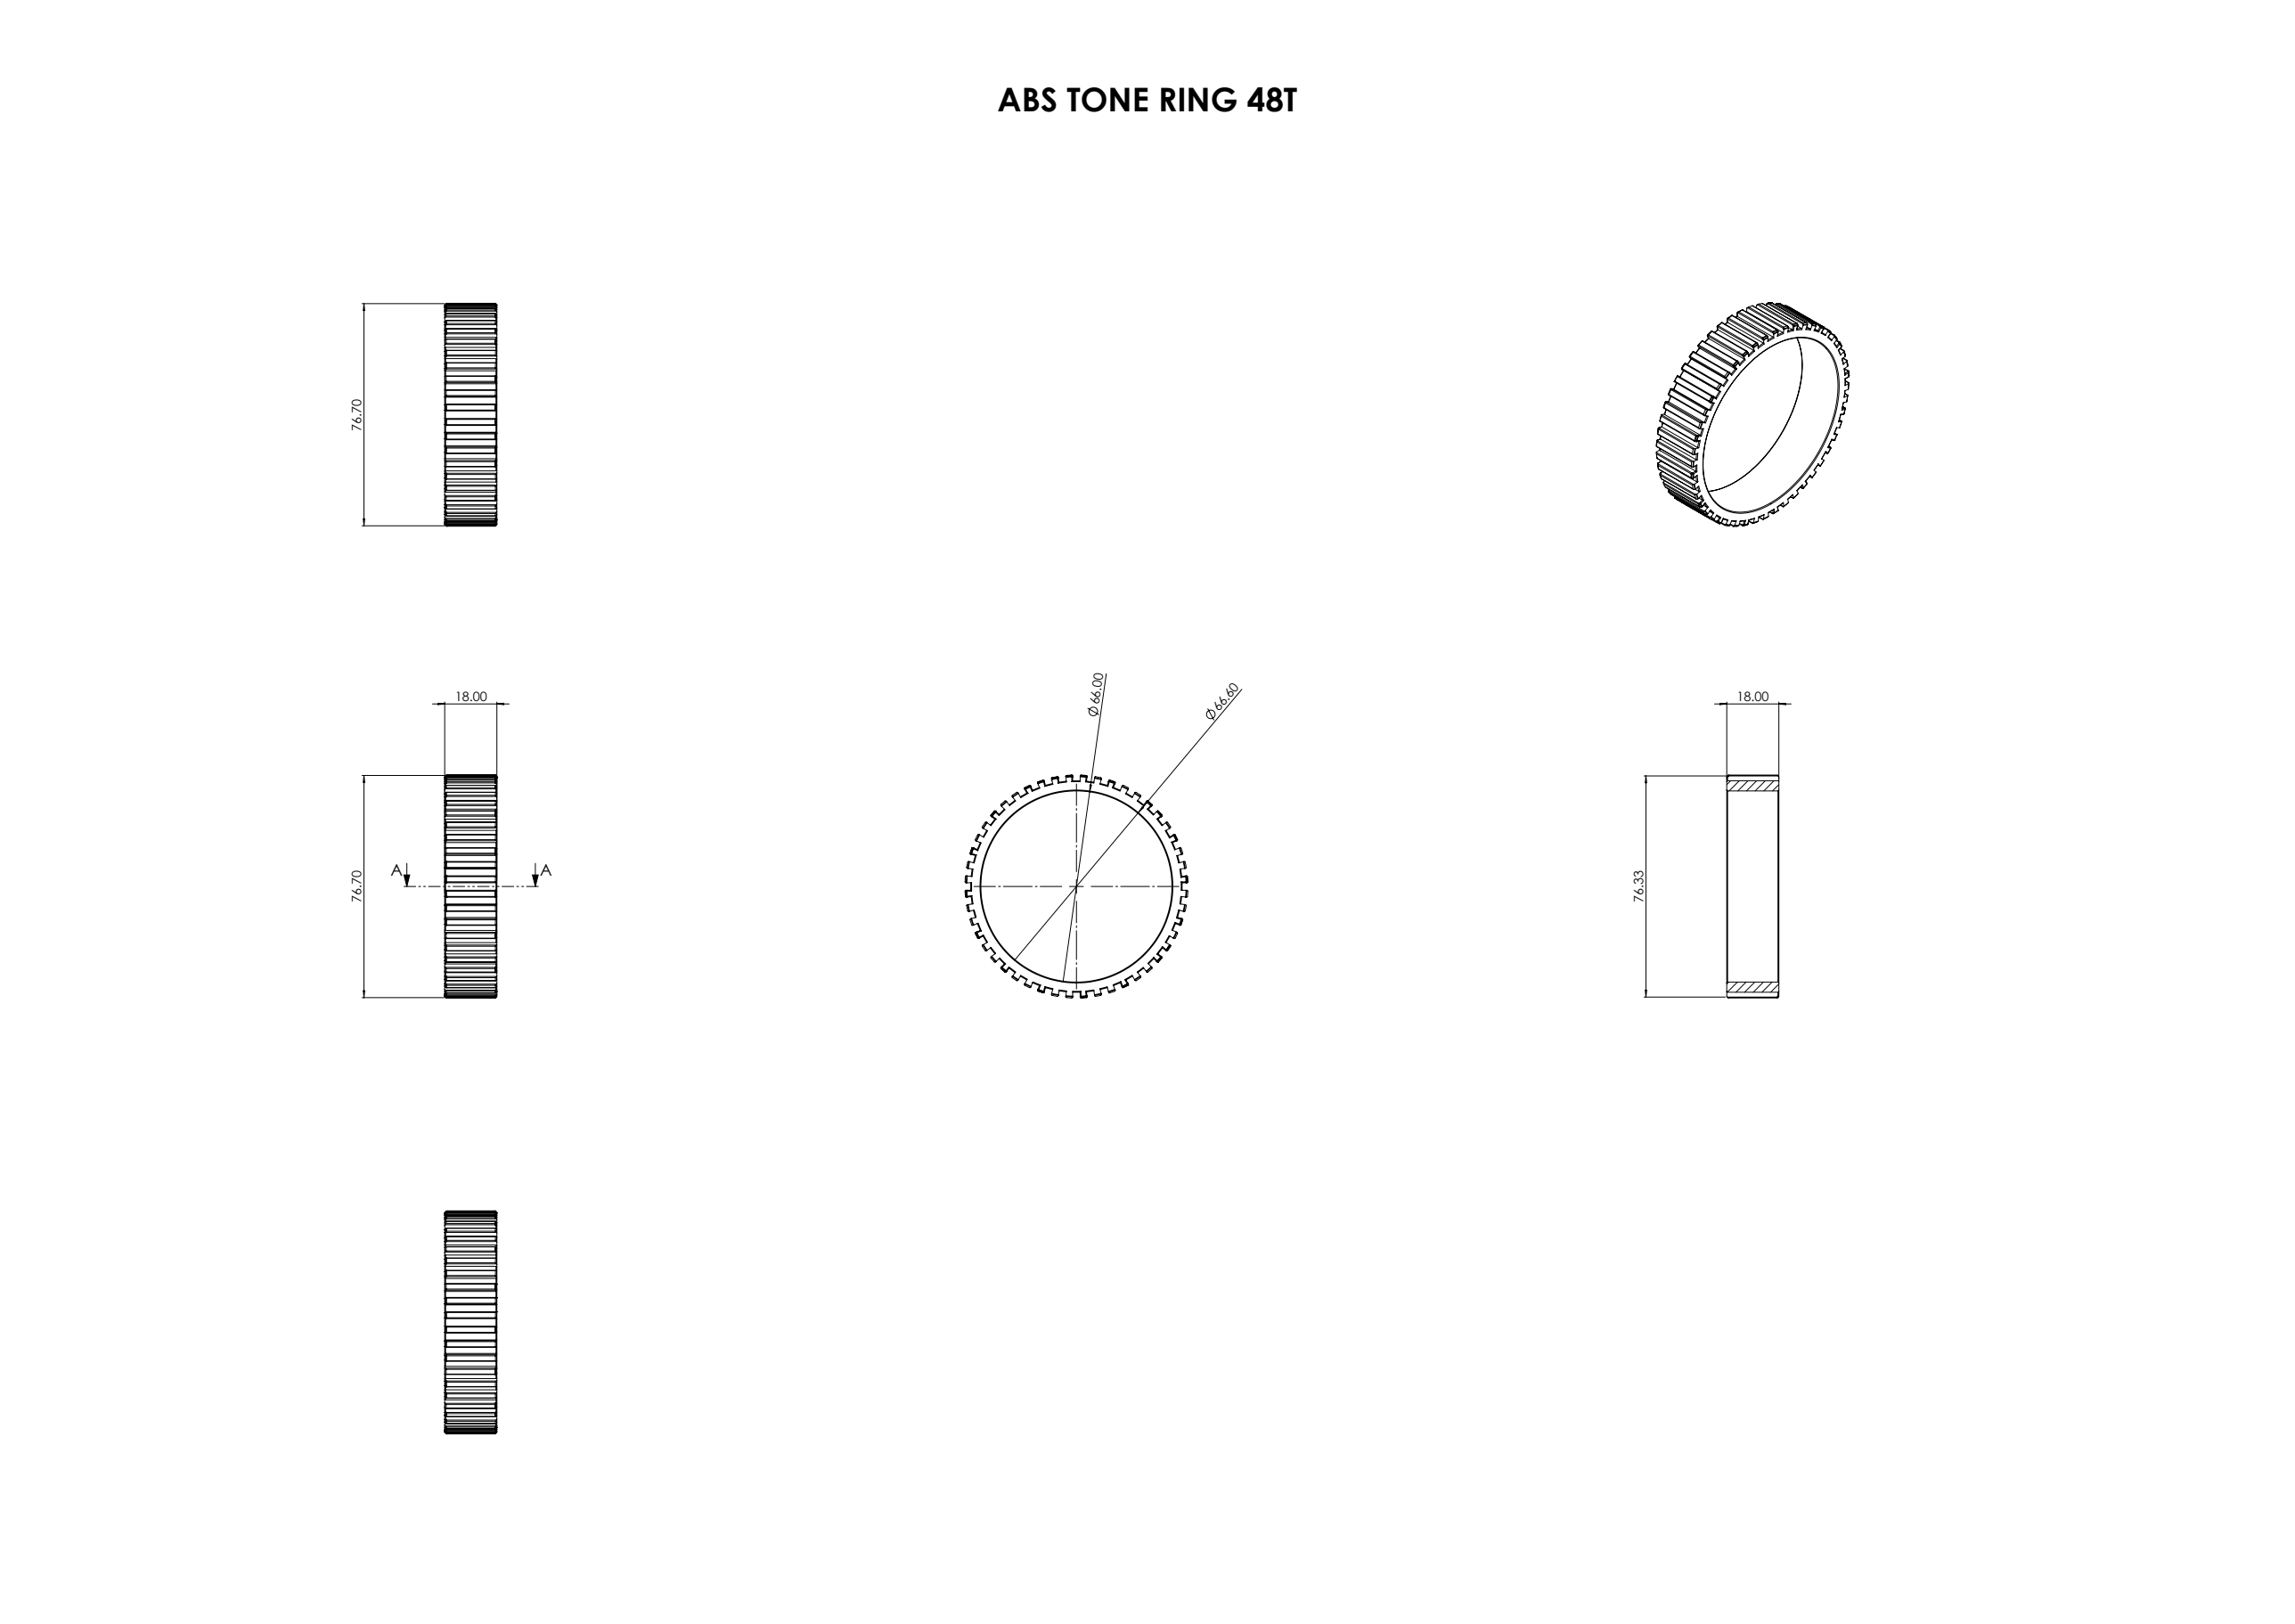
ISO-10303-21;
HEADER;
/* Generated by software containing ST-Developer
 * from STEP Tools, Inc. (www.steptools.com) 
 */

FILE_DESCRIPTION(
/* description */ (''),
/* implementation_level */ '2;1');

FILE_NAME(
/* name */ '02_ABS_Tone_Ring_48T.step',
/* time_stamp */ '2026-10-11T12:57:03-07:00',
/* author */ (''),
/* organization */ (''),
/* preprocessor_version */ 'ST-DEVELOPER v20.2',
/* originating_system */ 'Autodesk Translation Framework v15.15.0.0',
/* authorisation */ '');

FILE_SCHEMA (('AUTOMOTIVE_DESIGN { 1 0 10303 214 3 1 1 }'));
ENDSEC;

DATA;
#10=MECHANICAL_DESIGN_GEOMETRIC_PRESENTATION_REPRESENTATION('',(#257),#90374);
#111=ELLIPSE('',#40907,0.424264068711926,0.3);
#112=ELLIPSE('',#40914,0.424264068711924,0.3);
#113=ELLIPSE('',#40992,0.424264068711927,0.3);
#114=ELLIPSE('',#40999,0.424264068711929,0.3);
#115=ELLIPSE('',#41027,0.42426406871193,0.3);
#116=ELLIPSE('',#41034,0.424264068711928,0.3);
#117=ELLIPSE('',#41062,0.424264068711928,0.3);
#118=ELLIPSE('',#41077,0.424264068711929,0.3);
#119=ELLIPSE('',#41099,0.424264068711931,0.3);
#120=ELLIPSE('',#41114,0.424264068711924,0.3);
#121=ELLIPSE('',#41136,0.424264068711928,0.3);
#122=ELLIPSE('',#41205,0.424264068711926,0.3);
#123=ELLIPSE('',#41226,0.424264068711929,0.3);
#124=ELLIPSE('',#41247,0.424264068711929,0.3);
#125=ELLIPSE('',#41250,0.424264068711929,0.3);
#126=ELLIPSE('',#41280,0.424264068711931,0.3);
#127=ELLIPSE('',#41301,0.424264068711928,0.3);
#128=ELLIPSE('',#41322,0.424264068711927,0.3);
#129=ELLIPSE('',#41338,0.424264068711931,0.3);
#130=ELLIPSE('',#41341,0.424264068711928,0.3);
#131=ELLIPSE('',#41378,0.424264068711933,0.3);
#132=ELLIPSE('',#41386,0.424264068711929,0.3);
#133=ELLIPSE('',#41394,0.424264068711929,0.3);
#134=ELLIPSE('',#41417,0.424264068711928,0.3);
#135=ELLIPSE('',#41425,0.424264068711924,0.3);
#136=ELLIPSE('',#41443,0.424264068711929,0.3);
#137=ELLIPSE('',#41459,0.424264068711925,0.3);
#138=ELLIPSE('',#41468,0.424264068711925,0.3);
#139=ELLIPSE('',#41484,0.424264068711932,0.3);
#140=ELLIPSE('',#41505,0.424264068711926,0.3);
#141=ELLIPSE('',#41528,0.424264068711932,0.3);
#142=ELLIPSE('',#41536,0.424264068711931,0.3);
#143=ELLIPSE('',#41559,0.424264068711932,0.3);
#144=ELLIPSE('',#41570,0.424264068711924,0.3);
#145=ELLIPSE('',#41591,0.424264068711938,0.3);
#146=ELLIPSE('',#41612,0.424264068711929,0.3);
#147=ELLIPSE('',#41630,0.424264068711925,0.3);
#148=ELLIPSE('',#41640,0.424264068711933,0.3);
#149=ELLIPSE('',#41648,0.424264068711928,0.3);
#150=ELLIPSE('',#41671,0.424264068711924,0.3);
#151=ELLIPSE('',#41692,0.424264068711934,0.3);
#152=ELLIPSE('',#41700,0.424264068711936,0.3);
#153=ELLIPSE('',#41708,0.424264068711924,0.3);
#154=ELLIPSE('',#41726,0.424264068711933,0.3);
#155=ELLIPSE('',#41734,0.424264068711928,0.3);
#156=ELLIPSE('',#41757,0.424264068711939,0.3);
#157=ELLIPSE('',#41775,0.424264068711935,0.3);
#158=ELLIPSE('',#41784,0.424264068711927,0.3);
#159=ELLIPSE('',#41805,0.424264068711928,0.3);
#160=ELLIPSE('',#41826,0.424264068711934,0.3);
#161=ELLIPSE('',#41842,0.424264068711933,0.3);
#162=ELLIPSE('',#41865,0.424264068711929,0.3);
#163=ELLIPSE('',#41880,0.424264068711931,0.3);
#164=ELLIPSE('',#41886,0.424264068711923,0.3);
#165=ELLIPSE('',#41907,0.424264068711929,0.3);
#166=ELLIPSE('',#41925,0.424264068711927,0.3);
#167=ELLIPSE('',#41935,0.424264068711925,0.3);
#168=ELLIPSE('',#41943,0.424264068711927,0.3);
#169=ELLIPSE('',#41966,0.424264068711931,0.3);
#170=ELLIPSE('',#41977,0.424264068711927,0.3);
#171=ELLIPSE('',#41998,0.424264068711928,0.3);
#172=ELLIPSE('',#42006,0.424264068711927,0.3);
#173=ELLIPSE('',#42014,0.424264068711923,0.3);
#174=ELLIPSE('',#42037,0.42426406871193,0.3);
#175=ELLIPSE('',#42046,0.424264068711931,0.3);
#176=ELLIPSE('',#42067,0.424264068711931,0.3);
#177=ELLIPSE('',#42090,0.424264068711929,0.3);
#178=ELLIPSE('',#42098,0.424264068711927,0.3);
#179=ELLIPSE('',#42114,0.424264068711931,0.3);
#180=ELLIPSE('',#42137,0.424264068711925,0.3);
#181=ELLIPSE('',#42142,0.424264068711929,0.3);
#182=ELLIPSE('',#42165,0.424264068711925,0.3);
#183=ELLIPSE('',#42173,0.424264068711929,0.3);
#184=ELLIPSE('',#42188,0.424264068711931,0.3);
#185=ELLIPSE('',#42199,0.424264068711925,0.3);
#186=ELLIPSE('',#42209,0.424264068711925,0.3);
#187=ELLIPSE('',#42217,0.424264068711926,0.3);
#188=ELLIPSE('',#42240,0.424264068711921,0.3);
#189=ELLIPSE('',#42254,0.424264068711933,0.3);
#190=ELLIPSE('',#42275,0.424264068711929,0.3);
#191=ELLIPSE('',#42291,0.424264068711929,0.3);
#192=ELLIPSE('',#42312,0.424264068711932,0.3);
#193=ELLIPSE('',#42333,0.424264068711929,0.3);
#194=ELLIPSE('',#42356,0.424264068711932,0.3);
#195=ELLIPSE('',#42364,0.424264068711932,0.3);
#196=ELLIPSE('',#42374,0.424264068711929,0.3);
#197=ELLIPSE('',#42389,0.424264068711927,0.3);
#198=ELLIPSE('',#42404,0.424264068711929,0.3);
#199=ELLIPSE('',#42412,0.424264068711929,0.3);
#200=ELLIPSE('',#42430,0.424264068711929,0.3);
#201=ELLIPSE('',#42442,0.424264068711929,0.3);
#202=ELLIPSE('',#42454,0.424264068711927,0.3);
#203=ELLIPSE('',#42506,0.424264068711923,0.3);
#204=ELLIPSE('',#42563,0.42426406871193,0.3);
#205=ELLIPSE('',#42620,0.424264068711933,0.3);
#206=ELLIPSE('',#42643,0.424264068711929,0.3);
#207=ELLIPSE('',#42675,0.424264068711927,0.3);
#208=ELLIPSE('',#42703,0.424264068711926,0.3);
#209=ELLIPSE('',#42706,0.424264068711927,0.3);
#210=ELLIPSE('',#42748,0.42426406871193,0.3);
#223=SHAPE_REPRESENTATION_RELATIONSHIP('SRR','None',#90442,#240);
#240=ADVANCED_BREP_SHAPE_REPRESENTATION('',(#274),#90358);
#257=STYLED_ITEM('',(#90673),#274);
#274=MANIFOLD_SOLID_BREP('Body1',#40346);
#302=SPHERICAL_SURFACE('',#40910,0.3);
#303=SPHERICAL_SURFACE('',#40923,0.3);
#304=SPHERICAL_SURFACE('',#40925,0.3);
#305=SPHERICAL_SURFACE('',#40927,0.3);
#306=SPHERICAL_SURFACE('',#40995,0.3);
#307=SPHERICAL_SURFACE('',#41008,0.3);
#308=SPHERICAL_SURFACE('',#41010,0.3);
#309=SPHERICAL_SURFACE('',#41012,0.3);
#310=SPHERICAL_SURFACE('',#41030,0.3);
#311=SPHERICAL_SURFACE('',#41043,0.3);
#312=SPHERICAL_SURFACE('',#41045,0.3);
#313=SPHERICAL_SURFACE('',#41047,0.3);
#314=SPHERICAL_SURFACE('',#41065,0.3);
#315=SPHERICAL_SURFACE('',#41073,0.3);
#316=SPHERICAL_SURFACE('',#41080,0.3);
#317=SPHERICAL_SURFACE('',#41082,0.3);
#318=SPHERICAL_SURFACE('',#41102,0.3);
#319=SPHERICAL_SURFACE('',#41110,0.3);
#320=SPHERICAL_SURFACE('',#41117,0.3);
#321=SPHERICAL_SURFACE('',#41119,0.3);
#322=SPHERICAL_SURFACE('',#41139,0.3);
#323=SPHERICAL_SURFACE('',#41143,0.3);
#324=SPHERICAL_SURFACE('',#41208,0.3);
#325=SPHERICAL_SURFACE('',#41212,0.3);
#326=SPHERICAL_SURFACE('',#41229,0.3);
#327=SPHERICAL_SURFACE('',#41233,0.3);
#328=SPHERICAL_SURFACE('',#41253,0.3);
#329=SPHERICAL_SURFACE('',#41261,0.3);
#330=SPHERICAL_SURFACE('',#41265,0.3);
#331=SPHERICAL_SURFACE('',#41267,0.3);
#332=SPHERICAL_SURFACE('',#41283,0.3);
#333=SPHERICAL_SURFACE('',#41287,0.3);
#334=SPHERICAL_SURFACE('',#41304,0.3);
#335=SPHERICAL_SURFACE('',#41308,0.3);
#336=SPHERICAL_SURFACE('',#41325,0.3);
#337=SPHERICAL_SURFACE('',#41329,0.3);
#338=SPHERICAL_SURFACE('',#41344,0.3);
#339=SPHERICAL_SURFACE('',#41352,0.3);
#340=SPHERICAL_SURFACE('',#41356,0.3);
#341=SPHERICAL_SURFACE('',#41358,0.3);
#342=SPHERICAL_SURFACE('',#41374,0.3);
#343=SPHERICAL_SURFACE('',#41379,0.3);
#344=SPHERICAL_SURFACE('',#41387,0.3);
#345=SPHERICAL_SURFACE('',#41388,0.3);
#346=SPHERICAL_SURFACE('',#41397,0.3);
#347=SPHERICAL_SURFACE('',#41401,0.3);
#348=SPHERICAL_SURFACE('',#41418,0.3);
#349=SPHERICAL_SURFACE('',#41419,0.3);
#350=SPHERICAL_SURFACE('',#41428,0.3);
#351=SPHERICAL_SURFACE('',#41432,0.3);
#352=SPHERICAL_SURFACE('',#41444,0.3);
#353=SPHERICAL_SURFACE('',#41445,0.3);
#354=SPHERICAL_SURFACE('',#41455,0.3);
#355=SPHERICAL_SURFACE('',#41460,0.3);
#356=SPHERICAL_SURFACE('',#41471,0.3);
#357=SPHERICAL_SURFACE('',#41475,0.3);
#358=SPHERICAL_SURFACE('',#41487,0.3);
#359=SPHERICAL_SURFACE('',#41491,0.3);
#360=SPHERICAL_SURFACE('',#41508,0.3);
#361=SPHERICAL_SURFACE('',#41512,0.3);
#362=SPHERICAL_SURFACE('',#41529,0.3);
#363=SPHERICAL_SURFACE('',#41530,0.3);
#364=SPHERICAL_SURFACE('',#41539,0.3);
#365=SPHERICAL_SURFACE('',#41543,0.3);
#366=SPHERICAL_SURFACE('',#41560,0.3);
#367=SPHERICAL_SURFACE('',#41561,0.3);
#368=SPHERICAL_SURFACE('',#41573,0.3);
#369=SPHERICAL_SURFACE('',#41577,0.3);
#370=SPHERICAL_SURFACE('',#41594,0.3);
#371=SPHERICAL_SURFACE('',#41598,0.3);
#372=SPHERICAL_SURFACE('',#41615,0.3);
#373=SPHERICAL_SURFACE('',#41619,0.3);
#374=SPHERICAL_SURFACE('',#41631,0.3);
#375=SPHERICAL_SURFACE('',#41632,0.3);
#376=SPHERICAL_SURFACE('',#41641,0.3);
#377=SPHERICAL_SURFACE('',#41642,0.3);
#378=SPHERICAL_SURFACE('',#41651,0.3);
#379=SPHERICAL_SURFACE('',#41655,0.3);
#380=SPHERICAL_SURFACE('',#41672,0.3);
#381=SPHERICAL_SURFACE('',#41673,0.3);
#382=SPHERICAL_SURFACE('',#41688,0.3);
#383=SPHERICAL_SURFACE('',#41693,0.3);
#384=SPHERICAL_SURFACE('',#41701,0.3);
#385=SPHERICAL_SURFACE('',#41702,0.3);
#386=SPHERICAL_SURFACE('',#41711,0.3);
#387=SPHERICAL_SURFACE('',#41715,0.3);
#388=SPHERICAL_SURFACE('',#41727,0.3);
#389=SPHERICAL_SURFACE('',#41728,0.3);
#390=SPHERICAL_SURFACE('',#41737,0.3);
#391=SPHERICAL_SURFACE('',#41741,0.3);
#392=SPHERICAL_SURFACE('',#41758,0.3);
#393=SPHERICAL_SURFACE('',#41759,0.3);
#394=SPHERICAL_SURFACE('',#41771,0.3);
#395=SPHERICAL_SURFACE('',#41776,0.3);
#396=SPHERICAL_SURFACE('',#41787,0.3);
#397=SPHERICAL_SURFACE('',#41791,0.3);
#398=SPHERICAL_SURFACE('',#41808,0.3);
#399=SPHERICAL_SURFACE('',#41812,0.3);
#400=SPHERICAL_SURFACE('',#41829,0.3);
#401=SPHERICAL_SURFACE('',#41833,0.3);
#402=SPHERICAL_SURFACE('',#41845,0.3);
#403=SPHERICAL_SURFACE('',#41849,0.3);
#404=SPHERICAL_SURFACE('',#41866,0.3);
#405=SPHERICAL_SURFACE('',#41867,0.3);
#406=SPHERICAL_SURFACE('',#41876,0.3);
#407=SPHERICAL_SURFACE('',#41881,0.3);
#408=SPHERICAL_SURFACE('',#41889,0.3);
#409=SPHERICAL_SURFACE('',#41893,0.3);
#410=SPHERICAL_SURFACE('',#41910,0.3);
#411=SPHERICAL_SURFACE('',#41914,0.3);
#412=SPHERICAL_SURFACE('',#41926,0.3);
#413=SPHERICAL_SURFACE('',#41927,0.3);
#414=SPHERICAL_SURFACE('',#41936,0.3);
#415=SPHERICAL_SURFACE('',#41937,0.3);
#416=SPHERICAL_SURFACE('',#41946,0.3);
#417=SPHERICAL_SURFACE('',#41950,0.3);
#418=SPHERICAL_SURFACE('',#41967,0.3);
#419=SPHERICAL_SURFACE('',#41968,0.3);
#420=SPHERICAL_SURFACE('',#41978,0.3);
#421=SPHERICAL_SURFACE('',#41979,0.3);
#422=SPHERICAL_SURFACE('',#41994,0.3);
#423=SPHERICAL_SURFACE('',#41999,0.3);
#424=SPHERICAL_SURFACE('',#42007,0.3);
#425=SPHERICAL_SURFACE('',#42008,0.3);
#426=SPHERICAL_SURFACE('',#42017,0.3);
#427=SPHERICAL_SURFACE('',#42021,0.3);
#428=SPHERICAL_SURFACE('',#42038,0.3);
#429=SPHERICAL_SURFACE('',#42039,0.3);
#430=SPHERICAL_SURFACE('',#42049,0.3);
#431=SPHERICAL_SURFACE('',#42053,0.3);
#432=SPHERICAL_SURFACE('',#42070,0.3);
#433=SPHERICAL_SURFACE('',#42074,0.3);
#434=SPHERICAL_SURFACE('',#42091,0.3);
#435=SPHERICAL_SURFACE('',#42092,0.3);
#436=SPHERICAL_SURFACE('',#42101,0.3);
#437=SPHERICAL_SURFACE('',#42105,0.3);
#438=SPHERICAL_SURFACE('',#42117,0.3);
#439=SPHERICAL_SURFACE('',#42121,0.3);
#440=SPHERICAL_SURFACE('',#42138,0.3);
#441=SPHERICAL_SURFACE('',#42139,0.3);
#442=SPHERICAL_SURFACE('',#42145,0.3);
#443=SPHERICAL_SURFACE('',#42149,0.3);
#444=SPHERICAL_SURFACE('',#42161,0.3);
#445=SPHERICAL_SURFACE('',#42166,0.3);
#446=SPHERICAL_SURFACE('',#42174,0.3);
#447=SPHERICAL_SURFACE('',#42175,0.3);
#448=SPHERICAL_SURFACE('',#42184,0.3);
#449=SPHERICAL_SURFACE('',#42189,0.3);
#450=SPHERICAL_SURFACE('',#42200,0.3);
#451=SPHERICAL_SURFACE('',#42201,0.3);
#452=SPHERICAL_SURFACE('',#42210,0.3);
#453=SPHERICAL_SURFACE('',#42211,0.3);
#454=SPHERICAL_SURFACE('',#42220,0.3);
#455=SPHERICAL_SURFACE('',#42224,0.3);
#456=SPHERICAL_SURFACE('',#42241,0.3);
#457=SPHERICAL_SURFACE('',#42242,0.3);
#458=SPHERICAL_SURFACE('',#42257,0.3);
#459=SPHERICAL_SURFACE('',#42261,0.3);
#460=SPHERICAL_SURFACE('',#42278,0.3);
#461=SPHERICAL_SURFACE('',#42282,0.3);
#462=SPHERICAL_SURFACE('',#42294,0.3);
#463=SPHERICAL_SURFACE('',#42298,0.3);
#464=SPHERICAL_SURFACE('',#42315,0.3);
#465=SPHERICAL_SURFACE('',#42319,0.3);
#466=SPHERICAL_SURFACE('',#42336,0.3);
#467=SPHERICAL_SURFACE('',#42340,0.3);
#468=SPHERICAL_SURFACE('',#42352,0.3);
#469=SPHERICAL_SURFACE('',#42357,0.3);
#470=SPHERICAL_SURFACE('',#42365,0.3);
#471=SPHERICAL_SURFACE('',#42366,0.3);
#472=SPHERICAL_SURFACE('',#42375,0.3);
#473=SPHERICAL_SURFACE('',#42376,0.3);
#474=SPHERICAL_SURFACE('',#42385,0.3);
#475=SPHERICAL_SURFACE('',#42390,0.3);
#476=SPHERICAL_SURFACE('',#42405,0.3);
#477=SPHERICAL_SURFACE('',#42406,0.3);
#478=SPHERICAL_SURFACE('',#42415,0.3);
#479=SPHERICAL_SURFACE('',#42419,0.3);
#480=SPHERICAL_SURFACE('',#42431,0.3);
#481=SPHERICAL_SURFACE('',#42432,0.3);
#482=SPHERICAL_SURFACE('',#42438,0.3);
#483=SPHERICAL_SURFACE('',#42443,0.3);
#484=SPHERICAL_SURFACE('',#42455,0.3);
#485=SPHERICAL_SURFACE('',#42502,0.3);
#486=SPHERICAL_SURFACE('',#42507,0.3);
#487=SPHERICAL_SURFACE('',#42559,0.3);
#488=SPHERICAL_SURFACE('',#42564,0.3);
#489=SPHERICAL_SURFACE('',#42616,0.3);
#490=SPHERICAL_SURFACE('',#42621,0.3);
#491=SPHERICAL_SURFACE('',#42639,0.3);
#492=SPHERICAL_SURFACE('',#42645,0.3);
#493=SPHERICAL_SURFACE('',#42678,0.3);
#494=SPHERICAL_SURFACE('',#42686,0.3);
#495=SPHERICAL_SURFACE('',#42688,0.3);
#496=SPHERICAL_SURFACE('',#42709,0.3);
#497=SPHERICAL_SURFACE('',#42717,0.3);
#498=SPHERICAL_SURFACE('',#42721,0.3);
#499=SPHERICAL_SURFACE('',#42723,0.3);
#500=SPHERICAL_SURFACE('',#42740,0.3);
#501=SPHERICAL_SURFACE('',#42749,0.3);
#502=SPHERICAL_SURFACE('',#42750,0.3);
#503=SPHERICAL_SURFACE('',#42764,0.3);
#504=SPHERICAL_SURFACE('',#42771,0.3);
#577=CONICAL_SURFACE('',#40984,38.25,0.785398163397462);
#578=CONICAL_SURFACE('',#41019,38.25,0.785398163397462);
#579=CONICAL_SURFACE('',#41054,38.25,0.785398163397462);
#580=CONICAL_SURFACE('',#41088,38.25,0.785398163397462);
#581=CONICAL_SURFACE('',#41125,38.25,0.785398163397462);
#582=CONICAL_SURFACE('',#41196,38.25,0.785398163397462);
#583=CONICAL_SURFACE('',#41217,38.25,0.785398163397462);
#584=CONICAL_SURFACE('',#41238,38.25,0.785398163397462);
#585=CONICAL_SURFACE('',#41277,38.25,0.785398163397462);
#586=CONICAL_SURFACE('',#41292,38.25,0.785398163397462);
#587=CONICAL_SURFACE('',#41313,38.25,0.785398163397462);
#588=CONICAL_SURFACE('',#41334,38.25,0.785398163397462);
#589=CONICAL_SURFACE('',#41368,38.25,0.785398163397462);
#590=CONICAL_SURFACE('',#41406,38.25,0.785398163397462);
#591=CONICAL_SURFACE('',#41437,38.25,0.785398163397462);
#592=CONICAL_SURFACE('',#41480,38.25,0.785398163397462);
#593=CONICAL_SURFACE('',#41496,38.25,0.785398163397462);
#594=CONICAL_SURFACE('',#41517,38.25,0.785398163397462);
#595=CONICAL_SURFACE('',#41548,38.25,0.785398163397462);
#596=CONICAL_SURFACE('',#41582,38.25,0.785398163397462);
#597=CONICAL_SURFACE('',#41603,38.25,0.785398163397462);
#598=CONICAL_SURFACE('',#41624,38.25,0.785398163397462);
#599=CONICAL_SURFACE('',#41660,38.25,0.785398163397462);
#600=CONICAL_SURFACE('',#41720,38.25,0.785398163397462);
#601=CONICAL_SURFACE('',#41746,38.25,0.785398163397462);
#602=CONICAL_SURFACE('',#41796,38.25,0.785398163397462);
#603=CONICAL_SURFACE('',#41817,38.25,0.785398163397462);
#604=CONICAL_SURFACE('',#41838,38.25,0.785398163397462);
#605=CONICAL_SURFACE('',#41854,38.25,0.785398163397462);
#606=CONICAL_SURFACE('',#41898,38.25,0.785398163397462);
#607=CONICAL_SURFACE('',#41919,38.25,0.785398163397462);
#608=CONICAL_SURFACE('',#41955,38.25,0.785398163397462);
#609=CONICAL_SURFACE('',#42026,38.25,0.785398163397462);
#610=CONICAL_SURFACE('',#42058,38.25,0.785398163397462);
#611=CONICAL_SURFACE('',#42079,38.25,0.785398163397462);
#612=CONICAL_SURFACE('',#42110,38.25,0.785398163397462);
#613=CONICAL_SURFACE('',#42126,38.25,0.785398163397462);
#614=CONICAL_SURFACE('',#42154,38.25,0.785398163397462);
#615=CONICAL_SURFACE('',#42229,38.25,0.785398163397462);
#616=CONICAL_SURFACE('',#42266,38.25,0.785398163397462);
#617=CONICAL_SURFACE('',#42287,38.25,0.785398163397462);
#618=CONICAL_SURFACE('',#42303,38.25,0.785398163397462);
#619=CONICAL_SURFACE('',#42324,38.25,0.785398163397462);
#620=CONICAL_SURFACE('',#42345,38.25,0.785398163397462);
#621=CONICAL_SURFACE('',#42394,38.25,0.785398163397462);
#622=CONICAL_SURFACE('',#42424,38.25,0.785398163397462);
#623=CONICAL_SURFACE('',#42693,38.25,0.785398163397462);
#624=CONICAL_SURFACE('',#42733,38.25,0.785398163397462);
#625=CONICAL_SURFACE('',#42741,38.25,0.785398163397462);
#626=CONICAL_SURFACE('',#42772,38.25,0.785398163397462);
#627=CONICAL_SURFACE('',#42775,38.25,0.785398163397462);
#628=CONICAL_SURFACE('',#42924,38.25,0.785398163397462);
#629=CONICAL_SURFACE('',#42927,38.25,0.785398163397462);
#630=CONICAL_SURFACE('',#42930,38.25,0.785398163397462);
#631=CONICAL_SURFACE('',#42931,38.25,0.785398163397462);
#632=CONICAL_SURFACE('',#42932,38.25,0.785398163397462);
#633=CONICAL_SURFACE('',#42935,38.25,0.785398163397462);
#634=CONICAL_SURFACE('',#42936,38.25,0.785398163397462);
#635=CONICAL_SURFACE('',#42937,38.25,0.785398163397462);
#636=CONICAL_SURFACE('',#42940,38.25,0.785398163397462);
#637=CONICAL_SURFACE('',#42941,38.25,0.785398163397462);
#638=CONICAL_SURFACE('',#42942,38.25,0.785398163397462);
#639=CONICAL_SURFACE('',#42943,38.25,0.785398163397462);
#640=CONICAL_SURFACE('',#42944,38.25,0.785398163397462);
#641=CONICAL_SURFACE('',#42945,38.25,0.785398163397462);
#642=CONICAL_SURFACE('',#42948,38.25,0.785398163397462);
#643=CONICAL_SURFACE('',#42949,38.25,0.785398163397462);
#644=CONICAL_SURFACE('',#42950,38.25,0.785398163397462);
#645=CONICAL_SURFACE('',#42953,38.25,0.785398163397462);
#646=CONICAL_SURFACE('',#42954,38.25,0.785398163397462);
#647=CONICAL_SURFACE('',#42955,38.25,0.785398163397462);
#648=CONICAL_SURFACE('',#42958,38.25,0.785398163397462);
#649=CONICAL_SURFACE('',#42959,38.25,0.785398163397462);
#650=CONICAL_SURFACE('',#42960,38.25,0.785398163397462);
#651=CONICAL_SURFACE('',#42961,38.25,0.785398163397462);
#652=CONICAL_SURFACE('',#42962,38.25,0.785398163397462);
#653=CONICAL_SURFACE('',#42963,38.25,0.785398163397462);
#654=CONICAL_SURFACE('',#42966,38.25,0.785398163397462);
#655=CONICAL_SURFACE('',#42967,38.25,0.785398163397462);
#656=CONICAL_SURFACE('',#42968,38.25,0.785398163397462);
#657=CONICAL_SURFACE('',#42971,38.25,0.785398163397462);
#658=CONICAL_SURFACE('',#42972,38.25,0.785398163397462);
#659=CONICAL_SURFACE('',#42973,38.25,0.785398163397462);
#660=CONICAL_SURFACE('',#42976,38.25,0.785398163397462);
#661=CONICAL_SURFACE('',#42977,38.25,0.785398163397462);
#662=CONICAL_SURFACE('',#42978,38.25,0.785398163397462);
#663=CONICAL_SURFACE('',#42979,38.25,0.785398163397462);
#664=CONICAL_SURFACE('',#42980,38.25,0.785398163397462);
#665=CONICAL_SURFACE('',#42981,38.25,0.785398163397462);
#666=CONICAL_SURFACE('',#42984,38.25,0.785398163397462);
#667=CONICAL_SURFACE('',#42985,38.25,0.785398163397462);
#668=CONICAL_SURFACE('',#42986,38.25,0.785398163397462);
#669=CONICAL_SURFACE('',#42989,38.25,0.785398163397462);
#670=CONICAL_SURFACE('',#42990,38.25,0.785398163397462);
#671=CONICAL_SURFACE('',#42991,38.25,0.785398163397462);
#672=CONICAL_SURFACE('',#42996,38.25,0.785398163397462);
#801=TOROIDAL_SURFACE('',#40915,38.2,0.3);
#802=TOROIDAL_SURFACE('',#40981,37.8757359312881,0.3);
#803=TOROIDAL_SURFACE('',#40986,38.2,0.3);
#804=TOROIDAL_SURFACE('',#41000,38.2,0.3);
#805=TOROIDAL_SURFACE('',#41016,37.8757359312881,0.3);
#806=TOROIDAL_SURFACE('',#41021,38.2,0.3);
#807=TOROIDAL_SURFACE('',#41035,38.2,0.3);
#808=TOROIDAL_SURFACE('',#41051,37.8757359312881,0.3);
#809=TOROIDAL_SURFACE('',#41056,38.2,0.3);
#810=TOROIDAL_SURFACE('',#41067,38.2,0.3);
#811=TOROIDAL_SURFACE('',#41084,37.8757359312881,0.3);
#812=TOROIDAL_SURFACE('',#41090,38.2,0.3);
#813=TOROIDAL_SURFACE('',#41104,38.2,0.3);
#814=TOROIDAL_SURFACE('',#41121,37.8757359312881,0.3);
#815=TOROIDAL_SURFACE('',#41127,38.2,0.3);
#816=TOROIDAL_SURFACE('',#41193,37.8757359312881,0.3);
#817=TOROIDAL_SURFACE('',#41198,38.2,0.3);
#818=TOROIDAL_SURFACE('',#41214,37.8757359312881,0.3);
#819=TOROIDAL_SURFACE('',#41219,38.2,0.3);
#820=TOROIDAL_SURFACE('',#41235,37.8757359312881,0.3);
#821=TOROIDAL_SURFACE('',#41240,38.2,0.3);
#822=TOROIDAL_SURFACE('',#41255,38.2,0.3);
#823=TOROIDAL_SURFACE('',#41275,37.8757359312881,0.3);
#824=TOROIDAL_SURFACE('',#41289,37.8757359312881,0.3);
#825=TOROIDAL_SURFACE('',#41294,38.2,0.3);
#826=TOROIDAL_SURFACE('',#41310,37.8757359312881,0.3);
#827=TOROIDAL_SURFACE('',#41315,38.2,0.3);
#828=TOROIDAL_SURFACE('',#41331,37.8757359312881,0.3);
#829=TOROIDAL_SURFACE('',#41346,38.2,0.3);
#830=TOROIDAL_SURFACE('',#41366,37.8757359312881,0.3);
#831=TOROIDAL_SURFACE('',#41371,38.2,0.3);
#832=TOROIDAL_SURFACE('',#41403,37.8757359312881,0.3);
#833=TOROIDAL_SURFACE('',#41408,38.2,0.3);
#834=TOROIDAL_SURFACE('',#41434,37.8757359312881,0.3);
#835=TOROIDAL_SURFACE('',#41452,38.2,0.3);
#836=TOROIDAL_SURFACE('',#41477,37.8757359312881,0.3);
#837=TOROIDAL_SURFACE('',#41493,37.8757359312881,0.3);
#838=TOROIDAL_SURFACE('',#41498,38.2,0.3);
#839=TOROIDAL_SURFACE('',#41514,37.8757359312881,0.3);
#840=TOROIDAL_SURFACE('',#41519,38.2,0.3);
#841=TOROIDAL_SURFACE('',#41545,37.8757359312881,0.3);
#842=TOROIDAL_SURFACE('',#41550,38.2,0.3);
#843=TOROIDAL_SURFACE('',#41579,37.8757359312881,0.3);
#844=TOROIDAL_SURFACE('',#41584,38.2,0.3);
#845=TOROIDAL_SURFACE('',#41600,37.8757359312881,0.3);
#846=TOROIDAL_SURFACE('',#41605,38.2,0.3);
#847=TOROIDAL_SURFACE('',#41621,37.8757359312881,0.3);
#848=TOROIDAL_SURFACE('',#41657,37.8757359312881,0.3);
#849=TOROIDAL_SURFACE('',#41662,38.2,0.3);
#850=TOROIDAL_SURFACE('',#41685,38.2,0.3);
#851=TOROIDAL_SURFACE('',#41717,37.8757359312881,0.3);
#852=TOROIDAL_SURFACE('',#41743,37.8757359312881,0.3);
#853=TOROIDAL_SURFACE('',#41748,38.2,0.3);
#854=TOROIDAL_SURFACE('',#41768,38.2,0.3);
#855=TOROIDAL_SURFACE('',#41793,37.8757359312881,0.3);
#856=TOROIDAL_SURFACE('',#41798,38.2,0.3);
#857=TOROIDAL_SURFACE('',#41814,37.8757359312881,0.3);
#858=TOROIDAL_SURFACE('',#41819,38.2,0.3);
#859=TOROIDAL_SURFACE('',#41835,37.8757359312881,0.3);
#860=TOROIDAL_SURFACE('',#41851,37.8757359312881,0.3);
#861=TOROIDAL_SURFACE('',#41856,38.2,0.3);
#862=TOROIDAL_SURFACE('',#41873,38.2,0.3);
#863=TOROIDAL_SURFACE('',#41895,37.8757359312881,0.3);
#864=TOROIDAL_SURFACE('',#41900,38.2,0.3);
#865=TOROIDAL_SURFACE('',#41916,37.8757359312881,0.3);
#866=TOROIDAL_SURFACE('',#41952,37.8757359312881,0.3);
#867=TOROIDAL_SURFACE('',#41957,38.2,0.3);
#868=TOROIDAL_SURFACE('',#41991,38.2,0.3);
#869=TOROIDAL_SURFACE('',#42023,37.8757359312881,0.3);
#870=TOROIDAL_SURFACE('',#42028,38.2,0.3);
#871=TOROIDAL_SURFACE('',#42055,37.8757359312881,0.3);
#872=TOROIDAL_SURFACE('',#42060,38.2,0.3);
#873=TOROIDAL_SURFACE('',#42076,37.8757359312881,0.3);
#874=TOROIDAL_SURFACE('',#42081,38.2,0.3);
#875=TOROIDAL_SURFACE('',#42107,37.8757359312881,0.3);
#876=TOROIDAL_SURFACE('',#42123,37.8757359312881,0.3);
#877=TOROIDAL_SURFACE('',#42128,38.2,0.3);
#878=TOROIDAL_SURFACE('',#42151,37.8757359312881,0.3);
#879=TOROIDAL_SURFACE('',#42158,38.2,0.3);
#880=TOROIDAL_SURFACE('',#42181,38.2,0.3);
#881=TOROIDAL_SURFACE('',#42226,37.8757359312881,0.3);
#882=TOROIDAL_SURFACE('',#42231,38.2,0.3);
#883=TOROIDAL_SURFACE('',#42263,37.8757359312881,0.3);
#884=TOROIDAL_SURFACE('',#42268,38.2,0.3);
#885=TOROIDAL_SURFACE('',#42284,37.8757359312881,0.3);
#886=TOROIDAL_SURFACE('',#42300,37.8757359312881,0.3);
#887=TOROIDAL_SURFACE('',#42305,38.2,0.3);
#888=TOROIDAL_SURFACE('',#42321,37.8757359312881,0.3);
#889=TOROIDAL_SURFACE('',#42326,38.2,0.3);
#890=TOROIDAL_SURFACE('',#42342,37.8757359312881,0.3);
#891=TOROIDAL_SURFACE('',#42349,38.2,0.3);
#892=TOROIDAL_SURFACE('',#42382,38.2,0.3);
#893=TOROIDAL_SURFACE('',#42421,37.8757359312881,0.3);
#894=TOROIDAL_SURFACE('',#42435,38.2,0.3);
#895=TOROIDAL_SURFACE('',#42449,37.8757359312881,0.3);
#896=TOROIDAL_SURFACE('',#42459,37.8757359312881,0.3);
#897=TOROIDAL_SURFACE('',#42468,37.8757359312881,0.3);
#898=TOROIDAL_SURFACE('',#42472,37.8757359312881,0.3);
#899=TOROIDAL_SURFACE('',#42478,37.8757359312881,0.3);
#900=TOROIDAL_SURFACE('',#42485,37.8757359312881,0.3);
#901=TOROIDAL_SURFACE('',#42491,37.8757359312881,0.3);
#902=TOROIDAL_SURFACE('',#42495,37.8757359312881,0.3);
#903=TOROIDAL_SURFACE('',#42511,37.8757359312881,0.3);
#904=TOROIDAL_SURFACE('',#42515,37.8757359312881,0.3);
#905=TOROIDAL_SURFACE('',#42524,37.8757359312881,0.3);
#906=TOROIDAL_SURFACE('',#42529,37.8757359312881,0.3);
#907=TOROIDAL_SURFACE('',#42535,37.8757359312881,0.3);
#908=TOROIDAL_SURFACE('',#42542,37.8757359312881,0.3);
#909=TOROIDAL_SURFACE('',#42548,37.8757359312881,0.3);
#910=TOROIDAL_SURFACE('',#42552,37.8757359312881,0.3);
#911=TOROIDAL_SURFACE('',#42568,37.8757359312881,0.3);
#912=TOROIDAL_SURFACE('',#42573,37.8757359312881,0.3);
#913=TOROIDAL_SURFACE('',#42582,37.8757359312881,0.3);
#914=TOROIDAL_SURFACE('',#42586,37.8757359312881,0.3);
#915=TOROIDAL_SURFACE('',#42592,37.8757359312881,0.3);
#916=TOROIDAL_SURFACE('',#42599,37.8757359312881,0.3);
#917=TOROIDAL_SURFACE('',#42605,37.8757359312881,0.3);
#918=TOROIDAL_SURFACE('',#42609,37.8757359312881,0.3);
#919=TOROIDAL_SURFACE('',#42625,37.8757359312881,0.3);
#920=TOROIDAL_SURFACE('',#42629,37.8757359312881,0.3);
#921=TOROIDAL_SURFACE('',#42636,38.2,0.3);
#922=TOROIDAL_SURFACE('',#42650,37.8757359312881,0.3);
#923=TOROIDAL_SURFACE('',#42654,37.8757359312881,0.3);
#924=TOROIDAL_SURFACE('',#42660,37.8757359312881,0.3);
#925=TOROIDAL_SURFACE('',#42667,37.8757359312881,0.3);
#926=TOROIDAL_SURFACE('',#42682,38.2,0.3);
#927=TOROIDAL_SURFACE('',#42690,37.8757359312881,0.3);
#928=TOROIDAL_SURFACE('',#42695,38.2,0.3);
#929=TOROIDAL_SURFACE('',#42711,38.2,0.3);
#930=TOROIDAL_SURFACE('',#42731,37.8757359312881,0.3);
#931=TOROIDAL_SURFACE('',#42734,37.8757359312881,0.3);
#932=TOROIDAL_SURFACE('',#42737,38.2,0.3);
#933=TOROIDAL_SURFACE('',#42751,33.3,0.3);
#934=TOROIDAL_SURFACE('',#42758,37.8757359312881,0.3);
#935=TOROIDAL_SURFACE('',#42761,38.2,0.3);
#936=TOROIDAL_SURFACE('',#42765,37.8757359312881,0.3);
#937=TOROIDAL_SURFACE('',#42768,38.2,0.3);
#938=TOROIDAL_SURFACE('',#42778,33.3,0.3);
#939=TOROIDAL_SURFACE('',#42792,37.8757359312881,0.3);
#940=TOROIDAL_SURFACE('',#42802,37.8757359312881,0.3);
#941=TOROIDAL_SURFACE('',#42810,37.8757359312881,0.3);
#942=TOROIDAL_SURFACE('',#42819,37.8757359312881,0.3);
#943=TOROIDAL_SURFACE('',#42827,37.8757359312881,0.3);
#944=TOROIDAL_SURFACE('',#42835,37.8757359312881,0.3);
#945=TOROIDAL_SURFACE('',#42843,37.8757359312881,0.3);
#946=TOROIDAL_SURFACE('',#42852,37.8757359312881,0.3);
#947=TOROIDAL_SURFACE('',#42860,37.8757359312881,0.3);
#948=TOROIDAL_SURFACE('',#42870,37.8757359312881,0.3);
#949=TOROIDAL_SURFACE('',#42879,37.8757359312881,0.3);
#950=TOROIDAL_SURFACE('',#42887,37.8757359312881,0.3);
#951=TOROIDAL_SURFACE('',#42895,37.8757359312881,0.3);
#952=TOROIDAL_SURFACE('',#42905,37.8757359312881,0.3);
#953=TOROIDAL_SURFACE('',#42913,37.8757359312881,0.3);
#954=TOROIDAL_SURFACE('',#42916,37.8757359312881,0.3);
#1047=FACE_BOUND('',#4779,.T.);
#1048=FACE_BOUND('',#4852,.T.);
#1156=PLANE('',#40929);
#1157=PLANE('',#40931);
#1158=PLANE('',#41014);
#1159=PLANE('',#41049);
#1160=PLANE('',#41096);
#1161=PLANE('',#41133);
#1162=PLANE('',#41145);
#1163=PLANE('',#41273);
#1164=PLANE('',#41364);
#1165=PLANE('',#41380);
#1166=PLANE('',#41390);
#1167=PLANE('',#41421);
#1168=PLANE('',#41448);
#1169=PLANE('',#41461);
#1170=PLANE('',#41464);
#1171=PLANE('',#41532);
#1172=PLANE('',#41563);
#1173=PLANE('',#41566);
#1174=PLANE('',#41634);
#1175=PLANE('',#41644);
#1176=PLANE('',#41675);
#1177=PLANE('',#41678);
#1178=PLANE('',#41681);
#1179=PLANE('',#41694);
#1180=PLANE('',#41704);
#1181=PLANE('',#41730);
#1182=PLANE('',#41761);
#1183=PLANE('',#41764);
#1184=PLANE('',#41777);
#1185=PLANE('',#41780);
#1186=PLANE('',#41869);
#1187=PLANE('',#41882);
#1188=PLANE('',#41929);
#1189=PLANE('',#41939);
#1190=PLANE('',#41971);
#1191=PLANE('',#41981);
#1192=PLANE('',#41984);
#1193=PLANE('',#41987);
#1194=PLANE('',#42000);
#1195=PLANE('',#42010);
#1196=PLANE('',#42042);
#1197=PLANE('',#42094);
#1198=PLANE('',#42167);
#1199=PLANE('',#42177);
#1200=PLANE('',#42190);
#1201=PLANE('',#42193);
#1202=PLANE('',#42203);
#1203=PLANE('',#42213);
#1204=PLANE('',#42244);
#1205=PLANE('',#42247);
#1206=PLANE('',#42250);
#1207=PLANE('',#42358);
#1208=PLANE('',#42368);
#1209=PLANE('',#42378);
#1210=PLANE('',#42391);
#1211=PLANE('',#42397);
#1212=PLANE('',#42408);
#1213=PLANE('',#42444);
#1214=PLANE('',#42447);
#1215=PLANE('',#42458);
#1216=PLANE('',#42462);
#1217=PLANE('',#42463);
#1218=PLANE('',#42466);
#1219=PLANE('',#42471);
#1220=PLANE('',#42475);
#1221=PLANE('',#42476);
#1222=PLANE('',#42481);
#1223=PLANE('',#42483);
#1224=PLANE('',#42488);
#1225=PLANE('',#42489);
#1226=PLANE('',#42494);
#1227=PLANE('',#42498);
#1228=PLANE('',#42509);
#1229=PLANE('',#42510);
#1230=PLANE('',#42514);
#1231=PLANE('',#42518);
#1232=PLANE('',#42519);
#1233=PLANE('',#42522);
#1234=PLANE('',#42528);
#1235=PLANE('',#42532);
#1236=PLANE('',#42533);
#1237=PLANE('',#42538);
#1238=PLANE('',#42540);
#1239=PLANE('',#42545);
#1240=PLANE('',#42546);
#1241=PLANE('',#42551);
#1242=PLANE('',#42555);
#1243=PLANE('',#42566);
#1244=PLANE('',#42567);
#1245=PLANE('',#42572);
#1246=PLANE('',#42576);
#1247=PLANE('',#42577);
#1248=PLANE('',#42580);
#1249=PLANE('',#42585);
#1250=PLANE('',#42589);
#1251=PLANE('',#42590);
#1252=PLANE('',#42595);
#1253=PLANE('',#42597);
#1254=PLANE('',#42602);
#1255=PLANE('',#42603);
#1256=PLANE('',#42608);
#1257=PLANE('',#42612);
#1258=PLANE('',#42623);
#1259=PLANE('',#42624);
#1260=PLANE('',#42628);
#1261=PLANE('',#42632);
#1262=PLANE('',#42646);
#1263=PLANE('',#42648);
#1264=PLANE('',#42653);
#1265=PLANE('',#42657);
#1266=PLANE('',#42658);
#1267=PLANE('',#42663);
#1268=PLANE('',#42666);
#1269=PLANE('',#42670);
#1270=PLANE('',#42671);
#1271=PLANE('',#42729);
#1272=PLANE('',#42742);
#1273=PLANE('',#42774);
#1274=PLANE('',#42777);
#1275=PLANE('',#42782);
#1276=PLANE('',#42790);
#1277=PLANE('',#42796);
#1278=PLANE('',#42800);
#1279=PLANE('',#42808);
#1280=PLANE('',#42813);
#1281=PLANE('',#42817);
#1282=PLANE('',#42825);
#1283=PLANE('',#42833);
#1284=PLANE('',#42841);
#1285=PLANE('',#42846);
#1286=PLANE('',#42850);
#1287=PLANE('',#42858);
#1288=PLANE('',#42864);
#1289=PLANE('',#42868);
#1290=PLANE('',#42873);
#1291=PLANE('',#42877);
#1292=PLANE('',#42885);
#1293=PLANE('',#42893);
#1294=PLANE('',#42899);
#1295=PLANE('',#42903);
#1296=PLANE('',#42911);
#1297=PLANE('',#42917);
#1298=PLANE('',#42921);
#1299=PLANE('',#42994);
#1300=PLANE('',#42995);
#1301=PLANE('',#42997);
#1980=B_SPLINE_SURFACE_WITH_KNOTS('',3,3,((#68026,#68027,#68028,#68029),
(#68030,#68031,#68032,#68033),(#68034,#68035,#68036,#68037),(#68038,#68039,
#68040,#68041),(#68042,#68043,#68044,#68045)),.UNSPECIFIED.,.F.,.F.,.F.,
(4,1,4),(4,4),(0.,0.5,1.),(0.,0.0458781805670868),.UNSPECIFIED.);
#1981=B_SPLINE_SURFACE_WITH_KNOTS('',3,3,((#68102,#68103,#68104,#68105),
(#68106,#68107,#68108,#68109),(#68110,#68111,#68112,#68113),(#68114,#68115,
#68116,#68117),(#68118,#68119,#68120,#68121)),.UNSPECIFIED.,.F.,.F.,.F.,
(4,1,4),(4,4),(0.,0.5,1.),(0.,0.0458781805664131),.UNSPECIFIED.);
#1982=B_SPLINE_SURFACE_WITH_KNOTS('',3,3,((#68622,#68623,#68624,#68625),
(#68626,#68627,#68628,#68629),(#68630,#68631,#68632,#68633),(#68634,#68635,
#68636,#68637),(#68638,#68639,#68640,#68641)),.UNSPECIFIED.,.F.,.F.,.F.,
(4,1,4),(4,4),(0.,0.5,1.),(0.,0.0458781805670811),.UNSPECIFIED.);
#1983=B_SPLINE_SURFACE_WITH_KNOTS('',3,3,((#68698,#68699,#68700,#68701),
(#68702,#68703,#68704,#68705),(#68706,#68707,#68708,#68709),(#68710,#68711,
#68712,#68713),(#68714,#68715,#68716,#68717)),.UNSPECIFIED.,.F.,.F.,.F.,
(4,1,4),(4,4),(0.,0.5,1.),(0.,0.0458781805664166),.UNSPECIFIED.);
#1984=B_SPLINE_SURFACE_WITH_KNOTS('',3,3,((#68774,#68775,#68776,#68777),
(#68778,#68779,#68780,#68781),(#68782,#68783,#68784,#68785),(#68786,#68787,
#68788,#68789),(#68790,#68791,#68792,#68793)),.UNSPECIFIED.,.F.,.F.,.F.,
(4,1,4),(4,4),(0.,0.5,1.),(0.,0.0458781805670864),.UNSPECIFIED.);
#1985=B_SPLINE_SURFACE_WITH_KNOTS('',3,3,((#68850,#68851,#68852,#68853),
(#68854,#68855,#68856,#68857),(#68858,#68859,#68860,#68861),(#68862,#68863,
#68864,#68865),(#68866,#68867,#68868,#68869)),.UNSPECIFIED.,.F.,.F.,.F.,
(4,1,4),(4,4),(0.,0.5,1.),(0.,0.0458781805664115),.UNSPECIFIED.);
#1986=B_SPLINE_SURFACE_WITH_KNOTS('',3,3,((#68929,#68930,#68931,#68932),
(#68933,#68934,#68935,#68936),(#68937,#68938,#68939,#68940),(#68941,#68942,
#68943,#68944),(#68945,#68946,#68947,#68948)),.UNSPECIFIED.,.F.,.F.,.F.,
(4,1,4),(4,4),(0.,0.5,1.),(0.,0.0458781805671252),.UNSPECIFIED.);
#1987=B_SPLINE_SURFACE_WITH_KNOTS('',3,3,((#69004,#69005,#69006,#69007),
(#69008,#69009,#69010,#69011),(#69012,#69013,#69014,#69015),(#69016,#69017,
#69018,#69019),(#69020,#69021,#69022,#69023)),.UNSPECIFIED.,.F.,.F.,.F.,
(4,1,4),(4,4),(0.,0.5,1.),(0.,0.0458781805667822),.UNSPECIFIED.);
#1988=B_SPLINE_SURFACE_WITH_KNOTS('',3,3,((#69081,#69082,#69083,#69084),
(#69085,#69086,#69087,#69088),(#69089,#69090,#69091,#69092),(#69093,#69094,
#69095,#69096),(#69097,#69098,#69099,#69100)),.UNSPECIFIED.,.F.,.F.,.F.,
(4,1,4),(4,4),(0.,0.5,1.),(0.,0.0458781805671229),.UNSPECIFIED.);
#1989=B_SPLINE_SURFACE_WITH_KNOTS('',3,3,((#69156,#69157,#69158,#69159),
(#69160,#69161,#69162,#69163),(#69164,#69165,#69166,#69167),(#69168,#69169,
#69170,#69171),(#69172,#69173,#69174,#69175)),.UNSPECIFIED.,.F.,.F.,.F.,
(4,1,4),(4,4),(0.,0.5,1.),(0.,0.0458781805667724),.UNSPECIFIED.);
#1990=B_SPLINE_SURFACE_WITH_KNOTS('',3,3,((#69233,#69234,#69235,#69236),
(#69237,#69238,#69239,#69240),(#69241,#69242,#69243,#69244),(#69245,#69246,
#69247,#69248),(#69249,#69250,#69251,#69252)),.UNSPECIFIED.,.F.,.F.,.F.,
(4,1,4),(4,4),(0.,0.5,1.),(0.,0.045878180567128),.UNSPECIFIED.);
#1991=B_SPLINE_SURFACE_WITH_KNOTS('',3,3,((#69672,#69673,#69674,#69675),
(#69676,#69677,#69678,#69679),(#69680,#69681,#69682,#69683),(#69684,#69685,
#69686,#69687),(#69688,#69689,#69690,#69691)),.UNSPECIFIED.,.F.,.F.,.F.,
(4,1,4),(4,4),(0.,0.5,1.),(0.,0.0458781805671024),.UNSPECIFIED.);
#1992=B_SPLINE_SURFACE_WITH_KNOTS('',3,3,((#69755,#69756,#69757,#69758),
(#69759,#69760,#69761,#69762),(#69763,#69764,#69765,#69766),(#69767,#69768,
#69769,#69770),(#69771,#69772,#69773,#69774)),.UNSPECIFIED.,.F.,.F.,.F.,
(4,1,4),(4,4),(0.,0.5,1.),(0.,0.0458781805671248),.UNSPECIFIED.);
#1993=B_SPLINE_SURFACE_WITH_KNOTS('',3,3,((#69844,#69845,#69846,#69847),
(#69848,#69849,#69850,#69851),(#69852,#69853,#69854,#69855),(#69856,#69857,
#69858,#69859),(#69860,#69861,#69862,#69863)),.UNSPECIFIED.,.F.,.F.,.F.,
(4,1,4),(4,4),(0.,0.5,1.),(0.,0.0458781805671046),.UNSPECIFIED.);
#1994=B_SPLINE_SURFACE_WITH_KNOTS('',3,3,((#69913,#69914,#69915,#69916),
(#69917,#69918,#69919,#69920),(#69921,#69922,#69923,#69924),(#69925,#69926,
#69927,#69928),(#69929,#69930,#69931,#69932)),.UNSPECIFIED.,.F.,.F.,.F.,
(4,1,4),(4,4),(0.,0.5,1.),(0.,0.0458781805666752),.UNSPECIFIED.);
#1995=B_SPLINE_SURFACE_WITH_KNOTS('',3,3,((#69982,#69983,#69984,#69985),
(#69986,#69987,#69988,#69989),(#69990,#69991,#69992,#69993),(#69994,#69995,
#69996,#69997),(#69998,#69999,#70000,#70001)),.UNSPECIFIED.,.F.,.F.,.F.,
(4,1,4),(4,4),(0.,0.5,1.),(0.,0.0458781805671212),.UNSPECIFIED.);
#1996=B_SPLINE_SURFACE_WITH_KNOTS('',3,3,((#70065,#70066,#70067,#70068),
(#70069,#70070,#70071,#70072),(#70073,#70074,#70075,#70076),(#70077,#70078,
#70079,#70080),(#70081,#70082,#70083,#70084)),.UNSPECIFIED.,.F.,.F.,.F.,
(4,1,4),(4,4),(0.,0.5,1.),(0.,0.0458781805671206),.UNSPECIFIED.);
#1997=B_SPLINE_SURFACE_WITH_KNOTS('',3,3,((#70148,#70149,#70150,#70151),
(#70152,#70153,#70154,#70155),(#70156,#70157,#70158,#70159),(#70160,#70161,
#70162,#70163),(#70164,#70165,#70166,#70167)),.UNSPECIFIED.,.F.,.F.,.F.,
(4,1,4),(4,4),(0.,0.5,1.),(0.,0.0458781805671124),.UNSPECIFIED.);
#1998=B_SPLINE_SURFACE_WITH_KNOTS('',3,3,((#70229,#70230,#70231,#70232),
(#70233,#70234,#70235,#70236),(#70237,#70238,#70239,#70240),(#70241,#70242,
#70243,#70244),(#70245,#70246,#70247,#70248)),.UNSPECIFIED.,.F.,.F.,.F.,
(4,1,4),(4,4),(0.,0.5,1.),(0.,0.0458781805670977),.UNSPECIFIED.);
#1999=B_SPLINE_SURFACE_WITH_KNOTS('',3,3,((#70298,#70299,#70300,#70301),
(#70302,#70303,#70304,#70305),(#70306,#70307,#70308,#70309),(#70310,#70311,
#70312,#70313),(#70314,#70315,#70316,#70317)),.UNSPECIFIED.,.F.,.F.,.F.,
(4,1,4),(4,4),(0.,0.5,1.),(0.,0.0458781805665702),.UNSPECIFIED.);
#2000=B_SPLINE_SURFACE_WITH_KNOTS('',3,3,((#70361,#70362,#70363,#70364),
(#70365,#70366,#70367,#70368),(#70369,#70370,#70371,#70372),(#70373,#70374,
#70375,#70376),(#70377,#70378,#70379,#70380)),.UNSPECIFIED.,.F.,.F.,.F.,
(4,1,4),(4,4),(0.,0.5,1.),(0.,0.0458781805667346),.UNSPECIFIED.);
#2001=B_SPLINE_SURFACE_WITH_KNOTS('',3,3,((#70413,#70414,#70415,#70416),
(#70417,#70418,#70419,#70420),(#70421,#70422,#70423,#70424),(#70425,#70426,
#70427,#70428),(#70429,#70430,#70431,#70432)),.UNSPECIFIED.,.F.,.F.,.F.,
(4,1,4),(4,4),(0.,0.5,1.),(0.,0.045878180566734),.UNSPECIFIED.);
#2002=B_SPLINE_SURFACE_WITH_KNOTS('',3,3,((#70467,#70468,#70469,#70470),
(#70471,#70472,#70473,#70474),(#70475,#70476,#70477,#70478),(#70479,#70480,
#70481,#70482),(#70483,#70484,#70485,#70486)),.UNSPECIFIED.,.F.,.F.,.F.,
(4,1,4),(4,4),(0.,0.5,1.),(0.,0.0458781805670993),.UNSPECIFIED.);
#2003=B_SPLINE_SURFACE_WITH_KNOTS('',3,3,((#70544,#70545,#70546,#70547),
(#70548,#70549,#70550,#70551),(#70552,#70553,#70554,#70555),(#70556,#70557,
#70558,#70559),(#70560,#70561,#70562,#70563)),.UNSPECIFIED.,.F.,.F.,.F.,
(4,1,4),(4,4),(0.,0.5,1.),(0.,0.0458781805667679),.UNSPECIFIED.);
#2004=B_SPLINE_SURFACE_WITH_KNOTS('',3,3,((#70598,#70599,#70600,#70601),
(#70602,#70603,#70604,#70605),(#70606,#70607,#70608,#70609),(#70610,#70611,
#70612,#70613),(#70614,#70615,#70616,#70617)),.UNSPECIFIED.,.F.,.F.,.F.,
(4,1,4),(4,4),(0.,0.5,1.),(0.,0.0458781805671254),.UNSPECIFIED.);
#2005=B_SPLINE_SURFACE_WITH_KNOTS('',3,3,((#70667,#70668,#70669,#70670),
(#70671,#70672,#70673,#70674),(#70675,#70676,#70677,#70678),(#70679,#70680,
#70681,#70682),(#70683,#70684,#70685,#70686)),.UNSPECIFIED.,.F.,.F.,.F.,
(4,1,4),(4,4),(0.,0.5,1.),(0.,0.0458781805667828),.UNSPECIFIED.);
#2006=B_SPLINE_SURFACE_WITH_KNOTS('',3,3,((#70732,#70733,#70734,#70735),
(#70736,#70737,#70738,#70739),(#70740,#70741,#70742,#70743),(#70744,#70745,
#70746,#70747),(#70748,#70749,#70750,#70751)),.UNSPECIFIED.,.F.,.F.,.F.,
(4,1,4),(4,4),(0.,0.5,1.),(0.,0.04587818056678),.UNSPECIFIED.);
#2007=B_SPLINE_SURFACE_WITH_KNOTS('',3,3,((#70819,#70820,#70821,#70822),
(#70823,#70824,#70825,#70826),(#70827,#70828,#70829,#70830),(#70831,#70832,
#70833,#70834),(#70835,#70836,#70837,#70838)),.UNSPECIFIED.,.F.,.F.,.F.,
(4,1,4),(4,4),(0.,0.5,1.),(0.,0.0458781805671173),.UNSPECIFIED.);
#2008=B_SPLINE_SURFACE_WITH_KNOTS('',3,3,((#70894,#70895,#70896,#70897),
(#70898,#70899,#70900,#70901),(#70902,#70903,#70904,#70905),(#70906,#70907,
#70908,#70909),(#70910,#70911,#70912,#70913)),.UNSPECIFIED.,.F.,.F.,.F.,
(4,1,4),(4,4),(0.,0.5,1.),(0.,0.0458781805671103),.UNSPECIFIED.);
#2009=B_SPLINE_SURFACE_WITH_KNOTS('',3,3,((#70977,#70978,#70979,#70980),
(#70981,#70982,#70983,#70984),(#70985,#70986,#70987,#70988),(#70989,#70990,
#70991,#70992),(#70993,#70994,#70995,#70996)),.UNSPECIFIED.,.F.,.F.,.F.,
(4,1,4),(4,4),(0.,0.5,1.),(0.,0.0458781805671206),.UNSPECIFIED.);
#2010=B_SPLINE_SURFACE_WITH_KNOTS('',3,3,((#71054,#71055,#71056,#71057),
(#71058,#71059,#71060,#71061),(#71062,#71063,#71064,#71065),(#71066,#71067,
#71068,#71069),(#71070,#71071,#71072,#71073)),.UNSPECIFIED.,.F.,.F.,.F.,
(4,1,4),(4,4),(0.,0.5,1.),(0.,0.0458781805665721),.UNSPECIFIED.);
#2011=B_SPLINE_SURFACE_WITH_KNOTS('',3,3,((#71108,#71109,#71110,#71111),
(#71112,#71113,#71114,#71115),(#71116,#71117,#71118,#71119),(#71120,#71121,
#71122,#71123),(#71124,#71125,#71126,#71127)),.UNSPECIFIED.,.F.,.F.,.F.,
(4,1,4),(4,4),(0.,0.5,1.),(0.,0.0458781805671148),.UNSPECIFIED.);
#2012=B_SPLINE_SURFACE_WITH_KNOTS('',3,3,((#71185,#71186,#71187,#71188),
(#71189,#71190,#71191,#71192),(#71193,#71194,#71195,#71196),(#71197,#71198,
#71199,#71200),(#71201,#71202,#71203,#71204)),.UNSPECIFIED.,.F.,.F.,.F.,
(4,1,4),(4,4),(0.,0.5,1.),(0.,0.0458781805667336),.UNSPECIFIED.);
#2013=B_SPLINE_SURFACE_WITH_KNOTS('',3,3,((#71268,#71269,#71270,#71271),
(#71272,#71273,#71274,#71275),(#71276,#71277,#71278,#71279),(#71280,#71281,
#71282,#71283),(#71284,#71285,#71286,#71287)),.UNSPECIFIED.,.F.,.F.,.F.,
(4,1,4),(4,4),(0.,0.5,1.),(0.,0.0458781805671248),.UNSPECIFIED.);
#2014=B_SPLINE_SURFACE_WITH_KNOTS('',3,3,((#71351,#71352,#71353,#71354),
(#71355,#71356,#71357,#71358),(#71359,#71360,#71361,#71362),(#71363,#71364,
#71365,#71366),(#71367,#71368,#71369,#71370)),.UNSPECIFIED.,.F.,.F.,.F.,
(4,1,4),(4,4),(0.,0.5,1.),(0.,0.0458781805671175),.UNSPECIFIED.);
#2015=B_SPLINE_SURFACE_WITH_KNOTS('',3,3,((#71434,#71435,#71436,#71437),
(#71438,#71439,#71440,#71441),(#71442,#71443,#71444,#71445),(#71446,#71447,
#71448,#71449),(#71450,#71451,#71452,#71453)),.UNSPECIFIED.,.F.,.F.,.F.,
(4,1,4),(4,4),(0.,0.5,1.),(0.,0.0458781805671191),.UNSPECIFIED.);
#2016=B_SPLINE_SURFACE_WITH_KNOTS('',3,3,((#71503,#71504,#71505,#71506),
(#71507,#71508,#71509,#71510),(#71511,#71512,#71513,#71514),(#71515,#71516,
#71517,#71518),(#71519,#71520,#71521,#71522)),.UNSPECIFIED.,.F.,.F.,.F.,
(4,1,4),(4,4),(0.,0.5,1.),(0.,0.0458781805665616),.UNSPECIFIED.);
#2017=B_SPLINE_SURFACE_WITH_KNOTS('',3,3,((#71551,#71552,#71553,#71554),
(#71555,#71556,#71557,#71558),(#71559,#71560,#71561,#71562),(#71563,#71564,
#71565,#71566),(#71567,#71568,#71569,#71570)),.UNSPECIFIED.,.F.,.F.,.F.,
(4,1,4),(4,4),(0.,0.5,1.),(0.,0.045878180566425),.UNSPECIFIED.);
#2018=B_SPLINE_SURFACE_WITH_KNOTS('',3,3,((#71605,#71606,#71607,#71608),
(#71609,#71610,#71611,#71612),(#71613,#71614,#71615,#71616),(#71617,#71618,
#71619,#71620),(#71621,#71622,#71623,#71624)),.UNSPECIFIED.,.F.,.F.,.F.,
(4,1,4),(4,4),(0.,0.5,1.),(0.,0.0458781805670893),.UNSPECIFIED.);
#2019=B_SPLINE_SURFACE_WITH_KNOTS('',3,3,((#71682,#71683,#71684,#71685),
(#71686,#71687,#71688,#71689),(#71690,#71691,#71692,#71693),(#71694,#71695,
#71696,#71697),(#71698,#71699,#71700,#71701)),.UNSPECIFIED.,.F.,.F.,.F.,
(4,1,4),(4,4),(0.,0.5,1.),(0.,0.0458781805664109),.UNSPECIFIED.);
#2020=B_SPLINE_SURFACE_WITH_KNOTS('',3,3,((#71788,#71789,#71790,#71791),
(#71792,#71793,#71794,#71795),(#71796,#71797,#71798,#71799),(#71800,#71801,
#71802,#71803),(#71804,#71805,#71806,#71807)),.UNSPECIFIED.,.F.,.F.,.F.,
(4,1,4),(4,4),(0.,0.5,1.),(0.,0.0458781805667294),.UNSPECIFIED.);
#2021=B_SPLINE_SURFACE_WITH_KNOTS('',3,3,((#71840,#71841,#71842,#71843),
(#71844,#71845,#71846,#71847),(#71848,#71849,#71850,#71851),(#71852,#71853,
#71854,#71855),(#71856,#71857,#71858,#71859)),.UNSPECIFIED.,.F.,.F.,.F.,
(4,1,4),(4,4),(0.,0.5,1.),(0.,0.0458781805667752),.UNSPECIFIED.);
#2022=B_SPLINE_SURFACE_WITH_KNOTS('',3,3,((#71894,#71895,#71896,#71897),
(#71898,#71899,#71900,#71901),(#71902,#71903,#71904,#71905),(#71906,#71907,
#71908,#71909),(#71910,#71911,#71912,#71913)),.UNSPECIFIED.,.F.,.F.,.F.,
(4,1,4),(4,4),(0.,0.5,1.),(0.,0.0458781805671226),.UNSPECIFIED.);
#2023=B_SPLINE_SURFACE_WITH_KNOTS('',3,3,((#71963,#71964,#71965,#71966),
(#71967,#71968,#71969,#71970),(#71971,#71972,#71973,#71974),(#71975,#71976,
#71977,#71978),(#71979,#71980,#71981,#71982)),.UNSPECIFIED.,.F.,.F.,.F.,
(4,1,4),(4,4),(0.,0.5,1.),(0.,0.0458781805667819),.UNSPECIFIED.);
#2024=B_SPLINE_SURFACE_WITH_KNOTS('',3,3,((#72017,#72018,#72019,#72020),
(#72021,#72022,#72023,#72024),(#72025,#72026,#72027,#72028),(#72029,#72030,
#72031,#72032),(#72033,#72034,#72035,#72036)),.UNSPECIFIED.,.F.,.F.,.F.,
(4,1,4),(4,4),(0.,0.5,1.),(0.,0.0458781805671222),.UNSPECIFIED.);
#2025=B_SPLINE_SURFACE_WITH_KNOTS('',3,3,((#72094,#72095,#72096,#72097),
(#72098,#72099,#72100,#72101),(#72102,#72103,#72104,#72105),(#72106,#72107,
#72108,#72109),(#72110,#72111,#72112,#72113)),.UNSPECIFIED.,.F.,.F.,.F.,
(4,1,4),(4,4),(0.,0.5,1.),(0.,0.0458781805667355),.UNSPECIFIED.);
#2026=B_SPLINE_SURFACE_WITH_KNOTS('',3,3,((#72171,#72172,#72173,#72174),
(#72175,#72176,#72177,#72178),(#72179,#72180,#72181,#72182),(#72183,#72184,
#72185,#72186),(#72187,#72188,#72189,#72190)),.UNSPECIFIED.,.F.,.F.,.F.,
(4,1,4),(4,4),(0.,0.5,1.),(0.,0.0458781805667781),.UNSPECIFIED.);
#2027=B_SPLINE_SURFACE_WITH_KNOTS('',3,3,((#72258,#72259,#72260,#72261),
(#72262,#72263,#72264,#72265),(#72266,#72267,#72268,#72269),(#72270,#72271,
#72272,#72273),(#72274,#72275,#72276,#72277)),.UNSPECIFIED.,.F.,.F.,.F.,
(4,1,4),(4,4),(0.,0.5,1.),(0.,0.045878180567112),.UNSPECIFIED.);
#2028=B_SPLINE_SURFACE_WITH_KNOTS('',3,3,((#72341,#72342,#72343,#72344),
(#72345,#72346,#72347,#72348),(#72349,#72350,#72351,#72352),(#72353,#72354,
#72355,#72356),(#72357,#72358,#72359,#72360)),.UNSPECIFIED.,.F.,.F.,.F.,
(4,1,4),(4,4),(0.,0.5,1.),(0.,0.0458781805671177),.UNSPECIFIED.);
#2029=B_SPLINE_SURFACE_WITH_KNOTS('',3,3,((#72424,#72425,#72426,#72427),
(#72428,#72429,#72430,#72431),(#72432,#72433,#72434,#72435),(#72436,#72437,
#72438,#72439),(#72440,#72441,#72442,#72443)),.UNSPECIFIED.,.F.,.F.,.F.,
(4,1,4),(4,4),(0.,0.5,1.),(0.,0.0458781805671118),.UNSPECIFIED.);
#2030=B_SPLINE_SURFACE_WITH_KNOTS('',3,3,((#72499,#72500,#72501,#72502),
(#72503,#72504,#72505,#72506),(#72507,#72508,#72509,#72510),(#72511,#72512,
#72513,#72514),(#72515,#72516,#72517,#72518)),.UNSPECIFIED.,.F.,.F.,.F.,
(4,1,4),(4,4),(0.,0.5,1.),(0.,0.0458781805671198),.UNSPECIFIED.);
#2031=B_SPLINE_SURFACE_WITH_KNOTS('',3,3,((#72576,#72577,#72578,#72579),
(#72580,#72581,#72582,#72583),(#72584,#72585,#72586,#72587),(#72588,#72589,
#72590,#72591),(#72592,#72593,#72594,#72595)),.UNSPECIFIED.,.F.,.F.,.F.,
(4,1,4),(4,4),(0.,0.5,1.),(0.,0.0458781805667331),.UNSPECIFIED.);
#2032=B_SPLINE_SURFACE_WITH_KNOTS('',3,3,((#72624,#72625,#72626,#72627),
(#72628,#72629,#72630,#72631),(#72632,#72633,#72634,#72635),(#72636,#72637,
#72638,#72639),(#72640,#72641,#72642,#72643)),.UNSPECIFIED.,.F.,.F.,.F.,
(4,1,4),(4,4),(0.,0.5,1.),(0.,0.0458781805665584),.UNSPECIFIED.);
#2033=B_SPLINE_SURFACE_WITH_KNOTS('',3,3,((#72682,#72683,#72684,#72685),
(#72686,#72687,#72688,#72689),(#72690,#72691,#72692,#72693),(#72694,#72695,
#72696,#72697),(#72698,#72699,#72700,#72701)),.UNSPECIFIED.,.F.,.F.,.F.,
(4,1,4),(4,4),(0.,0.5,1.),(0.,0.0458781805671227),.UNSPECIFIED.);
#2034=B_SPLINE_SURFACE_WITH_KNOTS('',3,3,((#72765,#72766,#72767,#72768),
(#72769,#72770,#72771,#72772),(#72773,#72774,#72775,#72776),(#72777,#72778,
#72779,#72780),(#72781,#72782,#72783,#72784)),.UNSPECIFIED.,.F.,.F.,.F.,
(4,1,4),(4,4),(0.,0.5,1.),(0.,0.0458781805671102),.UNSPECIFIED.);
#2035=B_SPLINE_SURFACE_WITH_KNOTS('',3,3,((#72834,#72835,#72836,#72837),
(#72838,#72839,#72840,#72841),(#72842,#72843,#72844,#72845),(#72846,#72847,
#72848,#72849),(#72850,#72851,#72852,#72853)),.UNSPECIFIED.,.F.,.F.,.F.,
(4,1,4),(4,4),(0.,0.5,1.),(0.,0.0458781805665577),.UNSPECIFIED.);
#2036=B_SPLINE_SURFACE_WITH_KNOTS('',3,3,((#72882,#72883,#72884,#72885),
(#72886,#72887,#72888,#72889),(#72890,#72891,#72892,#72893),(#72894,#72895,
#72896,#72897),(#72898,#72899,#72900,#72901)),.UNSPECIFIED.,.F.,.F.,.F.,
(4,1,4),(4,4),(0.,0.5,1.),(0.,0.0458781805664203),.UNSPECIFIED.);
#2037=B_SPLINE_SURFACE_WITH_KNOTS('',3,3,((#72936,#72937,#72938,#72939),
(#72940,#72941,#72942,#72943),(#72944,#72945,#72946,#72947),(#72948,#72949,
#72950,#72951),(#72952,#72953,#72954,#72955)),.UNSPECIFIED.,.F.,.F.,.F.,
(4,1,4),(4,4),(0.,0.5,1.),(0.,0.0458781805670802),.UNSPECIFIED.);
#2038=B_SPLINE_SURFACE_WITH_KNOTS('',3,3,((#73013,#73014,#73015,#73016),
(#73017,#73018,#73019,#73020),(#73021,#73022,#73023,#73024),(#73025,#73026,
#73027,#73028),(#73029,#73030,#73031,#73032)),.UNSPECIFIED.,.F.,.F.,.F.,
(4,1,4),(4,4),(0.,0.5,1.),(0.,0.0458781805665695),.UNSPECIFIED.);
#2039=B_SPLINE_SURFACE_WITH_KNOTS('',3,3,((#73078,#73079,#73080,#73081),
(#73082,#73083,#73084,#73085),(#73086,#73087,#73088,#73089),(#73090,#73091,
#73092,#73093),(#73094,#73095,#73096,#73097)),.UNSPECIFIED.,.F.,.F.,.F.,
(4,1,4),(4,4),(0.,0.5,1.),(0.,0.0458781805664058),.UNSPECIFIED.);
#2040=B_SPLINE_SURFACE_WITH_KNOTS('',3,3,((#73184,#73185,#73186,#73187),
(#73188,#73189,#73190,#73191),(#73192,#73193,#73194,#73195),(#73196,#73197,
#73198,#73199),(#73200,#73201,#73202,#73203)),.UNSPECIFIED.,.F.,.F.,.F.,
(4,1,4),(4,4),(0.,0.5,1.),(0.,0.0458781805667336),.UNSPECIFIED.);
#2041=B_SPLINE_SURFACE_WITH_KNOTS('',3,3,((#73236,#73237,#73238,#73239),
(#73240,#73241,#73242,#73243),(#73244,#73245,#73246,#73247),(#73248,#73249,
#73250,#73251),(#73252,#73253,#73254,#73255)),.UNSPECIFIED.,.F.,.F.,.F.,
(4,1,4),(4,4),(0.,0.5,1.),(0.,0.0458781805667359),.UNSPECIFIED.);
#2042=B_SPLINE_SURFACE_WITH_KNOTS('',3,3,((#73290,#73291,#73292,#73293),
(#73294,#73295,#73296,#73297),(#73298,#73299,#73300,#73301),(#73302,#73303,
#73304,#73305),(#73306,#73307,#73308,#73309)),.UNSPECIFIED.,.F.,.F.,.F.,
(4,1,4),(4,4),(0.,0.5,1.),(0.,0.0458781805670993),.UNSPECIFIED.);
#2043=B_SPLINE_SURFACE_WITH_KNOTS('',3,3,((#73367,#73368,#73369,#73370),
(#73371,#73372,#73373,#73374),(#73375,#73376,#73377,#73378),(#73379,#73380,
#73381,#73382),(#73383,#73384,#73385,#73386)),.UNSPECIFIED.,.F.,.F.,.F.,
(4,1,4),(4,4),(0.,0.5,1.),(0.,0.0458781805667874),.UNSPECIFIED.);
#2044=B_SPLINE_SURFACE_WITH_KNOTS('',3,3,((#73438,#73439,#73440,#73441),
(#73442,#73443,#73444,#73445),(#73446,#73447,#73448,#73449),(#73450,#73451,
#73452,#73453),(#73454,#73455,#73456,#73457)),.UNSPECIFIED.,.F.,.F.,.F.,
(4,1,4),(4,4),(0.,0.5,1.),(0.,0.0458781805671104),.UNSPECIFIED.);
#2045=B_SPLINE_SURFACE_WITH_KNOTS('',3,3,((#73521,#73522,#73523,#73524),
(#73525,#73526,#73527,#73528),(#73529,#73530,#73531,#73532),(#73533,#73534,
#73535,#73536),(#73537,#73538,#73539,#73540)),.UNSPECIFIED.,.F.,.F.,.F.,
(4,1,4),(4,4),(0.,0.5,1.),(0.,0.0458781805671196),.UNSPECIFIED.);
#2046=B_SPLINE_SURFACE_WITH_KNOTS('',3,3,((#73598,#73599,#73600,#73601),
(#73602,#73603,#73604,#73605),(#73606,#73607,#73608,#73609),(#73610,#73611,
#73612,#73613),(#73614,#73615,#73616,#73617)),.UNSPECIFIED.,.F.,.F.,.F.,
(4,1,4),(4,4),(0.,0.5,1.),(0.,0.0458781805665721),.UNSPECIFIED.);
#2047=B_SPLINE_SURFACE_WITH_KNOTS('',3,3,((#73652,#73653,#73654,#73655),
(#73656,#73657,#73658,#73659),(#73660,#73661,#73662,#73663),(#73664,#73665,
#73666,#73667),(#73668,#73669,#73670,#73671)),.UNSPECIFIED.,.F.,.F.,.F.,
(4,1,4),(4,4),(0.,0.5,1.),(0.,0.0458781805671142),.UNSPECIFIED.);
#2048=B_SPLINE_SURFACE_WITH_KNOTS('',3,3,((#73727,#73728,#73729,#73730),
(#73731,#73732,#73733,#73734),(#73735,#73736,#73737,#73738),(#73739,#73740,
#73741,#73742),(#73743,#73744,#73745,#73746)),.UNSPECIFIED.,.F.,.F.,.F.,
(4,1,4),(4,4),(0.,0.5,1.),(0.,0.0458781805671177),.UNSPECIFIED.);
#2049=B_SPLINE_SURFACE_WITH_KNOTS('',3,3,((#73804,#73805,#73806,#73807),
(#73808,#73809,#73810,#73811),(#73812,#73813,#73814,#73815),(#73816,#73817,
#73818,#73819),(#73820,#73821,#73822,#73823)),.UNSPECIFIED.,.F.,.F.,.F.,
(4,1,4),(4,4),(0.,0.5,1.),(0.,0.0458781805667679),.UNSPECIFIED.);
#2050=B_SPLINE_SURFACE_WITH_KNOTS('',3,3,((#73837,#73838,#73839,#73840),
(#73841,#73842,#73843,#73844),(#73845,#73846,#73847,#73848),(#73849,#73850,
#73851,#73852),(#73853,#73854,#73855,#73856)),.UNSPECIFIED.,.F.,.F.,.F.,
(4,1,4),(4,4),(0.,0.5,1.),(0.,0.04587818056712),.UNSPECIFIED.);
#2051=B_SPLINE_SURFACE_WITH_KNOTS('',3,3,((#73906,#73907,#73908,#73909),
(#73910,#73911,#73912,#73913),(#73914,#73915,#73916,#73917),(#73918,#73919,
#73920,#73921),(#73922,#73923,#73924,#73925)),.UNSPECIFIED.,.F.,.F.,.F.,
(4,1,4),(4,4),(0.,0.5,1.),(0.,0.0458781805667838),.UNSPECIFIED.);
#2052=B_SPLINE_SURFACE_WITH_KNOTS('',3,3,((#73958,#73959,#73960,#73961),
(#73962,#73963,#73964,#73965),(#73966,#73967,#73968,#73969),(#73970,#73971,
#73972,#73973),(#73974,#73975,#73976,#73977)),.UNSPECIFIED.,.F.,.F.,.F.,
(4,1,4),(4,4),(0.,0.5,1.),(0.,0.0458781805667322),.UNSPECIFIED.);
#2053=B_SPLINE_SURFACE_WITH_KNOTS('',3,3,((#74006,#74007,#74008,#74009),
(#74010,#74011,#74012,#74013),(#74014,#74015,#74016,#74017),(#74018,#74019,
#74020,#74021),(#74022,#74023,#74024,#74025)),.UNSPECIFIED.,.F.,.F.,.F.,
(4,1,4),(4,4),(0.,0.5,1.),(0.,0.0458781805665558),.UNSPECIFIED.);
#2054=B_SPLINE_SURFACE_WITH_KNOTS('',3,3,((#74087,#74088,#74089,#74090),
(#74091,#74092,#74093,#74094),(#74095,#74096,#74097,#74098),(#74099,#74100,
#74101,#74102),(#74103,#74104,#74105,#74106)),.UNSPECIFIED.,.F.,.F.,.F.,
(4,1,4),(4,4),(0.,0.5,1.),(0.,0.0458781805665626),.UNSPECIFIED.);
#2055=B_SPLINE_SURFACE_WITH_KNOTS('',3,3,((#74135,#74136,#74137,#74138),
(#74139,#74140,#74141,#74142),(#74143,#74144,#74145,#74146),(#74147,#74148,
#74149,#74150),(#74151,#74152,#74153,#74154)),.UNSPECIFIED.,.F.,.F.,.F.,
(4,1,4),(4,4),(0.,0.5,1.),(0.,0.0458781805664257),.UNSPECIFIED.);
#2056=B_SPLINE_SURFACE_WITH_KNOTS('',3,3,((#74189,#74190,#74191,#74192),
(#74193,#74194,#74195,#74196),(#74197,#74198,#74199,#74200),(#74201,#74202,
#74203,#74204),(#74205,#74206,#74207,#74208)),.UNSPECIFIED.,.F.,.F.,.F.,
(4,1,4),(4,4),(0.,0.5,1.),(0.,0.0458781805670871),.UNSPECIFIED.);
#2057=B_SPLINE_SURFACE_WITH_KNOTS('',3,3,((#74266,#74267,#74268,#74269),
(#74270,#74271,#74272,#74273),(#74274,#74275,#74276,#74277),(#74278,#74279,
#74280,#74281),(#74282,#74283,#74284,#74285)),.UNSPECIFIED.,.F.,.F.,.F.,
(4,1,4),(4,4),(0.,0.5,1.),(0.,0.0458781805664109),.UNSPECIFIED.);
#2058=B_SPLINE_SURFACE_WITH_KNOTS('',3,3,((#74378,#74379,#74380,#74381),
(#74382,#74383,#74384,#74385),(#74386,#74387,#74388,#74389),(#74390,#74391,
#74392,#74393),(#74394,#74395,#74396,#74397)),.UNSPECIFIED.,.F.,.F.,.F.,
(4,1,4),(4,4),(0.,0.5,1.),(0.,0.0458781805671202),.UNSPECIFIED.);
#2059=B_SPLINE_SURFACE_WITH_KNOTS('',3,3,((#74461,#74462,#74463,#74464),
(#74465,#74466,#74467,#74468),(#74469,#74470,#74471,#74472),(#74473,#74474,
#74475,#74476),(#74477,#74478,#74479,#74480)),.UNSPECIFIED.,.F.,.F.,.F.,
(4,1,4),(4,4),(0.,0.5,1.),(0.,0.045878180567117),.UNSPECIFIED.);
#2060=B_SPLINE_SURFACE_WITH_KNOTS('',3,3,((#74536,#74537,#74538,#74539),
(#74540,#74541,#74542,#74543),(#74544,#74545,#74546,#74547),(#74548,#74549,
#74550,#74551),(#74552,#74553,#74554,#74555)),.UNSPECIFIED.,.F.,.F.,.F.,
(4,1,4),(4,4),(0.,0.5,1.),(0.,0.0458781805671145),.UNSPECIFIED.);
#2061=B_SPLINE_SURFACE_WITH_KNOTS('',3,3,((#74619,#74620,#74621,#74622),
(#74623,#74624,#74625,#74626),(#74627,#74628,#74629,#74630),(#74631,#74632,
#74633,#74634),(#74635,#74636,#74637,#74638)),.UNSPECIFIED.,.F.,.F.,.F.,
(4,1,4),(4,4),(0.,0.5,1.),(0.,0.0458781805671221),.UNSPECIFIED.);
#2062=B_SPLINE_SURFACE_WITH_KNOTS('',3,3,((#74702,#74703,#74704,#74705),
(#74706,#74707,#74708,#74709),(#74710,#74711,#74712,#74713),(#74714,#74715,
#74716,#74717),(#74718,#74719,#74720,#74721)),.UNSPECIFIED.,.F.,.F.,.F.,
(4,1,4),(4,4),(0.,0.5,1.),(0.,0.045878180567114),.UNSPECIFIED.);
#2063=B_SPLINE_SURFACE_WITH_KNOTS('',3,3,((#74771,#74772,#74773,#74774),
(#74775,#74776,#74777,#74778),(#74779,#74780,#74781,#74782),(#74783,#74784,
#74785,#74786),(#74787,#74788,#74789,#74790)),.UNSPECIFIED.,.F.,.F.,.F.,
(4,1,4),(4,4),(0.,0.5,1.),(0.,0.045878180566732),.UNSPECIFIED.);
#2064=B_SPLINE_SURFACE_WITH_KNOTS('',3,3,((#74823,#74824,#74825,#74826),
(#74827,#74828,#74829,#74830),(#74831,#74832,#74833,#74834),(#74835,#74836,
#74837,#74838),(#74839,#74840,#74841,#74842)),.UNSPECIFIED.,.F.,.F.,.F.,
(4,1,4),(4,4),(0.,0.5,1.),(0.,0.0458781805667396),.UNSPECIFIED.);
#2065=B_SPLINE_SURFACE_WITH_KNOTS('',3,3,((#74871,#74872,#74873,#74874),
(#74875,#74876,#74877,#74878),(#74879,#74880,#74881,#74882),(#74883,#74884,
#74885,#74886),(#74887,#74888,#74889,#74890)),.UNSPECIFIED.,.F.,.F.,.F.,
(4,1,4),(4,4),(0.,0.5,1.),(0.,0.0458781805667346),.UNSPECIFIED.);
#2066=B_SPLINE_SURFACE_WITH_KNOTS('',3,3,((#74919,#74920,#74921,#74922),
(#74923,#74924,#74925,#74926),(#74927,#74928,#74929,#74930),(#74931,#74932,
#74933,#74934),(#74935,#74936,#74937,#74938)),.UNSPECIFIED.,.F.,.F.,.F.,
(4,1,4),(4,4),(0.,0.5,1.),(0.,0.045878180566557),.UNSPECIFIED.);
#2067=B_SPLINE_SURFACE_WITH_KNOTS('',3,3,((#75049,#75050,#75051,#75052),
(#75053,#75054,#75055,#75056),(#75057,#75058,#75059,#75060),(#75061,#75062,
#75063,#75064),(#75065,#75066,#75067,#75068)),.UNSPECIFIED.,.F.,.F.,.F.,
(4,1,4),(4,4),(0.,0.5,1.),(0.,0.0458781805667708),.UNSPECIFIED.);
#2068=B_SPLINE_SURFACE_WITH_KNOTS('',3,3,((#75103,#75104,#75105,#75106),
(#75107,#75108,#75109,#75110),(#75111,#75112,#75113,#75114),(#75115,#75116,
#75117,#75118),(#75119,#75120,#75121,#75122)),.UNSPECIFIED.,.F.,.F.,.F.,
(4,1,4),(4,4),(0.,0.5,1.),(0.,0.0458781805671245),.UNSPECIFIED.);
#2069=B_SPLINE_SURFACE_WITH_KNOTS('',3,3,((#75172,#75173,#75174,#75175),
(#75176,#75177,#75178,#75179),(#75180,#75181,#75182,#75183),(#75184,#75185,
#75186,#75187),(#75188,#75189,#75190,#75191)),.UNSPECIFIED.,.F.,.F.,.F.,
(4,1,4),(4,4),(0.,0.5,1.),(0.,0.0458781805667811),.UNSPECIFIED.);
#2070=B_SPLINE_SURFACE_WITH_KNOTS('',3,3,((#75199,#75200,#75201,#75202),
(#75203,#75204,#75205,#75206),(#75207,#75208,#75209,#75210),(#75211,#75212,
#75213,#75214),(#75215,#75216,#75217,#75218)),.UNSPECIFIED.,.F.,.F.,.F.,
(4,1,4),(4,4),(0.,0.5,1.),(0.,0.0458781805667809),.UNSPECIFIED.);
#2071=B_SPLINE_SURFACE_WITH_KNOTS('',3,3,((#75299,#75300,#75301,#75302),
(#75303,#75304,#75305,#75306),(#75307,#75308,#75309,#75310),(#75311,#75312,
#75313,#75314),(#75315,#75316,#75317,#75318)),.UNSPECIFIED.,.F.,.F.,.F.,
(4,1,4),(4,4),(0.,0.5,1.),(0.0848913392683917,0.130769519836251),
 .UNSPECIFIED.);
#2072=B_SPLINE_SURFACE_WITH_KNOTS('',3,3,((#75522,#75523,#75524,#75525),
(#75526,#75527,#75528,#75529),(#75530,#75531,#75532,#75533),(#75534,#75535,
#75536,#75537),(#75538,#75539,#75540,#75541)),.UNSPECIFIED.,.F.,.F.,.F.,
(4,1,4),(4,4),(0.,0.5,1.),(0.,0.045878180566409),.UNSPECIFIED.);
#2073=B_SPLINE_SURFACE_WITH_KNOTS('',3,3,((#75755,#75756,#75757,#75758),
(#75759,#75760,#75761,#75762),(#75763,#75764,#75765,#75766),(#75767,#75768,
#75769,#75770),(#75771,#75772,#75773,#75774)),.UNSPECIFIED.,.F.,.F.,.F.,
(4,1,4),(4,4),(0.,0.5,1.),(0.,0.0458781805664144),.UNSPECIFIED.);
#2074=B_SPLINE_SURFACE_WITH_KNOTS('',3,3,((#75981,#75982,#75983,#75984),
(#75985,#75986,#75987,#75988),(#75989,#75990,#75991,#75992),(#75993,#75994,
#75995,#75996),(#75997,#75998,#75999,#76000)),.UNSPECIFIED.,.F.,.F.,.F.,
(4,1,4),(4,4),(0.,0.5,1.),(0.,0.045878180566409),.UNSPECIFIED.);
#2075=B_SPLINE_SURFACE_WITH_KNOTS('',3,3,((#76061,#76062,#76063,#76064),
(#76065,#76066,#76067,#76068),(#76069,#76070,#76071,#76072),(#76073,#76074,
#76075,#76076),(#76077,#76078,#76079,#76080)),.UNSPECIFIED.,.F.,.F.,.F.,
(4,1,4),(4,4),(0.,0.5,1.),(0.,0.0458781805665586),.UNSPECIFIED.);
#2076=B_SPLINE_SURFACE_WITH_KNOTS('',3,3,((#76223,#76224,#76225,#76226),
(#76227,#76228,#76229,#76230),(#76231,#76232,#76233,#76234),(#76235,#76236,
#76237,#76238),(#76239,#76240,#76241,#76242)),.UNSPECIFIED.,.F.,.F.,.F.,
(4,1,4),(4,4),(0.,0.5,1.),(0.,0.0458781805670896),.UNSPECIFIED.);
#2077=B_SPLINE_SURFACE_WITH_KNOTS('',3,3,((#76324,#76325,#76326,#76327),
(#76328,#76329,#76330,#76331),(#76332,#76333,#76334,#76335),(#76336,#76337,
#76338,#76339),(#76340,#76341,#76342,#76343)),.UNSPECIFIED.,.F.,.F.,.F.,
(4,1,4),(4,4),(0.,0.5,1.),(0.,0.0458781805670864),.UNSPECIFIED.);
#2078=B_SPLINE_SURFACE_WITH_KNOTS('',3,3,((#76393,#76394,#76395,#76396),
(#76397,#76398,#76399,#76400),(#76401,#76402,#76403,#76404),(#76405,#76406,
#76407,#76408),(#76409,#76410,#76411,#76412)),.UNSPECIFIED.,.F.,.F.,.F.,
(4,1,4),(4,4),(0.,0.5,1.),(0.,0.0458781805664134),.UNSPECIFIED.);
#2079=B_SPLINE_SURFACE_WITH_KNOTS('',3,3,((#76467,#76468,#76469,#76470),
(#76471,#76472,#76473,#76474),(#76475,#76476,#76477,#76478),(#76479,#76480,
#76481,#76482),(#76483,#76484,#76485,#76486)),.UNSPECIFIED.,.F.,.F.,.F.,
(4,1,4),(4,4),(0.,0.5,1.),(0.,0.0883236961657942),.UNSPECIFIED.);
#2080=B_SPLINE_SURFACE_WITH_KNOTS('',3,3,((#76502,#76503,#76504,#76505),
(#76506,#76507,#76508,#76509),(#76510,#76511,#76512,#76513),(#76514,#76515,
#76516,#76517),(#76518,#76519,#76520,#76521)),.UNSPECIFIED.,.F.,.F.,.F.,
(4,1,4),(4,4),(0.,0.5,1.),(0.,0.0458781805664131),.UNSPECIFIED.);
#2081=B_SPLINE_SURFACE_WITH_KNOTS('',3,3,((#76552,#76553,#76554,#76555),
(#76556,#76557,#76558,#76559),(#76560,#76561,#76562,#76563),(#76564,#76565,
#76566,#76567),(#76568,#76569,#76570,#76571)),.UNSPECIFIED.,.F.,.F.,.F.,
(4,1,4),(4,4),(0.,0.5,1.),(0.,0.0883236961657975),.UNSPECIFIED.);
#2082=B_SPLINE_SURFACE_WITH_KNOTS('',3,3,((#76593,#76594,#76595,#76596),
(#76597,#76598,#76599,#76600),(#76601,#76602,#76603,#76604),(#76605,#76606,
#76607,#76608),(#76609,#76610,#76611,#76612)),.UNSPECIFIED.,.F.,.F.,.F.,
(4,1,4),(4,4),(0.,0.5,1.),(0.,0.0883236961657995),.UNSPECIFIED.);
#2363=FACE_OUTER_BOUND('',#4767,.T.);
#2364=FACE_OUTER_BOUND('',#4768,.T.);
#2365=FACE_OUTER_BOUND('',#4769,.T.);
#2366=FACE_OUTER_BOUND('',#4770,.T.);
#2367=FACE_OUTER_BOUND('',#4771,.T.);
#2368=FACE_OUTER_BOUND('',#4772,.T.);
#2369=FACE_OUTER_BOUND('',#4773,.T.);
#2370=FACE_OUTER_BOUND('',#4774,.T.);
#2371=FACE_OUTER_BOUND('',#4775,.T.);
#2372=FACE_OUTER_BOUND('',#4776,.T.);
#2373=FACE_OUTER_BOUND('',#4777,.T.);
#2374=FACE_OUTER_BOUND('',#4778,.T.);
#2375=FACE_OUTER_BOUND('',#4780,.T.);
#2376=FACE_OUTER_BOUND('',#4781,.T.);
#2377=FACE_OUTER_BOUND('',#4782,.T.);
#2378=FACE_OUTER_BOUND('',#4783,.T.);
#2379=FACE_OUTER_BOUND('',#4784,.T.);
#2380=FACE_OUTER_BOUND('',#4785,.T.);
#2381=FACE_OUTER_BOUND('',#4786,.T.);
#2382=FACE_OUTER_BOUND('',#4787,.T.);
#2383=FACE_OUTER_BOUND('',#4788,.T.);
#2384=FACE_OUTER_BOUND('',#4789,.T.);
#2385=FACE_OUTER_BOUND('',#4790,.T.);
#2386=FACE_OUTER_BOUND('',#4791,.T.);
#2387=FACE_OUTER_BOUND('',#4792,.T.);
#2388=FACE_OUTER_BOUND('',#4793,.T.);
#2389=FACE_OUTER_BOUND('',#4794,.T.);
#2390=FACE_OUTER_BOUND('',#4795,.T.);
#2391=FACE_OUTER_BOUND('',#4796,.T.);
#2392=FACE_OUTER_BOUND('',#4797,.T.);
#2393=FACE_OUTER_BOUND('',#4798,.T.);
#2394=FACE_OUTER_BOUND('',#4799,.T.);
#2395=FACE_OUTER_BOUND('',#4800,.T.);
#2396=FACE_OUTER_BOUND('',#4801,.T.);
#2397=FACE_OUTER_BOUND('',#4802,.T.);
#2398=FACE_OUTER_BOUND('',#4803,.T.);
#2399=FACE_OUTER_BOUND('',#4804,.T.);
#2400=FACE_OUTER_BOUND('',#4805,.T.);
#2401=FACE_OUTER_BOUND('',#4806,.T.);
#2402=FACE_OUTER_BOUND('',#4807,.T.);
#2403=FACE_OUTER_BOUND('',#4808,.T.);
#2404=FACE_OUTER_BOUND('',#4809,.T.);
#2405=FACE_OUTER_BOUND('',#4810,.T.);
#2406=FACE_OUTER_BOUND('',#4811,.T.);
#2407=FACE_OUTER_BOUND('',#4812,.T.);
#2408=FACE_OUTER_BOUND('',#4813,.T.);
#2409=FACE_OUTER_BOUND('',#4814,.T.);
#2410=FACE_OUTER_BOUND('',#4815,.T.);
#2411=FACE_OUTER_BOUND('',#4816,.T.);
#2412=FACE_OUTER_BOUND('',#4817,.T.);
#2413=FACE_OUTER_BOUND('',#4818,.T.);
#2414=FACE_OUTER_BOUND('',#4819,.T.);
#2415=FACE_OUTER_BOUND('',#4820,.T.);
#2416=FACE_OUTER_BOUND('',#4821,.T.);
#2417=FACE_OUTER_BOUND('',#4822,.T.);
#2418=FACE_OUTER_BOUND('',#4823,.T.);
#2419=FACE_OUTER_BOUND('',#4824,.T.);
#2420=FACE_OUTER_BOUND('',#4825,.T.);
#2421=FACE_OUTER_BOUND('',#4826,.T.);
#2422=FACE_OUTER_BOUND('',#4827,.T.);
#2423=FACE_OUTER_BOUND('',#4828,.T.);
#2424=FACE_OUTER_BOUND('',#4829,.T.);
#2425=FACE_OUTER_BOUND('',#4830,.T.);
#2426=FACE_OUTER_BOUND('',#4831,.T.);
#2427=FACE_OUTER_BOUND('',#4832,.T.);
#2428=FACE_OUTER_BOUND('',#4833,.T.);
#2429=FACE_OUTER_BOUND('',#4834,.T.);
#2430=FACE_OUTER_BOUND('',#4835,.T.);
#2431=FACE_OUTER_BOUND('',#4836,.T.);
#2432=FACE_OUTER_BOUND('',#4837,.T.);
#2433=FACE_OUTER_BOUND('',#4838,.T.);
#2434=FACE_OUTER_BOUND('',#4839,.T.);
#2435=FACE_OUTER_BOUND('',#4840,.T.);
#2436=FACE_OUTER_BOUND('',#4841,.T.);
#2437=FACE_OUTER_BOUND('',#4842,.T.);
#2438=FACE_OUTER_BOUND('',#4843,.T.);
#2439=FACE_OUTER_BOUND('',#4844,.T.);
#2440=FACE_OUTER_BOUND('',#4845,.T.);
#2441=FACE_OUTER_BOUND('',#4846,.T.);
#2442=FACE_OUTER_BOUND('',#4847,.T.);
#2443=FACE_OUTER_BOUND('',#4848,.T.);
#2444=FACE_OUTER_BOUND('',#4849,.T.);
#2445=FACE_OUTER_BOUND('',#4850,.T.);
#2446=FACE_OUTER_BOUND('',#4851,.T.);
#2447=FACE_OUTER_BOUND('',#4853,.T.);
#2448=FACE_OUTER_BOUND('',#4854,.T.);
#2449=FACE_OUTER_BOUND('',#4855,.T.);
#2450=FACE_OUTER_BOUND('',#4856,.T.);
#2451=FACE_OUTER_BOUND('',#4857,.T.);
#2452=FACE_OUTER_BOUND('',#4858,.T.);
#2453=FACE_OUTER_BOUND('',#4859,.T.);
#2454=FACE_OUTER_BOUND('',#4860,.T.);
#2455=FACE_OUTER_BOUND('',#4861,.T.);
#2456=FACE_OUTER_BOUND('',#4862,.T.);
#2457=FACE_OUTER_BOUND('',#4863,.T.);
#2458=FACE_OUTER_BOUND('',#4864,.T.);
#2459=FACE_OUTER_BOUND('',#4865,.T.);
#2460=FACE_OUTER_BOUND('',#4866,.T.);
#2461=FACE_OUTER_BOUND('',#4867,.T.);
#2462=FACE_OUTER_BOUND('',#4868,.T.);
#2463=FACE_OUTER_BOUND('',#4869,.T.);
#2464=FACE_OUTER_BOUND('',#4870,.T.);
#2465=FACE_OUTER_BOUND('',#4871,.T.);
#2466=FACE_OUTER_BOUND('',#4872,.T.);
#2467=FACE_OUTER_BOUND('',#4873,.T.);
#2468=FACE_OUTER_BOUND('',#4874,.T.);
#2469=FACE_OUTER_BOUND('',#4875,.T.);
#2470=FACE_OUTER_BOUND('',#4876,.T.);
#2471=FACE_OUTER_BOUND('',#4877,.T.);
#2472=FACE_OUTER_BOUND('',#4878,.T.);
#2473=FACE_OUTER_BOUND('',#4879,.T.);
#2474=FACE_OUTER_BOUND('',#4880,.T.);
#2475=FACE_OUTER_BOUND('',#4881,.T.);
#2476=FACE_OUTER_BOUND('',#4882,.T.);
#2477=FACE_OUTER_BOUND('',#4883,.T.);
#2478=FACE_OUTER_BOUND('',#4884,.T.);
#2479=FACE_OUTER_BOUND('',#4885,.T.);
#2480=FACE_OUTER_BOUND('',#4886,.T.);
#2481=FACE_OUTER_BOUND('',#4887,.T.);
#2482=FACE_OUTER_BOUND('',#4888,.T.);
#2483=FACE_OUTER_BOUND('',#4889,.T.);
#2484=FACE_OUTER_BOUND('',#4890,.T.);
#2485=FACE_OUTER_BOUND('',#4891,.T.);
#2486=FACE_OUTER_BOUND('',#4892,.T.);
#2487=FACE_OUTER_BOUND('',#4893,.T.);
#2488=FACE_OUTER_BOUND('',#4894,.T.);
#2489=FACE_OUTER_BOUND('',#4895,.T.);
#2490=FACE_OUTER_BOUND('',#4896,.T.);
#2491=FACE_OUTER_BOUND('',#4897,.T.);
#2492=FACE_OUTER_BOUND('',#4898,.T.);
#2493=FACE_OUTER_BOUND('',#4899,.T.);
#2494=FACE_OUTER_BOUND('',#4900,.T.);
#2495=FACE_OUTER_BOUND('',#4901,.T.);
#2496=FACE_OUTER_BOUND('',#4902,.T.);
#2497=FACE_OUTER_BOUND('',#4903,.T.);
#2498=FACE_OUTER_BOUND('',#4904,.T.);
#2499=FACE_OUTER_BOUND('',#4905,.T.);
#2500=FACE_OUTER_BOUND('',#4906,.T.);
#2501=FACE_OUTER_BOUND('',#4907,.T.);
#2502=FACE_OUTER_BOUND('',#4908,.T.);
#2503=FACE_OUTER_BOUND('',#4909,.T.);
#2504=FACE_OUTER_BOUND('',#4910,.T.);
#2505=FACE_OUTER_BOUND('',#4911,.T.);
#2506=FACE_OUTER_BOUND('',#4912,.T.);
#2507=FACE_OUTER_BOUND('',#4913,.T.);
#2508=FACE_OUTER_BOUND('',#4914,.T.);
#2509=FACE_OUTER_BOUND('',#4915,.T.);
#2510=FACE_OUTER_BOUND('',#4916,.T.);
#2511=FACE_OUTER_BOUND('',#4917,.T.);
#2512=FACE_OUTER_BOUND('',#4918,.T.);
#2513=FACE_OUTER_BOUND('',#4919,.T.);
#2514=FACE_OUTER_BOUND('',#4920,.T.);
#2515=FACE_OUTER_BOUND('',#4921,.T.);
#2516=FACE_OUTER_BOUND('',#4922,.T.);
#2517=FACE_OUTER_BOUND('',#4923,.T.);
#2518=FACE_OUTER_BOUND('',#4924,.T.);
#2519=FACE_OUTER_BOUND('',#4925,.T.);
#2520=FACE_OUTER_BOUND('',#4926,.T.);
#2521=FACE_OUTER_BOUND('',#4927,.T.);
#2522=FACE_OUTER_BOUND('',#4928,.T.);
#2523=FACE_OUTER_BOUND('',#4929,.T.);
#2524=FACE_OUTER_BOUND('',#4930,.T.);
#2525=FACE_OUTER_BOUND('',#4931,.T.);
#2526=FACE_OUTER_BOUND('',#4932,.T.);
#2527=FACE_OUTER_BOUND('',#4933,.T.);
#2528=FACE_OUTER_BOUND('',#4934,.T.);
#2529=FACE_OUTER_BOUND('',#4935,.T.);
#2530=FACE_OUTER_BOUND('',#4936,.T.);
#2531=FACE_OUTER_BOUND('',#4937,.T.);
#2532=FACE_OUTER_BOUND('',#4938,.T.);
#2533=FACE_OUTER_BOUND('',#4939,.T.);
#2534=FACE_OUTER_BOUND('',#4940,.T.);
#2535=FACE_OUTER_BOUND('',#4941,.T.);
#2536=FACE_OUTER_BOUND('',#4942,.T.);
#2537=FACE_OUTER_BOUND('',#4943,.T.);
#2538=FACE_OUTER_BOUND('',#4944,.T.);
#2539=FACE_OUTER_BOUND('',#4945,.T.);
#2540=FACE_OUTER_BOUND('',#4946,.T.);
#2541=FACE_OUTER_BOUND('',#4947,.T.);
#2542=FACE_OUTER_BOUND('',#4948,.T.);
#2543=FACE_OUTER_BOUND('',#4949,.T.);
#2544=FACE_OUTER_BOUND('',#4950,.T.);
#2545=FACE_OUTER_BOUND('',#4951,.T.);
#2546=FACE_OUTER_BOUND('',#4952,.T.);
#2547=FACE_OUTER_BOUND('',#4953,.T.);
#2548=FACE_OUTER_BOUND('',#4954,.T.);
#2549=FACE_OUTER_BOUND('',#4955,.T.);
#2550=FACE_OUTER_BOUND('',#4956,.T.);
#2551=FACE_OUTER_BOUND('',#4957,.T.);
#2552=FACE_OUTER_BOUND('',#4958,.T.);
#2553=FACE_OUTER_BOUND('',#4959,.T.);
#2554=FACE_OUTER_BOUND('',#4960,.T.);
#2555=FACE_OUTER_BOUND('',#4961,.T.);
#2556=FACE_OUTER_BOUND('',#4962,.T.);
#2557=FACE_OUTER_BOUND('',#4963,.T.);
#2558=FACE_OUTER_BOUND('',#4964,.T.);
#2559=FACE_OUTER_BOUND('',#4965,.T.);
#2560=FACE_OUTER_BOUND('',#4966,.T.);
#2561=FACE_OUTER_BOUND('',#4967,.T.);
#2562=FACE_OUTER_BOUND('',#4968,.T.);
#2563=FACE_OUTER_BOUND('',#4969,.T.);
#2564=FACE_OUTER_BOUND('',#4970,.T.);
#2565=FACE_OUTER_BOUND('',#4971,.T.);
#2566=FACE_OUTER_BOUND('',#4972,.T.);
#2567=FACE_OUTER_BOUND('',#4973,.T.);
#2568=FACE_OUTER_BOUND('',#4974,.T.);
#2569=FACE_OUTER_BOUND('',#4975,.T.);
#2570=FACE_OUTER_BOUND('',#4976,.T.);
#2571=FACE_OUTER_BOUND('',#4977,.T.);
#2572=FACE_OUTER_BOUND('',#4978,.T.);
#2573=FACE_OUTER_BOUND('',#4979,.T.);
#2574=FACE_OUTER_BOUND('',#4980,.T.);
#2575=FACE_OUTER_BOUND('',#4981,.T.);
#2576=FACE_OUTER_BOUND('',#4982,.T.);
#2577=FACE_OUTER_BOUND('',#4983,.T.);
#2578=FACE_OUTER_BOUND('',#4984,.T.);
#2579=FACE_OUTER_BOUND('',#4985,.T.);
#2580=FACE_OUTER_BOUND('',#4986,.T.);
#2581=FACE_OUTER_BOUND('',#4987,.T.);
#2582=FACE_OUTER_BOUND('',#4988,.T.);
#2583=FACE_OUTER_BOUND('',#4989,.T.);
#2584=FACE_OUTER_BOUND('',#4990,.T.);
#2585=FACE_OUTER_BOUND('',#4991,.T.);
#2586=FACE_OUTER_BOUND('',#4992,.T.);
#2587=FACE_OUTER_BOUND('',#4993,.T.);
#2588=FACE_OUTER_BOUND('',#4994,.T.);
#2589=FACE_OUTER_BOUND('',#4995,.T.);
#2590=FACE_OUTER_BOUND('',#4996,.T.);
#2591=FACE_OUTER_BOUND('',#4997,.T.);
#2592=FACE_OUTER_BOUND('',#4998,.T.);
#2593=FACE_OUTER_BOUND('',#4999,.T.);
#2594=FACE_OUTER_BOUND('',#5000,.T.);
#2595=FACE_OUTER_BOUND('',#5001,.T.);
#2596=FACE_OUTER_BOUND('',#5002,.T.);
#2597=FACE_OUTER_BOUND('',#5003,.T.);
#2598=FACE_OUTER_BOUND('',#5004,.T.);
#2599=FACE_OUTER_BOUND('',#5005,.T.);
#2600=FACE_OUTER_BOUND('',#5006,.T.);
#2601=FACE_OUTER_BOUND('',#5007,.T.);
#2602=FACE_OUTER_BOUND('',#5008,.T.);
#2603=FACE_OUTER_BOUND('',#5009,.T.);
#2604=FACE_OUTER_BOUND('',#5010,.T.);
#2605=FACE_OUTER_BOUND('',#5011,.T.);
#2606=FACE_OUTER_BOUND('',#5012,.T.);
#2607=FACE_OUTER_BOUND('',#5013,.T.);
#2608=FACE_OUTER_BOUND('',#5014,.T.);
#2609=FACE_OUTER_BOUND('',#5015,.T.);
#2610=FACE_OUTER_BOUND('',#5016,.T.);
#2611=FACE_OUTER_BOUND('',#5017,.T.);
#2612=FACE_OUTER_BOUND('',#5018,.T.);
#2613=FACE_OUTER_BOUND('',#5019,.T.);
#2614=FACE_OUTER_BOUND('',#5020,.T.);
#2615=FACE_OUTER_BOUND('',#5021,.T.);
#2616=FACE_OUTER_BOUND('',#5022,.T.);
#2617=FACE_OUTER_BOUND('',#5023,.T.);
#2618=FACE_OUTER_BOUND('',#5024,.T.);
#2619=FACE_OUTER_BOUND('',#5025,.T.);
#2620=FACE_OUTER_BOUND('',#5026,.T.);
#2621=FACE_OUTER_BOUND('',#5027,.T.);
#2622=FACE_OUTER_BOUND('',#5028,.T.);
#2623=FACE_OUTER_BOUND('',#5029,.T.);
#2624=FACE_OUTER_BOUND('',#5030,.T.);
#2625=FACE_OUTER_BOUND('',#5031,.T.);
#2626=FACE_OUTER_BOUND('',#5032,.T.);
#2627=FACE_OUTER_BOUND('',#5033,.T.);
#2628=FACE_OUTER_BOUND('',#5034,.T.);
#2629=FACE_OUTER_BOUND('',#5035,.T.);
#2630=FACE_OUTER_BOUND('',#5036,.T.);
#2631=FACE_OUTER_BOUND('',#5037,.T.);
#2632=FACE_OUTER_BOUND('',#5038,.T.);
#2633=FACE_OUTER_BOUND('',#5039,.T.);
#2634=FACE_OUTER_BOUND('',#5040,.T.);
#2635=FACE_OUTER_BOUND('',#5041,.T.);
#2636=FACE_OUTER_BOUND('',#5042,.T.);
#2637=FACE_OUTER_BOUND('',#5043,.T.);
#2638=FACE_OUTER_BOUND('',#5044,.T.);
#2639=FACE_OUTER_BOUND('',#5045,.T.);
#2640=FACE_OUTER_BOUND('',#5046,.T.);
#2641=FACE_OUTER_BOUND('',#5047,.T.);
#2642=FACE_OUTER_BOUND('',#5048,.T.);
#2643=FACE_OUTER_BOUND('',#5049,.T.);
#2644=FACE_OUTER_BOUND('',#5050,.T.);
#2645=FACE_OUTER_BOUND('',#5051,.T.);
#2646=FACE_OUTER_BOUND('',#5052,.T.);
#2647=FACE_OUTER_BOUND('',#5053,.T.);
#2648=FACE_OUTER_BOUND('',#5054,.T.);
#2649=FACE_OUTER_BOUND('',#5055,.T.);
#2650=FACE_OUTER_BOUND('',#5056,.T.);
#2651=FACE_OUTER_BOUND('',#5057,.T.);
#2652=FACE_OUTER_BOUND('',#5058,.T.);
#2653=FACE_OUTER_BOUND('',#5059,.T.);
#2654=FACE_OUTER_BOUND('',#5060,.T.);
#2655=FACE_OUTER_BOUND('',#5061,.T.);
#2656=FACE_OUTER_BOUND('',#5062,.T.);
#2657=FACE_OUTER_BOUND('',#5063,.T.);
#2658=FACE_OUTER_BOUND('',#5064,.T.);
#2659=FACE_OUTER_BOUND('',#5065,.T.);
#2660=FACE_OUTER_BOUND('',#5066,.T.);
#2661=FACE_OUTER_BOUND('',#5067,.T.);
#2662=FACE_OUTER_BOUND('',#5068,.T.);
#2663=FACE_OUTER_BOUND('',#5069,.T.);
#2664=FACE_OUTER_BOUND('',#5070,.T.);
#2665=FACE_OUTER_BOUND('',#5071,.T.);
#2666=FACE_OUTER_BOUND('',#5072,.T.);
#2667=FACE_OUTER_BOUND('',#5073,.T.);
#2668=FACE_OUTER_BOUND('',#5074,.T.);
#2669=FACE_OUTER_BOUND('',#5075,.T.);
#2670=FACE_OUTER_BOUND('',#5076,.T.);
#2671=FACE_OUTER_BOUND('',#5077,.T.);
#2672=FACE_OUTER_BOUND('',#5078,.T.);
#2673=FACE_OUTER_BOUND('',#5079,.T.);
#2674=FACE_OUTER_BOUND('',#5080,.T.);
#2675=FACE_OUTER_BOUND('',#5081,.T.);
#2676=FACE_OUTER_BOUND('',#5082,.T.);
#2677=FACE_OUTER_BOUND('',#5083,.T.);
#2678=FACE_OUTER_BOUND('',#5084,.T.);
#2679=FACE_OUTER_BOUND('',#5085,.T.);
#2680=FACE_OUTER_BOUND('',#5086,.T.);
#2681=FACE_OUTER_BOUND('',#5087,.T.);
#2682=FACE_OUTER_BOUND('',#5088,.T.);
#2683=FACE_OUTER_BOUND('',#5089,.T.);
#2684=FACE_OUTER_BOUND('',#5090,.T.);
#2685=FACE_OUTER_BOUND('',#5091,.T.);
#2686=FACE_OUTER_BOUND('',#5092,.T.);
#2687=FACE_OUTER_BOUND('',#5093,.T.);
#2688=FACE_OUTER_BOUND('',#5094,.T.);
#2689=FACE_OUTER_BOUND('',#5095,.T.);
#2690=FACE_OUTER_BOUND('',#5096,.T.);
#2691=FACE_OUTER_BOUND('',#5097,.T.);
#2692=FACE_OUTER_BOUND('',#5098,.T.);
#2693=FACE_OUTER_BOUND('',#5099,.T.);
#2694=FACE_OUTER_BOUND('',#5100,.T.);
#2695=FACE_OUTER_BOUND('',#5101,.T.);
#2696=FACE_OUTER_BOUND('',#5102,.T.);
#2697=FACE_OUTER_BOUND('',#5103,.T.);
#2698=FACE_OUTER_BOUND('',#5104,.T.);
#2699=FACE_OUTER_BOUND('',#5105,.T.);
#2700=FACE_OUTER_BOUND('',#5106,.T.);
#2701=FACE_OUTER_BOUND('',#5107,.T.);
#2702=FACE_OUTER_BOUND('',#5108,.T.);
#2703=FACE_OUTER_BOUND('',#5109,.T.);
#2704=FACE_OUTER_BOUND('',#5110,.T.);
#2705=FACE_OUTER_BOUND('',#5111,.T.);
#2706=FACE_OUTER_BOUND('',#5112,.T.);
#2707=FACE_OUTER_BOUND('',#5113,.T.);
#2708=FACE_OUTER_BOUND('',#5114,.T.);
#2709=FACE_OUTER_BOUND('',#5115,.T.);
#2710=FACE_OUTER_BOUND('',#5116,.T.);
#2711=FACE_OUTER_BOUND('',#5117,.T.);
#2712=FACE_OUTER_BOUND('',#5118,.T.);
#2713=FACE_OUTER_BOUND('',#5119,.T.);
#2714=FACE_OUTER_BOUND('',#5120,.T.);
#2715=FACE_OUTER_BOUND('',#5121,.T.);
#2716=FACE_OUTER_BOUND('',#5122,.T.);
#2717=FACE_OUTER_BOUND('',#5123,.T.);
#2718=FACE_OUTER_BOUND('',#5124,.T.);
#2719=FACE_OUTER_BOUND('',#5125,.T.);
#2720=FACE_OUTER_BOUND('',#5126,.T.);
#2721=FACE_OUTER_BOUND('',#5127,.T.);
#2722=FACE_OUTER_BOUND('',#5128,.T.);
#2723=FACE_OUTER_BOUND('',#5129,.T.);
#2724=FACE_OUTER_BOUND('',#5130,.T.);
#2725=FACE_OUTER_BOUND('',#5131,.T.);
#2726=FACE_OUTER_BOUND('',#5132,.T.);
#2727=FACE_OUTER_BOUND('',#5133,.T.);
#2728=FACE_OUTER_BOUND('',#5134,.T.);
#2729=FACE_OUTER_BOUND('',#5135,.T.);
#2730=FACE_OUTER_BOUND('',#5136,.T.);
#2731=FACE_OUTER_BOUND('',#5137,.T.);
#2732=FACE_OUTER_BOUND('',#5138,.T.);
#2733=FACE_OUTER_BOUND('',#5139,.T.);
#2734=FACE_OUTER_BOUND('',#5140,.T.);
#2735=FACE_OUTER_BOUND('',#5141,.T.);
#2736=FACE_OUTER_BOUND('',#5142,.T.);
#2737=FACE_OUTER_BOUND('',#5143,.T.);
#2738=FACE_OUTER_BOUND('',#5144,.T.);
#2739=FACE_OUTER_BOUND('',#5145,.T.);
#2740=FACE_OUTER_BOUND('',#5146,.T.);
#2741=FACE_OUTER_BOUND('',#5147,.T.);
#2742=FACE_OUTER_BOUND('',#5148,.T.);
#2743=FACE_OUTER_BOUND('',#5149,.T.);
#2744=FACE_OUTER_BOUND('',#5150,.T.);
#2745=FACE_OUTER_BOUND('',#5151,.T.);
#2746=FACE_OUTER_BOUND('',#5152,.T.);
#2747=FACE_OUTER_BOUND('',#5153,.T.);
#2748=FACE_OUTER_BOUND('',#5154,.T.);
#2749=FACE_OUTER_BOUND('',#5155,.T.);
#2750=FACE_OUTER_BOUND('',#5156,.T.);
#2751=FACE_OUTER_BOUND('',#5157,.T.);
#2752=FACE_OUTER_BOUND('',#5158,.T.);
#2753=FACE_OUTER_BOUND('',#5159,.T.);
#2754=FACE_OUTER_BOUND('',#5160,.T.);
#2755=FACE_OUTER_BOUND('',#5161,.T.);
#2756=FACE_OUTER_BOUND('',#5162,.T.);
#2757=FACE_OUTER_BOUND('',#5163,.T.);
#2758=FACE_OUTER_BOUND('',#5164,.T.);
#2759=FACE_OUTER_BOUND('',#5165,.T.);
#2760=FACE_OUTER_BOUND('',#5166,.T.);
#2761=FACE_OUTER_BOUND('',#5167,.T.);
#2762=FACE_OUTER_BOUND('',#5168,.T.);
#2763=FACE_OUTER_BOUND('',#5169,.T.);
#2764=FACE_OUTER_BOUND('',#5170,.T.);
#2765=FACE_OUTER_BOUND('',#5171,.T.);
#2766=FACE_OUTER_BOUND('',#5172,.T.);
#2767=FACE_OUTER_BOUND('',#5173,.T.);
#2768=FACE_OUTER_BOUND('',#5174,.T.);
#2769=FACE_OUTER_BOUND('',#5175,.T.);
#2770=FACE_OUTER_BOUND('',#5176,.T.);
#2771=FACE_OUTER_BOUND('',#5177,.T.);
#2772=FACE_OUTER_BOUND('',#5178,.T.);
#2773=FACE_OUTER_BOUND('',#5179,.T.);
#2774=FACE_OUTER_BOUND('',#5180,.T.);
#2775=FACE_OUTER_BOUND('',#5181,.T.);
#2776=FACE_OUTER_BOUND('',#5182,.T.);
#2777=FACE_OUTER_BOUND('',#5183,.T.);
#2778=FACE_OUTER_BOUND('',#5184,.T.);
#2779=FACE_OUTER_BOUND('',#5185,.T.);
#2780=FACE_OUTER_BOUND('',#5186,.T.);
#2781=FACE_OUTER_BOUND('',#5187,.T.);
#2782=FACE_OUTER_BOUND('',#5188,.T.);
#2783=FACE_OUTER_BOUND('',#5189,.T.);
#2784=FACE_OUTER_BOUND('',#5190,.T.);
#2785=FACE_OUTER_BOUND('',#5191,.T.);
#2786=FACE_OUTER_BOUND('',#5192,.T.);
#2787=FACE_OUTER_BOUND('',#5193,.T.);
#2788=FACE_OUTER_BOUND('',#5194,.T.);
#2789=FACE_OUTER_BOUND('',#5195,.T.);
#2790=FACE_OUTER_BOUND('',#5196,.T.);
#2791=FACE_OUTER_BOUND('',#5197,.T.);
#2792=FACE_OUTER_BOUND('',#5198,.T.);
#2793=FACE_OUTER_BOUND('',#5199,.T.);
#2794=FACE_OUTER_BOUND('',#5200,.T.);
#2795=FACE_OUTER_BOUND('',#5201,.T.);
#2796=FACE_OUTER_BOUND('',#5202,.T.);
#2797=FACE_OUTER_BOUND('',#5203,.T.);
#2798=FACE_OUTER_BOUND('',#5204,.T.);
#2799=FACE_OUTER_BOUND('',#5205,.T.);
#2800=FACE_OUTER_BOUND('',#5206,.T.);
#2801=FACE_OUTER_BOUND('',#5207,.T.);
#2802=FACE_OUTER_BOUND('',#5208,.T.);
#2803=FACE_OUTER_BOUND('',#5209,.T.);
#2804=FACE_OUTER_BOUND('',#5210,.T.);
#2805=FACE_OUTER_BOUND('',#5211,.T.);
#2806=FACE_OUTER_BOUND('',#5212,.T.);
#2807=FACE_OUTER_BOUND('',#5213,.T.);
#2808=FACE_OUTER_BOUND('',#5214,.T.);
#2809=FACE_OUTER_BOUND('',#5215,.T.);
#2810=FACE_OUTER_BOUND('',#5216,.T.);
#2811=FACE_OUTER_BOUND('',#5217,.T.);
#2812=FACE_OUTER_BOUND('',#5218,.T.);
#2813=FACE_OUTER_BOUND('',#5219,.T.);
#2814=FACE_OUTER_BOUND('',#5220,.T.);
#2815=FACE_OUTER_BOUND('',#5221,.T.);
#2816=FACE_OUTER_BOUND('',#5222,.T.);
#2817=FACE_OUTER_BOUND('',#5223,.T.);
#2818=FACE_OUTER_BOUND('',#5224,.T.);
#2819=FACE_OUTER_BOUND('',#5225,.T.);
#2820=FACE_OUTER_BOUND('',#5226,.T.);
#2821=FACE_OUTER_BOUND('',#5227,.T.);
#2822=FACE_OUTER_BOUND('',#5228,.T.);
#2823=FACE_OUTER_BOUND('',#5229,.T.);
#2824=FACE_OUTER_BOUND('',#5230,.T.);
#2825=FACE_OUTER_BOUND('',#5231,.T.);
#2826=FACE_OUTER_BOUND('',#5232,.T.);
#2827=FACE_OUTER_BOUND('',#5233,.T.);
#2828=FACE_OUTER_BOUND('',#5234,.T.);
#2829=FACE_OUTER_BOUND('',#5235,.T.);
#2830=FACE_OUTER_BOUND('',#5236,.T.);
#2831=FACE_OUTER_BOUND('',#5237,.T.);
#2832=FACE_OUTER_BOUND('',#5238,.T.);
#2833=FACE_OUTER_BOUND('',#5239,.T.);
#2834=FACE_OUTER_BOUND('',#5240,.T.);
#2835=FACE_OUTER_BOUND('',#5241,.T.);
#2836=FACE_OUTER_BOUND('',#5242,.T.);
#2837=FACE_OUTER_BOUND('',#5243,.T.);
#2838=FACE_OUTER_BOUND('',#5244,.T.);
#2839=FACE_OUTER_BOUND('',#5245,.T.);
#2840=FACE_OUTER_BOUND('',#5246,.T.);
#2841=FACE_OUTER_BOUND('',#5247,.T.);
#2842=FACE_OUTER_BOUND('',#5248,.T.);
#2843=FACE_OUTER_BOUND('',#5249,.T.);
#2844=FACE_OUTER_BOUND('',#5250,.T.);
#2845=FACE_OUTER_BOUND('',#5251,.T.);
#2846=FACE_OUTER_BOUND('',#5252,.T.);
#2847=FACE_OUTER_BOUND('',#5253,.T.);
#2848=FACE_OUTER_BOUND('',#5254,.T.);
#2849=FACE_OUTER_BOUND('',#5255,.T.);
#2850=FACE_OUTER_BOUND('',#5256,.T.);
#2851=FACE_OUTER_BOUND('',#5257,.T.);
#2852=FACE_OUTER_BOUND('',#5258,.T.);
#2853=FACE_OUTER_BOUND('',#5259,.T.);
#2854=FACE_OUTER_BOUND('',#5260,.T.);
#2855=FACE_OUTER_BOUND('',#5261,.T.);
#2856=FACE_OUTER_BOUND('',#5262,.T.);
#2857=FACE_OUTER_BOUND('',#5263,.T.);
#2858=FACE_OUTER_BOUND('',#5264,.T.);
#2859=FACE_OUTER_BOUND('',#5265,.T.);
#2860=FACE_OUTER_BOUND('',#5266,.T.);
#2861=FACE_OUTER_BOUND('',#5267,.T.);
#2862=FACE_OUTER_BOUND('',#5268,.T.);
#2863=FACE_OUTER_BOUND('',#5269,.T.);
#2864=FACE_OUTER_BOUND('',#5270,.T.);
#2865=FACE_OUTER_BOUND('',#5271,.T.);
#2866=FACE_OUTER_BOUND('',#5272,.T.);
#2867=FACE_OUTER_BOUND('',#5273,.T.);
#2868=FACE_OUTER_BOUND('',#5274,.T.);
#2869=FACE_OUTER_BOUND('',#5275,.T.);
#2870=FACE_OUTER_BOUND('',#5276,.T.);
#2871=FACE_OUTER_BOUND('',#5277,.T.);
#2872=FACE_OUTER_BOUND('',#5278,.T.);
#2873=FACE_OUTER_BOUND('',#5279,.T.);
#2874=FACE_OUTER_BOUND('',#5280,.T.);
#2875=FACE_OUTER_BOUND('',#5281,.T.);
#2876=FACE_OUTER_BOUND('',#5282,.T.);
#2877=FACE_OUTER_BOUND('',#5283,.T.);
#2878=FACE_OUTER_BOUND('',#5284,.T.);
#2879=FACE_OUTER_BOUND('',#5285,.T.);
#2880=FACE_OUTER_BOUND('',#5286,.T.);
#2881=FACE_OUTER_BOUND('',#5287,.T.);
#2882=FACE_OUTER_BOUND('',#5288,.T.);
#2883=FACE_OUTER_BOUND('',#5289,.T.);
#2884=FACE_OUTER_BOUND('',#5290,.T.);
#2885=FACE_OUTER_BOUND('',#5291,.T.);
#2886=FACE_OUTER_BOUND('',#5292,.T.);
#2887=FACE_OUTER_BOUND('',#5293,.T.);
#2888=FACE_OUTER_BOUND('',#5294,.T.);
#2889=FACE_OUTER_BOUND('',#5295,.T.);
#2890=FACE_OUTER_BOUND('',#5296,.T.);
#2891=FACE_OUTER_BOUND('',#5297,.T.);
#2892=FACE_OUTER_BOUND('',#5298,.T.);
#2893=FACE_OUTER_BOUND('',#5299,.T.);
#2894=FACE_OUTER_BOUND('',#5300,.T.);
#2895=FACE_OUTER_BOUND('',#5301,.T.);
#2896=FACE_OUTER_BOUND('',#5302,.T.);
#2897=FACE_OUTER_BOUND('',#5303,.T.);
#2898=FACE_OUTER_BOUND('',#5304,.T.);
#2899=FACE_OUTER_BOUND('',#5305,.T.);
#2900=FACE_OUTER_BOUND('',#5306,.T.);
#2901=FACE_OUTER_BOUND('',#5307,.T.);
#2902=FACE_OUTER_BOUND('',#5308,.T.);
#2903=FACE_OUTER_BOUND('',#5309,.T.);
#2904=FACE_OUTER_BOUND('',#5310,.T.);
#2905=FACE_OUTER_BOUND('',#5311,.T.);
#2906=FACE_OUTER_BOUND('',#5312,.T.);
#2907=FACE_OUTER_BOUND('',#5313,.T.);
#2908=FACE_OUTER_BOUND('',#5314,.T.);
#2909=FACE_OUTER_BOUND('',#5315,.T.);
#2910=FACE_OUTER_BOUND('',#5316,.T.);
#2911=FACE_OUTER_BOUND('',#5317,.T.);
#2912=FACE_OUTER_BOUND('',#5318,.T.);
#2913=FACE_OUTER_BOUND('',#5319,.T.);
#2914=FACE_OUTER_BOUND('',#5320,.T.);
#2915=FACE_OUTER_BOUND('',#5321,.T.);
#2916=FACE_OUTER_BOUND('',#5322,.T.);
#2917=FACE_OUTER_BOUND('',#5323,.T.);
#2918=FACE_OUTER_BOUND('',#5324,.T.);
#2919=FACE_OUTER_BOUND('',#5325,.T.);
#2920=FACE_OUTER_BOUND('',#5326,.T.);
#2921=FACE_OUTER_BOUND('',#5327,.T.);
#2922=FACE_OUTER_BOUND('',#5328,.T.);
#2923=FACE_OUTER_BOUND('',#5329,.T.);
#2924=FACE_OUTER_BOUND('',#5330,.T.);
#2925=FACE_OUTER_BOUND('',#5331,.T.);
#2926=FACE_OUTER_BOUND('',#5332,.T.);
#2927=FACE_OUTER_BOUND('',#5333,.T.);
#2928=FACE_OUTER_BOUND('',#5334,.T.);
#2929=FACE_OUTER_BOUND('',#5335,.T.);
#2930=FACE_OUTER_BOUND('',#5336,.T.);
#2931=FACE_OUTER_BOUND('',#5337,.T.);
#2932=FACE_OUTER_BOUND('',#5338,.T.);
#2933=FACE_OUTER_BOUND('',#5339,.T.);
#2934=FACE_OUTER_BOUND('',#5340,.T.);
#2935=FACE_OUTER_BOUND('',#5341,.T.);
#2936=FACE_OUTER_BOUND('',#5342,.T.);
#2937=FACE_OUTER_BOUND('',#5343,.T.);
#2938=FACE_OUTER_BOUND('',#5344,.T.);
#2939=FACE_OUTER_BOUND('',#5345,.T.);
#2940=FACE_OUTER_BOUND('',#5346,.T.);
#2941=FACE_OUTER_BOUND('',#5347,.T.);
#2942=FACE_OUTER_BOUND('',#5348,.T.);
#2943=FACE_OUTER_BOUND('',#5349,.T.);
#2944=FACE_OUTER_BOUND('',#5350,.T.);
#2945=FACE_OUTER_BOUND('',#5351,.T.);
#2946=FACE_OUTER_BOUND('',#5352,.T.);
#2947=FACE_OUTER_BOUND('',#5353,.T.);
#2948=FACE_OUTER_BOUND('',#5354,.T.);
#2949=FACE_OUTER_BOUND('',#5355,.T.);
#2950=FACE_OUTER_BOUND('',#5356,.T.);
#2951=FACE_OUTER_BOUND('',#5357,.T.);
#2952=FACE_OUTER_BOUND('',#5358,.T.);
#2953=FACE_OUTER_BOUND('',#5359,.T.);
#2954=FACE_OUTER_BOUND('',#5360,.T.);
#2955=FACE_OUTER_BOUND('',#5361,.T.);
#2956=FACE_OUTER_BOUND('',#5362,.T.);
#2957=FACE_OUTER_BOUND('',#5363,.T.);
#2958=FACE_OUTER_BOUND('',#5364,.T.);
#2959=FACE_OUTER_BOUND('',#5365,.T.);
#2960=FACE_OUTER_BOUND('',#5366,.T.);
#2961=FACE_OUTER_BOUND('',#5367,.T.);
#2962=FACE_OUTER_BOUND('',#5368,.T.);
#2963=FACE_OUTER_BOUND('',#5369,.T.);
#2964=FACE_OUTER_BOUND('',#5370,.T.);
#2965=FACE_OUTER_BOUND('',#5371,.T.);
#2966=FACE_OUTER_BOUND('',#5372,.T.);
#2967=FACE_OUTER_BOUND('',#5373,.T.);
#2968=FACE_OUTER_BOUND('',#5374,.T.);
#2969=FACE_OUTER_BOUND('',#5375,.T.);
#2970=FACE_OUTER_BOUND('',#5376,.T.);
#2971=FACE_OUTER_BOUND('',#5377,.T.);
#2972=FACE_OUTER_BOUND('',#5378,.T.);
#2973=FACE_OUTER_BOUND('',#5379,.T.);
#2974=FACE_OUTER_BOUND('',#5380,.T.);
#2975=FACE_OUTER_BOUND('',#5381,.T.);
#2976=FACE_OUTER_BOUND('',#5382,.T.);
#2977=FACE_OUTER_BOUND('',#5383,.T.);
#2978=FACE_OUTER_BOUND('',#5384,.T.);
#2979=FACE_OUTER_BOUND('',#5385,.T.);
#2980=FACE_OUTER_BOUND('',#5386,.T.);
#2981=FACE_OUTER_BOUND('',#5387,.T.);
#2982=FACE_OUTER_BOUND('',#5388,.T.);
#2983=FACE_OUTER_BOUND('',#5389,.T.);
#2984=FACE_OUTER_BOUND('',#5390,.T.);
#2985=FACE_OUTER_BOUND('',#5391,.T.);
#2986=FACE_OUTER_BOUND('',#5392,.T.);
#2987=FACE_OUTER_BOUND('',#5393,.T.);
#2988=FACE_OUTER_BOUND('',#5394,.T.);
#2989=FACE_OUTER_BOUND('',#5395,.T.);
#2990=FACE_OUTER_BOUND('',#5396,.T.);
#2991=FACE_OUTER_BOUND('',#5397,.T.);
#2992=FACE_OUTER_BOUND('',#5398,.T.);
#2993=FACE_OUTER_BOUND('',#5399,.T.);
#2994=FACE_OUTER_BOUND('',#5400,.T.);
#2995=FACE_OUTER_BOUND('',#5401,.T.);
#2996=FACE_OUTER_BOUND('',#5402,.T.);
#2997=FACE_OUTER_BOUND('',#5403,.T.);
#2998=FACE_OUTER_BOUND('',#5404,.T.);
#2999=FACE_OUTER_BOUND('',#5405,.T.);
#3000=FACE_OUTER_BOUND('',#5406,.T.);
#3001=FACE_OUTER_BOUND('',#5407,.T.);
#3002=FACE_OUTER_BOUND('',#5408,.T.);
#3003=FACE_OUTER_BOUND('',#5409,.T.);
#3004=FACE_OUTER_BOUND('',#5410,.T.);
#3005=FACE_OUTER_BOUND('',#5411,.T.);
#3006=FACE_OUTER_BOUND('',#5412,.T.);
#3007=FACE_OUTER_BOUND('',#5413,.T.);
#3008=FACE_OUTER_BOUND('',#5414,.T.);
#3009=FACE_OUTER_BOUND('',#5415,.T.);
#3010=FACE_OUTER_BOUND('',#5416,.T.);
#3011=FACE_OUTER_BOUND('',#5417,.T.);
#3012=FACE_OUTER_BOUND('',#5418,.T.);
#3013=FACE_OUTER_BOUND('',#5419,.T.);
#3014=FACE_OUTER_BOUND('',#5420,.T.);
#3015=FACE_OUTER_BOUND('',#5421,.T.);
#3016=FACE_OUTER_BOUND('',#5422,.T.);
#3017=FACE_OUTER_BOUND('',#5423,.T.);
#3018=FACE_OUTER_BOUND('',#5424,.T.);
#3019=FACE_OUTER_BOUND('',#5425,.T.);
#3020=FACE_OUTER_BOUND('',#5426,.T.);
#3021=FACE_OUTER_BOUND('',#5427,.T.);
#3022=FACE_OUTER_BOUND('',#5428,.T.);
#3023=FACE_OUTER_BOUND('',#5429,.T.);
#3024=FACE_OUTER_BOUND('',#5430,.T.);
#3025=FACE_OUTER_BOUND('',#5431,.T.);
#3026=FACE_OUTER_BOUND('',#5432,.T.);
#3027=FACE_OUTER_BOUND('',#5433,.T.);
#3028=FACE_OUTER_BOUND('',#5434,.T.);
#3029=FACE_OUTER_BOUND('',#5435,.T.);
#3030=FACE_OUTER_BOUND('',#5436,.T.);
#3031=FACE_OUTER_BOUND('',#5437,.T.);
#3032=FACE_OUTER_BOUND('',#5438,.T.);
#3033=FACE_OUTER_BOUND('',#5439,.T.);
#3034=FACE_OUTER_BOUND('',#5440,.T.);
#3035=FACE_OUTER_BOUND('',#5441,.T.);
#3036=FACE_OUTER_BOUND('',#5442,.T.);
#3037=FACE_OUTER_BOUND('',#5443,.T.);
#3038=FACE_OUTER_BOUND('',#5444,.T.);
#3039=FACE_OUTER_BOUND('',#5445,.T.);
#3040=FACE_OUTER_BOUND('',#5446,.T.);
#3041=FACE_OUTER_BOUND('',#5447,.T.);
#3042=FACE_OUTER_BOUND('',#5448,.T.);
#3043=FACE_OUTER_BOUND('',#5449,.T.);
#3044=FACE_OUTER_BOUND('',#5450,.T.);
#3045=FACE_OUTER_BOUND('',#5451,.T.);
#3046=FACE_OUTER_BOUND('',#5452,.T.);
#3047=FACE_OUTER_BOUND('',#5453,.T.);
#3048=FACE_OUTER_BOUND('',#5454,.T.);
#3049=FACE_OUTER_BOUND('',#5455,.T.);
#3050=FACE_OUTER_BOUND('',#5456,.T.);
#3051=FACE_OUTER_BOUND('',#5457,.T.);
#3052=FACE_OUTER_BOUND('',#5458,.T.);
#3053=FACE_OUTER_BOUND('',#5459,.T.);
#3054=FACE_OUTER_BOUND('',#5460,.T.);
#3055=FACE_OUTER_BOUND('',#5461,.T.);
#3056=FACE_OUTER_BOUND('',#5462,.T.);
#3057=FACE_OUTER_BOUND('',#5463,.T.);
#3058=FACE_OUTER_BOUND('',#5464,.T.);
#3059=FACE_OUTER_BOUND('',#5465,.T.);
#3060=FACE_OUTER_BOUND('',#5466,.T.);
#3061=FACE_OUTER_BOUND('',#5467,.T.);
#3062=FACE_OUTER_BOUND('',#5468,.T.);
#3063=FACE_OUTER_BOUND('',#5469,.T.);
#3064=FACE_OUTER_BOUND('',#5470,.T.);
#3065=FACE_OUTER_BOUND('',#5471,.T.);
#3066=FACE_OUTER_BOUND('',#5472,.T.);
#3067=FACE_OUTER_BOUND('',#5473,.T.);
#3068=FACE_OUTER_BOUND('',#5474,.T.);
#3069=FACE_OUTER_BOUND('',#5475,.T.);
#3070=FACE_OUTER_BOUND('',#5476,.T.);
#3071=FACE_OUTER_BOUND('',#5477,.T.);
#3072=FACE_OUTER_BOUND('',#5478,.T.);
#3073=FACE_OUTER_BOUND('',#5479,.T.);
#3074=FACE_OUTER_BOUND('',#5480,.T.);
#3075=FACE_OUTER_BOUND('',#5481,.T.);
#3076=FACE_OUTER_BOUND('',#5482,.T.);
#3077=FACE_OUTER_BOUND('',#5483,.T.);
#3078=FACE_OUTER_BOUND('',#5484,.T.);
#3079=FACE_OUTER_BOUND('',#5485,.T.);
#3080=FACE_OUTER_BOUND('',#5486,.T.);
#3081=FACE_OUTER_BOUND('',#5487,.T.);
#3082=FACE_OUTER_BOUND('',#5488,.T.);
#3083=FACE_OUTER_BOUND('',#5489,.T.);
#3084=FACE_OUTER_BOUND('',#5490,.T.);
#3085=FACE_OUTER_BOUND('',#5491,.T.);
#3086=FACE_OUTER_BOUND('',#5492,.T.);
#3087=FACE_OUTER_BOUND('',#5493,.T.);
#3088=FACE_OUTER_BOUND('',#5494,.T.);
#3089=FACE_OUTER_BOUND('',#5495,.T.);
#3090=FACE_OUTER_BOUND('',#5496,.T.);
#3091=FACE_OUTER_BOUND('',#5497,.T.);
#3092=FACE_OUTER_BOUND('',#5498,.T.);
#3093=FACE_OUTER_BOUND('',#5499,.T.);
#3094=FACE_OUTER_BOUND('',#5500,.T.);
#3095=FACE_OUTER_BOUND('',#5501,.T.);
#3096=FACE_OUTER_BOUND('',#5502,.T.);
#3097=FACE_OUTER_BOUND('',#5503,.T.);
#3098=FACE_OUTER_BOUND('',#5504,.T.);
#3099=FACE_OUTER_BOUND('',#5505,.T.);
#3100=FACE_OUTER_BOUND('',#5506,.T.);
#3101=FACE_OUTER_BOUND('',#5507,.T.);
#3102=FACE_OUTER_BOUND('',#5508,.T.);
#3103=FACE_OUTER_BOUND('',#5509,.T.);
#3104=FACE_OUTER_BOUND('',#5510,.T.);
#3105=FACE_OUTER_BOUND('',#5511,.T.);
#3106=FACE_OUTER_BOUND('',#5512,.T.);
#3107=FACE_OUTER_BOUND('',#5513,.T.);
#3108=FACE_OUTER_BOUND('',#5514,.T.);
#3109=FACE_OUTER_BOUND('',#5515,.T.);
#3110=FACE_OUTER_BOUND('',#5516,.T.);
#3111=FACE_OUTER_BOUND('',#5517,.T.);
#3112=FACE_OUTER_BOUND('',#5518,.T.);
#3113=FACE_OUTER_BOUND('',#5519,.T.);
#3114=FACE_OUTER_BOUND('',#5520,.T.);
#3115=FACE_OUTER_BOUND('',#5521,.T.);
#3116=FACE_OUTER_BOUND('',#5522,.T.);
#3117=FACE_OUTER_BOUND('',#5523,.T.);
#3118=FACE_OUTER_BOUND('',#5524,.T.);
#3119=FACE_OUTER_BOUND('',#5525,.T.);
#3120=FACE_OUTER_BOUND('',#5526,.T.);
#3121=FACE_OUTER_BOUND('',#5527,.T.);
#3122=FACE_OUTER_BOUND('',#5528,.T.);
#3123=FACE_OUTER_BOUND('',#5529,.T.);
#3124=FACE_OUTER_BOUND('',#5530,.T.);
#3125=FACE_OUTER_BOUND('',#5531,.T.);
#3126=FACE_OUTER_BOUND('',#5532,.T.);
#3127=FACE_OUTER_BOUND('',#5533,.T.);
#3128=FACE_OUTER_BOUND('',#5534,.T.);
#3129=FACE_OUTER_BOUND('',#5535,.T.);
#3130=FACE_OUTER_BOUND('',#5536,.T.);
#3131=FACE_OUTER_BOUND('',#5537,.T.);
#3132=FACE_OUTER_BOUND('',#5538,.T.);
#3133=FACE_OUTER_BOUND('',#5539,.T.);
#3134=FACE_OUTER_BOUND('',#5540,.T.);
#3135=FACE_OUTER_BOUND('',#5541,.T.);
#3136=FACE_OUTER_BOUND('',#5542,.T.);
#3137=FACE_OUTER_BOUND('',#5543,.T.);
#3138=FACE_OUTER_BOUND('',#5544,.T.);
#3139=FACE_OUTER_BOUND('',#5545,.T.);
#3140=FACE_OUTER_BOUND('',#5546,.T.);
#3141=FACE_OUTER_BOUND('',#5547,.T.);
#3142=FACE_OUTER_BOUND('',#5548,.T.);
#3143=FACE_OUTER_BOUND('',#5549,.T.);
#3144=FACE_OUTER_BOUND('',#5550,.T.);
#3145=FACE_OUTER_BOUND('',#5551,.T.);
#3146=FACE_OUTER_BOUND('',#5552,.T.);
#3147=FACE_OUTER_BOUND('',#5553,.T.);
#3148=FACE_OUTER_BOUND('',#5554,.T.);
#3149=FACE_OUTER_BOUND('',#5555,.T.);
#3150=FACE_OUTER_BOUND('',#5556,.T.);
#3151=FACE_OUTER_BOUND('',#5557,.T.);
#3152=FACE_OUTER_BOUND('',#5558,.T.);
#3153=FACE_OUTER_BOUND('',#5559,.T.);
#3154=FACE_OUTER_BOUND('',#5560,.T.);
#3155=FACE_OUTER_BOUND('',#5561,.T.);
#3156=FACE_OUTER_BOUND('',#5562,.T.);
#3157=FACE_OUTER_BOUND('',#5563,.T.);
#3158=FACE_OUTER_BOUND('',#5564,.T.);
#3159=FACE_OUTER_BOUND('',#5565,.T.);
#3160=FACE_OUTER_BOUND('',#5566,.T.);
#3161=FACE_OUTER_BOUND('',#5567,.T.);
#3162=FACE_OUTER_BOUND('',#5568,.T.);
#3163=FACE_OUTER_BOUND('',#5569,.T.);
#3164=FACE_OUTER_BOUND('',#5570,.T.);
#3165=FACE_OUTER_BOUND('',#5571,.T.);
#3166=FACE_OUTER_BOUND('',#5572,.T.);
#3167=FACE_OUTER_BOUND('',#5573,.T.);
#3168=FACE_OUTER_BOUND('',#5574,.T.);
#3169=FACE_OUTER_BOUND('',#5575,.T.);
#3170=FACE_OUTER_BOUND('',#5576,.T.);
#3171=FACE_OUTER_BOUND('',#5577,.T.);
#3172=FACE_OUTER_BOUND('',#5578,.T.);
#3173=FACE_OUTER_BOUND('',#5579,.T.);
#3174=FACE_OUTER_BOUND('',#5580,.T.);
#3175=FACE_OUTER_BOUND('',#5581,.T.);
#3176=FACE_OUTER_BOUND('',#5582,.T.);
#3177=FACE_OUTER_BOUND('',#5583,.T.);
#3178=FACE_OUTER_BOUND('',#5584,.T.);
#3179=FACE_OUTER_BOUND('',#5585,.T.);
#3180=FACE_OUTER_BOUND('',#5586,.T.);
#3181=FACE_OUTER_BOUND('',#5587,.T.);
#3182=FACE_OUTER_BOUND('',#5588,.T.);
#3183=FACE_OUTER_BOUND('',#5589,.T.);
#3184=FACE_OUTER_BOUND('',#5590,.T.);
#3185=FACE_OUTER_BOUND('',#5591,.T.);
#3186=FACE_OUTER_BOUND('',#5592,.T.);
#3187=FACE_OUTER_BOUND('',#5593,.T.);
#3188=FACE_OUTER_BOUND('',#5594,.T.);
#3189=FACE_OUTER_BOUND('',#5595,.T.);
#3190=FACE_OUTER_BOUND('',#5596,.T.);
#3191=FACE_OUTER_BOUND('',#5597,.T.);
#3192=FACE_OUTER_BOUND('',#5598,.T.);
#3193=FACE_OUTER_BOUND('',#5599,.T.);
#3194=FACE_OUTER_BOUND('',#5600,.T.);
#3195=FACE_OUTER_BOUND('',#5601,.T.);
#3196=FACE_OUTER_BOUND('',#5602,.T.);
#3197=FACE_OUTER_BOUND('',#5603,.T.);
#3198=FACE_OUTER_BOUND('',#5604,.T.);
#3199=FACE_OUTER_BOUND('',#5605,.T.);
#3200=FACE_OUTER_BOUND('',#5606,.T.);
#3201=FACE_OUTER_BOUND('',#5607,.T.);
#3202=FACE_OUTER_BOUND('',#5608,.T.);
#3203=FACE_OUTER_BOUND('',#5609,.T.);
#3204=FACE_OUTER_BOUND('',#5610,.T.);
#3205=FACE_OUTER_BOUND('',#5611,.T.);
#3206=FACE_OUTER_BOUND('',#5612,.T.);
#3207=FACE_OUTER_BOUND('',#5613,.T.);
#3208=FACE_OUTER_BOUND('',#5614,.T.);
#3209=FACE_OUTER_BOUND('',#5615,.T.);
#3210=FACE_OUTER_BOUND('',#5616,.T.);
#3211=FACE_OUTER_BOUND('',#5617,.T.);
#3212=FACE_OUTER_BOUND('',#5618,.T.);
#3213=FACE_OUTER_BOUND('',#5619,.T.);
#3214=FACE_OUTER_BOUND('',#5620,.T.);
#3215=FACE_OUTER_BOUND('',#5621,.T.);
#3216=FACE_OUTER_BOUND('',#5622,.T.);
#3217=FACE_OUTER_BOUND('',#5623,.T.);
#3218=FACE_OUTER_BOUND('',#5624,.T.);
#3219=FACE_OUTER_BOUND('',#5625,.T.);
#3220=FACE_OUTER_BOUND('',#5626,.T.);
#3221=FACE_OUTER_BOUND('',#5627,.T.);
#3222=FACE_OUTER_BOUND('',#5628,.T.);
#3223=FACE_OUTER_BOUND('',#5629,.T.);
#3224=FACE_OUTER_BOUND('',#5630,.T.);
#3225=FACE_OUTER_BOUND('',#5631,.T.);
#3226=FACE_OUTER_BOUND('',#5632,.T.);
#3227=FACE_OUTER_BOUND('',#5633,.T.);
#3228=FACE_OUTER_BOUND('',#5634,.T.);
#3229=FACE_OUTER_BOUND('',#5635,.T.);
#3230=FACE_OUTER_BOUND('',#5636,.T.);
#3231=FACE_OUTER_BOUND('',#5637,.T.);
#3232=FACE_OUTER_BOUND('',#5638,.T.);
#3233=FACE_OUTER_BOUND('',#5639,.T.);
#3234=FACE_OUTER_BOUND('',#5640,.T.);
#3235=FACE_OUTER_BOUND('',#5641,.T.);
#3236=FACE_OUTER_BOUND('',#5642,.T.);
#3237=FACE_OUTER_BOUND('',#5643,.T.);
#3238=FACE_OUTER_BOUND('',#5644,.T.);
#3239=FACE_OUTER_BOUND('',#5645,.T.);
#3240=FACE_OUTER_BOUND('',#5646,.T.);
#3241=FACE_OUTER_BOUND('',#5647,.T.);
#3242=FACE_OUTER_BOUND('',#5648,.T.);
#3243=FACE_OUTER_BOUND('',#5649,.T.);
#3244=FACE_OUTER_BOUND('',#5650,.T.);
#3245=FACE_OUTER_BOUND('',#5651,.T.);
#3246=FACE_OUTER_BOUND('',#5652,.T.);
#3247=FACE_OUTER_BOUND('',#5653,.T.);
#3248=FACE_OUTER_BOUND('',#5654,.T.);
#3249=FACE_OUTER_BOUND('',#5655,.T.);
#3250=FACE_OUTER_BOUND('',#5656,.T.);
#3251=FACE_OUTER_BOUND('',#5657,.T.);
#3252=FACE_OUTER_BOUND('',#5658,.T.);
#3253=FACE_OUTER_BOUND('',#5659,.T.);
#3254=FACE_OUTER_BOUND('',#5660,.T.);
#3255=FACE_OUTER_BOUND('',#5661,.T.);
#3256=FACE_OUTER_BOUND('',#5662,.T.);
#3257=FACE_OUTER_BOUND('',#5663,.T.);
#3258=FACE_OUTER_BOUND('',#5664,.T.);
#3259=FACE_OUTER_BOUND('',#5665,.T.);
#3260=FACE_OUTER_BOUND('',#5666,.T.);
#3261=FACE_OUTER_BOUND('',#5667,.T.);
#3262=FACE_OUTER_BOUND('',#5668,.T.);
#3263=FACE_OUTER_BOUND('',#5669,.T.);
#3264=FACE_OUTER_BOUND('',#5670,.T.);
#3265=FACE_OUTER_BOUND('',#5671,.T.);
#3266=FACE_OUTER_BOUND('',#5672,.T.);
#3267=FACE_OUTER_BOUND('',#5673,.T.);
#3268=FACE_OUTER_BOUND('',#5674,.T.);
#3269=FACE_OUTER_BOUND('',#5675,.T.);
#3270=FACE_OUTER_BOUND('',#5676,.T.);
#3271=FACE_OUTER_BOUND('',#5677,.T.);
#3272=FACE_OUTER_BOUND('',#5678,.T.);
#3273=FACE_OUTER_BOUND('',#5679,.T.);
#3274=FACE_OUTER_BOUND('',#5680,.T.);
#3275=FACE_OUTER_BOUND('',#5681,.T.);
#3276=FACE_OUTER_BOUND('',#5682,.T.);
#3277=FACE_OUTER_BOUND('',#5683,.T.);
#3278=FACE_OUTER_BOUND('',#5684,.T.);
#3279=FACE_OUTER_BOUND('',#5685,.T.);
#3280=FACE_OUTER_BOUND('',#5686,.T.);
#3281=FACE_OUTER_BOUND('',#5687,.T.);
#3282=FACE_OUTER_BOUND('',#5688,.T.);
#3283=FACE_OUTER_BOUND('',#5689,.T.);
#3284=FACE_OUTER_BOUND('',#5690,.T.);
#3285=FACE_OUTER_BOUND('',#5691,.T.);
#3286=FACE_OUTER_BOUND('',#5692,.T.);
#3287=FACE_OUTER_BOUND('',#5693,.T.);
#3288=FACE_OUTER_BOUND('',#5694,.T.);
#3289=FACE_OUTER_BOUND('',#5695,.T.);
#3290=FACE_OUTER_BOUND('',#5696,.T.);
#3291=FACE_OUTER_BOUND('',#5697,.T.);
#3292=FACE_OUTER_BOUND('',#5698,.T.);
#3293=FACE_OUTER_BOUND('',#5699,.T.);
#3294=FACE_OUTER_BOUND('',#5700,.T.);
#3295=FACE_OUTER_BOUND('',#5701,.T.);
#3296=FACE_OUTER_BOUND('',#5702,.T.);
#3297=FACE_OUTER_BOUND('',#5703,.T.);
#3298=FACE_OUTER_BOUND('',#5704,.T.);
#3299=FACE_OUTER_BOUND('',#5705,.T.);
#3300=FACE_OUTER_BOUND('',#5706,.T.);
#3301=FACE_OUTER_BOUND('',#5707,.T.);
#3302=FACE_OUTER_BOUND('',#5708,.T.);
#3303=FACE_OUTER_BOUND('',#5709,.T.);
#3304=FACE_OUTER_BOUND('',#5710,.T.);
#3305=FACE_OUTER_BOUND('',#5711,.T.);
#3306=FACE_OUTER_BOUND('',#5712,.T.);
#3307=FACE_OUTER_BOUND('',#5713,.T.);
#3308=FACE_OUTER_BOUND('',#5714,.T.);
#3309=FACE_OUTER_BOUND('',#5715,.T.);
#3310=FACE_OUTER_BOUND('',#5716,.T.);
#3311=FACE_OUTER_BOUND('',#5717,.T.);
#3312=FACE_OUTER_BOUND('',#5718,.T.);
#3313=FACE_OUTER_BOUND('',#5719,.T.);
#3314=FACE_OUTER_BOUND('',#5720,.T.);
#3315=FACE_OUTER_BOUND('',#5721,.T.);
#3316=FACE_OUTER_BOUND('',#5722,.T.);
#3317=FACE_OUTER_BOUND('',#5723,.T.);
#3318=FACE_OUTER_BOUND('',#5724,.T.);
#3319=FACE_OUTER_BOUND('',#5725,.T.);
#3320=FACE_OUTER_BOUND('',#5726,.T.);
#3321=FACE_OUTER_BOUND('',#5727,.T.);
#3322=FACE_OUTER_BOUND('',#5728,.T.);
#3323=FACE_OUTER_BOUND('',#5729,.T.);
#3324=FACE_OUTER_BOUND('',#5730,.T.);
#3325=FACE_OUTER_BOUND('',#5731,.T.);
#3326=FACE_OUTER_BOUND('',#5732,.T.);
#3327=FACE_OUTER_BOUND('',#5733,.T.);
#3328=FACE_OUTER_BOUND('',#5734,.T.);
#3329=FACE_OUTER_BOUND('',#5735,.T.);
#3330=FACE_OUTER_BOUND('',#5736,.T.);
#3331=FACE_OUTER_BOUND('',#5737,.T.);
#3332=FACE_OUTER_BOUND('',#5738,.T.);
#3333=FACE_OUTER_BOUND('',#5739,.T.);
#3334=FACE_OUTER_BOUND('',#5740,.T.);
#3335=FACE_OUTER_BOUND('',#5741,.T.);
#3336=FACE_OUTER_BOUND('',#5742,.T.);
#3337=FACE_OUTER_BOUND('',#5743,.T.);
#3338=FACE_OUTER_BOUND('',#5744,.T.);
#3339=FACE_OUTER_BOUND('',#5745,.T.);
#3340=FACE_OUTER_BOUND('',#5746,.T.);
#3341=FACE_OUTER_BOUND('',#5747,.T.);
#3342=FACE_OUTER_BOUND('',#5748,.T.);
#3343=FACE_OUTER_BOUND('',#5749,.T.);
#3344=FACE_OUTER_BOUND('',#5750,.T.);
#3345=FACE_OUTER_BOUND('',#5751,.T.);
#3346=FACE_OUTER_BOUND('',#5752,.T.);
#3347=FACE_OUTER_BOUND('',#5753,.T.);
#3348=FACE_OUTER_BOUND('',#5754,.T.);
#3349=FACE_OUTER_BOUND('',#5755,.T.);
#3350=FACE_OUTER_BOUND('',#5756,.T.);
#3351=FACE_OUTER_BOUND('',#5757,.T.);
#3352=FACE_OUTER_BOUND('',#5758,.T.);
#3353=FACE_OUTER_BOUND('',#5759,.T.);
#3354=FACE_OUTER_BOUND('',#5760,.T.);
#3355=FACE_OUTER_BOUND('',#5761,.T.);
#3356=FACE_OUTER_BOUND('',#5762,.T.);
#3357=FACE_OUTER_BOUND('',#5763,.T.);
#3358=FACE_OUTER_BOUND('',#5764,.T.);
#3359=FACE_OUTER_BOUND('',#5765,.T.);
#3360=FACE_OUTER_BOUND('',#5766,.T.);
#3361=FACE_OUTER_BOUND('',#5767,.T.);
#3362=FACE_OUTER_BOUND('',#5768,.T.);
#3363=FACE_OUTER_BOUND('',#5769,.T.);
#3364=FACE_OUTER_BOUND('',#5770,.T.);
#3365=FACE_OUTER_BOUND('',#5771,.T.);
#3366=FACE_OUTER_BOUND('',#5772,.T.);
#3367=FACE_OUTER_BOUND('',#5773,.T.);
#3368=FACE_OUTER_BOUND('',#5774,.T.);
#3369=FACE_OUTER_BOUND('',#5775,.T.);
#3370=FACE_OUTER_BOUND('',#5776,.T.);
#3371=FACE_OUTER_BOUND('',#5777,.T.);
#3372=FACE_OUTER_BOUND('',#5778,.T.);
#3373=FACE_OUTER_BOUND('',#5779,.T.);
#3374=FACE_OUTER_BOUND('',#5780,.T.);
#3375=FACE_OUTER_BOUND('',#5781,.T.);
#3376=FACE_OUTER_BOUND('',#5782,.T.);
#3377=FACE_OUTER_BOUND('',#5783,.T.);
#3378=FACE_OUTER_BOUND('',#5784,.T.);
#3379=FACE_OUTER_BOUND('',#5785,.T.);
#3380=FACE_OUTER_BOUND('',#5786,.T.);
#3381=FACE_OUTER_BOUND('',#5787,.T.);
#3382=FACE_OUTER_BOUND('',#5788,.T.);
#3383=FACE_OUTER_BOUND('',#5789,.T.);
#3384=FACE_OUTER_BOUND('',#5790,.T.);
#3385=FACE_OUTER_BOUND('',#5791,.T.);
#3386=FACE_OUTER_BOUND('',#5792,.T.);
#3387=FACE_OUTER_BOUND('',#5793,.T.);
#3388=FACE_OUTER_BOUND('',#5794,.T.);
#3389=FACE_OUTER_BOUND('',#5795,.T.);
#3390=FACE_OUTER_BOUND('',#5796,.T.);
#3391=FACE_OUTER_BOUND('',#5797,.T.);
#3392=FACE_OUTER_BOUND('',#5798,.T.);
#3393=FACE_OUTER_BOUND('',#5799,.T.);
#3394=FACE_OUTER_BOUND('',#5800,.T.);
#3395=FACE_OUTER_BOUND('',#5801,.T.);
#3396=FACE_OUTER_BOUND('',#5802,.T.);
#3397=FACE_OUTER_BOUND('',#5803,.T.);
#3398=FACE_OUTER_BOUND('',#5804,.T.);
#3399=FACE_OUTER_BOUND('',#5805,.T.);
#3400=FACE_OUTER_BOUND('',#5806,.T.);
#3401=FACE_OUTER_BOUND('',#5807,.T.);
#3402=FACE_OUTER_BOUND('',#5808,.T.);
#3403=FACE_OUTER_BOUND('',#5809,.T.);
#3404=FACE_OUTER_BOUND('',#5810,.T.);
#3405=FACE_OUTER_BOUND('',#5811,.T.);
#4767=EDGE_LOOP('',(#26333,#26334,#26335,#26336));
#4768=EDGE_LOOP('',(#26337,#26338,#26339,#26340));
#4769=EDGE_LOOP('',(#26341,#26342,#26343));
#4770=EDGE_LOOP('',(#26344,#26345,#26346,#26347));
#4771=EDGE_LOOP('',(#26348,#26349,#26350,#26351));
#4772=EDGE_LOOP('',(#26352,#26353,#26354,#26355,#26356));
#4773=EDGE_LOOP('',(#26357,#26358,#26359,#26360));
#4774=EDGE_LOOP('',(#26361,#26362,#26363));
#4775=EDGE_LOOP('',(#26364,#26365,#26366));
#4776=EDGE_LOOP('',(#26367,#26368,#26369));
#4777=EDGE_LOOP('',(#26370,#26371,#26372,#26373,#26374,#26375,#26376,#26377));
#4778=EDGE_LOOP('',(#26378,#26379,#26380,#26381,#26382,#26383,#26384,#26385,
#26386,#26387,#26388,#26389,#26390,#26391,#26392,#26393,#26394,#26395,#26396,
#26397,#26398,#26399,#26400,#26401,#26402,#26403,#26404,#26405,#26406,#26407,
#26408,#26409,#26410,#26411,#26412,#26413,#26414,#26415,#26416,#26417,#26418,
#26419,#26420,#26421,#26422,#26423,#26424,#26425,#26426,#26427,#26428,#26429,
#26430,#26431,#26432,#26433,#26434,#26435,#26436,#26437,#26438,#26439,#26440,
#26441,#26442,#26443,#26444,#26445,#26446,#26447,#26448,#26449,#26450,#26451,
#26452,#26453,#26454,#26455,#26456,#26457,#26458,#26459,#26460,#26461,#26462,
#26463,#26464,#26465,#26466,#26467,#26468,#26469,#26470,#26471,#26472,#26473,
#26474,#26475,#26476,#26477,#26478,#26479,#26480,#26481,#26482,#26483,#26484,
#26485,#26486,#26487,#26488,#26489,#26490,#26491,#26492,#26493,#26494,#26495,
#26496,#26497,#26498,#26499,#26500,#26501,#26502,#26503,#26504,#26505,#26506,
#26507,#26508,#26509,#26510,#26511,#26512,#26513,#26514,#26515,#26516,#26517,
#26518,#26519,#26520,#26521,#26522,#26523,#26524,#26525,#26526,#26527,#26528,
#26529,#26530,#26531,#26532,#26533,#26534,#26535,#26536,#26537,#26538,#26539,
#26540,#26541,#26542,#26543,#26544,#26545,#26546,#26547,#26548,#26549,#26550,
#26551,#26552,#26553,#26554,#26555,#26556,#26557,#26558,#26559,#26560,#26561,
#26562,#26563,#26564,#26565,#26566,#26567,#26568,#26569,#26570,#26571,#26572));
#4779=EDGE_LOOP('',(#26573));
#4780=EDGE_LOOP('',(#26574,#26575,#26576,#26577));
#4781=EDGE_LOOP('',(#26578,#26579,#26580,#26581));
#4782=EDGE_LOOP('',(#26582,#26583,#26584,#26585));
#4783=EDGE_LOOP('',(#26586,#26587,#26588,#26589));
#4784=EDGE_LOOP('',(#26590,#26591,#26592,#26593));
#4785=EDGE_LOOP('',(#26594,#26595,#26596,#26597));
#4786=EDGE_LOOP('',(#26598,#26599,#26600));
#4787=EDGE_LOOP('',(#26601,#26602,#26603,#26604));
#4788=EDGE_LOOP('',(#26605,#26606,#26607,#26608));
#4789=EDGE_LOOP('',(#26609,#26610,#26611,#26612,#26613));
#4790=EDGE_LOOP('',(#26614,#26615,#26616,#26617));
#4791=EDGE_LOOP('',(#26618,#26619,#26620));
#4792=EDGE_LOOP('',(#26621,#26622,#26623));
#4793=EDGE_LOOP('',(#26624,#26625,#26626));
#4794=EDGE_LOOP('',(#26627,#26628,#26629,#26630,#26631,#26632,#26633,#26634));
#4795=EDGE_LOOP('',(#26635,#26636,#26637,#26638));
#4796=EDGE_LOOP('',(#26639,#26640,#26641,#26642));
#4797=EDGE_LOOP('',(#26643,#26644,#26645,#26646));
#4798=EDGE_LOOP('',(#26647,#26648,#26649,#26650));
#4799=EDGE_LOOP('',(#26651,#26652,#26653,#26654));
#4800=EDGE_LOOP('',(#26655,#26656,#26657,#26658));
#4801=EDGE_LOOP('',(#26659,#26660,#26661));
#4802=EDGE_LOOP('',(#26662,#26663,#26664,#26665));
#4803=EDGE_LOOP('',(#26666,#26667,#26668,#26669));
#4804=EDGE_LOOP('',(#26670,#26671,#26672,#26673,#26674));
#4805=EDGE_LOOP('',(#26675,#26676,#26677,#26678));
#4806=EDGE_LOOP('',(#26679,#26680,#26681));
#4807=EDGE_LOOP('',(#26682,#26683,#26684));
#4808=EDGE_LOOP('',(#26685,#26686,#26687));
#4809=EDGE_LOOP('',(#26688,#26689,#26690,#26691,#26692,#26693,#26694,#26695));
#4810=EDGE_LOOP('',(#26696,#26697,#26698,#26699));
#4811=EDGE_LOOP('',(#26700,#26701,#26702,#26703));
#4812=EDGE_LOOP('',(#26704,#26705,#26706,#26707));
#4813=EDGE_LOOP('',(#26708,#26709,#26710,#26711));
#4814=EDGE_LOOP('',(#26712,#26713,#26714,#26715));
#4815=EDGE_LOOP('',(#26716,#26717,#26718,#26719));
#4816=EDGE_LOOP('',(#26720,#26721,#26722));
#4817=EDGE_LOOP('',(#26723,#26724,#26725,#26726));
#4818=EDGE_LOOP('',(#26727,#26728,#26729,#26730,#26731));
#4819=EDGE_LOOP('',(#26732,#26733,#26734));
#4820=EDGE_LOOP('',(#26735,#26736,#26737,#26738));
#4821=EDGE_LOOP('',(#26739,#26740,#26741,#26742));
#4822=EDGE_LOOP('',(#26743,#26744,#26745));
#4823=EDGE_LOOP('',(#26746,#26747,#26748));
#4824=EDGE_LOOP('',(#26749,#26750,#26751,#26752));
#4825=EDGE_LOOP('',(#26753,#26754,#26755,#26756));
#4826=EDGE_LOOP('',(#26757,#26758,#26759,#26760));
#4827=EDGE_LOOP('',(#26761,#26762,#26763,#26764));
#4828=EDGE_LOOP('',(#26765,#26766,#26767,#26768));
#4829=EDGE_LOOP('',(#26769,#26770,#26771,#26772,#26773,#26774));
#4830=EDGE_LOOP('',(#26775,#26776,#26777,#26778));
#4831=EDGE_LOOP('',(#26779,#26780,#26781,#26782));
#4832=EDGE_LOOP('',(#26783,#26784,#26785));
#4833=EDGE_LOOP('',(#26786,#26787,#26788,#26789));
#4834=EDGE_LOOP('',(#26790,#26791,#26792,#26793,#26794));
#4835=EDGE_LOOP('',(#26795,#26796,#26797));
#4836=EDGE_LOOP('',(#26798,#26799,#26800,#26801));
#4837=EDGE_LOOP('',(#26802,#26803,#26804,#26805));
#4838=EDGE_LOOP('',(#26806,#26807,#26808));
#4839=EDGE_LOOP('',(#26809,#26810,#26811));
#4840=EDGE_LOOP('',(#26812,#26813,#26814,#26815));
#4841=EDGE_LOOP('',(#26816,#26817,#26818,#26819));
#4842=EDGE_LOOP('',(#26820,#26821,#26822,#26823));
#4843=EDGE_LOOP('',(#26824,#26825,#26826,#26827));
#4844=EDGE_LOOP('',(#26828,#26829,#26830,#26831));
#4845=EDGE_LOOP('',(#26832,#26833,#26834,#26835,#26836,#26837));
#4846=EDGE_LOOP('',(#26838,#26839,#26840,#26841));
#4847=EDGE_LOOP('',(#26842,#26843,#26844,#26845));
#4848=EDGE_LOOP('',(#26846,#26847,#26848));
#4849=EDGE_LOOP('',(#26849,#26850,#26851,#26852));
#4850=EDGE_LOOP('',(#26853,#26854,#26855));
#4851=EDGE_LOOP('',(#26856,#26857,#26858,#26859,#26860,#26861,#26862,#26863,
#26864,#26865,#26866,#26867,#26868,#26869,#26870,#26871,#26872,#26873,#26874,
#26875,#26876,#26877,#26878,#26879,#26880,#26881,#26882,#26883,#26884,#26885,
#26886,#26887,#26888,#26889,#26890,#26891,#26892,#26893,#26894,#26895,#26896,
#26897,#26898,#26899,#26900,#26901,#26902,#26903,#26904,#26905,#26906,#26907,
#26908,#26909,#26910,#26911,#26912,#26913,#26914,#26915,#26916,#26917,#26918,
#26919,#26920,#26921,#26922,#26923,#26924,#26925,#26926,#26927,#26928,#26929,
#26930,#26931,#26932,#26933,#26934,#26935,#26936,#26937,#26938,#26939,#26940,
#26941,#26942,#26943,#26944,#26945,#26946,#26947,#26948,#26949,#26950,#26951,
#26952,#26953,#26954,#26955,#26956,#26957,#26958,#26959,#26960,#26961,#26962,
#26963,#26964,#26965,#26966,#26967,#26968,#26969,#26970,#26971,#26972,#26973,
#26974,#26975,#26976,#26977,#26978,#26979,#26980,#26981,#26982,#26983,#26984,
#26985,#26986,#26987,#26988,#26989,#26990,#26991,#26992,#26993,#26994,#26995,
#26996,#26997,#26998,#26999,#27000,#27001,#27002,#27003,#27004,#27005,#27006,
#27007,#27008,#27009,#27010,#27011,#27012,#27013,#27014,#27015,#27016,#27017,
#27018,#27019,#27020,#27021,#27022,#27023,#27024,#27025,#27026,#27027,#27028,
#27029,#27030,#27031,#27032,#27033,#27034,#27035,#27036,#27037,#27038,#27039,
#27040,#27041,#27042,#27043,#27044,#27045,#27046,#27047));
#4852=EDGE_LOOP('',(#27048));
#4853=EDGE_LOOP('',(#27049,#27050,#27051,#27052));
#4854=EDGE_LOOP('',(#27053,#27054,#27055,#27056));
#4855=EDGE_LOOP('',(#27057,#27058,#27059,#27060));
#4856=EDGE_LOOP('',(#27061,#27062,#27063,#27064));
#4857=EDGE_LOOP('',(#27065,#27066,#27067,#27068));
#4858=EDGE_LOOP('',(#27069,#27070,#27071,#27072));
#4859=EDGE_LOOP('',(#27073,#27074,#27075));
#4860=EDGE_LOOP('',(#27076,#27077,#27078,#27079));
#4861=EDGE_LOOP('',(#27080,#27081,#27082));
#4862=EDGE_LOOP('',(#27083,#27084,#27085,#27086));
#4863=EDGE_LOOP('',(#27087,#27088,#27089,#27090));
#4864=EDGE_LOOP('',(#27091,#27092,#27093,#27094));
#4865=EDGE_LOOP('',(#27095,#27096,#27097,#27098));
#4866=EDGE_LOOP('',(#27099,#27100,#27101,#27102));
#4867=EDGE_LOOP('',(#27103,#27104,#27105,#27106));
#4868=EDGE_LOOP('',(#27107,#27108,#27109));
#4869=EDGE_LOOP('',(#27110,#27111,#27112,#27113));
#4870=EDGE_LOOP('',(#27114,#27115,#27116));
#4871=EDGE_LOOP('',(#27117,#27118,#27119,#27120));
#4872=EDGE_LOOP('',(#27121,#27122,#27123,#27124));
#4873=EDGE_LOOP('',(#27125,#27126,#27127,#27128));
#4874=EDGE_LOOP('',(#27129,#27130,#27131,#27132));
#4875=EDGE_LOOP('',(#27133,#27134,#27135,#27136));
#4876=EDGE_LOOP('',(#27137,#27138,#27139,#27140));
#4877=EDGE_LOOP('',(#27141,#27142,#27143,#27144));
#4878=EDGE_LOOP('',(#27145,#27146,#27147));
#4879=EDGE_LOOP('',(#27148,#27149,#27150,#27151));
#4880=EDGE_LOOP('',(#27152,#27153,#27154,#27155,#27156));
#4881=EDGE_LOOP('',(#27157,#27158,#27159));
#4882=EDGE_LOOP('',(#27160,#27161,#27162,#27163));
#4883=EDGE_LOOP('',(#27164,#27165,#27166));
#4884=EDGE_LOOP('',(#27167,#27168,#27169));
#4885=EDGE_LOOP('',(#27170,#27171,#27172,#27173));
#4886=EDGE_LOOP('',(#27174,#27175,#27176,#27177));
#4887=EDGE_LOOP('',(#27178,#27179,#27180,#27181,#27182,#27183,#27184));
#4888=EDGE_LOOP('',(#27185,#27186,#27187,#27188));
#4889=EDGE_LOOP('',(#27189,#27190,#27191,#27192,#27193));
#4890=EDGE_LOOP('',(#27194,#27195,#27196,#27197));
#4891=EDGE_LOOP('',(#27198,#27199,#27200,#27201));
#4892=EDGE_LOOP('',(#27202,#27203,#27204));
#4893=EDGE_LOOP('',(#27205,#27206,#27207,#27208));
#4894=EDGE_LOOP('',(#27209,#27210,#27211));
#4895=EDGE_LOOP('',(#27212,#27213,#27214,#27215));
#4896=EDGE_LOOP('',(#27216,#27217,#27218,#27219));
#4897=EDGE_LOOP('',(#27220,#27221,#27222,#27223));
#4898=EDGE_LOOP('',(#27224,#27225,#27226,#27227));
#4899=EDGE_LOOP('',(#27228,#27229,#27230,#27231));
#4900=EDGE_LOOP('',(#27232,#27233,#27234,#27235));
#4901=EDGE_LOOP('',(#27236,#27237,#27238));
#4902=EDGE_LOOP('',(#27239,#27240,#27241,#27242));
#4903=EDGE_LOOP('',(#27243,#27244,#27245));
#4904=EDGE_LOOP('',(#27246,#27247,#27248,#27249));
#4905=EDGE_LOOP('',(#27250,#27251,#27252,#27253));
#4906=EDGE_LOOP('',(#27254,#27255,#27256,#27257));
#4907=EDGE_LOOP('',(#27258,#27259,#27260,#27261));
#4908=EDGE_LOOP('',(#27262,#27263,#27264,#27265));
#4909=EDGE_LOOP('',(#27266,#27267,#27268,#27269));
#4910=EDGE_LOOP('',(#27270,#27271,#27272));
#4911=EDGE_LOOP('',(#27273,#27274,#27275,#27276));
#4912=EDGE_LOOP('',(#27277,#27278,#27279));
#4913=EDGE_LOOP('',(#27280,#27281,#27282,#27283));
#4914=EDGE_LOOP('',(#27284,#27285,#27286,#27287));
#4915=EDGE_LOOP('',(#27288,#27289,#27290,#27291));
#4916=EDGE_LOOP('',(#27292,#27293,#27294,#27295));
#4917=EDGE_LOOP('',(#27296,#27297,#27298,#27299));
#4918=EDGE_LOOP('',(#27300,#27301,#27302));
#4919=EDGE_LOOP('',(#27303,#27304,#27305,#27306));
#4920=EDGE_LOOP('',(#27307,#27308,#27309,#27310,#27311));
#4921=EDGE_LOOP('',(#27312,#27313,#27314));
#4922=EDGE_LOOP('',(#27315,#27316,#27317,#27318));
#4923=EDGE_LOOP('',(#27319,#27320,#27321));
#4924=EDGE_LOOP('',(#27322,#27323,#27324));
#4925=EDGE_LOOP('',(#27325,#27326,#27327,#27328));
#4926=EDGE_LOOP('',(#27329,#27330,#27331,#27332));
#4927=EDGE_LOOP('',(#27333,#27334,#27335,#27336,#27337,#27338,#27339));
#4928=EDGE_LOOP('',(#27340,#27341,#27342,#27343));
#4929=EDGE_LOOP('',(#27344,#27345,#27346,#27347,#27348));
#4930=EDGE_LOOP('',(#27349,#27350,#27351,#27352));
#4931=EDGE_LOOP('',(#27353,#27354,#27355,#27356));
#4932=EDGE_LOOP('',(#27357,#27358,#27359));
#4933=EDGE_LOOP('',(#27360,#27361,#27362,#27363));
#4934=EDGE_LOOP('',(#27364,#27365,#27366));
#4935=EDGE_LOOP('',(#27367,#27368,#27369,#27370,#27371,#27372,#27373,#27374));
#4936=EDGE_LOOP('',(#27375,#27376,#27377,#27378));
#4937=EDGE_LOOP('',(#27379,#27380,#27381,#27382));
#4938=EDGE_LOOP('',(#27383,#27384,#27385));
#4939=EDGE_LOOP('',(#27386,#27387,#27388));
#4940=EDGE_LOOP('',(#27389,#27390,#27391,#27392,#27393,#27394,#27395,#27396));
#4941=EDGE_LOOP('',(#27397,#27398,#27399,#27400));
#4942=EDGE_LOOP('',(#27401,#27402,#27403,#27404));
#4943=EDGE_LOOP('',(#27405,#27406,#27407));
#4944=EDGE_LOOP('',(#27408,#27409,#27410,#27411));
#4945=EDGE_LOOP('',(#27412,#27413,#27414));
#4946=EDGE_LOOP('',(#27415,#27416,#27417,#27418));
#4947=EDGE_LOOP('',(#27419,#27420,#27421,#27422));
#4948=EDGE_LOOP('',(#27423,#27424,#27425,#27426));
#4949=EDGE_LOOP('',(#27427,#27428,#27429,#27430));
#4950=EDGE_LOOP('',(#27431,#27432,#27433,#27434));
#4951=EDGE_LOOP('',(#27435,#27436,#27437,#27438));
#4952=EDGE_LOOP('',(#27439,#27440,#27441));
#4953=EDGE_LOOP('',(#27442,#27443,#27444));
#4954=EDGE_LOOP('',(#27445,#27446,#27447,#27448,#27449,#27450,#27451,#27452));
#4955=EDGE_LOOP('',(#27453,#27454,#27455,#27456));
#4956=EDGE_LOOP('',(#27457,#27458,#27459,#27460));
#4957=EDGE_LOOP('',(#27461,#27462,#27463));
#4958=EDGE_LOOP('',(#27464,#27465,#27466,#27467));
#4959=EDGE_LOOP('',(#27468,#27469,#27470));
#4960=EDGE_LOOP('',(#27471,#27472,#27473,#27474));
#4961=EDGE_LOOP('',(#27475,#27476,#27477,#27478));
#4962=EDGE_LOOP('',(#27479,#27480,#27481,#27482));
#4963=EDGE_LOOP('',(#27483,#27484,#27485,#27486));
#4964=EDGE_LOOP('',(#27487,#27488,#27489));
#4965=EDGE_LOOP('',(#27490,#27491,#27492));
#4966=EDGE_LOOP('',(#27493,#27494,#27495,#27496));
#4967=EDGE_LOOP('',(#27497,#27498,#27499,#27500,#27501,#27502,#27503,#27504));
#4968=EDGE_LOOP('',(#27505,#27506,#27507,#27508));
#4969=EDGE_LOOP('',(#27509,#27510,#27511,#27512));
#4970=EDGE_LOOP('',(#27513,#27514,#27515));
#4971=EDGE_LOOP('',(#27516,#27517,#27518,#27519));
#4972=EDGE_LOOP('',(#27520,#27521,#27522));
#4973=EDGE_LOOP('',(#27523,#27524,#27525,#27526,#27527,#27528,#27529,#27530));
#4974=EDGE_LOOP('',(#27531,#27532,#27533,#27534));
#4975=EDGE_LOOP('',(#27535,#27536,#27537,#27538,#27539,#27540,#27541,#27542));
#4976=EDGE_LOOP('',(#27543,#27544,#27545,#27546));
#4977=EDGE_LOOP('',(#27547,#27548,#27549,#27550));
#4978=EDGE_LOOP('',(#27551,#27552,#27553));
#4979=EDGE_LOOP('',(#27554,#27555,#27556,#27557));
#4980=EDGE_LOOP('',(#27558,#27559,#27560));
#4981=EDGE_LOOP('',(#27561,#27562,#27563,#27564));
#4982=EDGE_LOOP('',(#27565,#27566,#27567,#27568));
#4983=EDGE_LOOP('',(#27569,#27570,#27571,#27572));
#4984=EDGE_LOOP('',(#27573,#27574,#27575,#27576));
#4985=EDGE_LOOP('',(#27577,#27578,#27579));
#4986=EDGE_LOOP('',(#27580,#27581,#27582,#27583));
#4987=EDGE_LOOP('',(#27584,#27585,#27586));
#4988=EDGE_LOOP('',(#27587,#27588,#27589,#27590));
#4989=EDGE_LOOP('',(#27591,#27592,#27593,#27594));
#4990=EDGE_LOOP('',(#27595,#27596,#27597,#27598));
#4991=EDGE_LOOP('',(#27599,#27600,#27601,#27602));
#4992=EDGE_LOOP('',(#27603,#27604,#27605,#27606));
#4993=EDGE_LOOP('',(#27607,#27608,#27609,#27610));
#4994=EDGE_LOOP('',(#27611,#27612,#27613));
#4995=EDGE_LOOP('',(#27614,#27615,#27616,#27617));
#4996=EDGE_LOOP('',(#27618,#27619,#27620));
#4997=EDGE_LOOP('',(#27621,#27622,#27623,#27624));
#4998=EDGE_LOOP('',(#27625,#27626,#27627,#27628));
#4999=EDGE_LOOP('',(#27629,#27630,#27631,#27632));
#5000=EDGE_LOOP('',(#27633,#27634,#27635,#27636));
#5001=EDGE_LOOP('',(#27637,#27638,#27639,#27640));
#5002=EDGE_LOOP('',(#27641,#27642,#27643,#27644));
#5003=EDGE_LOOP('',(#27645,#27646,#27647));
#5004=EDGE_LOOP('',(#27648,#27649,#27650));
#5005=EDGE_LOOP('',(#27651,#27652,#27653,#27654,#27655,#27656,#27657,#27658));
#5006=EDGE_LOOP('',(#27659,#27660,#27661,#27662));
#5007=EDGE_LOOP('',(#27663,#27664,#27665,#27666));
#5008=EDGE_LOOP('',(#27667,#27668,#27669));
#5009=EDGE_LOOP('',(#27670,#27671,#27672,#27673));
#5010=EDGE_LOOP('',(#27674,#27675,#27676));
#5011=EDGE_LOOP('',(#27677,#27678,#27679,#27680));
#5012=EDGE_LOOP('',(#27681,#27682,#27683,#27684));
#5013=EDGE_LOOP('',(#27685,#27686,#27687,#27688));
#5014=EDGE_LOOP('',(#27689,#27690,#27691,#27692));
#5015=EDGE_LOOP('',(#27693,#27694,#27695,#27696));
#5016=EDGE_LOOP('',(#27697,#27698,#27699,#27700));
#5017=EDGE_LOOP('',(#27701,#27702,#27703));
#5018=EDGE_LOOP('',(#27704,#27705,#27706));
#5019=EDGE_LOOP('',(#27707,#27708,#27709,#27710,#27711,#27712,#27713,#27714));
#5020=EDGE_LOOP('',(#27715,#27716,#27717,#27718));
#5021=EDGE_LOOP('',(#27719,#27720,#27721,#27722,#27723,#27724,#27725,#27726));
#5022=EDGE_LOOP('',(#27727,#27728,#27729,#27730));
#5023=EDGE_LOOP('',(#27731,#27732,#27733,#27734));
#5024=EDGE_LOOP('',(#27735,#27736,#27737));
#5025=EDGE_LOOP('',(#27738,#27739,#27740,#27741));
#5026=EDGE_LOOP('',(#27742,#27743,#27744));
#5027=EDGE_LOOP('',(#27745,#27746,#27747,#27748));
#5028=EDGE_LOOP('',(#27749,#27750,#27751,#27752));
#5029=EDGE_LOOP('',(#27753,#27754,#27755,#27756));
#5030=EDGE_LOOP('',(#27757,#27758,#27759,#27760));
#5031=EDGE_LOOP('',(#27761,#27762,#27763,#27764));
#5032=EDGE_LOOP('',(#27765,#27766,#27767,#27768));
#5033=EDGE_LOOP('',(#27769,#27770,#27771));
#5034=EDGE_LOOP('',(#27772,#27773,#27774,#27775));
#5035=EDGE_LOOP('',(#27776,#27777,#27778));
#5036=EDGE_LOOP('',(#27779,#27780,#27781,#27782));
#5037=EDGE_LOOP('',(#27783,#27784,#27785,#27786));
#5038=EDGE_LOOP('',(#27787,#27788,#27789,#27790));
#5039=EDGE_LOOP('',(#27791,#27792,#27793,#27794));
#5040=EDGE_LOOP('',(#27795,#27796,#27797,#27798));
#5041=EDGE_LOOP('',(#27799,#27800,#27801,#27802));
#5042=EDGE_LOOP('',(#27803,#27804,#27805));
#5043=EDGE_LOOP('',(#27806,#27807,#27808,#27809));
#5044=EDGE_LOOP('',(#27810,#27811,#27812));
#5045=EDGE_LOOP('',(#27813,#27814,#27815,#27816));
#5046=EDGE_LOOP('',(#27817,#27818,#27819,#27820));
#5047=EDGE_LOOP('',(#27821,#27822,#27823,#27824));
#5048=EDGE_LOOP('',(#27825,#27826,#27827,#27828));
#5049=EDGE_LOOP('',(#27829,#27830,#27831));
#5050=EDGE_LOOP('',(#27832,#27833,#27834));
#5051=EDGE_LOOP('',(#27835,#27836,#27837,#27838,#27839,#27840,#27841,#27842));
#5052=EDGE_LOOP('',(#27843,#27844,#27845,#27846));
#5053=EDGE_LOOP('',(#27847,#27848,#27849,#27850));
#5054=EDGE_LOOP('',(#27851,#27852,#27853));
#5055=EDGE_LOOP('',(#27854,#27855,#27856));
#5056=EDGE_LOOP('',(#27857,#27858,#27859,#27860,#27861,#27862,#27863,#27864));
#5057=EDGE_LOOP('',(#27865,#27866,#27867,#27868));
#5058=EDGE_LOOP('',(#27869,#27870,#27871,#27872));
#5059=EDGE_LOOP('',(#27873,#27874,#27875));
#5060=EDGE_LOOP('',(#27876,#27877,#27878,#27879));
#5061=EDGE_LOOP('',(#27880,#27881,#27882));
#5062=EDGE_LOOP('',(#27883,#27884,#27885,#27886));
#5063=EDGE_LOOP('',(#27887,#27888,#27889,#27890));
#5064=EDGE_LOOP('',(#27891,#27892,#27893,#27894));
#5065=EDGE_LOOP('',(#27895,#27896,#27897,#27898));
#5066=EDGE_LOOP('',(#27899,#27900,#27901,#27902));
#5067=EDGE_LOOP('',(#27903,#27904,#27905,#27906));
#5068=EDGE_LOOP('',(#27907,#27908,#27909));
#5069=EDGE_LOOP('',(#27910,#27911,#27912));
#5070=EDGE_LOOP('',(#27913,#27914,#27915,#27916,#27917,#27918,#27919,#27920));
#5071=EDGE_LOOP('',(#27921,#27922,#27923,#27924));
#5072=EDGE_LOOP('',(#27925,#27926,#27927,#27928,#27929,#27930,#27931,#27932));
#5073=EDGE_LOOP('',(#27933,#27934,#27935,#27936));
#5074=EDGE_LOOP('',(#27937,#27938,#27939,#27940,#27941,#27942,#27943,#27944));
#5075=EDGE_LOOP('',(#27945,#27946,#27947,#27948));
#5076=EDGE_LOOP('',(#27949,#27950,#27951,#27952));
#5077=EDGE_LOOP('',(#27953,#27954,#27955));
#5078=EDGE_LOOP('',(#27956,#27957,#27958,#27959));
#5079=EDGE_LOOP('',(#27960,#27961,#27962));
#5080=EDGE_LOOP('',(#27963,#27964,#27965,#27966,#27967,#27968,#27969,#27970));
#5081=EDGE_LOOP('',(#27971,#27972,#27973,#27974));
#5082=EDGE_LOOP('',(#27975,#27976,#27977,#27978));
#5083=EDGE_LOOP('',(#27979,#27980,#27981));
#5084=EDGE_LOOP('',(#27982,#27983,#27984));
#5085=EDGE_LOOP('',(#27985,#27986,#27987,#27988,#27989,#27990,#27991,#27992));
#5086=EDGE_LOOP('',(#27993,#27994,#27995,#27996));
#5087=EDGE_LOOP('',(#27997,#27998,#27999,#28000));
#5088=EDGE_LOOP('',(#28001,#28002,#28003));
#5089=EDGE_LOOP('',(#28004,#28005,#28006,#28007));
#5090=EDGE_LOOP('',(#28008,#28009,#28010));
#5091=EDGE_LOOP('',(#28011,#28012,#28013,#28014));
#5092=EDGE_LOOP('',(#28015,#28016,#28017,#28018));
#5093=EDGE_LOOP('',(#28019,#28020,#28021,#28022));
#5094=EDGE_LOOP('',(#28023,#28024,#28025,#28026));
#5095=EDGE_LOOP('',(#28027,#28028,#28029));
#5096=EDGE_LOOP('',(#28030,#28031,#28032));
#5097=EDGE_LOOP('',(#28033,#28034,#28035,#28036,#28037,#28038,#28039,#28040));
#5098=EDGE_LOOP('',(#28041,#28042,#28043,#28044));
#5099=EDGE_LOOP('',(#28045,#28046,#28047,#28048));
#5100=EDGE_LOOP('',(#28049,#28050,#28051));
#5101=EDGE_LOOP('',(#28052,#28053,#28054,#28055));
#5102=EDGE_LOOP('',(#28056,#28057,#28058));
#5103=EDGE_LOOP('',(#28059,#28060,#28061,#28062));
#5104=EDGE_LOOP('',(#28063,#28064,#28065,#28066));
#5105=EDGE_LOOP('',(#28067,#28068,#28069,#28070));
#5106=EDGE_LOOP('',(#28071,#28072,#28073,#28074));
#5107=EDGE_LOOP('',(#28075,#28076,#28077,#28078));
#5108=EDGE_LOOP('',(#28079,#28080,#28081,#28082));
#5109=EDGE_LOOP('',(#28083,#28084,#28085));
#5110=EDGE_LOOP('',(#28086,#28087,#28088));
#5111=EDGE_LOOP('',(#28089,#28090,#28091,#28092,#28093,#28094,#28095,#28096));
#5112=EDGE_LOOP('',(#28097,#28098,#28099,#28100));
#5113=EDGE_LOOP('',(#28101,#28102,#28103,#28104,#28105,#28106,#28107,#28108));
#5114=EDGE_LOOP('',(#28109,#28110,#28111,#28112));
#5115=EDGE_LOOP('',(#28113,#28114,#28115,#28116));
#5116=EDGE_LOOP('',(#28117,#28118,#28119));
#5117=EDGE_LOOP('',(#28120,#28121,#28122,#28123));
#5118=EDGE_LOOP('',(#28124,#28125,#28126));
#5119=EDGE_LOOP('',(#28127,#28128,#28129,#28130,#28131,#28132,#28133,#28134));
#5120=EDGE_LOOP('',(#28135,#28136,#28137,#28138));
#5121=EDGE_LOOP('',(#28139,#28140,#28141,#28142,#28143,#28144,#28145,#28146));
#5122=EDGE_LOOP('',(#28147,#28148,#28149,#28150));
#5123=EDGE_LOOP('',(#28151,#28152,#28153,#28154));
#5124=EDGE_LOOP('',(#28155,#28156,#28157));
#5125=EDGE_LOOP('',(#28158,#28159,#28160,#28161));
#5126=EDGE_LOOP('',(#28162,#28163,#28164));
#5127=EDGE_LOOP('',(#28165,#28166,#28167,#28168));
#5128=EDGE_LOOP('',(#28169,#28170,#28171,#28172));
#5129=EDGE_LOOP('',(#28173,#28174,#28175,#28176));
#5130=EDGE_LOOP('',(#28177,#28178,#28179,#28180));
#5131=EDGE_LOOP('',(#28181,#28182,#28183,#28184));
#5132=EDGE_LOOP('',(#28185,#28186,#28187,#28188));
#5133=EDGE_LOOP('',(#28189,#28190,#28191));
#5134=EDGE_LOOP('',(#28192,#28193,#28194,#28195));
#5135=EDGE_LOOP('',(#28196,#28197,#28198));
#5136=EDGE_LOOP('',(#28199,#28200,#28201,#28202));
#5137=EDGE_LOOP('',(#28203,#28204,#28205,#28206));
#5138=EDGE_LOOP('',(#28207,#28208,#28209,#28210));
#5139=EDGE_LOOP('',(#28211,#28212,#28213,#28214));
#5140=EDGE_LOOP('',(#28215,#28216,#28217,#28218));
#5141=EDGE_LOOP('',(#28219,#28220,#28221,#28222));
#5142=EDGE_LOOP('',(#28223,#28224,#28225));
#5143=EDGE_LOOP('',(#28226,#28227,#28228,#28229));
#5144=EDGE_LOOP('',(#28230,#28231,#28232));
#5145=EDGE_LOOP('',(#28233,#28234,#28235,#28236));
#5146=EDGE_LOOP('',(#28237,#28238,#28239,#28240));
#5147=EDGE_LOOP('',(#28241,#28242,#28243,#28244));
#5148=EDGE_LOOP('',(#28245,#28246,#28247,#28248));
#5149=EDGE_LOOP('',(#28249,#28250,#28251));
#5150=EDGE_LOOP('',(#28252,#28253,#28254,#28255));
#5151=EDGE_LOOP('',(#28256,#28257,#28258));
#5152=EDGE_LOOP('',(#28259,#28260,#28261,#28262));
#5153=EDGE_LOOP('',(#28263,#28264,#28265,#28266));
#5154=EDGE_LOOP('',(#28267,#28268,#28269,#28270));
#5155=EDGE_LOOP('',(#28271,#28272,#28273,#28274));
#5156=EDGE_LOOP('',(#28275,#28276,#28277,#28278));
#5157=EDGE_LOOP('',(#28279,#28280,#28281,#28282));
#5158=EDGE_LOOP('',(#28283,#28284,#28285));
#5159=EDGE_LOOP('',(#28286,#28287,#28288));
#5160=EDGE_LOOP('',(#28289,#28290,#28291,#28292,#28293,#28294,#28295,#28296));
#5161=EDGE_LOOP('',(#28297,#28298,#28299,#28300));
#5162=EDGE_LOOP('',(#28301,#28302,#28303,#28304));
#5163=EDGE_LOOP('',(#28305,#28306,#28307));
#5164=EDGE_LOOP('',(#28308,#28309,#28310,#28311));
#5165=EDGE_LOOP('',(#28312,#28313,#28314));
#5166=EDGE_LOOP('',(#28315,#28316,#28317,#28318,#28319,#28320,#28321,#28322));
#5167=EDGE_LOOP('',(#28323,#28324,#28325,#28326));
#5168=EDGE_LOOP('',(#28327,#28328,#28329,#28330));
#5169=EDGE_LOOP('',(#28331,#28332,#28333));
#5170=EDGE_LOOP('',(#28334,#28335,#28336,#28337));
#5171=EDGE_LOOP('',(#28338,#28339,#28340));
#5172=EDGE_LOOP('',(#28341,#28342,#28343,#28344));
#5173=EDGE_LOOP('',(#28345,#28346,#28347,#28348));
#5174=EDGE_LOOP('',(#28349,#28350,#28351,#28352));
#5175=EDGE_LOOP('',(#28353,#28354,#28355,#28356));
#5176=EDGE_LOOP('',(#28357,#28358,#28359,#28360));
#5177=EDGE_LOOP('',(#28361,#28362,#28363,#28364));
#5178=EDGE_LOOP('',(#28365,#28366,#28367));
#5179=EDGE_LOOP('',(#28368,#28369,#28370,#28371));
#5180=EDGE_LOOP('',(#28372,#28373,#28374));
#5181=EDGE_LOOP('',(#28375,#28376,#28377,#28378));
#5182=EDGE_LOOP('',(#28379,#28380,#28381,#28382));
#5183=EDGE_LOOP('',(#28383,#28384,#28385,#28386));
#5184=EDGE_LOOP('',(#28387,#28388,#28389,#28390));
#5185=EDGE_LOOP('',(#28391,#28392,#28393));
#5186=EDGE_LOOP('',(#28394,#28395,#28396));
#5187=EDGE_LOOP('',(#28397,#28398,#28399,#28400,#28401,#28402,#28403,#28404));
#5188=EDGE_LOOP('',(#28405,#28406,#28407,#28408));
#5189=EDGE_LOOP('',(#28409,#28410,#28411,#28412));
#5190=EDGE_LOOP('',(#28413,#28414,#28415));
#5191=EDGE_LOOP('',(#28416,#28417,#28418));
#5192=EDGE_LOOP('',(#28419,#28420,#28421,#28422,#28423,#28424,#28425,#28426));
#5193=EDGE_LOOP('',(#28427,#28428,#28429,#28430));
#5194=EDGE_LOOP('',(#28431,#28432,#28433,#28434));
#5195=EDGE_LOOP('',(#28435,#28436,#28437));
#5196=EDGE_LOOP('',(#28438,#28439,#28440,#28441));
#5197=EDGE_LOOP('',(#28442,#28443,#28444));
#5198=EDGE_LOOP('',(#28445,#28446,#28447,#28448));
#5199=EDGE_LOOP('',(#28449,#28450,#28451,#28452));
#5200=EDGE_LOOP('',(#28453,#28454,#28455,#28456));
#5201=EDGE_LOOP('',(#28457,#28458,#28459,#28460));
#5202=EDGE_LOOP('',(#28461,#28462,#28463,#28464));
#5203=EDGE_LOOP('',(#28465,#28466,#28467,#28468));
#5204=EDGE_LOOP('',(#28469,#28470,#28471));
#5205=EDGE_LOOP('',(#28472,#28473,#28474));
#5206=EDGE_LOOP('',(#28475,#28476,#28477,#28478));
#5207=EDGE_LOOP('',(#28479,#28480,#28481,#28482,#28483,#28484,#28485,#28486));
#5208=EDGE_LOOP('',(#28487,#28488,#28489,#28490));
#5209=EDGE_LOOP('',(#28491,#28492,#28493,#28494));
#5210=EDGE_LOOP('',(#28495,#28496,#28497));
#5211=EDGE_LOOP('',(#28498,#28499,#28500));
#5212=EDGE_LOOP('',(#28501,#28502,#28503,#28504,#28505,#28506,#28507,#28508));
#5213=EDGE_LOOP('',(#28509,#28510,#28511,#28512));
#5214=EDGE_LOOP('',(#28513,#28514,#28515,#28516,#28517,#28518,#28519,#28520));
#5215=EDGE_LOOP('',(#28521,#28522,#28523,#28524));
#5216=EDGE_LOOP('',(#28525,#28526,#28527,#28528,#28529,#28530,#28531,#28532));
#5217=EDGE_LOOP('',(#28533,#28534,#28535,#28536));
#5218=EDGE_LOOP('',(#28537,#28538,#28539,#28540));
#5219=EDGE_LOOP('',(#28541,#28542,#28543));
#5220=EDGE_LOOP('',(#28544,#28545,#28546,#28547));
#5221=EDGE_LOOP('',(#28548,#28549,#28550));
#5222=EDGE_LOOP('',(#28551,#28552,#28553,#28554,#28555,#28556,#28557,#28558));
#5223=EDGE_LOOP('',(#28559,#28560,#28561,#28562));
#5224=EDGE_LOOP('',(#28563,#28564,#28565,#28566));
#5225=EDGE_LOOP('',(#28567,#28568,#28569));
#5226=EDGE_LOOP('',(#28570,#28571,#28572));
#5227=EDGE_LOOP('',(#28573,#28574,#28575,#28576,#28577,#28578,#28579,#28580));
#5228=EDGE_LOOP('',(#28581,#28582,#28583,#28584));
#5229=EDGE_LOOP('',(#28585,#28586,#28587,#28588));
#5230=EDGE_LOOP('',(#28589,#28590,#28591));
#5231=EDGE_LOOP('',(#28592,#28593,#28594,#28595));
#5232=EDGE_LOOP('',(#28596,#28597,#28598));
#5233=EDGE_LOOP('',(#28599,#28600,#28601,#28602));
#5234=EDGE_LOOP('',(#28603,#28604,#28605,#28606));
#5235=EDGE_LOOP('',(#28607,#28608,#28609,#28610));
#5236=EDGE_LOOP('',(#28611,#28612,#28613,#28614));
#5237=EDGE_LOOP('',(#28615,#28616,#28617,#28618));
#5238=EDGE_LOOP('',(#28619,#28620,#28621,#28622));
#5239=EDGE_LOOP('',(#28623,#28624,#28625));
#5240=EDGE_LOOP('',(#28626,#28627,#28628));
#5241=EDGE_LOOP('',(#28629,#28630,#28631,#28632));
#5242=EDGE_LOOP('',(#28633,#28634,#28635,#28636,#28637,#28638,#28639,#28640));
#5243=EDGE_LOOP('',(#28641,#28642,#28643,#28644));
#5244=EDGE_LOOP('',(#28645,#28646,#28647,#28648));
#5245=EDGE_LOOP('',(#28649,#28650,#28651));
#5246=EDGE_LOOP('',(#28652,#28653,#28654,#28655));
#5247=EDGE_LOOP('',(#28656,#28657,#28658));
#5248=EDGE_LOOP('',(#28659,#28660,#28661,#28662));
#5249=EDGE_LOOP('',(#28663,#28664,#28665,#28666));
#5250=EDGE_LOOP('',(#28667,#28668,#28669,#28670));
#5251=EDGE_LOOP('',(#28671,#28672,#28673,#28674));
#5252=EDGE_LOOP('',(#28675,#28676,#28677,#28678));
#5253=EDGE_LOOP('',(#28679,#28680,#28681,#28682));
#5254=EDGE_LOOP('',(#28683,#28684,#28685));
#5255=EDGE_LOOP('',(#28686,#28687,#28688,#28689));
#5256=EDGE_LOOP('',(#28690,#28691,#28692));
#5257=EDGE_LOOP('',(#28693,#28694,#28695,#28696));
#5258=EDGE_LOOP('',(#28697,#28698,#28699,#28700));
#5259=EDGE_LOOP('',(#28701,#28702,#28703,#28704));
#5260=EDGE_LOOP('',(#28705,#28706,#28707,#28708));
#5261=EDGE_LOOP('',(#28709,#28710,#28711,#28712));
#5262=EDGE_LOOP('',(#28713,#28714,#28715,#28716));
#5263=EDGE_LOOP('',(#28717,#28718,#28719));
#5264=EDGE_LOOP('',(#28720,#28721,#28722));
#5265=EDGE_LOOP('',(#28723,#28724,#28725,#28726,#28727,#28728,#28729,#28730));
#5266=EDGE_LOOP('',(#28731,#28732,#28733,#28734));
#5267=EDGE_LOOP('',(#28735,#28736,#28737,#28738));
#5268=EDGE_LOOP('',(#28739,#28740,#28741));
#5269=EDGE_LOOP('',(#28742,#28743,#28744,#28745));
#5270=EDGE_LOOP('',(#28746,#28747,#28748));
#5271=EDGE_LOOP('',(#28749,#28750,#28751,#28752));
#5272=EDGE_LOOP('',(#28753,#28754,#28755,#28756));
#5273=EDGE_LOOP('',(#28757,#28758,#28759,#28760));
#5274=EDGE_LOOP('',(#28761,#28762,#28763,#28764));
#5275=EDGE_LOOP('',(#28765,#28766,#28767));
#5276=EDGE_LOOP('',(#28768,#28769,#28770,#28771));
#5277=EDGE_LOOP('',(#28772,#28773,#28774));
#5278=EDGE_LOOP('',(#28775,#28776,#28777,#28778));
#5279=EDGE_LOOP('',(#28779,#28780,#28781,#28782));
#5280=EDGE_LOOP('',(#28783,#28784,#28785,#28786));
#5281=EDGE_LOOP('',(#28787,#28788,#28789,#28790));
#5282=EDGE_LOOP('',(#28791,#28792,#28793,#28794));
#5283=EDGE_LOOP('',(#28795,#28796,#28797,#28798));
#5284=EDGE_LOOP('',(#28799,#28800,#28801));
#5285=EDGE_LOOP('',(#28802,#28803,#28804));
#5286=EDGE_LOOP('',(#28805,#28806,#28807,#28808));
#5287=EDGE_LOOP('',(#28809,#28810,#28811,#28812));
#5288=EDGE_LOOP('',(#28813,#28814,#28815));
#5289=EDGE_LOOP('',(#28816,#28817,#28818,#28819));
#5290=EDGE_LOOP('',(#28820,#28821,#28822));
#5291=EDGE_LOOP('',(#28823,#28824,#28825,#28826));
#5292=EDGE_LOOP('',(#28827,#28828,#28829,#28830));
#5293=EDGE_LOOP('',(#28831,#28832,#28833,#28834));
#5294=EDGE_LOOP('',(#28835,#28836,#28837,#28838));
#5295=EDGE_LOOP('',(#28839,#28840,#28841));
#5296=EDGE_LOOP('',(#28842,#28843,#28844,#28845));
#5297=EDGE_LOOP('',(#28846,#28847,#28848));
#5298=EDGE_LOOP('',(#28849,#28850,#28851,#28852,#28853,#28854,#28855,#28856));
#5299=EDGE_LOOP('',(#28857,#28858,#28859,#28860));
#5300=EDGE_LOOP('',(#28861,#28862,#28863,#28864));
#5301=EDGE_LOOP('',(#28865,#28866,#28867));
#5302=EDGE_LOOP('',(#28868,#28869,#28870));
#5303=EDGE_LOOP('',(#28871,#28872,#28873,#28874,#28875,#28876,#28877,#28878));
#5304=EDGE_LOOP('',(#28879,#28880,#28881,#28882));
#5305=EDGE_LOOP('',(#28883,#28884,#28885,#28886));
#5306=EDGE_LOOP('',(#28887,#28888,#28889));
#5307=EDGE_LOOP('',(#28890,#28891,#28892,#28893));
#5308=EDGE_LOOP('',(#28894,#28895,#28896));
#5309=EDGE_LOOP('',(#28897,#28898,#28899,#28900,#28901,#28902,#28903,#28904));
#5310=EDGE_LOOP('',(#28905,#28906,#28907,#28908));
#5311=EDGE_LOOP('',(#28909,#28910,#28911,#28912,#28913,#28914,#28915,#28916));
#5312=EDGE_LOOP('',(#28917,#28918,#28919,#28920));
#5313=EDGE_LOOP('',(#28921,#28922,#28923,#28924));
#5314=EDGE_LOOP('',(#28925,#28926,#28927));
#5315=EDGE_LOOP('',(#28928,#28929,#28930));
#5316=EDGE_LOOP('',(#28931,#28932,#28933,#28934,#28935,#28936,#28937,#28938));
#5317=EDGE_LOOP('',(#28939,#28940,#28941,#28942));
#5318=EDGE_LOOP('',(#28943,#28944,#28945,#28946));
#5319=EDGE_LOOP('',(#28947,#28948,#28949));
#5320=EDGE_LOOP('',(#28950,#28951,#28952));
#5321=EDGE_LOOP('',(#28953,#28954,#28955,#28956,#28957,#28958,#28959,#28960));
#5322=EDGE_LOOP('',(#28961,#28962,#28963,#28964));
#5323=EDGE_LOOP('',(#28965,#28966,#28967,#28968));
#5324=EDGE_LOOP('',(#28969,#28970,#28971));
#5325=EDGE_LOOP('',(#28972,#28973,#28974,#28975));
#5326=EDGE_LOOP('',(#28976,#28977,#28978));
#5327=EDGE_LOOP('',(#28979,#28980,#28981,#28982));
#5328=EDGE_LOOP('',(#28983,#28984,#28985,#28986));
#5329=EDGE_LOOP('',(#28987,#28988,#28989,#28990));
#5330=EDGE_LOOP('',(#28991,#28992,#28993,#28994));
#5331=EDGE_LOOP('',(#28995,#28996,#28997,#28998));
#5332=EDGE_LOOP('',(#28999,#29000,#29001,#29002));
#5333=EDGE_LOOP('',(#29003,#29004,#29005));
#5334=EDGE_LOOP('',(#29006,#29007,#29008));
#5335=EDGE_LOOP('',(#29009,#29010,#29011,#29012,#29013,#29014,#29015,#29016));
#5336=EDGE_LOOP('',(#29017,#29018,#29019,#29020));
#5337=EDGE_LOOP('',(#29021,#29022,#29023,#29024,#29025,#29026,#29027,#29028));
#5338=EDGE_LOOP('',(#29029,#29030,#29031,#29032));
#5339=EDGE_LOOP('',(#29033,#29034,#29035,#29036,#29037,#29038,#29039,#29040));
#5340=EDGE_LOOP('',(#29041,#29042,#29043,#29044));
#5341=EDGE_LOOP('',(#29045,#29046,#29047,#29048));
#5342=EDGE_LOOP('',(#29049,#29050,#29051));
#5343=EDGE_LOOP('',(#29052,#29053,#29054,#29055));
#5344=EDGE_LOOP('',(#29056,#29057,#29058));
#5345=EDGE_LOOP('',(#29059,#29060,#29061,#29062));
#5346=EDGE_LOOP('',(#29063,#29064,#29065,#29066));
#5347=EDGE_LOOP('',(#29067,#29068,#29069,#29070));
#5348=EDGE_LOOP('',(#29071,#29072,#29073,#29074));
#5349=EDGE_LOOP('',(#29075,#29076,#29077,#29078));
#5350=EDGE_LOOP('',(#29079,#29080,#29081,#29082));
#5351=EDGE_LOOP('',(#29083,#29084,#29085));
#5352=EDGE_LOOP('',(#29086,#29087,#29088,#29089));
#5353=EDGE_LOOP('',(#29090,#29091,#29092));
#5354=EDGE_LOOP('',(#29093,#29094,#29095,#29096));
#5355=EDGE_LOOP('',(#29097,#29098,#29099,#29100));
#5356=EDGE_LOOP('',(#29101,#29102,#29103,#29104));
#5357=EDGE_LOOP('',(#29105,#29106,#29107,#29108));
#5358=EDGE_LOOP('',(#29109,#29110,#29111));
#5359=EDGE_LOOP('',(#29112,#29113,#29114,#29115));
#5360=EDGE_LOOP('',(#29116,#29117,#29118));
#5361=EDGE_LOOP('',(#29119,#29120,#29121,#29122));
#5362=EDGE_LOOP('',(#29123,#29124,#29125,#29126));
#5363=EDGE_LOOP('',(#29127,#29128,#29129,#29130));
#5364=EDGE_LOOP('',(#29131,#29132,#29133,#29134));
#5365=EDGE_LOOP('',(#29135,#29136,#29137,#29138));
#5366=EDGE_LOOP('',(#29139,#29140,#29141,#29142));
#5367=EDGE_LOOP('',(#29143,#29144,#29145));
#5368=EDGE_LOOP('',(#29146,#29147,#29148,#29149));
#5369=EDGE_LOOP('',(#29150,#29151,#29152));
#5370=EDGE_LOOP('',(#29153,#29154,#29155,#29156));
#5371=EDGE_LOOP('',(#29157,#29158,#29159,#29160));
#5372=EDGE_LOOP('',(#29161,#29162,#29163,#29164));
#5373=EDGE_LOOP('',(#29165,#29166,#29167,#29168));
#5374=EDGE_LOOP('',(#29169,#29170,#29171,#29172));
#5375=EDGE_LOOP('',(#29173,#29174,#29175,#29176));
#5376=EDGE_LOOP('',(#29177,#29178,#29179));
#5377=EDGE_LOOP('',(#29180,#29181,#29182,#29183));
#5378=EDGE_LOOP('',(#29184,#29185,#29186));
#5379=EDGE_LOOP('',(#29187,#29188,#29189,#29190));
#5380=EDGE_LOOP('',(#29191,#29192,#29193,#29194));
#5381=EDGE_LOOP('',(#29195,#29196,#29197,#29198));
#5382=EDGE_LOOP('',(#29199,#29200,#29201,#29202));
#5383=EDGE_LOOP('',(#29203,#29204,#29205));
#5384=EDGE_LOOP('',(#29206,#29207,#29208,#29209));
#5385=EDGE_LOOP('',(#29210,#29211,#29212));
#5386=EDGE_LOOP('',(#29213,#29214,#29215,#29216,#29217,#29218,#29219,#29220));
#5387=EDGE_LOOP('',(#29221,#29222,#29223,#29224));
#5388=EDGE_LOOP('',(#29225,#29226,#29227,#29228));
#5389=EDGE_LOOP('',(#29229,#29230,#29231));
#5390=EDGE_LOOP('',(#29232,#29233,#29234));
#5391=EDGE_LOOP('',(#29235,#29236,#29237,#29238,#29239,#29240,#29241,#29242));
#5392=EDGE_LOOP('',(#29243,#29244,#29245,#29246));
#5393=EDGE_LOOP('',(#29247,#29248,#29249,#29250));
#5394=EDGE_LOOP('',(#29251,#29252,#29253));
#5395=EDGE_LOOP('',(#29254,#29255,#29256));
#5396=EDGE_LOOP('',(#29257,#29258,#29259,#29260,#29261,#29262,#29263,#29264));
#5397=EDGE_LOOP('',(#29265,#29266,#29267,#29268));
#5398=EDGE_LOOP('',(#29269,#29270,#29271,#29272));
#5399=EDGE_LOOP('',(#29273,#29274,#29275));
#5400=EDGE_LOOP('',(#29276,#29277,#29278,#29279));
#5401=EDGE_LOOP('',(#29280,#29281,#29282));
#5402=EDGE_LOOP('',(#29283,#29284,#29285,#29286,#29287,#29288,#29289,#29290));
#5403=EDGE_LOOP('',(#29291,#29292,#29293,#29294));
#5404=EDGE_LOOP('',(#29295,#29296,#29297,#29298,#29299,#29300));
#5405=EDGE_LOOP('',(#29301,#29302,#29303,#29304,#29305,#29306,#29307,#29308,
#29309,#29310));
#5406=EDGE_LOOP('',(#29311,#29312,#29313,#29314));
#5407=EDGE_LOOP('',(#29315,#29316,#29317,#29318));
#5408=EDGE_LOOP('',(#29319,#29320,#29321));
#5409=EDGE_LOOP('',(#29322,#29323,#29324));
#5410=EDGE_LOOP('',(#29325,#29326,#29327,#29328,#29329,#29330,#29331,#29332));
#5411=EDGE_LOOP('',(#29333,#29334,#29335,#29336));
#5412=EDGE_LOOP('',(#29337,#29338,#29339,#29340));
#5413=EDGE_LOOP('',(#29341,#29342,#29343));
#5414=EDGE_LOOP('',(#29344,#29345,#29346,#29347));
#5415=EDGE_LOOP('',(#29348,#29349,#29350));
#5416=EDGE_LOOP('',(#29351,#29352,#29353,#29354));
#5417=EDGE_LOOP('',(#29355,#29356,#29357,#29358));
#5418=EDGE_LOOP('',(#29359,#29360,#29361,#29362));
#5419=EDGE_LOOP('',(#29363,#29364,#29365,#29366));
#5420=EDGE_LOOP('',(#29367,#29368,#29369));
#5421=EDGE_LOOP('',(#29370,#29371,#29372));
#5422=EDGE_LOOP('',(#29373,#29374,#29375,#29376));
#5423=EDGE_LOOP('',(#29377,#29378,#29379,#29380));
#5424=EDGE_LOOP('',(#29381,#29382,#29383));
#5425=EDGE_LOOP('',(#29384,#29385,#29386,#29387));
#5426=EDGE_LOOP('',(#29388,#29389,#29390));
#5427=EDGE_LOOP('',(#29391,#29392,#29393,#29394,#29395,#29396,#29397,#29398));
#5428=EDGE_LOOP('',(#29399,#29400,#29401,#29402));
#5429=EDGE_LOOP('',(#29403,#29404,#29405,#29406,#29407,#29408,#29409,#29410));
#5430=EDGE_LOOP('',(#29411,#29412,#29413,#29414));
#5431=EDGE_LOOP('',(#29415,#29416,#29417,#29418));
#5432=EDGE_LOOP('',(#29419,#29420,#29421));
#5433=EDGE_LOOP('',(#29422,#29423,#29424,#29425));
#5434=EDGE_LOOP('',(#29426,#29427,#29428,#29429,#29430,#29431));
#5435=EDGE_LOOP('',(#29432,#29433,#29434,#29435));
#5436=EDGE_LOOP('',(#29436,#29437,#29438,#29439));
#5437=EDGE_LOOP('',(#29440,#29441,#29442,#29443));
#5438=EDGE_LOOP('',(#29444,#29445,#29446,#29447,#29448,#29449,#29450,#29451));
#5439=EDGE_LOOP('',(#29452,#29453,#29454,#29455));
#5440=EDGE_LOOP('',(#29456,#29457,#29458,#29459,#29460,#29461,#29462,#29463));
#5441=EDGE_LOOP('',(#29464,#29465,#29466,#29467));
#5442=EDGE_LOOP('',(#29468,#29469,#29470,#29471));
#5443=EDGE_LOOP('',(#29472,#29473,#29474,#29475));
#5444=EDGE_LOOP('',(#29476,#29477,#29478,#29479));
#5445=EDGE_LOOP('',(#29480,#29481,#29482,#29483));
#5446=EDGE_LOOP('',(#29484,#29485,#29486,#29487));
#5447=EDGE_LOOP('',(#29488,#29489,#29490,#29491,#29492,#29493,#29494,#29495));
#5448=EDGE_LOOP('',(#29496,#29497,#29498,#29499));
#5449=EDGE_LOOP('',(#29500,#29501,#29502,#29503));
#5450=EDGE_LOOP('',(#29504,#29505,#29506,#29507));
#5451=EDGE_LOOP('',(#29508,#29509,#29510,#29511));
#5452=EDGE_LOOP('',(#29512,#29513,#29514,#29515,#29516,#29517,#29518,#29519));
#5453=EDGE_LOOP('',(#29520,#29521,#29522,#29523));
#5454=EDGE_LOOP('',(#29524,#29525,#29526,#29527));
#5455=EDGE_LOOP('',(#29528,#29529,#29530,#29531));
#5456=EDGE_LOOP('',(#29532,#29533,#29534,#29535,#29536,#29537,#29538,#29539));
#5457=EDGE_LOOP('',(#29540,#29541,#29542,#29543));
#5458=EDGE_LOOP('',(#29544,#29545,#29546,#29547));
#5459=EDGE_LOOP('',(#29548,#29549,#29550,#29551));
#5460=EDGE_LOOP('',(#29552,#29553,#29554,#29555));
#5461=EDGE_LOOP('',(#29556,#29557,#29558,#29559));
#5462=EDGE_LOOP('',(#29560,#29561,#29562,#29563,#29564,#29565,#29566,#29567));
#5463=EDGE_LOOP('',(#29568,#29569,#29570,#29571));
#5464=EDGE_LOOP('',(#29572,#29573,#29574));
#5465=EDGE_LOOP('',(#29575,#29576,#29577,#29578));
#5466=EDGE_LOOP('',(#29579,#29580,#29581));
#5467=EDGE_LOOP('',(#29582,#29583,#29584,#29585));
#5468=EDGE_LOOP('',(#29586,#29587,#29588,#29589));
#5469=EDGE_LOOP('',(#29590,#29591,#29592,#29593,#29594,#29595));
#5470=EDGE_LOOP('',(#29596,#29597,#29598,#29599));
#5471=EDGE_LOOP('',(#29600,#29601,#29602,#29603));
#5472=EDGE_LOOP('',(#29604,#29605,#29606,#29607));
#5473=EDGE_LOOP('',(#29608,#29609,#29610,#29611));
#5474=EDGE_LOOP('',(#29612,#29613,#29614,#29615));
#5475=EDGE_LOOP('',(#29616,#29617,#29618,#29619));
#5476=EDGE_LOOP('',(#29620,#29621,#29622,#29623,#29624,#29625,#29626,#29627));
#5477=EDGE_LOOP('',(#29628,#29629,#29630,#29631));
#5478=EDGE_LOOP('',(#29632,#29633,#29634,#29635,#29636,#29637,#29638,#29639));
#5479=EDGE_LOOP('',(#29640,#29641,#29642,#29643));
#5480=EDGE_LOOP('',(#29644,#29645,#29646,#29647));
#5481=EDGE_LOOP('',(#29648,#29649,#29650,#29651));
#5482=EDGE_LOOP('',(#29652,#29653,#29654,#29655));
#5483=EDGE_LOOP('',(#29656,#29657,#29658,#29659));
#5484=EDGE_LOOP('',(#29660,#29661,#29662,#29663));
#5485=EDGE_LOOP('',(#29664,#29665,#29666,#29667,#29668,#29669,#29670,#29671));
#5486=EDGE_LOOP('',(#29672,#29673,#29674,#29675));
#5487=EDGE_LOOP('',(#29676,#29677,#29678,#29679));
#5488=EDGE_LOOP('',(#29680,#29681,#29682,#29683));
#5489=EDGE_LOOP('',(#29684,#29685,#29686,#29687));
#5490=EDGE_LOOP('',(#29688,#29689,#29690,#29691,#29692,#29693,#29694,#29695));
#5491=EDGE_LOOP('',(#29696,#29697,#29698,#29699));
#5492=EDGE_LOOP('',(#29700,#29701,#29702,#29703));
#5493=EDGE_LOOP('',(#29704,#29705,#29706,#29707));
#5494=EDGE_LOOP('',(#29708,#29709,#29710,#29711,#29712,#29713,#29714,#29715));
#5495=EDGE_LOOP('',(#29716,#29717,#29718,#29719));
#5496=EDGE_LOOP('',(#29720,#29721,#29722,#29723));
#5497=EDGE_LOOP('',(#29724,#29725,#29726,#29727));
#5498=EDGE_LOOP('',(#29728,#29729,#29730,#29731));
#5499=EDGE_LOOP('',(#29732,#29733,#29734,#29735));
#5500=EDGE_LOOP('',(#29736,#29737,#29738,#29739,#29740,#29741,#29742,#29743));
#5501=EDGE_LOOP('',(#29744,#29745,#29746,#29747));
#5502=EDGE_LOOP('',(#29748,#29749,#29750));
#5503=EDGE_LOOP('',(#29751,#29752,#29753,#29754));
#5504=EDGE_LOOP('',(#29755,#29756,#29757));
#5505=EDGE_LOOP('',(#29758,#29759,#29760,#29761));
#5506=EDGE_LOOP('',(#29762,#29763,#29764,#29765));
#5507=EDGE_LOOP('',(#29766,#29767,#29768,#29769,#29770,#29771));
#5508=EDGE_LOOP('',(#29772,#29773,#29774,#29775));
#5509=EDGE_LOOP('',(#29776,#29777,#29778,#29779));
#5510=EDGE_LOOP('',(#29780,#29781,#29782,#29783));
#5511=EDGE_LOOP('',(#29784,#29785,#29786,#29787));
#5512=EDGE_LOOP('',(#29788,#29789,#29790,#29791));
#5513=EDGE_LOOP('',(#29792,#29793,#29794,#29795));
#5514=EDGE_LOOP('',(#29796,#29797,#29798,#29799,#29800,#29801,#29802,#29803));
#5515=EDGE_LOOP('',(#29804,#29805,#29806,#29807));
#5516=EDGE_LOOP('',(#29808,#29809,#29810,#29811,#29812,#29813,#29814,#29815));
#5517=EDGE_LOOP('',(#29816,#29817,#29818,#29819));
#5518=EDGE_LOOP('',(#29820,#29821,#29822,#29823));
#5519=EDGE_LOOP('',(#29824,#29825,#29826,#29827));
#5520=EDGE_LOOP('',(#29828,#29829,#29830,#29831));
#5521=EDGE_LOOP('',(#29832,#29833,#29834,#29835));
#5522=EDGE_LOOP('',(#29836,#29837,#29838,#29839));
#5523=EDGE_LOOP('',(#29840,#29841,#29842,#29843,#29844,#29845,#29846,#29847));
#5524=EDGE_LOOP('',(#29848,#29849,#29850,#29851));
#5525=EDGE_LOOP('',(#29852,#29853,#29854,#29855));
#5526=EDGE_LOOP('',(#29856,#29857,#29858,#29859));
#5527=EDGE_LOOP('',(#29860,#29861,#29862,#29863));
#5528=EDGE_LOOP('',(#29864,#29865,#29866,#29867,#29868,#29869,#29870,#29871));
#5529=EDGE_LOOP('',(#29872,#29873,#29874,#29875));
#5530=EDGE_LOOP('',(#29876,#29877,#29878,#29879));
#5531=EDGE_LOOP('',(#29880,#29881,#29882,#29883));
#5532=EDGE_LOOP('',(#29884,#29885,#29886,#29887,#29888,#29889,#29890,#29891));
#5533=EDGE_LOOP('',(#29892,#29893,#29894,#29895));
#5534=EDGE_LOOP('',(#29896,#29897,#29898,#29899));
#5535=EDGE_LOOP('',(#29900,#29901,#29902,#29903));
#5536=EDGE_LOOP('',(#29904,#29905,#29906,#29907));
#5537=EDGE_LOOP('',(#29908,#29909,#29910,#29911));
#5538=EDGE_LOOP('',(#29912,#29913,#29914,#29915,#29916,#29917,#29918,#29919));
#5539=EDGE_LOOP('',(#29920,#29921,#29922,#29923));
#5540=EDGE_LOOP('',(#29924,#29925,#29926));
#5541=EDGE_LOOP('',(#29927,#29928,#29929,#29930));
#5542=EDGE_LOOP('',(#29931,#29932,#29933));
#5543=EDGE_LOOP('',(#29934,#29935,#29936,#29937));
#5544=EDGE_LOOP('',(#29938,#29939,#29940,#29941));
#5545=EDGE_LOOP('',(#29942,#29943,#29944,#29945,#29946,#29947));
#5546=EDGE_LOOP('',(#29948,#29949,#29950,#29951));
#5547=EDGE_LOOP('',(#29952,#29953,#29954,#29955));
#5548=EDGE_LOOP('',(#29956,#29957,#29958,#29959));
#5549=EDGE_LOOP('',(#29960,#29961,#29962,#29963));
#5550=EDGE_LOOP('',(#29964,#29965,#29966,#29967));
#5551=EDGE_LOOP('',(#29968,#29969,#29970,#29971,#29972,#29973,#29974,#29975));
#5552=EDGE_LOOP('',(#29976,#29977,#29978,#29979));
#5553=EDGE_LOOP('',(#29980,#29981,#29982,#29983));
#5554=EDGE_LOOP('',(#29984,#29985,#29986));
#5555=EDGE_LOOP('',(#29987,#29988,#29989,#29990));
#5556=EDGE_LOOP('',(#29991,#29992,#29993,#29994));
#5557=EDGE_LOOP('',(#29995,#29996,#29997));
#5558=EDGE_LOOP('',(#29998,#29999,#30000,#30001,#30002,#30003,#30004,#30005));
#5559=EDGE_LOOP('',(#30006,#30007,#30008,#30009,#30010,#30011,#30012,#30013));
#5560=EDGE_LOOP('',(#30014,#30015,#30016,#30017));
#5561=EDGE_LOOP('',(#30018,#30019,#30020,#30021));
#5562=EDGE_LOOP('',(#30022,#30023,#30024,#30025));
#5563=EDGE_LOOP('',(#30026,#30027,#30028,#30029));
#5564=EDGE_LOOP('',(#30030,#30031,#30032,#30033));
#5565=EDGE_LOOP('',(#30034,#30035,#30036,#30037));
#5566=EDGE_LOOP('',(#30038,#30039,#30040,#30041,#30042,#30043,#30044,#30045));
#5567=EDGE_LOOP('',(#30046,#30047,#30048,#30049));
#5568=EDGE_LOOP('',(#30050,#30051,#30052,#30053));
#5569=EDGE_LOOP('',(#30054,#30055,#30056,#30057,#30058,#30059,#30060,#30061));
#5570=EDGE_LOOP('',(#30062,#30063,#30064,#30065));
#5571=EDGE_LOOP('',(#30066,#30067,#30068,#30069));
#5572=EDGE_LOOP('',(#30070,#30071,#30072,#30073));
#5573=EDGE_LOOP('',(#30074,#30075,#30076,#30077));
#5574=EDGE_LOOP('',(#30078,#30079,#30080,#30081));
#5575=EDGE_LOOP('',(#30082,#30083,#30084,#30085,#30086,#30087,#30088,#30089));
#5576=EDGE_LOOP('',(#30090,#30091,#30092,#30093));
#5577=EDGE_LOOP('',(#30094,#30095,#30096,#30097));
#5578=EDGE_LOOP('',(#30098,#30099,#30100));
#5579=EDGE_LOOP('',(#30101,#30102,#30103,#30104,#30105));
#5580=EDGE_LOOP('',(#30106,#30107,#30108,#30109));
#5581=EDGE_LOOP('',(#30110,#30111,#30112));
#5582=EDGE_LOOP('',(#30113,#30114,#30115));
#5583=EDGE_LOOP('',(#30116,#30117,#30118,#30119));
#5584=EDGE_LOOP('',(#30120,#30121,#30122,#30123));
#5585=EDGE_LOOP('',(#30124,#30125,#30126,#30127));
#5586=EDGE_LOOP('',(#30128,#30129,#30130,#30131));
#5587=EDGE_LOOP('',(#30132,#30133,#30134,#30135));
#5588=EDGE_LOOP('',(#30136,#30137,#30138,#30139));
#5589=EDGE_LOOP('',(#30140,#30141,#30142,#30143));
#5590=EDGE_LOOP('',(#30144,#30145,#30146,#30147));
#5591=EDGE_LOOP('',(#30148,#30149,#30150));
#5592=EDGE_LOOP('',(#30151,#30152,#30153,#30154));
#5593=EDGE_LOOP('',(#30155,#30156,#30157,#30158,#30159));
#5594=EDGE_LOOP('',(#30160,#30161,#30162));
#5595=EDGE_LOOP('',(#30163,#30164,#30165,#30166));
#5596=EDGE_LOOP('',(#30167,#30168,#30169));
#5597=EDGE_LOOP('',(#30170,#30171,#30172));
#5598=EDGE_LOOP('',(#30173,#30174,#30175,#30176));
#5599=EDGE_LOOP('',(#30177,#30178,#30179,#30180));
#5600=EDGE_LOOP('',(#30181,#30182,#30183,#30184,#30185,#30186,#30187));
#5601=EDGE_LOOP('',(#30188,#30189,#30190,#30191));
#5602=EDGE_LOOP('',(#30192,#30193,#30194,#30195,#30196));
#5603=EDGE_LOOP('',(#30197,#30198,#30199,#30200));
#5604=EDGE_LOOP('',(#30201,#30202,#30203,#30204,#30205));
#5605=EDGE_LOOP('',(#30206,#30207,#30208,#30209));
#5606=EDGE_LOOP('',(#30210,#30211,#30212));
#5607=EDGE_LOOP('',(#30213,#30214,#30215,#30216));
#5608=EDGE_LOOP('',(#30217,#30218,#30219,#30220,#30221,#30222,#30223,#30224));
#5609=EDGE_LOOP('',(#30225,#30226,#30227,#30228));
#5610=EDGE_LOOP('',(#30229,#30230,#30231,#30232));
#5611=EDGE_LOOP('',(#30233,#30234,#30235));
#5612=EDGE_LOOP('',(#30236,#30237,#30238));
#5613=EDGE_LOOP('',(#30239,#30240,#30241,#30242,#30243));
#5614=EDGE_LOOP('',(#30244,#30245,#30246,#30247,#30248,#30249));
#5615=EDGE_LOOP('',(#30250,#30251,#30252,#30253));
#5616=EDGE_LOOP('',(#30254,#30255,#30256,#30257,#30258));
#5617=EDGE_LOOP('',(#30259,#30260,#30261,#30262));
#5618=EDGE_LOOP('',(#30263,#30264,#30265));
#5619=EDGE_LOOP('',(#30266,#30267,#30268,#30269));
#5620=EDGE_LOOP('',(#30270,#30271,#30272,#30273,#30274));
#5621=EDGE_LOOP('',(#30275,#30276,#30277,#30278));
#5622=EDGE_LOOP('',(#30279,#30280,#30281));
#5623=EDGE_LOOP('',(#30282,#30283,#30284,#30285));
#5624=EDGE_LOOP('',(#30286,#30287,#30288,#30289));
#5625=EDGE_LOOP('',(#30290,#30291,#30292,#30293));
#5626=EDGE_LOOP('',(#30294,#30295,#30296,#30297));
#5627=EDGE_LOOP('',(#30298,#30299,#30300,#30301));
#5628=EDGE_LOOP('',(#30302,#30303,#30304,#30305));
#5629=EDGE_LOOP('',(#30306,#30307,#30308,#30309,#30310));
#5630=EDGE_LOOP('',(#30311,#30312,#30313,#30314));
#5631=EDGE_LOOP('',(#30315,#30316,#30317,#30318));
#5632=EDGE_LOOP('',(#30319,#30320,#30321,#30322));
#5633=EDGE_LOOP('',(#30323,#30324,#30325,#30326));
#5634=EDGE_LOOP('',(#30327,#30328,#30329,#30330));
#5635=EDGE_LOOP('',(#30331,#30332,#30333,#30334));
#5636=EDGE_LOOP('',(#30335,#30336,#30337,#30338));
#5637=EDGE_LOOP('',(#30339,#30340,#30341,#30342));
#5638=EDGE_LOOP('',(#30343,#30344,#30345,#30346));
#5639=EDGE_LOOP('',(#30347,#30348,#30349,#30350));
#5640=EDGE_LOOP('',(#30351,#30352,#30353,#30354));
#5641=EDGE_LOOP('',(#30355,#30356,#30357,#30358));
#5642=EDGE_LOOP('',(#30359,#30360,#30361,#30362,#30363,#30364,#30365,#30366));
#5643=EDGE_LOOP('',(#30367,#30368,#30369,#30370));
#5644=EDGE_LOOP('',(#30371,#30372,#30373,#30374));
#5645=EDGE_LOOP('',(#30375,#30376,#30377,#30378));
#5646=EDGE_LOOP('',(#30379,#30380,#30381,#30382));
#5647=EDGE_LOOP('',(#30383,#30384,#30385,#30386));
#5648=EDGE_LOOP('',(#30387,#30388,#30389,#30390));
#5649=EDGE_LOOP('',(#30391,#30392,#30393,#30394));
#5650=EDGE_LOOP('',(#30395,#30396,#30397,#30398));
#5651=EDGE_LOOP('',(#30399,#30400,#30401,#30402));
#5652=EDGE_LOOP('',(#30403,#30404,#30405,#30406));
#5653=EDGE_LOOP('',(#30407,#30408,#30409,#30410));
#5654=EDGE_LOOP('',(#30411,#30412,#30413,#30414));
#5655=EDGE_LOOP('',(#30415,#30416,#30417,#30418));
#5656=EDGE_LOOP('',(#30419,#30420,#30421,#30422));
#5657=EDGE_LOOP('',(#30423,#30424,#30425,#30426));
#5658=EDGE_LOOP('',(#30427,#30428,#30429,#30430));
#5659=EDGE_LOOP('',(#30431,#30432,#30433,#30434));
#5660=EDGE_LOOP('',(#30435,#30436,#30437,#30438));
#5661=EDGE_LOOP('',(#30439,#30440,#30441,#30442));
#5662=EDGE_LOOP('',(#30443,#30444,#30445,#30446));
#5663=EDGE_LOOP('',(#30447,#30448,#30449,#30450));
#5664=EDGE_LOOP('',(#30451,#30452,#30453,#30454));
#5665=EDGE_LOOP('',(#30455,#30456,#30457,#30458));
#5666=EDGE_LOOP('',(#30459,#30460,#30461,#30462));
#5667=EDGE_LOOP('',(#30463,#30464,#30465,#30466));
#5668=EDGE_LOOP('',(#30467,#30468,#30469,#30470));
#5669=EDGE_LOOP('',(#30471,#30472,#30473,#30474));
#5670=EDGE_LOOP('',(#30475,#30476,#30477,#30478));
#5671=EDGE_LOOP('',(#30479,#30480,#30481,#30482));
#5672=EDGE_LOOP('',(#30483,#30484,#30485,#30486));
#5673=EDGE_LOOP('',(#30487,#30488,#30489,#30490));
#5674=EDGE_LOOP('',(#30491,#30492,#30493,#30494));
#5675=EDGE_LOOP('',(#30495,#30496,#30497,#30498));
#5676=EDGE_LOOP('',(#30499,#30500,#30501,#30502));
#5677=EDGE_LOOP('',(#30503,#30504,#30505,#30506));
#5678=EDGE_LOOP('',(#30507,#30508,#30509,#30510));
#5679=EDGE_LOOP('',(#30511,#30512,#30513,#30514));
#5680=EDGE_LOOP('',(#30515,#30516,#30517,#30518));
#5681=EDGE_LOOP('',(#30519,#30520,#30521,#30522));
#5682=EDGE_LOOP('',(#30523,#30524,#30525,#30526));
#5683=EDGE_LOOP('',(#30527,#30528,#30529,#30530));
#5684=EDGE_LOOP('',(#30531,#30532,#30533,#30534));
#5685=EDGE_LOOP('',(#30535,#30536,#30537,#30538,#30539,#30540,#30541,#30542));
#5686=EDGE_LOOP('',(#30543,#30544,#30545,#30546));
#5687=EDGE_LOOP('',(#30547,#30548,#30549,#30550));
#5688=EDGE_LOOP('',(#30551,#30552,#30553,#30554));
#5689=EDGE_LOOP('',(#30555,#30556,#30557,#30558));
#5690=EDGE_LOOP('',(#30559,#30560,#30561,#30562));
#5691=EDGE_LOOP('',(#30563,#30564,#30565,#30566));
#5692=EDGE_LOOP('',(#30567,#30568,#30569,#30570));
#5693=EDGE_LOOP('',(#30571,#30572,#30573,#30574));
#5694=EDGE_LOOP('',(#30575,#30576,#30577,#30578));
#5695=EDGE_LOOP('',(#30579,#30580,#30581,#30582));
#5696=EDGE_LOOP('',(#30583,#30584,#30585,#30586));
#5697=EDGE_LOOP('',(#30587,#30588,#30589,#30590));
#5698=EDGE_LOOP('',(#30591,#30592,#30593,#30594));
#5699=EDGE_LOOP('',(#30595,#30596,#30597,#30598));
#5700=EDGE_LOOP('',(#30599,#30600,#30601,#30602));
#5701=EDGE_LOOP('',(#30603,#30604,#30605,#30606,#30607,#30608,#30609,#30610));
#5702=EDGE_LOOP('',(#30611,#30612,#30613,#30614));
#5703=EDGE_LOOP('',(#30615,#30616,#30617,#30618));
#5704=EDGE_LOOP('',(#30619,#30620,#30621,#30622));
#5705=EDGE_LOOP('',(#30623,#30624,#30625,#30626));
#5706=EDGE_LOOP('',(#30627,#30628,#30629,#30630));
#5707=EDGE_LOOP('',(#30631,#30632,#30633,#30634));
#5708=EDGE_LOOP('',(#30635,#30636,#30637,#30638,#30639,#30640,#30641,#30642));
#5709=EDGE_LOOP('',(#30643,#30644,#30645,#30646));
#5710=EDGE_LOOP('',(#30647,#30648,#30649,#30650));
#5711=EDGE_LOOP('',(#30651,#30652,#30653,#30654));
#5712=EDGE_LOOP('',(#30655,#30656,#30657,#30658));
#5713=EDGE_LOOP('',(#30659,#30660,#30661,#30662));
#5714=EDGE_LOOP('',(#30663,#30664,#30665,#30666));
#5715=EDGE_LOOP('',(#30667,#30668,#30669,#30670));
#5716=EDGE_LOOP('',(#30671,#30672,#30673,#30674));
#5717=EDGE_LOOP('',(#30675,#30676,#30677,#30678));
#5718=EDGE_LOOP('',(#30679,#30680,#30681,#30682));
#5719=EDGE_LOOP('',(#30683,#30684,#30685,#30686));
#5720=EDGE_LOOP('',(#30687,#30688,#30689,#30690));
#5721=EDGE_LOOP('',(#30691,#30692,#30693,#30694));
#5722=EDGE_LOOP('',(#30695,#30696,#30697,#30698));
#5723=EDGE_LOOP('',(#30699,#30700,#30701,#30702));
#5724=EDGE_LOOP('',(#30703,#30704,#30705,#30706));
#5725=EDGE_LOOP('',(#30707,#30708,#30709,#30710));
#5726=EDGE_LOOP('',(#30711,#30712,#30713,#30714));
#5727=EDGE_LOOP('',(#30715,#30716,#30717,#30718));
#5728=EDGE_LOOP('',(#30719,#30720,#30721,#30722));
#5729=EDGE_LOOP('',(#30723,#30724,#30725,#30726));
#5730=EDGE_LOOP('',(#30727,#30728,#30729,#30730));
#5731=EDGE_LOOP('',(#30731,#30732,#30733,#30734,#30735,#30736,#30737,#30738));
#5732=EDGE_LOOP('',(#30739,#30740,#30741,#30742));
#5733=EDGE_LOOP('',(#30743,#30744,#30745,#30746));
#5734=EDGE_LOOP('',(#30747,#30748,#30749,#30750));
#5735=EDGE_LOOP('',(#30751,#30752,#30753,#30754));
#5736=EDGE_LOOP('',(#30755,#30756,#30757,#30758));
#5737=EDGE_LOOP('',(#30759,#30760,#30761,#30762));
#5738=EDGE_LOOP('',(#30763,#30764,#30765,#30766));
#5739=EDGE_LOOP('',(#30767,#30768,#30769,#30770));
#5740=EDGE_LOOP('',(#30771,#30772,#30773,#30774));
#5741=EDGE_LOOP('',(#30775,#30776,#30777,#30778));
#5742=EDGE_LOOP('',(#30779,#30780,#30781,#30782));
#5743=EDGE_LOOP('',(#30783,#30784,#30785,#30786));
#5744=EDGE_LOOP('',(#30787,#30788,#30789,#30790));
#5745=EDGE_LOOP('',(#30791,#30792,#30793,#30794));
#5746=EDGE_LOOP('',(#30795,#30796,#30797,#30798,#30799,#30800,#30801,#30802,
#30803,#30804));
#5747=EDGE_LOOP('',(#30805,#30806,#30807,#30808));
#5748=EDGE_LOOP('',(#30809,#30810,#30811,#30812));
#5749=EDGE_LOOP('',(#30813,#30814,#30815,#30816));
#5750=EDGE_LOOP('',(#30817,#30818,#30819,#30820));
#5751=EDGE_LOOP('',(#30821,#30822,#30823,#30824,#30825,#30826));
#5752=EDGE_LOOP('',(#30827,#30828,#30829,#30830));
#5753=EDGE_LOOP('',(#30831,#30832,#30833,#30834,#30835,#30836));
#5754=EDGE_LOOP('',(#30837,#30838,#30839,#30840));
#5755=EDGE_LOOP('',(#30841,#30842,#30843,#30844,#30845,#30846));
#5756=EDGE_LOOP('',(#30847,#30848,#30849,#30850,#30851,#30852));
#5757=EDGE_LOOP('',(#30853,#30854,#30855,#30856,#30857,#30858));
#5758=EDGE_LOOP('',(#30859,#30860,#30861,#30862));
#5759=EDGE_LOOP('',(#30863,#30864,#30865,#30866,#30867));
#5760=EDGE_LOOP('',(#30868,#30869,#30870,#30871,#30872,#30873));
#5761=EDGE_LOOP('',(#30874,#30875,#30876,#30877,#30878,#30879));
#5762=EDGE_LOOP('',(#30880,#30881,#30882,#30883));
#5763=EDGE_LOOP('',(#30884,#30885,#30886,#30887,#30888,#30889));
#5764=EDGE_LOOP('',(#30890,#30891,#30892,#30893,#30894,#30895));
#5765=EDGE_LOOP('',(#30896,#30897,#30898,#30899,#30900));
#5766=EDGE_LOOP('',(#30901,#30902,#30903,#30904,#30905,#30906));
#5767=EDGE_LOOP('',(#30907,#30908,#30909,#30910,#30911,#30912));
#5768=EDGE_LOOP('',(#30913,#30914,#30915,#30916,#30917,#30918));
#5769=EDGE_LOOP('',(#30919,#30920,#30921,#30922));
#5770=EDGE_LOOP('',(#30923,#30924,#30925,#30926,#30927,#30928));
#5771=EDGE_LOOP('',(#30929,#30930,#30931,#30932,#30933));
#5772=EDGE_LOOP('',(#30934,#30935,#30936,#30937,#30938,#30939));
#5773=EDGE_LOOP('',(#30940,#30941,#30942,#30943));
#5774=EDGE_LOOP('',(#30944,#30945,#30946,#30947,#30948,#30949));
#5775=EDGE_LOOP('',(#30950,#30951,#30952,#30953,#30954,#30955));
#5776=EDGE_LOOP('',(#30956,#30957,#30958,#30959,#30960,#30961));
#5777=EDGE_LOOP('',(#30962,#30963,#30964,#30965));
#5778=EDGE_LOOP('',(#30966,#30967,#30968,#30969,#30970,#30971));
#5779=EDGE_LOOP('',(#30972,#30973,#30974,#30975,#30976,#30977));
#5780=EDGE_LOOP('',(#30978,#30979,#30980,#30981,#30982));
#5781=EDGE_LOOP('',(#30983,#30984,#30985,#30986,#30987,#30988));
#5782=EDGE_LOOP('',(#30989,#30990,#30991,#30992,#30993,#30994));
#5783=EDGE_LOOP('',(#30995,#30996,#30997,#30998,#30999,#31000));
#5784=EDGE_LOOP('',(#31001,#31002,#31003,#31004));
#5785=EDGE_LOOP('',(#31005,#31006,#31007,#31008,#31009,#31010));
#5786=EDGE_LOOP('',(#31011,#31012,#31013,#31014,#31015,#31016));
#5787=EDGE_LOOP('',(#31017,#31018,#31019,#31020,#31021,#31022));
#5788=EDGE_LOOP('',(#31023,#31024,#31025,#31026));
#5789=EDGE_LOOP('',(#31027,#31028,#31029,#31030,#31031,#31032));
#5790=EDGE_LOOP('',(#31033,#31034,#31035,#31036,#31037,#31038));
#5791=EDGE_LOOP('',(#31039,#31040,#31041,#31042,#31043,#31044));
#5792=EDGE_LOOP('',(#31045,#31046,#31047,#31048));
#5793=EDGE_LOOP('',(#31049,#31050,#31051,#31052,#31053,#31054));
#5794=EDGE_LOOP('',(#31055,#31056,#31057,#31058,#31059,#31060));
#5795=EDGE_LOOP('',(#31061,#31062,#31063,#31064,#31065));
#5796=EDGE_LOOP('',(#31066,#31067,#31068,#31069,#31070,#31071));
#5797=EDGE_LOOP('',(#31072,#31073,#31074,#31075,#31076,#31077));
#5798=EDGE_LOOP('',(#31078,#31079,#31080,#31081,#31082,#31083));
#5799=EDGE_LOOP('',(#31084,#31085,#31086,#31087));
#5800=EDGE_LOOP('',(#31088,#31089,#31090,#31091,#31092,#31093));
#5801=EDGE_LOOP('',(#31094,#31095,#31096,#31097,#31098,#31099));
#5802=EDGE_LOOP('',(#31100,#31101,#31102,#31103,#31104,#31105));
#5803=EDGE_LOOP('',(#31106,#31107,#31108,#31109));
#5804=EDGE_LOOP('',(#31110,#31111,#31112,#31113,#31114,#31115));
#5805=EDGE_LOOP('',(#31116,#31117,#31118,#31119,#31120,#31121));
#5806=EDGE_LOOP('',(#31122,#31123,#31124,#31125,#31126,#31127));
#5807=EDGE_LOOP('',(#31128,#31129,#31130,#31131));
#5808=EDGE_LOOP('',(#31132,#31133,#31134,#31135,#31136,#31137,#31138,#31139));
#5809=EDGE_LOOP('',(#31140,#31141,#31142,#31143,#31144,#31145,#31146,#31147));
#5810=EDGE_LOOP('',(#31148,#31149,#31150,#31151,#31152));
#5811=EDGE_LOOP('',(#31153,#31154,#31155,#31156,#31157,#31158,#31159,#31160));
#7194=CIRCLE('',#40906,0.3);
#7195=CIRCLE('',#40908,0.3);
#7196=CIRCLE('',#40909,0.299999999997753);
#7197=CIRCLE('',#40911,0.3);
#7198=CIRCLE('',#40913,0.300000000000004);
#7199=CIRCLE('',#40916,38.4121320343559);
#7200=CIRCLE('',#40917,0.299999999999996);
#7201=CIRCLE('',#40918,38.5);
#7202=CIRCLE('',#40920,0.299999999999997);
#7203=CIRCLE('',#40921,0.299999999999999);
#7204=CIRCLE('',#40922,0.29999999999815);
#7205=CIRCLE('',#40924,0.3);
#7206=CIRCLE('',#40926,0.3);
#7207=CIRCLE('',#40928,0.3);
#7208=CIRCLE('',#40930,0.3);
#7209=CIRCLE('',#40932,37.8757359312881);
#7210=CIRCLE('',#40933,37.8757359312881);
#7211=CIRCLE('',#40934,37.8757359312881);
#7212=CIRCLE('',#40935,37.8757359312881);
#7213=CIRCLE('',#40936,37.8757359312881);
#7214=CIRCLE('',#40937,37.8757359312881);
#7215=CIRCLE('',#40938,37.8757359312881);
#7216=CIRCLE('',#40939,37.8757359312881);
#7217=CIRCLE('',#40940,37.8757359312881);
#7218=CIRCLE('',#40941,37.8757359312881);
#7219=CIRCLE('',#40942,37.8757359312881);
#7220=CIRCLE('',#40943,37.8757359312881);
#7221=CIRCLE('',#40944,37.8757359312881);
#7222=CIRCLE('',#40945,37.8757359312881);
#7223=CIRCLE('',#40946,37.8757359312881);
#7224=CIRCLE('',#40947,37.8757359312881);
#7225=CIRCLE('',#40948,37.8757359312881);
#7226=CIRCLE('',#40949,37.8757359312881);
#7227=CIRCLE('',#40950,37.8757359312881);
#7228=CIRCLE('',#40951,37.8757359312881);
#7229=CIRCLE('',#40952,37.8757359312881);
#7230=CIRCLE('',#40953,37.8757359312881);
#7231=CIRCLE('',#40954,37.8757359312881);
#7232=CIRCLE('',#40955,37.8757359312881);
#7233=CIRCLE('',#40956,37.8757359312881);
#7234=CIRCLE('',#40957,37.8757359312881);
#7235=CIRCLE('',#40958,37.8757359312881);
#7236=CIRCLE('',#40959,37.8757359312881);
#7237=CIRCLE('',#40960,37.8757359312881);
#7238=CIRCLE('',#40961,37.8757359312881);
#7239=CIRCLE('',#40962,37.8757359312881);
#7240=CIRCLE('',#40963,37.8757359312881);
#7241=CIRCLE('',#40964,37.8757359312881);
#7242=CIRCLE('',#40965,37.8757359312881);
#7243=CIRCLE('',#40966,37.8757359312881);
#7244=CIRCLE('',#40967,37.8757359312881);
#7245=CIRCLE('',#40968,37.8757359312881);
#7246=CIRCLE('',#40969,37.8757359312881);
#7247=CIRCLE('',#40970,37.8757359312881);
#7248=CIRCLE('',#40971,37.8757359312881);
#7249=CIRCLE('',#40972,37.8757359312881);
#7250=CIRCLE('',#40973,37.8757359312881);
#7251=CIRCLE('',#40974,37.8757359312881);
#7252=CIRCLE('',#40975,37.8757359312881);
#7253=CIRCLE('',#40976,37.8757359312881);
#7254=CIRCLE('',#40977,37.8757359312881);
#7255=CIRCLE('',#40978,37.8757359312881);
#7256=CIRCLE('',#40979,37.8757359312881);
#7257=CIRCLE('',#40980,33.3);
#7258=CIRCLE('',#40982,38.087867965644);
#7259=CIRCLE('',#40983,0.3);
#7260=CIRCLE('',#40985,38.4121320343559);
#7261=CIRCLE('',#40987,38.5);
#7262=CIRCLE('',#40988,0.300000000000002);
#7263=CIRCLE('',#40991,0.3);
#7264=CIRCLE('',#40993,0.3);
#7265=CIRCLE('',#40994,0.299999999997725);
#7266=CIRCLE('',#40996,0.3);
#7267=CIRCLE('',#40998,0.300000000000001);
#7268=CIRCLE('',#41001,38.4121320343559);
#7269=CIRCLE('',#41002,0.299999999999998);
#7270=CIRCLE('',#41003,38.5);
#7271=CIRCLE('',#41005,0.299999999999997);
#7272=CIRCLE('',#41006,0.300000000000001);
#7273=CIRCLE('',#41007,0.299999999998163);
#7274=CIRCLE('',#41009,0.3);
#7275=CIRCLE('',#41011,0.3);
#7276=CIRCLE('',#41013,0.3);
#7277=CIRCLE('',#41015,0.3);
#7278=CIRCLE('',#41017,38.087867965644);
#7279=CIRCLE('',#41018,0.3);
#7280=CIRCLE('',#41020,38.4121320343559);
#7281=CIRCLE('',#41022,38.5);
#7282=CIRCLE('',#41023,0.300000000000002);
#7283=CIRCLE('',#41026,0.3);
#7284=CIRCLE('',#41028,0.3);
#7285=CIRCLE('',#41029,0.299999999997753);
#7286=CIRCLE('',#41031,0.3);
#7287=CIRCLE('',#41033,0.300000000000002);
#7288=CIRCLE('',#41036,38.412132034356);
#7289=CIRCLE('',#41037,0.299999999999996);
#7290=CIRCLE('',#41038,38.5);
#7291=CIRCLE('',#41040,0.299999999999997);
#7292=CIRCLE('',#41041,0.299999999999999);
#7293=CIRCLE('',#41042,0.299999999998144);
#7294=CIRCLE('',#41044,0.3);
#7295=CIRCLE('',#41046,0.3);
#7296=CIRCLE('',#41048,0.3);
#7297=CIRCLE('',#41050,0.3);
#7298=CIRCLE('',#41052,38.087867965644);
#7299=CIRCLE('',#41053,0.3);
#7300=CIRCLE('',#41055,38.412132034356);
#7301=CIRCLE('',#41057,38.5);
#7302=CIRCLE('',#41058,0.300000000000002);
#7303=CIRCLE('',#41061,0.299999999999998);
#7304=CIRCLE('',#41063,0.299999999999998);
#7305=CIRCLE('',#41064,0.29999999999914);
#7306=CIRCLE('',#41066,0.3);
#7307=CIRCLE('',#41068,38.412132034356);
#7308=CIRCLE('',#41069,0.299999999999986);
#7309=CIRCLE('',#41070,38.5);
#7310=CIRCLE('',#41072,0.299999999999997);
#7311=CIRCLE('',#41074,0.3);
#7312=CIRCLE('',#41076,0.29999999999999);
#7313=CIRCLE('',#41078,0.300000000000001);
#7314=CIRCLE('',#41079,0.299999999999081);
#7315=CIRCLE('',#41081,0.3);
#7316=CIRCLE('',#41083,0.299999999999998);
#7317=CIRCLE('',#41085,38.087867965644);
#7318=CIRCLE('',#41086,0.3);
#7319=CIRCLE('',#41087,37.8757359312881);
#7320=CIRCLE('',#41089,38.412132034356);
#7321=CIRCLE('',#41091,38.5);
#7322=CIRCLE('',#41092,0.299999999999999);
#7323=CIRCLE('',#41095,0.299999999999998);
#7324=CIRCLE('',#41098,0.299999999999999);
#7325=CIRCLE('',#41100,0.300000000000002);
#7326=CIRCLE('',#41101,0.299999999998996);
#7327=CIRCLE('',#41103,0.3);
#7328=CIRCLE('',#41105,38.4121320343559);
#7329=CIRCLE('',#41106,0.299999999999997);
#7330=CIRCLE('',#41107,38.5);
#7331=CIRCLE('',#41109,0.299999999999994);
#7332=CIRCLE('',#41111,0.3);
#7333=CIRCLE('',#41113,0.299999999999999);
#7334=CIRCLE('',#41115,0.3);
#7335=CIRCLE('',#41116,0.299999999999051);
#7336=CIRCLE('',#41118,0.3);
#7337=CIRCLE('',#41120,0.300000000000001);
#7338=CIRCLE('',#41122,38.087867965644);
#7339=CIRCLE('',#41123,0.3);
#7340=CIRCLE('',#41124,37.8757359312881);
#7341=CIRCLE('',#41126,38.4121320343559);
#7342=CIRCLE('',#41128,38.5);
#7343=CIRCLE('',#41129,0.299999999999997);
#7344=CIRCLE('',#41132,0.300000000000001);
#7345=CIRCLE('',#41135,0.299999999999995);
#7346=CIRCLE('',#41137,0.300000000000001);
#7347=CIRCLE('',#41138,0.299999999999152);
#7348=CIRCLE('',#41140,0.3);
#7349=CIRCLE('',#41142,0.3);
#7350=CIRCLE('',#41144,0.3);
#7351=CIRCLE('',#41146,37.8757359312881);
#7352=CIRCLE('',#41147,37.8757359312881);
#7353=CIRCLE('',#41148,37.8757359312881);
#7354=CIRCLE('',#41149,37.8757359312881);
#7355=CIRCLE('',#41150,37.8757359312881);
#7356=CIRCLE('',#41151,37.8757359312881);
#7357=CIRCLE('',#41152,37.8757359312881);
#7358=CIRCLE('',#41153,37.8757359312881);
#7359=CIRCLE('',#41154,37.8757359312881);
#7360=CIRCLE('',#41155,37.8757359312881);
#7361=CIRCLE('',#41156,37.8757359312881);
#7362=CIRCLE('',#41157,37.8757359312881);
#7363=CIRCLE('',#41158,37.8757359312881);
#7364=CIRCLE('',#41159,37.8757359312881);
#7365=CIRCLE('',#41160,37.8757359312881);
#7366=CIRCLE('',#41161,37.8757359312881);
#7367=CIRCLE('',#41162,37.8757359312881);
#7368=CIRCLE('',#41163,37.8757359312881);
#7369=CIRCLE('',#41164,37.8757359312881);
#7370=CIRCLE('',#41165,37.8757359312881);
#7371=CIRCLE('',#41166,37.8757359312881);
#7372=CIRCLE('',#41167,37.8757359312881);
#7373=CIRCLE('',#41168,37.8757359312881);
#7374=CIRCLE('',#41169,37.8757359312881);
#7375=CIRCLE('',#41170,37.8757359312881);
#7376=CIRCLE('',#41171,37.8757359312881);
#7377=CIRCLE('',#41172,37.8757359312881);
#7378=CIRCLE('',#41173,37.8757359312881);
#7379=CIRCLE('',#41174,37.8757359312881);
#7380=CIRCLE('',#41175,37.8757359312881);
#7381=CIRCLE('',#41176,37.8757359312881);
#7382=CIRCLE('',#41177,37.8757359312881);
#7383=CIRCLE('',#41178,37.8757359312881);
#7384=CIRCLE('',#41179,37.8757359312881);
#7385=CIRCLE('',#41180,37.8757359312881);
#7386=CIRCLE('',#41181,37.8757359312881);
#7387=CIRCLE('',#41182,37.8757359312881);
#7388=CIRCLE('',#41183,37.8757359312881);
#7389=CIRCLE('',#41184,37.8757359312881);
#7390=CIRCLE('',#41185,37.8757359312881);
#7391=CIRCLE('',#41186,37.8757359312881);
#7392=CIRCLE('',#41187,37.8757359312881);
#7393=CIRCLE('',#41188,37.8757359312881);
#7394=CIRCLE('',#41189,37.8757359312881);
#7395=CIRCLE('',#41190,37.8757359312881);
#7396=CIRCLE('',#41191,37.8757359312881);
#7397=CIRCLE('',#41192,33.3);
#7398=CIRCLE('',#41194,38.087867965644);
#7399=CIRCLE('',#41195,0.3);
#7400=CIRCLE('',#41197,38.412132034356);
#7401=CIRCLE('',#41199,38.5);
#7402=CIRCLE('',#41200,0.300000000000003);
#7403=CIRCLE('',#41202,38.5);
#7404=CIRCLE('',#41204,0.299999999999999);
#7405=CIRCLE('',#41206,0.3);
#7406=CIRCLE('',#41207,0.299999999998215);
#7407=CIRCLE('',#41209,0.3);
#7408=CIRCLE('',#41211,0.3);
#7409=CIRCLE('',#41213,0.3);
#7410=CIRCLE('',#41215,38.087867965644);
#7411=CIRCLE('',#41216,0.3);
#7412=CIRCLE('',#41218,38.412132034356);
#7413=CIRCLE('',#41220,38.5);
#7414=CIRCLE('',#41221,0.300000000000001);
#7415=CIRCLE('',#41223,38.5);
#7416=CIRCLE('',#41225,0.299999999999998);
#7417=CIRCLE('',#41227,0.299999999999998);
#7418=CIRCLE('',#41228,0.299999999999141);
#7419=CIRCLE('',#41230,0.3);
#7420=CIRCLE('',#41232,0.3);
#7421=CIRCLE('',#41234,0.3);
#7422=CIRCLE('',#41236,38.087867965644);
#7423=CIRCLE('',#41237,0.3);
#7424=CIRCLE('',#41239,38.4121320343559);
#7425=CIRCLE('',#41241,38.5);
#7426=CIRCLE('',#41242,0.300000000000002);
#7427=CIRCLE('',#41244,38.5);
#7428=CIRCLE('',#41246,0.300000000000002);
#7429=CIRCLE('',#41249,0.300000000000001);
#7430=CIRCLE('',#41251,0.300000000000001);
#7431=CIRCLE('',#41252,0.29999999999857);
#7432=CIRCLE('',#41254,0.3);
#7433=CIRCLE('',#41256,38.412132034356);
#7434=CIRCLE('',#41257,0.299999999999997);
#7435=CIRCLE('',#41258,38.5);
#7436=CIRCLE('',#41260,0.299999999999997);
#7437=CIRCLE('',#41262,0.3);
#7438=CIRCLE('',#41263,0.299999999999999);
#7439=CIRCLE('',#41264,0.299999999998807);
#7440=CIRCLE('',#41266,0.299999999999998);
#7441=CIRCLE('',#41268,0.3);
#7442=CIRCLE('',#41270,38.5);
#7443=CIRCLE('',#41272,0.299999999999998);
#7444=CIRCLE('',#41274,0.3);
#7445=CIRCLE('',#41276,38.087867965644);
#7446=CIRCLE('',#41279,0.300000000000002);
#7447=CIRCLE('',#41281,0.300000000000002);
#7448=CIRCLE('',#41282,0.299999999998997);
#7449=CIRCLE('',#41284,0.3);
#7450=CIRCLE('',#41286,0.299999999999993);
#7451=CIRCLE('',#41288,0.3);
#7452=CIRCLE('',#41290,38.087867965644);
#7453=CIRCLE('',#41291,0.3);
#7454=CIRCLE('',#41293,38.412132034356);
#7455=CIRCLE('',#41295,38.5);
#7456=CIRCLE('',#41296,0.299999999999995);
#7457=CIRCLE('',#41298,38.5);
#7458=CIRCLE('',#41300,0.299999999999999);
#7459=CIRCLE('',#41302,0.299999999999999);
#7460=CIRCLE('',#41303,0.299999999999106);
#7461=CIRCLE('',#41305,0.3);
#7462=CIRCLE('',#41307,0.299999999999996);
#7463=CIRCLE('',#41309,0.3);
#7464=CIRCLE('',#41311,38.087867965644);
#7465=CIRCLE('',#41312,0.3);
#7466=CIRCLE('',#41314,38.412132034356);
#7467=CIRCLE('',#41316,38.5);
#7468=CIRCLE('',#41317,0.299999999999996);
#7469=CIRCLE('',#41319,38.5);
#7470=CIRCLE('',#41321,0.299999999999998);
#7471=CIRCLE('',#41323,0.3);
#7472=CIRCLE('',#41324,0.299999999998809);
#7473=CIRCLE('',#41326,0.3);
#7474=CIRCLE('',#41328,0.299999999999997);
#7475=CIRCLE('',#41330,0.3);
#7476=CIRCLE('',#41332,38.087867965644);
#7477=CIRCLE('',#41333,0.3);
#7478=CIRCLE('',#41335,38.412132034356);
#7479=CIRCLE('',#41337,0.300000000000001);
#7480=CIRCLE('',#41340,0.3);
#7481=CIRCLE('',#41342,0.300000000000001);
#7482=CIRCLE('',#41343,0.299999999998212);
#7483=CIRCLE('',#41345,0.3);
#7484=CIRCLE('',#41347,38.4121320343559);
#7485=CIRCLE('',#41348,0.299999999999998);
#7486=CIRCLE('',#41349,38.5);
#7487=CIRCLE('',#41351,0.300000000000004);
#7488=CIRCLE('',#41353,0.3);
#7489=CIRCLE('',#41354,0.299999999999999);
#7490=CIRCLE('',#41355,0.299999999998551);
#7491=CIRCLE('',#41357,0.300000000000001);
#7492=CIRCLE('',#41359,0.3);
#7493=CIRCLE('',#41361,38.5);
#7494=CIRCLE('',#41363,0.300000000000001);
#7495=CIRCLE('',#41365,0.3);
#7496=CIRCLE('',#41367,38.087867965644);
#7497=CIRCLE('',#41369,0.300000000000002);
#7498=CIRCLE('',#41370,0.300000000000004);
#7499=CIRCLE('',#41372,38.5);
#7500=CIRCLE('',#41373,0.299999999999997);
#7501=CIRCLE('',#41375,0.299999999999999);
#7502=CIRCLE('',#41377,0.300000000000011);
#7503=CIRCLE('',#41381,0.3);
#7504=CIRCLE('',#41382,0.299999999999998);
#7505=CIRCLE('',#41383,0.300000000000003);
#7506=CIRCLE('',#41385,0.299999999999994);
#7507=CIRCLE('',#41389,0.300000000000001);
#7508=CIRCLE('',#41391,0.3);
#7509=CIRCLE('',#41393,0.300000000000002);
#7510=CIRCLE('',#41395,0.3);
#7511=CIRCLE('',#41396,0.299999999998203);
#7512=CIRCLE('',#41398,0.3);
#7513=CIRCLE('',#41400,0.3);
#7514=CIRCLE('',#41402,0.3);
#7515=CIRCLE('',#41404,38.087867965644);
#7516=CIRCLE('',#41405,0.3);
#7517=CIRCLE('',#41407,38.412132034356);
#7518=CIRCLE('',#41409,38.5);
#7519=CIRCLE('',#41410,0.299999999999992);
#7520=CIRCLE('',#41412,38.5);
#7521=CIRCLE('',#41413,0.300000000000003);
#7522=CIRCLE('',#41414,0.300000000000002);
#7523=CIRCLE('',#41416,0.299999999999994);
#7524=CIRCLE('',#41420,0.300000000000001);
#7525=CIRCLE('',#41422,0.3);
#7526=CIRCLE('',#41424,0.299999999999998);
#7527=CIRCLE('',#41426,0.299999999999998);
#7528=CIRCLE('',#41427,0.299999999999155);
#7529=CIRCLE('',#41429,0.3);
#7530=CIRCLE('',#41431,0.299999999999994);
#7531=CIRCLE('',#41433,0.3);
#7532=CIRCLE('',#41435,38.087867965644);
#7533=CIRCLE('',#41436,0.3);
#7534=CIRCLE('',#41438,38.412132034356);
#7535=CIRCLE('',#41439,0.300000000000003);
#7536=CIRCLE('',#41440,0.300000000000003);
#7537=CIRCLE('',#41442,0.299999999999994);
#7538=CIRCLE('',#41446,0.299999999999998);
#7539=CIRCLE('',#41449,0.3);
#7540=CIRCLE('',#41450,0.299999999999999);
#7541=CIRCLE('',#41451,0.300000000000003);
#7542=CIRCLE('',#41453,38.5);
#7543=CIRCLE('',#41454,0.299999999999999);
#7544=CIRCLE('',#41456,0.299999999999998);
#7545=CIRCLE('',#41458,0.300000000000011);
#7546=CIRCLE('',#41462,0.3);
#7547=CIRCLE('',#41465,0.3);
#7548=CIRCLE('',#41467,0.3);
#7549=CIRCLE('',#41469,0.299999999999998);
#7550=CIRCLE('',#41470,0.299999999998855);
#7551=CIRCLE('',#41472,0.3);
#7552=CIRCLE('',#41474,0.300000000000002);
#7553=CIRCLE('',#41476,0.3);
#7554=CIRCLE('',#41478,38.087867965644);
#7555=CIRCLE('',#41479,0.3);
#7556=CIRCLE('',#41481,38.412132034356);
#7557=CIRCLE('',#41483,0.3);
#7558=CIRCLE('',#41485,0.299999999999999);
#7559=CIRCLE('',#41486,0.299999999998599);
#7560=CIRCLE('',#41488,0.3);
#7561=CIRCLE('',#41490,0.299999999999993);
#7562=CIRCLE('',#41492,0.3);
#7563=CIRCLE('',#41494,38.087867965644);
#7564=CIRCLE('',#41495,0.3);
#7565=CIRCLE('',#41497,38.412132034356);
#7566=CIRCLE('',#41499,38.5);
#7567=CIRCLE('',#41500,0.29999999999999);
#7568=CIRCLE('',#41502,38.5);
#7569=CIRCLE('',#41504,0.3);
#7570=CIRCLE('',#41506,0.3);
#7571=CIRCLE('',#41507,0.299999999998876);
#7572=CIRCLE('',#41509,0.3);
#7573=CIRCLE('',#41511,0.299999999999998);
#7574=CIRCLE('',#41513,0.3);
#7575=CIRCLE('',#41515,38.087867965644);
#7576=CIRCLE('',#41516,0.3);
#7577=CIRCLE('',#41518,38.412132034356);
#7578=CIRCLE('',#41520,38.5);
#7579=CIRCLE('',#41521,0.299999999999995);
#7580=CIRCLE('',#41523,38.5);
#7581=CIRCLE('',#41524,0.299999999999999);
#7582=CIRCLE('',#41525,0.299999999999998);
#7583=CIRCLE('',#41527,0.299999999999994);
#7584=CIRCLE('',#41531,0.299999999999999);
#7585=CIRCLE('',#41533,0.3);
#7586=CIRCLE('',#41535,0.3);
#7587=CIRCLE('',#41537,0.3);
#7588=CIRCLE('',#41538,0.299999999998817);
#7589=CIRCLE('',#41540,0.3);
#7590=CIRCLE('',#41542,0.300000000000003);
#7591=CIRCLE('',#41544,0.3);
#7592=CIRCLE('',#41546,38.087867965644);
#7593=CIRCLE('',#41547,0.3);
#7594=CIRCLE('',#41549,38.412132034356);
#7595=CIRCLE('',#41551,38.5);
#7596=CIRCLE('',#41552,0.299999999999992);
#7597=CIRCLE('',#41554,38.5);
#7598=CIRCLE('',#41555,0.3);
#7599=CIRCLE('',#41556,0.299999999999997);
#7600=CIRCLE('',#41558,0.299999999999994);
#7601=CIRCLE('',#41562,0.299999999999999);
#7602=CIRCLE('',#41564,0.3);
#7603=CIRCLE('',#41567,0.3);
#7604=CIRCLE('',#41569,0.299999999999992);
#7605=CIRCLE('',#41571,0.300000000000001);
#7606=CIRCLE('',#41572,0.299999999999146);
#7607=CIRCLE('',#41574,0.3);
#7608=CIRCLE('',#41576,0.3);
#7609=CIRCLE('',#41578,0.3);
#7610=CIRCLE('',#41580,38.087867965644);
#7611=CIRCLE('',#41581,0.3);
#7612=CIRCLE('',#41583,38.412132034356);
#7613=CIRCLE('',#41585,38.5);
#7614=CIRCLE('',#41586,0.299999999999999);
#7615=CIRCLE('',#41588,38.5);
#7616=CIRCLE('',#41590,0.300000000000006);
#7617=CIRCLE('',#41592,0.300000000000002);
#7618=CIRCLE('',#41593,0.299999999998997);
#7619=CIRCLE('',#41595,0.3);
#7620=CIRCLE('',#41597,0.299999999999998);
#7621=CIRCLE('',#41599,0.3);
#7622=CIRCLE('',#41601,38.087867965644);
#7623=CIRCLE('',#41602,0.3);
#7624=CIRCLE('',#41604,38.412132034356);
#7625=CIRCLE('',#41606,38.5);
#7626=CIRCLE('',#41607,0.299999999999997);
#7627=CIRCLE('',#41609,38.5);
#7628=CIRCLE('',#41611,0.299999999999998);
#7629=CIRCLE('',#41613,0.3);
#7630=CIRCLE('',#41614,0.299999999998819);
#7631=CIRCLE('',#41616,0.3);
#7632=CIRCLE('',#41618,0.299999999999997);
#7633=CIRCLE('',#41620,0.3);
#7634=CIRCLE('',#41622,38.087867965644);
#7635=CIRCLE('',#41623,0.3);
#7636=CIRCLE('',#41625,38.412132034356);
#7637=CIRCLE('',#41626,0.3);
#7638=CIRCLE('',#41627,0.299999999999997);
#7639=CIRCLE('',#41629,0.299999999999994);
#7640=CIRCLE('',#41633,0.299999999999999);
#7641=CIRCLE('',#41635,0.3);
#7642=CIRCLE('',#41636,0.3);
#7643=CIRCLE('',#41637,0.300000000000002);
#7644=CIRCLE('',#41639,0.299999999999994);
#7645=CIRCLE('',#41643,0.299999999999999);
#7646=CIRCLE('',#41645,0.3);
#7647=CIRCLE('',#41647,0.299999999999998);
#7648=CIRCLE('',#41649,0.3);
#7649=CIRCLE('',#41650,0.29999999999775);
#7650=CIRCLE('',#41652,0.3);
#7651=CIRCLE('',#41654,0.299999999999997);
#7652=CIRCLE('',#41656,0.3);
#7653=CIRCLE('',#41658,38.087867965644);
#7654=CIRCLE('',#41659,0.3);
#7655=CIRCLE('',#41661,38.412132034356);
#7656=CIRCLE('',#41663,38.5);
#7657=CIRCLE('',#41664,0.299999999999997);
#7658=CIRCLE('',#41666,38.5);
#7659=CIRCLE('',#41667,0.299999999999999);
#7660=CIRCLE('',#41668,0.300000000000002);
#7661=CIRCLE('',#41670,0.299999999999994);
#7662=CIRCLE('',#41674,0.3);
#7663=CIRCLE('',#41676,0.3);
#7664=CIRCLE('',#41679,0.3);
#7665=CIRCLE('',#41682,0.3);
#7666=CIRCLE('',#41683,0.300000000000002);
#7667=CIRCLE('',#41684,0.3);
#7668=CIRCLE('',#41686,38.5);
#7669=CIRCLE('',#41687,0.299999999999992);
#7670=CIRCLE('',#41689,0.300000000000001);
#7671=CIRCLE('',#41691,0.300000000000011);
#7672=CIRCLE('',#41695,0.3);
#7673=CIRCLE('',#41696,0.299999999999999);
#7674=CIRCLE('',#41697,0.300000000000002);
#7675=CIRCLE('',#41699,0.299999999999994);
#7676=CIRCLE('',#41703,0.300000000000002);
#7677=CIRCLE('',#41705,0.3);
#7678=CIRCLE('',#41707,0.299999999999992);
#7679=CIRCLE('',#41709,0.299999999999998);
#7680=CIRCLE('',#41710,0.299999999999148);
#7681=CIRCLE('',#41712,0.3);
#7682=CIRCLE('',#41714,0.299999999999994);
#7683=CIRCLE('',#41716,0.3);
#7684=CIRCLE('',#41718,38.087867965644);
#7685=CIRCLE('',#41719,0.3);
#7686=CIRCLE('',#41721,38.412132034356);
#7687=CIRCLE('',#41722,0.300000000000003);
#7688=CIRCLE('',#41723,0.300000000000003);
#7689=CIRCLE('',#41725,0.299999999999994);
#7690=CIRCLE('',#41729,0.300000000000001);
#7691=CIRCLE('',#41731,0.3);
#7692=CIRCLE('',#41733,0.300000000000005);
#7693=CIRCLE('',#41735,0.300000000000003);
#7694=CIRCLE('',#41736,0.2999999999991);
#7695=CIRCLE('',#41738,0.3);
#7696=CIRCLE('',#41740,0.299999999999996);
#7697=CIRCLE('',#41742,0.3);
#7698=CIRCLE('',#41744,38.087867965644);
#7699=CIRCLE('',#41745,0.3);
#7700=CIRCLE('',#41747,38.412132034356);
#7701=CIRCLE('',#41749,38.5);
#7702=CIRCLE('',#41750,0.29999999999999);
#7703=CIRCLE('',#41752,38.5);
#7704=CIRCLE('',#41753,0.300000000000002);
#7705=CIRCLE('',#41754,0.299999999999999);
#7706=CIRCLE('',#41756,0.299999999999994);
#7707=CIRCLE('',#41760,0.300000000000001);
#7708=CIRCLE('',#41762,0.3);
#7709=CIRCLE('',#41765,0.3);
#7710=CIRCLE('',#41766,0.299999999999999);
#7711=CIRCLE('',#41767,0.299999999999998);
#7712=CIRCLE('',#41769,38.5);
#7713=CIRCLE('',#41770,0.299999999999999);
#7714=CIRCLE('',#41772,0.300000000000001);
#7715=CIRCLE('',#41774,0.300000000000011);
#7716=CIRCLE('',#41778,0.3);
#7717=CIRCLE('',#41781,0.3);
#7718=CIRCLE('',#41783,0.299999999999998);
#7719=CIRCLE('',#41785,0.299999999999999);
#7720=CIRCLE('',#41786,0.299999999998599);
#7721=CIRCLE('',#41788,0.3);
#7722=CIRCLE('',#41790,0.299999999999997);
#7723=CIRCLE('',#41792,0.3);
#7724=CIRCLE('',#41794,38.087867965644);
#7725=CIRCLE('',#41795,0.3);
#7726=CIRCLE('',#41797,38.412132034356);
#7727=CIRCLE('',#41799,38.5);
#7728=CIRCLE('',#41800,0.3);
#7729=CIRCLE('',#41802,38.5);
#7730=CIRCLE('',#41804,0.299999999999998);
#7731=CIRCLE('',#41806,0.3);
#7732=CIRCLE('',#41807,0.29999999999886);
#7733=CIRCLE('',#41809,0.3);
#7734=CIRCLE('',#41811,0.299999999999997);
#7735=CIRCLE('',#41813,0.3);
#7736=CIRCLE('',#41815,38.087867965644);
#7737=CIRCLE('',#41816,0.3);
#7738=CIRCLE('',#41818,38.4121320343559);
#7739=CIRCLE('',#41820,38.5);
#7740=CIRCLE('',#41821,0.299999999999997);
#7741=CIRCLE('',#41823,38.5);
#7742=CIRCLE('',#41825,0.299999999999998);
#7743=CIRCLE('',#41827,0.299999999999998);
#7744=CIRCLE('',#41828,0.299999999998856);
#7745=CIRCLE('',#41830,0.3);
#7746=CIRCLE('',#41832,0.299999999999998);
#7747=CIRCLE('',#41834,0.3);
#7748=CIRCLE('',#41836,38.087867965644);
#7749=CIRCLE('',#41837,0.3);
#7750=CIRCLE('',#41839,38.412132034356);
#7751=CIRCLE('',#41841,0.3);
#7752=CIRCLE('',#41843,0.3);
#7753=CIRCLE('',#41844,0.299999999998808);
#7754=CIRCLE('',#41846,0.3);
#7755=CIRCLE('',#41848,0.299999999999997);
#7756=CIRCLE('',#41850,0.3);
#7757=CIRCLE('',#41852,38.087867965644);
#7758=CIRCLE('',#41853,0.3);
#7759=CIRCLE('',#41855,38.412132034356);
#7760=CIRCLE('',#41857,38.5);
#7761=CIRCLE('',#41858,0.299999999999998);
#7762=CIRCLE('',#41860,38.5);
#7763=CIRCLE('',#41861,0.3);
#7764=CIRCLE('',#41862,0.299999999999997);
#7765=CIRCLE('',#41864,0.299999999999994);
#7766=CIRCLE('',#41868,0.299999999999999);
#7767=CIRCLE('',#41870,0.3);
#7768=CIRCLE('',#41871,0.300000000000001);
#7769=CIRCLE('',#41872,0.300000000000003);
#7770=CIRCLE('',#41874,38.5);
#7771=CIRCLE('',#41875,0.299999999999996);
#7772=CIRCLE('',#41877,0.3);
#7773=CIRCLE('',#41879,0.300000000000011);
#7774=CIRCLE('',#41883,0.3);
#7775=CIRCLE('',#41885,0.299999999999996);
#7776=CIRCLE('',#41887,0.299999999999999);
#7777=CIRCLE('',#41888,0.299999999999114);
#7778=CIRCLE('',#41890,0.3);
#7779=CIRCLE('',#41892,0.299999999999996);
#7780=CIRCLE('',#41894,0.3);
#7781=CIRCLE('',#41896,38.087867965644);
#7782=CIRCLE('',#41897,0.3);
#7783=CIRCLE('',#41899,38.412132034356);
#7784=CIRCLE('',#41901,38.5);
#7785=CIRCLE('',#41902,0.299999999999986);
#7786=CIRCLE('',#41904,38.5);
#7787=CIRCLE('',#41906,0.3);
#7788=CIRCLE('',#41908,0.3);
#7789=CIRCLE('',#41909,0.299999999998806);
#7790=CIRCLE('',#41911,0.3);
#7791=CIRCLE('',#41913,0.299999999999997);
#7792=CIRCLE('',#41915,0.3);
#7793=CIRCLE('',#41917,38.087867965644);
#7794=CIRCLE('',#41918,0.3);
#7795=CIRCLE('',#41920,38.412132034356);
#7796=CIRCLE('',#41921,0.3);
#7797=CIRCLE('',#41922,0.300000000000003);
#7798=CIRCLE('',#41924,0.299999999999994);
#7799=CIRCLE('',#41928,0.300000000000002);
#7800=CIRCLE('',#41930,0.3);
#7801=CIRCLE('',#41931,0.3);
#7802=CIRCLE('',#41932,0.299999999999999);
#7803=CIRCLE('',#41934,0.299999999999994);
#7804=CIRCLE('',#41938,0.300000000000001);
#7805=CIRCLE('',#41940,0.3);
#7806=CIRCLE('',#41942,0.3);
#7807=CIRCLE('',#41944,0.3);
#7808=CIRCLE('',#41945,0.299999999997747);
#7809=CIRCLE('',#41947,0.3);
#7810=CIRCLE('',#41949,0.299999999999997);
#7811=CIRCLE('',#41951,0.3);
#7812=CIRCLE('',#41953,38.087867965644);
#7813=CIRCLE('',#41954,0.3);
#7814=CIRCLE('',#41956,38.412132034356);
#7815=CIRCLE('',#41958,38.5);
#7816=CIRCLE('',#41959,0.299999999999993);
#7817=CIRCLE('',#41961,38.5);
#7818=CIRCLE('',#41962,0.300000000000001);
#7819=CIRCLE('',#41963,0.299999999999998);
#7820=CIRCLE('',#41965,0.299999999999994);
#7821=CIRCLE('',#41969,0.299999999999999);
#7822=CIRCLE('',#41972,0.3);
#7823=CIRCLE('',#41973,0.3);
#7824=CIRCLE('',#41974,0.299999999999999);
#7825=CIRCLE('',#41976,0.299999999999994);
#7826=CIRCLE('',#41980,0.300000000000001);
#7827=CIRCLE('',#41982,0.3);
#7828=CIRCLE('',#41985,0.3);
#7829=CIRCLE('',#41988,0.3);
#7830=CIRCLE('',#41989,0.3);
#7831=CIRCLE('',#41990,0.3);
#7832=CIRCLE('',#41992,38.5);
#7833=CIRCLE('',#41993,0.299999999999997);
#7834=CIRCLE('',#41995,0.300000000000001);
#7835=CIRCLE('',#41997,0.300000000000011);
#7836=CIRCLE('',#42001,0.3);
#7837=CIRCLE('',#42002,0.299999999999998);
#7838=CIRCLE('',#42003,0.299999999999998);
#7839=CIRCLE('',#42005,0.299999999999994);
#7840=CIRCLE('',#42009,0.300000000000001);
#7841=CIRCLE('',#42011,0.3);
#7842=CIRCLE('',#42013,0.300000000000002);
#7843=CIRCLE('',#42015,0.300000000000001);
#7844=CIRCLE('',#42016,0.299999999998215);
#7845=CIRCLE('',#42018,0.3);
#7846=CIRCLE('',#42020,0.3);
#7847=CIRCLE('',#42022,0.3);
#7848=CIRCLE('',#42024,38.087867965644);
#7849=CIRCLE('',#42025,0.3);
#7850=CIRCLE('',#42027,38.412132034356);
#7851=CIRCLE('',#42029,38.5);
#7852=CIRCLE('',#42030,0.299999999999997);
#7853=CIRCLE('',#42032,38.5);
#7854=CIRCLE('',#42033,0.299999999999999);
#7855=CIRCLE('',#42034,0.299999999999999);
#7856=CIRCLE('',#42036,0.299999999999994);
#7857=CIRCLE('',#42040,0.299999999999998);
#7858=CIRCLE('',#42043,0.3);
#7859=CIRCLE('',#42045,0.299999999999998);
#7860=CIRCLE('',#42047,0.299999999999998);
#7861=CIRCLE('',#42048,0.299999999998599);
#7862=CIRCLE('',#42050,0.3);
#7863=CIRCLE('',#42052,0.300000000000002);
#7864=CIRCLE('',#42054,0.3);
#7865=CIRCLE('',#42056,38.087867965644);
#7866=CIRCLE('',#42057,0.3);
#7867=CIRCLE('',#42059,38.412132034356);
#7868=CIRCLE('',#42061,38.5);
#7869=CIRCLE('',#42062,0.299999999999995);
#7870=CIRCLE('',#42064,38.5);
#7871=CIRCLE('',#42066,0.299999999999998);
#7872=CIRCLE('',#42068,0.3);
#7873=CIRCLE('',#42069,0.299999999998861);
#7874=CIRCLE('',#42071,0.3);
#7875=CIRCLE('',#42073,0.300000000000001);
#7876=CIRCLE('',#42075,0.3);
#7877=CIRCLE('',#42077,38.087867965644);
#7878=CIRCLE('',#42078,0.3);
#7879=CIRCLE('',#42080,38.4121320343559);
#7880=CIRCLE('',#42082,38.5);
#7881=CIRCLE('',#42083,0.299999999999996);
#7882=CIRCLE('',#42085,38.5);
#7883=CIRCLE('',#42086,0.3);
#7884=CIRCLE('',#42087,0.299999999999995);
#7885=CIRCLE('',#42089,0.299999999999994);
#7886=CIRCLE('',#42093,0.3);
#7887=CIRCLE('',#42095,0.3);
#7888=CIRCLE('',#42097,0.3);
#7889=CIRCLE('',#42099,0.3);
#7890=CIRCLE('',#42100,0.299999999998866);
#7891=CIRCLE('',#42102,0.3);
#7892=CIRCLE('',#42104,0.299999999999997);
#7893=CIRCLE('',#42106,0.3);
#7894=CIRCLE('',#42108,38.087867965644);
#7895=CIRCLE('',#42109,0.3);
#7896=CIRCLE('',#42111,38.412132034356);
#7897=CIRCLE('',#42113,0.299999999999996);
#7898=CIRCLE('',#42115,0.3);
#7899=CIRCLE('',#42116,0.299999999998814);
#7900=CIRCLE('',#42118,0.3);
#7901=CIRCLE('',#42120,0.299999999999992);
#7902=CIRCLE('',#42122,0.3);
#7903=CIRCLE('',#42124,38.087867965644);
#7904=CIRCLE('',#42125,0.3);
#7905=CIRCLE('',#42127,38.4121320343559);
#7906=CIRCLE('',#42129,38.5);
#7907=CIRCLE('',#42130,0.299999999999993);
#7908=CIRCLE('',#42132,38.5);
#7909=CIRCLE('',#42133,0.299999999999999);
#7910=CIRCLE('',#42134,0.300000000000002);
#7911=CIRCLE('',#42136,0.299999999999994);
#7912=CIRCLE('',#42141,0.300000000000004);
#7913=CIRCLE('',#42143,0.299999999999998);
#7914=CIRCLE('',#42144,0.299999999999137);
#7915=CIRCLE('',#42146,0.3);
#7916=CIRCLE('',#42148,0.299999999999991);
#7917=CIRCLE('',#42150,0.3);
#7918=CIRCLE('',#42152,38.087867965644);
#7919=CIRCLE('',#42153,0.3);
#7920=CIRCLE('',#42155,38.412132034356);
#7921=CIRCLE('',#42156,0.299999999999999);
#7922=CIRCLE('',#42157,0.299999999999998);
#7923=CIRCLE('',#42159,38.5);
#7924=CIRCLE('',#42160,0.299999999999999);
#7925=CIRCLE('',#42162,0.299999999999998);
#7926=CIRCLE('',#42164,0.300000000000011);
#7927=CIRCLE('',#42168,0.3);
#7928=CIRCLE('',#42169,0.3);
#7929=CIRCLE('',#42170,0.299999999999999);
#7930=CIRCLE('',#42172,0.299999999999994);
#7931=CIRCLE('',#42176,0.299999999999999);
#7932=CIRCLE('',#42178,0.3);
#7933=CIRCLE('',#42179,0.300000000000001);
#7934=CIRCLE('',#42180,0.299999999999999);
#7935=CIRCLE('',#42182,38.5);
#7936=CIRCLE('',#42183,0.299999999999997);
#7937=CIRCLE('',#42185,0.300000000000002);
#7938=CIRCLE('',#42187,0.300000000000011);
#7939=CIRCLE('',#42191,0.3);
#7940=CIRCLE('',#42194,0.3);
#7941=CIRCLE('',#42195,0.3);
#7942=CIRCLE('',#42196,0.299999999999997);
#7943=CIRCLE('',#42198,0.299999999999994);
#7944=CIRCLE('',#42202,0.300000000000002);
#7945=CIRCLE('',#42204,0.3);
#7946=CIRCLE('',#42205,0.3);
#7947=CIRCLE('',#42206,0.299999999999999);
#7948=CIRCLE('',#42208,0.299999999999994);
#7949=CIRCLE('',#42212,0.300000000000001);
#7950=CIRCLE('',#42214,0.3);
#7951=CIRCLE('',#42216,0.3);
#7952=CIRCLE('',#42218,0.3);
#7953=CIRCLE('',#42219,0.29999999999775);
#7954=CIRCLE('',#42221,0.3);
#7955=CIRCLE('',#42223,0.299999999999997);
#7956=CIRCLE('',#42225,0.3);
#7957=CIRCLE('',#42227,38.087867965644);
#7958=CIRCLE('',#42228,0.3);
#7959=CIRCLE('',#42230,38.412132034356);
#7960=CIRCLE('',#42232,38.5);
#7961=CIRCLE('',#42233,0.300000000000002);
#7962=CIRCLE('',#42235,38.5);
#7963=CIRCLE('',#42236,0.3);
#7964=CIRCLE('',#42237,0.299999999999999);
#7965=CIRCLE('',#42239,0.299999999999994);
#7966=CIRCLE('',#42243,0.3);
#7967=CIRCLE('',#42245,0.3);
#7968=CIRCLE('',#42248,0.3);
#7969=CIRCLE('',#42251,0.3);
#7970=CIRCLE('',#42253,0.300000000000006);
#7971=CIRCLE('',#42255,0.300000000000002);
#7972=CIRCLE('',#42256,0.299999999998989);
#7973=CIRCLE('',#42258,0.3);
#7974=CIRCLE('',#42260,0.299999999999998);
#7975=CIRCLE('',#42262,0.3);
#7976=CIRCLE('',#42264,38.087867965644);
#7977=CIRCLE('',#42265,0.3);
#7978=CIRCLE('',#42267,38.412132034356);
#7979=CIRCLE('',#42269,38.5);
#7980=CIRCLE('',#42270,0.299999999999994);
#7981=CIRCLE('',#42272,38.5);
#7982=CIRCLE('',#42274,0.299999999999998);
#7983=CIRCLE('',#42276,0.3);
#7984=CIRCLE('',#42277,0.299999999998862);
#7985=CIRCLE('',#42279,0.3);
#7986=CIRCLE('',#42281,0.299999999999993);
#7987=CIRCLE('',#42283,0.3);
#7988=CIRCLE('',#42285,38.087867965644);
#7989=CIRCLE('',#42286,0.3);
#7990=CIRCLE('',#42288,38.4121320343559);
#7991=CIRCLE('',#42290,0.3);
#7992=CIRCLE('',#42292,0.3);
#7993=CIRCLE('',#42293,0.299999999998811);
#7994=CIRCLE('',#42295,0.3);
#7995=CIRCLE('',#42297,0.299999999999996);
#7996=CIRCLE('',#42299,0.3);
#7997=CIRCLE('',#42301,38.087867965644);
#7998=CIRCLE('',#42302,0.3);
#7999=CIRCLE('',#42304,38.4121320343559);
#8000=CIRCLE('',#42306,38.5);
#8001=CIRCLE('',#42307,0.299999999999998);
#8002=CIRCLE('',#42309,38.5);
#8003=CIRCLE('',#42311,0.300000000000003);
#8004=CIRCLE('',#42313,0.299999999999999);
#8005=CIRCLE('',#42314,0.2999999999991);
#8006=CIRCLE('',#42316,0.3);
#8007=CIRCLE('',#42318,0.3);
#8008=CIRCLE('',#42320,0.3);
#8009=CIRCLE('',#42322,38.087867965644);
#8010=CIRCLE('',#42323,0.3);
#8011=CIRCLE('',#42325,38.412132034356);
#8012=CIRCLE('',#42327,38.5);
#8013=CIRCLE('',#42328,0.299999999999996);
#8014=CIRCLE('',#42330,38.5);
#8015=CIRCLE('',#42332,0.3);
#8016=CIRCLE('',#42334,0.299999999999998);
#8017=CIRCLE('',#42335,0.299999999998821);
#8018=CIRCLE('',#42337,0.3);
#8019=CIRCLE('',#42339,0.299999999999997);
#8020=CIRCLE('',#42341,0.3);
#8021=CIRCLE('',#42343,38.087867965644);
#8022=CIRCLE('',#42344,0.3);
#8023=CIRCLE('',#42346,38.412132034356);
#8024=CIRCLE('',#42347,0.300000000000002);
#8025=CIRCLE('',#42348,0.299999999999997);
#8026=CIRCLE('',#42350,38.5);
#8027=CIRCLE('',#42351,0.300000000000003);
#8028=CIRCLE('',#42353,0.300000000000001);
#8029=CIRCLE('',#42355,0.300000000000011);
#8030=CIRCLE('',#42359,0.3);
#8031=CIRCLE('',#42360,0.300000000000002);
#8032=CIRCLE('',#42361,0.299999999999999);
#8033=CIRCLE('',#42363,0.299999999999994);
#8034=CIRCLE('',#42367,0.3);
#8035=CIRCLE('',#42369,0.3);
#8036=CIRCLE('',#42370,0.3);
#8037=CIRCLE('',#42371,0.299999999999999);
#8038=CIRCLE('',#42373,0.299999999999994);
#8039=CIRCLE('',#42377,0.300000000000001);
#8040=CIRCLE('',#42379,0.3);
#8041=CIRCLE('',#42380,0.300000000000001);
#8042=CIRCLE('',#42381,0.300000000000002);
#8043=CIRCLE('',#42383,38.5);
#8044=CIRCLE('',#42384,0.299999999999991);
#8045=CIRCLE('',#42386,0.300000000000002);
#8046=CIRCLE('',#42388,0.300000000000011);
#8047=CIRCLE('',#42392,0.3);
#8048=CIRCLE('',#42395,38.087867965644);
#8049=CIRCLE('',#42396,38.5);
#8050=CIRCLE('',#42398,0.3);
#8051=CIRCLE('',#42399,0.3);
#8052=CIRCLE('',#42400,0.299999999999999);
#8053=CIRCLE('',#42401,0.3);
#8054=CIRCLE('',#42403,0.299999999999994);
#8055=CIRCLE('',#42407,0.300000000000001);
#8056=CIRCLE('',#42409,0.3);
#8057=CIRCLE('',#42411,0.299999999999998);
#8058=CIRCLE('',#42413,0.299999999999998);
#8059=CIRCLE('',#42414,0.299999999999144);
#8060=CIRCLE('',#42416,0.3);
#8061=CIRCLE('',#42418,0.299999999999991);
#8062=CIRCLE('',#42420,0.3);
#8063=CIRCLE('',#42422,38.087867965644);
#8064=CIRCLE('',#42423,0.3);
#8065=CIRCLE('',#42425,38.4121320343559);
#8066=CIRCLE('',#42426,0.299999999999999);
#8067=CIRCLE('',#42427,0.299999999999996);
#8068=CIRCLE('',#42429,0.299999999999994);
#8069=CIRCLE('',#42433,0.299999999999999);
#8070=CIRCLE('',#42434,0.300000000000001);
#8071=CIRCLE('',#42436,38.5);
#8072=CIRCLE('',#42437,0.299999999999999);
#8073=CIRCLE('',#42439,0.299999999999998);
#8074=CIRCLE('',#42441,0.300000000000011);
#8075=CIRCLE('',#42445,0.3);
#8076=CIRCLE('',#42448,0.3);
#8077=CIRCLE('',#42450,0.299999999999994);
#8078=CIRCLE('',#42451,38.087867965644);
#8079=CIRCLE('',#42453,0.3);
#8080=CIRCLE('',#42456,0.3);
#8081=CIRCLE('',#42457,0.3);
#8082=CIRCLE('',#42460,38.087867965644);
#8083=CIRCLE('',#42464,0.3);
#8084=CIRCLE('',#42467,0.3);
#8085=CIRCLE('',#42469,38.087867965644);
#8086=CIRCLE('',#42473,38.087867965644);
#8087=CIRCLE('',#42477,0.3);
#8088=CIRCLE('',#42479,38.087867965644);
#8089=CIRCLE('',#42484,0.3);
#8090=CIRCLE('',#42486,38.087867965644);
#8091=CIRCLE('',#42490,0.3);
#8092=CIRCLE('',#42492,38.087867965644);
#8093=CIRCLE('',#42496,38.087867965644);
#8094=CIRCLE('',#42499,0.3);
#8095=CIRCLE('',#42500,0.3);
#8096=CIRCLE('',#42501,0.299999999999999);
#8097=CIRCLE('',#42503,0.3);
#8098=CIRCLE('',#42505,0.300000000000011);
#8099=CIRCLE('',#42512,38.087867965644);
#8100=CIRCLE('',#42516,38.087867965644);
#8101=CIRCLE('',#42520,0.3);
#8102=CIRCLE('',#42523,0.3);
#8103=CIRCLE('',#42525,38.087867965644);
#8104=CIRCLE('',#42527,0.3);
#8105=CIRCLE('',#42530,38.087867965644);
#8106=CIRCLE('',#42534,0.3);
#8107=CIRCLE('',#42536,38.087867965644);
#8108=CIRCLE('',#42541,0.3);
#8109=CIRCLE('',#42543,38.087867965644);
#8110=CIRCLE('',#42547,0.3);
#8111=CIRCLE('',#42549,38.087867965644);
#8112=CIRCLE('',#42553,38.087867965644);
#8113=CIRCLE('',#42556,0.3);
#8114=CIRCLE('',#42557,0.3);
#8115=CIRCLE('',#42558,0.300000000000002);
#8116=CIRCLE('',#42560,0.3);
#8117=CIRCLE('',#42562,0.300000000000011);
#8118=CIRCLE('',#42569,38.087867965644);
#8119=CIRCLE('',#42571,0.3);
#8120=CIRCLE('',#42574,38.087867965644);
#8121=CIRCLE('',#42578,0.3);
#8122=CIRCLE('',#42581,0.3);
#8123=CIRCLE('',#42583,38.087867965644);
#8124=CIRCLE('',#42587,38.087867965644);
#8125=CIRCLE('',#42591,0.3);
#8126=CIRCLE('',#42593,38.087867965644);
#8127=CIRCLE('',#42598,0.3);
#8128=CIRCLE('',#42600,38.087867965644);
#8129=CIRCLE('',#42604,0.3);
#8130=CIRCLE('',#42606,38.087867965644);
#8131=CIRCLE('',#42610,38.087867965644);
#8132=CIRCLE('',#42613,0.3);
#8133=CIRCLE('',#42614,0.3);
#8134=CIRCLE('',#42615,0.300000000000002);
#8135=CIRCLE('',#42617,0.3);
#8136=CIRCLE('',#42619,0.300000000000011);
#8137=CIRCLE('',#42626,38.087867965644);
#8138=CIRCLE('',#42630,38.087867965644);
#8139=CIRCLE('',#42633,0.3);
#8140=CIRCLE('',#42634,0.300000000000001);
#8141=CIRCLE('',#42635,0.300000000000005);
#8142=CIRCLE('',#42637,38.5);
#8143=CIRCLE('',#42638,0.299999999999995);
#8144=CIRCLE('',#42640,0.299999999999999);
#8145=CIRCLE('',#42642,0.300000000000011);
#8146=CIRCLE('',#42647,0.3);
#8147=CIRCLE('',#42649,0.3);
#8148=CIRCLE('',#42651,38.087867965644);
#8149=CIRCLE('',#42655,38.087867965644);
#8150=CIRCLE('',#42659,0.3);
#8151=CIRCLE('',#42661,38.087867965644);
#8152=CIRCLE('',#42664,0.3);
#8153=CIRCLE('',#42668,38.087867965644);
#8154=CIRCLE('',#42672,0.3);
#8155=CIRCLE('',#42674,0.3);
#8156=CIRCLE('',#42676,0.3);
#8157=CIRCLE('',#42677,0.299999999997756);
#8158=CIRCLE('',#42679,0.3);
#8159=CIRCLE('',#42681,0.299999999999997);
#8160=CIRCLE('',#42683,38.412132034356);
#8161=CIRCLE('',#42684,0.299999999999996);
#8162=CIRCLE('',#42685,38.5);
#8163=CIRCLE('',#42687,0.3);
#8164=CIRCLE('',#42689,0.3);
#8165=CIRCLE('',#42691,38.087867965644);
#8166=CIRCLE('',#42692,0.3);
#8167=CIRCLE('',#42694,38.412132034356);
#8168=CIRCLE('',#42696,38.5);
#8169=CIRCLE('',#42697,0.300000000000002);
#8170=CIRCLE('',#42700,0.3);
#8171=CIRCLE('',#42702,0.300000000000001);
#8172=CIRCLE('',#42705,0.3);
#8173=CIRCLE('',#42707,0.3);
#8174=CIRCLE('',#42708,0.29999999999775);
#8175=CIRCLE('',#42710,0.3);
#8176=CIRCLE('',#42712,38.412132034356);
#8177=CIRCLE('',#42713,0.299999999999999);
#8178=CIRCLE('',#42714,38.5);
#8179=CIRCLE('',#42716,0.299999999999997);
#8180=CIRCLE('',#42718,0.3);
#8181=CIRCLE('',#42719,0.3);
#8182=CIRCLE('',#42720,0.299999999998153);
#8183=CIRCLE('',#42722,0.3);
#8184=CIRCLE('',#42724,0.3);
#8185=CIRCLE('',#42726,38.5);
#8186=CIRCLE('',#42728,0.3);
#8187=CIRCLE('',#42730,0.3);
#8188=CIRCLE('',#42732,38.087867965644);
#8189=CIRCLE('',#42735,38.087867965644);
#8190=CIRCLE('',#42736,0.300000000000002);
#8191=CIRCLE('',#42738,0.299999999999997);
#8192=CIRCLE('',#42739,38.412132034356);
#8193=CIRCLE('',#42743,0.3);
#8194=CIRCLE('',#42744,0.3);
#8195=CIRCLE('',#42745,0.299999999999999);
#8196=CIRCLE('',#42747,0.299999999999994);
#8197=CIRCLE('',#42752,33.);
#8198=CIRCLE('',#42753,33.);
#8199=CIRCLE('',#42754,0.3);
#8200=CIRCLE('',#42756,33.);
#8201=CIRCLE('',#42757,33.);
#8202=CIRCLE('',#42759,38.087867965644);
#8203=CIRCLE('',#42760,0.300000000000004);
#8204=CIRCLE('',#42762,0.300000000000001);
#8205=CIRCLE('',#42763,38.4121320343559);
#8206=CIRCLE('',#42766,38.087867965644);
#8207=CIRCLE('',#42767,0.300000000000002);
#8208=CIRCLE('',#42769,0.299999999999993);
#8209=CIRCLE('',#42770,38.412132034356);
#8210=CIRCLE('',#42779,0.3);
#8211=CIRCLE('',#42781,0.3);
#8212=CIRCLE('',#42785,0.3);
#8213=CIRCLE('',#42787,0.3);
#8214=CIRCLE('',#42793,38.087867965644);
#8215=CIRCLE('',#42797,0.3);
#8216=CIRCLE('',#42803,38.087867965644);
#8217=CIRCLE('',#42811,38.087867965644);
#8218=CIRCLE('',#42820,38.087867965644);
#8219=CIRCLE('',#42828,38.087867965644);
#8220=CIRCLE('',#42836,38.087867965644);
#8221=CIRCLE('',#42844,38.087867965644);
#8222=CIRCLE('',#42853,38.087867965644);
#8223=CIRCLE('',#42861,38.087867965644);
#8224=CIRCLE('',#42865,0.3);
#8225=CIRCLE('',#42871,38.087867965644);
#8226=CIRCLE('',#42880,38.087867965644);
#8227=CIRCLE('',#42888,38.087867965644);
#8228=CIRCLE('',#42896,38.087867965644);
#8229=CIRCLE('',#42900,0.3);
#8230=CIRCLE('',#42906,38.087867965644);
#8231=CIRCLE('',#42914,38.087867965644);
#8232=CIRCLE('',#42918,0.3);
#8233=CIRCLE('',#42919,0.3);
#8234=CIRCLE('',#42925,38.5);
#8235=CIRCLE('',#42928,38.5);
#8236=CIRCLE('',#42933,38.5);
#8237=CIRCLE('',#42938,38.5);
#8238=CIRCLE('',#42946,38.5);
#8239=CIRCLE('',#42951,38.5);
#8240=CIRCLE('',#42956,38.5);
#8241=CIRCLE('',#42964,38.5);
#8242=CIRCLE('',#42969,38.5);
#8243=CIRCLE('',#42974,38.5);
#8244=CIRCLE('',#42982,38.5);
#8245=CIRCLE('',#42987,38.5);
#8246=CIRCLE('',#42992,38.5);
#9674=B_SPLINE_CURVE_WITH_KNOTS('',3,(#68050,#68051,#68052,#68053),
 .UNSPECIFIED.,.F.,.F.,(4,4),(-0.0458781805670868,0.),.UNSPECIFIED.);
#9675=B_SPLINE_CURVE_WITH_KNOTS('',3,(#68055,#68056,#68057,#68058),
 .UNSPECIFIED.,.F.,.F.,(4,4),(0.,0.0458781805670868),.UNSPECIFIED.);
#9676=B_SPLINE_CURVE_WITH_KNOTS('',3,(#68078,#68079,#68080,#68081,#68082,
#68083,#68084,#68085),.UNSPECIFIED.,.F.,.F.,(4,2,2,4),(-0.000347076601499395,
0.,0.0153026771616971,0.0323450549295143),.UNSPECIFIED.);
#9677=B_SPLINE_CURVE_WITH_KNOTS('',3,(#68092,#68093,#68094,#68095,#68096,
#68097,#68098,#68099,#68100,#68101),.UNSPECIFIED.,.F.,.F.,(4,2,2,2,4),(-0.112045606680405,
-0.110611693715149,-0.0954349222053129,-0.0802581506954765,-0.0802157928231075),
 .UNSPECIFIED.);
#9678=B_SPLINE_CURVE_WITH_KNOTS('',3,(#68125,#68126,#68127,#68128),
 .UNSPECIFIED.,.F.,.F.,(4,4),(-0.0458781805664131,0.),.UNSPECIFIED.);
#9679=B_SPLINE_CURVE_WITH_KNOTS('',3,(#68130,#68131,#68132,#68133),
 .UNSPECIFIED.,.F.,.F.,(4,4),(0.,0.0458781805664131),.UNSPECIFIED.);
#9680=B_SPLINE_CURVE_WITH_KNOTS('',3,(#68148,#68149,#68150,#68151,#68152,
#68153),.UNSPECIFIED.,.F.,.F.,(4,2,4),(0.0222170009937288,0.0333260526322424,
0.044441887561283),.UNSPECIFIED.);
#9681=B_SPLINE_CURVE_WITH_KNOTS('',3,(#68449,#68450,#68451,#68452,#68453,
#68454,#68455,#68456,#68457,#68458,#68459,#68460,#68461,#68462,#68463,#68464,
#68465,#68466,#68467),.UNSPECIFIED.,.F.,.F.,(4,3,3,3,3,3,4),(0.,0.00744324341952001,
0.0150897391630985,0.0227304222580373,0.029965145148507,0.0341762641937729,
0.0347332983695568),.UNSPECIFIED.);
#9682=B_SPLINE_CURVE_WITH_KNOTS('',3,(#68477,#68478,#68479,#68480,#68481,
#68482,#68483,#68484,#68485,#68486,#68487,#68488,#68489,#68490,#68491,#68492,
#68493,#68494,#68495),.UNSPECIFIED.,.F.,.F.,(4,3,3,3,3,3,4),(0.,0.00744322147100868,
0.0150897242479162,0.0227304222579707,0.0299651530525656,0.0341762641937285,
0.0347332983695172),.UNSPECIFIED.);
#9683=B_SPLINE_CURVE_WITH_KNOTS('',3,(#68505,#68506,#68507,#68508,#68509,
#68510,#68511,#68512,#68513,#68514,#68515,#68516,#68517,#68518,#68519,#68520,
#68521,#68522,#68523),.UNSPECIFIED.,.F.,.F.,(4,3,3,3,3,3,4),(0.,0.00744320435370726,
0.0150897126157594,0.0227304222579515,0.0299651592168987,0.0341762641936531,
0.034733298369438),.UNSPECIFIED.);
#9684=B_SPLINE_CURVE_WITH_KNOTS('',3,(#68606,#68607,#68608,#68609),
 .UNSPECIFIED.,.F.,.F.,(4,4),(-0.045878180566409,0.),.UNSPECIFIED.);
#9685=B_SPLINE_CURVE_WITH_KNOTS('',3,(#68646,#68647,#68648,#68649),
 .UNSPECIFIED.,.F.,.F.,(4,4),(-0.0458781805670811,0.),.UNSPECIFIED.);
#9686=B_SPLINE_CURVE_WITH_KNOTS('',3,(#68651,#68652,#68653,#68654),
 .UNSPECIFIED.,.F.,.F.,(4,4),(0.,0.0458781805670811),.UNSPECIFIED.);
#9687=B_SPLINE_CURVE_WITH_KNOTS('',3,(#68674,#68675,#68676,#68677,#68678,
#68679,#68680,#68681),.UNSPECIFIED.,.F.,.F.,(4,2,2,4),(-0.0003470766014915,
0.,0.0153026771616932,0.0323450549295876),.UNSPECIFIED.);
#9688=B_SPLINE_CURVE_WITH_KNOTS('',3,(#68688,#68689,#68690,#68691,#68692,
#68693,#68694,#68695,#68696,#68697),.UNSPECIFIED.,.F.,.F.,(4,2,2,2,4),(-0.112045606680405,
-0.110611693715149,-0.0954349222053128,-0.0802581506954763,-0.0802157928231085),
 .UNSPECIFIED.);
#9689=B_SPLINE_CURVE_WITH_KNOTS('',3,(#68721,#68722,#68723,#68724),
 .UNSPECIFIED.,.F.,.F.,(4,4),(-0.0458781805664166,0.),.UNSPECIFIED.);
#9690=B_SPLINE_CURVE_WITH_KNOTS('',3,(#68726,#68727,#68728,#68729),
 .UNSPECIFIED.,.F.,.F.,(4,4),(0.,0.0458781805664166),.UNSPECIFIED.);
#9691=B_SPLINE_CURVE_WITH_KNOTS('',3,(#68744,#68745,#68746,#68747,#68748,
#68749),.UNSPECIFIED.,.F.,.F.,(4,2,4),(0.0222170009937291,0.0333260526322424,
0.044441887561283),.UNSPECIFIED.);
#9692=B_SPLINE_CURVE_WITH_KNOTS('',3,(#68758,#68759,#68760,#68761),
 .UNSPECIFIED.,.F.,.F.,(4,4),(-0.0458781805664144,0.),.UNSPECIFIED.);
#9693=B_SPLINE_CURVE_WITH_KNOTS('',3,(#68798,#68799,#68800,#68801),
 .UNSPECIFIED.,.F.,.F.,(4,4),(-0.0458781805670864,0.),.UNSPECIFIED.);
#9694=B_SPLINE_CURVE_WITH_KNOTS('',3,(#68803,#68804,#68805,#68806),
 .UNSPECIFIED.,.F.,.F.,(4,4),(0.,0.0458781805670864),.UNSPECIFIED.);
#9695=B_SPLINE_CURVE_WITH_KNOTS('',3,(#68826,#68827,#68828,#68829,#68830,
#68831,#68832,#68833),.UNSPECIFIED.,.F.,.F.,(4,2,2,4),(-0.000347076601484255,
0.,0.0153026771616858,0.0323450549293956),.UNSPECIFIED.);
#9696=B_SPLINE_CURVE_WITH_KNOTS('',3,(#68840,#68841,#68842,#68843,#68844,
#68845,#68846,#68847,#68848,#68849),.UNSPECIFIED.,.F.,.F.,(4,2,2,2,4),(-0.112045606680405,
-0.110611693715151,-0.0954349222053137,-0.0802581506954766,-0.0802157928231077),
 .UNSPECIFIED.);
#9697=B_SPLINE_CURVE_WITH_KNOTS('',3,(#68873,#68874,#68875,#68876),
 .UNSPECIFIED.,.F.,.F.,(4,4),(-0.0458781805664115,0.),.UNSPECIFIED.);
#9698=B_SPLINE_CURVE_WITH_KNOTS('',3,(#68878,#68879,#68880,#68881),
 .UNSPECIFIED.,.F.,.F.,(4,4),(0.,0.0458781805664115),.UNSPECIFIED.);
#9699=B_SPLINE_CURVE_WITH_KNOTS('',3,(#68896,#68897,#68898,#68899,#68900,
#68901),.UNSPECIFIED.,.F.,.F.,(4,2,4),(0.0222170009937291,0.0333260526322424,
0.044441887561283),.UNSPECIFIED.);
#9700=B_SPLINE_CURVE_WITH_KNOTS('',3,(#68910,#68911,#68912,#68913),
 .UNSPECIFIED.,.F.,.F.,(4,4),(-0.045878180566409,0.),.UNSPECIFIED.);
#9701=B_SPLINE_CURVE_WITH_KNOTS('',3,(#68953,#68954,#68955,#68956),
 .UNSPECIFIED.,.F.,.F.,(4,4),(-0.0458781805671252,0.),.UNSPECIFIED.);
#9702=B_SPLINE_CURVE_WITH_KNOTS('',3,(#68958,#68959,#68960,#68961),
 .UNSPECIFIED.,.F.,.F.,(4,4),(0.,0.0458781805671252),.UNSPECIFIED.);
#9703=B_SPLINE_CURVE_WITH_KNOTS('',3,(#68972,#68973,#68974,#68975,#68976,
#68977,#68978,#68979),.UNSPECIFIED.,.F.,.F.,(4,2,2,4),(-0.000347076601650634,
0.,0.0153026771616405,0.0323450549291064),.UNSPECIFIED.);
#9704=B_SPLINE_CURVE_WITH_KNOTS('',3,(#68986,#68987,#68988,#68989,#68990,
#68991,#68992,#68993,#68994,#68995),.UNSPECIFIED.,.F.,.F.,(4,2,2,2,4),(0.108010287307677,
0.109444200272932,0.124620971782768,0.139797743292604,0.139840101164974),
 .UNSPECIFIED.);
#9705=B_SPLINE_CURVE_WITH_KNOTS('',3,(#69027,#69028,#69029,#69030),
 .UNSPECIFIED.,.F.,.F.,(4,4),(-0.0458781805667822,0.),.UNSPECIFIED.);
#9706=B_SPLINE_CURVE_WITH_KNOTS('',3,(#69032,#69033,#69034,#69035),
 .UNSPECIFIED.,.F.,.F.,(4,4),(0.,0.0458781805667822),.UNSPECIFIED.);
#9707=B_SPLINE_CURVE_WITH_KNOTS('',3,(#69049,#69050,#69051,#69052),
 .UNSPECIFIED.,.F.,.F.,(4,4),(-0.0458781805667811,0.),.UNSPECIFIED.);
#9708=B_SPLINE_CURVE_WITH_KNOTS('',3,(#69068,#69069,#69070,#69071),
 .UNSPECIFIED.,.F.,.F.,(4,4),(0.,0.0458781805667811),.UNSPECIFIED.);
#9709=B_SPLINE_CURVE_WITH_KNOTS('',3,(#69105,#69106,#69107,#69108),
 .UNSPECIFIED.,.F.,.F.,(4,4),(-0.0458781805671229,0.),.UNSPECIFIED.);
#9710=B_SPLINE_CURVE_WITH_KNOTS('',3,(#69110,#69111,#69112,#69113),
 .UNSPECIFIED.,.F.,.F.,(4,4),(0.,0.0458781805671229),.UNSPECIFIED.);
#9711=B_SPLINE_CURVE_WITH_KNOTS('',3,(#69124,#69125,#69126,#69127,#69128,
#69129,#69130,#69131),.UNSPECIFIED.,.F.,.F.,(4,2,2,4),(-0.000347076601706745,
0.,0.0153026771616907,0.0323450549295787),.UNSPECIFIED.);
#9712=B_SPLINE_CURVE_WITH_KNOTS('',3,(#69138,#69139,#69140,#69141,#69142,
#69143,#69144,#69145,#69146,#69147),.UNSPECIFIED.,.F.,.F.,(4,2,2,2,4),(0.108010287307677,
0.109444200272933,0.124620971782769,0.139797743292606,0.139840101164975),
 .UNSPECIFIED.);
#9713=B_SPLINE_CURVE_WITH_KNOTS('',3,(#69179,#69180,#69181,#69182),
 .UNSPECIFIED.,.F.,.F.,(4,4),(-0.0458781805667724,0.),.UNSPECIFIED.);
#9714=B_SPLINE_CURVE_WITH_KNOTS('',3,(#69184,#69185,#69186,#69187),
 .UNSPECIFIED.,.F.,.F.,(4,4),(0.,0.0458781805667724),.UNSPECIFIED.);
#9715=B_SPLINE_CURVE_WITH_KNOTS('',3,(#69201,#69202,#69203,#69204),
 .UNSPECIFIED.,.F.,.F.,(4,4),(-0.0458781805667679,0.),.UNSPECIFIED.);
#9716=B_SPLINE_CURVE_WITH_KNOTS('',3,(#69220,#69221,#69222,#69223),
 .UNSPECIFIED.,.F.,.F.,(4,4),(0.,0.0458781805667679),.UNSPECIFIED.);
#9717=B_SPLINE_CURVE_WITH_KNOTS('',3,(#69257,#69258,#69259,#69260),
 .UNSPECIFIED.,.F.,.F.,(4,4),(-0.045878180567128,0.),.UNSPECIFIED.);
#9718=B_SPLINE_CURVE_WITH_KNOTS('',3,(#69262,#69263,#69264,#69265),
 .UNSPECIFIED.,.F.,.F.,(4,4),(0.,0.045878180567128),.UNSPECIFIED.);
#9719=B_SPLINE_CURVE_WITH_KNOTS('',3,(#69271,#69272,#69273,#69274,#69275,
#69276,#69277,#69278,#69279,#69280,#69281,#69282,#69283,#69284),
 .UNSPECIFIED.,.F.,.F.,(4,2,2,2,2,2,4),(-0.112045619239962,-0.110611693715148,
-0.0954349222053123,-0.0802581506954765,-0.0677819987765255,-0.06154392281705,
-0.0553058468575746),.UNSPECIFIED.);
#9720=B_SPLINE_CURVE_WITH_KNOTS('',3,(#69654,#69655,#69656,#69657),
 .UNSPECIFIED.,.F.,.F.,(4,4),(-0.0458781805667874,0.),.UNSPECIFIED.);
#9721=B_SPLINE_CURVE_WITH_KNOTS('',3,(#69696,#69697,#69698,#69699),
 .UNSPECIFIED.,.F.,.F.,(4,4),(-0.0458781805671024,0.),.UNSPECIFIED.);
#9722=B_SPLINE_CURVE_WITH_KNOTS('',3,(#69701,#69702,#69703,#69704),
 .UNSPECIFIED.,.F.,.F.,(4,4),(0.,0.0458781805671024),.UNSPECIFIED.);
#9723=B_SPLINE_CURVE_WITH_KNOTS('',3,(#69710,#69711,#69712,#69713,#69714,
#69715,#69716,#69717,#69718,#69719,#69720,#69721,#69722,#69723),
 .UNSPECIFIED.,.F.,.F.,(4,2,2,2,2,2,4),(-0.11204561923996,-0.110611693715148,
-0.0954349222053124,-0.0802581506954765,-0.0677819987765257,-0.0615439228170502,
-0.0553058468575748),.UNSPECIFIED.);
#9724=B_SPLINE_CURVE_WITH_KNOTS('',3,(#69737,#69738,#69739,#69740),
 .UNSPECIFIED.,.F.,.F.,(4,4),(-0.0458781805665695,0.),.UNSPECIFIED.);
#9725=B_SPLINE_CURVE_WITH_KNOTS('',3,(#69779,#69780,#69781,#69782),
 .UNSPECIFIED.,.F.,.F.,(4,4),(-0.0458781805671248,0.),.UNSPECIFIED.);
#9726=B_SPLINE_CURVE_WITH_KNOTS('',3,(#69784,#69785,#69786,#69787),
 .UNSPECIFIED.,.F.,.F.,(4,4),(0.,0.0458781805671248),.UNSPECIFIED.);
#9727=B_SPLINE_CURVE_WITH_KNOTS('',3,(#69793,#69794,#69795,#69796,#69797,
#69798,#69799,#69800,#69801,#69802,#69803,#69804,#69805,#69806),
 .UNSPECIFIED.,.F.,.F.,(4,2,2,2,2,2,4),(-0.112045619239959,-0.110611693715147,
-0.0954349222053113,-0.0802581506954755,-0.0677819987765242,-0.0615439228170485,
-0.0553058468575729),.UNSPECIFIED.);
#9728=B_SPLINE_CURVE_WITH_KNOTS('',3,(#69820,#69821,#69822,#69823),
 .UNSPECIFIED.,.F.,.F.,(4,4),(-0.0458781805667828,0.),.UNSPECIFIED.);
#9729=B_SPLINE_CURVE_WITH_KNOTS('',3,(#69868,#69869,#69870,#69871),
 .UNSPECIFIED.,.F.,.F.,(4,4),(-0.0458781805671046,0.),.UNSPECIFIED.);
#9730=B_SPLINE_CURVE_WITH_KNOTS('',3,(#69873,#69874,#69875,#69876),
 .UNSPECIFIED.,.F.,.F.,(4,4),(0.,0.0458781805671046),.UNSPECIFIED.);
#9731=B_SPLINE_CURVE_WITH_KNOTS('',3,(#69887,#69888,#69889,#69890,#69891,
#69892,#69893,#69894),.UNSPECIFIED.,.F.,.F.,(4,2,2,4),(-0.000347076601642684,
0.,0.0153026771617058,0.032345054929432),.UNSPECIFIED.);
#9732=B_SPLINE_CURVE_WITH_KNOTS('',3,(#69901,#69902,#69903,#69904,#69905,
#69906,#69907,#69908,#69909,#69910),.UNSPECIFIED.,.F.,.F.,(4,2,2,2,4),(-0.112045606680404,
-0.110611693715149,-0.0954349222053132,-0.0802581506954773,-0.080215792823107),
 .UNSPECIFIED.);
#9733=B_SPLINE_CURVE_WITH_KNOTS('',3,(#69936,#69937,#69938,#69939),
 .UNSPECIFIED.,.F.,.F.,(4,4),(-0.0458781805666752,0.),.UNSPECIFIED.);
#9734=B_SPLINE_CURVE_WITH_KNOTS('',3,(#69941,#69942,#69943,#69944),
 .UNSPECIFIED.,.F.,.F.,(4,4),(0.,0.0458781805666752),.UNSPECIFIED.);
#9735=B_SPLINE_CURVE_WITH_KNOTS('',3,(#69961,#69962,#69963,#69964),
 .UNSPECIFIED.,.F.,.F.,(4,4),(0.,0.0883236961657995),.UNSPECIFIED.);
#9736=B_SPLINE_CURVE_WITH_KNOTS('',3,(#69968,#69969,#69970,#69971,#69972,
#69973),.UNSPECIFIED.,.F.,.F.,(4,2,4),(0.0222170009937305,0.0333260526322425,
0.0444418875612832),.UNSPECIFIED.);
#9737=B_SPLINE_CURVE_WITH_KNOTS('',3,(#70006,#70007,#70008,#70009),
 .UNSPECIFIED.,.F.,.F.,(4,4),(-0.0458781805671212,0.),.UNSPECIFIED.);
#9738=B_SPLINE_CURVE_WITH_KNOTS('',3,(#70011,#70012,#70013,#70014),
 .UNSPECIFIED.,.F.,.F.,(4,4),(0.,0.0458781805671212),.UNSPECIFIED.);
#9739=B_SPLINE_CURVE_WITH_KNOTS('',3,(#70020,#70021,#70022,#70023,#70024,
#70025,#70026,#70027,#70028,#70029,#70030,#70031,#70032,#70033),
 .UNSPECIFIED.,.F.,.F.,(4,2,2,2,2,2,4),(-0.112045619239959,-0.110611693715147,
-0.0954349222053112,-0.0802581506954752,-0.0677819987765244,-0.0615439228170491,
-0.0553058468575737),.UNSPECIFIED.);
#9740=B_SPLINE_CURVE_WITH_KNOTS('',3,(#70047,#70048,#70049,#70050),
 .UNSPECIFIED.,.F.,.F.,(4,4),(-0.0458781805667679,0.),.UNSPECIFIED.);
#9741=B_SPLINE_CURVE_WITH_KNOTS('',3,(#70089,#70090,#70091,#70092),
 .UNSPECIFIED.,.F.,.F.,(4,4),(-0.0458781805671206,0.),.UNSPECIFIED.);
#9742=B_SPLINE_CURVE_WITH_KNOTS('',3,(#70094,#70095,#70096,#70097),
 .UNSPECIFIED.,.F.,.F.,(4,4),(0.,0.0458781805671206),.UNSPECIFIED.);
#9743=B_SPLINE_CURVE_WITH_KNOTS('',3,(#70103,#70104,#70105,#70106,#70107,
#70108,#70109,#70110,#70111,#70112,#70113,#70114,#70115,#70116),
 .UNSPECIFIED.,.F.,.F.,(4,2,2,2,2,2,4),(-0.112045619239963,-0.110611693715148,
-0.0954349222053121,-0.0802581506954761,-0.0677819987765253,-0.0615439228170498,
-0.0553058468575744),.UNSPECIFIED.);
#9744=B_SPLINE_CURVE_WITH_KNOTS('',3,(#70130,#70131,#70132,#70133),
 .UNSPECIFIED.,.F.,.F.,(4,4),(-0.045878180566734,0.),.UNSPECIFIED.);
#9745=B_SPLINE_CURVE_WITH_KNOTS('',3,(#70172,#70173,#70174,#70175),
 .UNSPECIFIED.,.F.,.F.,(4,4),(-0.0458781805671124,0.),.UNSPECIFIED.);
#9746=B_SPLINE_CURVE_WITH_KNOTS('',3,(#70177,#70178,#70179,#70180),
 .UNSPECIFIED.,.F.,.F.,(4,4),(0.,0.0458781805671124),.UNSPECIFIED.);
#9747=B_SPLINE_CURVE_WITH_KNOTS('',3,(#70186,#70187,#70188,#70189,#70190,
#70191,#70192,#70193,#70194,#70195,#70196,#70197,#70198,#70199),
 .UNSPECIFIED.,.F.,.F.,(4,2,2,2,2,2,4),(-0.11204561923996,-0.110611693715147,
-0.095434922205311,-0.080258150695475,-0.0677819987765241,-0.0615439228170487,
-0.0553058468575733),.UNSPECIFIED.);
#9748=B_SPLINE_CURVE_WITH_KNOTS('',3,(#70213,#70214,#70215,#70216),
 .UNSPECIFIED.,.F.,.F.,(4,4),(-0.0458781805667346,0.),.UNSPECIFIED.);
#9749=B_SPLINE_CURVE_WITH_KNOTS('',3,(#70253,#70254,#70255,#70256),
 .UNSPECIFIED.,.F.,.F.,(4,4),(-0.0458781805670977,0.),.UNSPECIFIED.);
#9750=B_SPLINE_CURVE_WITH_KNOTS('',3,(#70258,#70259,#70260,#70261),
 .UNSPECIFIED.,.F.,.F.,(4,4),(0.,0.0458781805670977),.UNSPECIFIED.);
#9751=B_SPLINE_CURVE_WITH_KNOTS('',3,(#70272,#70273,#70274,#70275,#70276,
#70277,#70278,#70279),.UNSPECIFIED.,.F.,.F.,(4,2,2,4),(-0.000347076601612338,
0.,0.0153026771617837,0.0323450549295477),.UNSPECIFIED.);
#9752=B_SPLINE_CURVE_WITH_KNOTS('',3,(#70286,#70287,#70288,#70289,#70290,
#70291,#70292,#70293,#70294,#70295),.UNSPECIFIED.,.F.,.F.,(4,2,2,2,4),(-0.112045606680404,
-0.110611693715149,-0.0954349222053116,-0.0802581506954743,-0.0802157928231058),
 .UNSPECIFIED.);
#9753=B_SPLINE_CURVE_WITH_KNOTS('',3,(#70321,#70322,#70323,#70324),
 .UNSPECIFIED.,.F.,.F.,(4,4),(-0.0458781805665702,0.),.UNSPECIFIED.);
#9754=B_SPLINE_CURVE_WITH_KNOTS('',3,(#70326,#70327,#70328,#70329),
 .UNSPECIFIED.,.F.,.F.,(4,4),(0.,0.0458781805665702),.UNSPECIFIED.);
#9755=B_SPLINE_CURVE_WITH_KNOTS('',3,(#70346,#70347,#70348,#70349),
 .UNSPECIFIED.,.F.,.F.,(4,4),(0.,0.0883236961657975),.UNSPECIFIED.);
#9756=B_SPLINE_CURVE_WITH_KNOTS('',3,(#70353,#70354,#70355,#70356,#70357,
#70358),.UNSPECIFIED.,.F.,.F.,(4,2,4),(0.0222170009937299,0.033326052632243,
0.0444418875612829),.UNSPECIFIED.);
#9757=B_SPLINE_CURVE_WITH_KNOTS('',3,(#70385,#70386,#70387,#70388),
 .UNSPECIFIED.,.F.,.F.,(4,4),(0.,0.0458781805667346),.UNSPECIFIED.);
#9758=B_SPLINE_CURVE_WITH_KNOTS('',3,(#70406,#70407,#70408,#70409,#70410,
#70411),.UNSPECIFIED.,.F.,.F.,(4,2,4),(0.0222170009937297,0.0333260526322424,
0.0444418875612829),.UNSPECIFIED.);
#9759=B_SPLINE_CURVE_WITH_KNOTS('',3,(#70437,#70438,#70439,#70440),
 .UNSPECIFIED.,.F.,.F.,(4,4),(0.,0.045878180566734),.UNSPECIFIED.);
#9760=B_SPLINE_CURVE_WITH_KNOTS('',3,(#70454,#70455,#70456,#70457,#70458,
#70459),.UNSPECIFIED.,.F.,.F.,(4,2,4),(0.0222170009937345,0.0333260526322431,
0.0444418875612845),.UNSPECIFIED.);
#9761=B_SPLINE_CURVE_WITH_KNOTS('',3,(#70491,#70492,#70493,#70494),
 .UNSPECIFIED.,.F.,.F.,(4,4),(-0.0458781805670993,0.),.UNSPECIFIED.);
#9762=B_SPLINE_CURVE_WITH_KNOTS('',3,(#70496,#70497,#70498,#70499),
 .UNSPECIFIED.,.F.,.F.,(4,4),(0.,0.0458781805670993),.UNSPECIFIED.);
#9763=B_SPLINE_CURVE_WITH_KNOTS('',3,(#70505,#70506,#70507,#70508,#70509,
#70510,#70511,#70512,#70513,#70514,#70515,#70516,#70517,#70518),
 .UNSPECIFIED.,.F.,.F.,(4,2,2,2,2,2,4),(-0.112045619239962,-0.110611693715147,
-0.0954349222053112,-0.0802581506954753,-0.0677819987765244,-0.061543922817049,
-0.0553058468575735),.UNSPECIFIED.);
#9764=B_SPLINE_CURVE_WITH_KNOTS('',3,(#70532,#70533,#70534,#70535),
 .UNSPECIFIED.,.F.,.F.,(4,4),(-0.0458781805665721,0.),.UNSPECIFIED.);
#9765=B_SPLINE_CURVE_WITH_KNOTS('',3,(#70568,#70569,#70570,#70571),
 .UNSPECIFIED.,.F.,.F.,(4,4),(0.,0.0458781805667679),.UNSPECIFIED.);
#9766=B_SPLINE_CURVE_WITH_KNOTS('',3,(#70585,#70586,#70587,#70588,#70589,
#70590),.UNSPECIFIED.,.F.,.F.,(4,2,4),(0.0222170009937316,0.0333260526322429,
0.0444418875612838),.UNSPECIFIED.);
#9767=B_SPLINE_CURVE_WITH_KNOTS('',3,(#70622,#70623,#70624,#70625),
 .UNSPECIFIED.,.F.,.F.,(4,4),(-0.0458781805671254,0.),.UNSPECIFIED.);
#9768=B_SPLINE_CURVE_WITH_KNOTS('',3,(#70627,#70628,#70629,#70630),
 .UNSPECIFIED.,.F.,.F.,(4,4),(0.,0.0458781805671254),.UNSPECIFIED.);
#9769=B_SPLINE_CURVE_WITH_KNOTS('',3,(#70636,#70637,#70638,#70639,#70640,
#70641,#70642,#70643,#70644,#70645,#70646,#70647,#70648,#70649),
 .UNSPECIFIED.,.F.,.F.,(4,2,2,2,2,2,4),(-0.11204561923996,-0.110611693715148,
-0.095434922205312,-0.0802581506954755,-0.0677819987765242,-0.0615439228170485,
-0.0553058468575728),.UNSPECIFIED.);
#9770=B_SPLINE_CURVE_WITH_KNOTS('',3,(#70663,#70664,#70665,#70666),
 .UNSPECIFIED.,.F.,.F.,(4,4),(-0.04587818056678,0.),.UNSPECIFIED.);
#9771=B_SPLINE_CURVE_WITH_KNOTS('',3,(#70691,#70692,#70693,#70694),
 .UNSPECIFIED.,.F.,.F.,(4,4),(0.,0.0458781805667828),.UNSPECIFIED.);
#9772=B_SPLINE_CURVE_WITH_KNOTS('',3,(#70705,#70706,#70707,#70708,#70709,
#70710,#70711,#70712,#70713,#70714,#70715,#70716,#70717,#70718),
 .UNSPECIFIED.,.F.,.F.,(4,2,2,2,2,2,4),(0.0553058468575743,0.0615439228170501,
0.0677819987765258,0.0802581506954773,0.0954349222053131,0.110611693715149,
0.112045606679733),.UNSPECIFIED.);
#9773=B_SPLINE_CURVE_WITH_KNOTS('',3,(#70723,#70724,#70725,#70726,#70727,
#70728),.UNSPECIFIED.,.F.,.F.,(4,2,4),(0.133326015406808,0.144441850335849,
0.155550901974358),.UNSPECIFIED.);
#9774=B_SPLINE_CURVE_WITH_KNOTS('',3,(#70756,#70757,#70758,#70759),
 .UNSPECIFIED.,.F.,.F.,(4,4),(0.,0.04587818056678),.UNSPECIFIED.);
#9775=B_SPLINE_CURVE_WITH_KNOTS('',3,(#70777,#70778,#70779,#70780,#70781,
#70782),.UNSPECIFIED.,.F.,.F.,(4,2,4),(0.0222170009937285,0.0333260526322418,
0.0444418875612829),.UNSPECIFIED.);
#9776=B_SPLINE_CURVE_WITH_KNOTS('',3,(#70786,#70787,#70788,#70789,#70790,
#70791,#70792,#70793,#70794,#70795,#70796,#70797,#70798,#70799),
 .UNSPECIFIED.,.F.,.F.,(4,2,2,2,2,2,4),(0.0553058468575751,0.0615439228170508,
0.0677819987765264,0.0802581506954776,0.0954349222053136,0.11061169371515,
0.112045606679733),.UNSPECIFIED.);
#9777=B_SPLINE_CURVE_WITH_KNOTS('',3,(#70804,#70805,#70806,#70807,#70808,
#70809),.UNSPECIFIED.,.F.,.F.,(4,2,4),(0.133326015406808,0.14444185033585,
0.15555090197436),.UNSPECIFIED.);
#9778=B_SPLINE_CURVE_WITH_KNOTS('',3,(#70843,#70844,#70845,#70846),
 .UNSPECIFIED.,.F.,.F.,(4,4),(-0.0458781805671173,0.),.UNSPECIFIED.);
#9779=B_SPLINE_CURVE_WITH_KNOTS('',3,(#70848,#70849,#70850,#70851),
 .UNSPECIFIED.,.F.,.F.,(4,4),(0.,0.0458781805671173),.UNSPECIFIED.);
#9780=B_SPLINE_CURVE_WITH_KNOTS('',3,(#70857,#70858,#70859,#70860,#70861,
#70862,#70863,#70864,#70865,#70866,#70867,#70868,#70869,#70870),
 .UNSPECIFIED.,.F.,.F.,(4,2,2,2,2,2,4),(-0.112045619239959,-0.110611693715147,
-0.0954349222053107,-0.0802581506954748,-0.067781998776524,-0.0615439228170486,
-0.0553058468575732),.UNSPECIFIED.);
#9781=B_SPLINE_CURVE_WITH_KNOTS('',3,(#70884,#70885,#70886,#70887),
 .UNSPECIFIED.,.F.,.F.,(4,4),(-0.0458781805665586,0.),.UNSPECIFIED.);
#9782=B_SPLINE_CURVE_WITH_KNOTS('',3,(#70918,#70919,#70920,#70921),
 .UNSPECIFIED.,.F.,.F.,(4,4),(-0.0458781805671103,0.),.UNSPECIFIED.);
#9783=B_SPLINE_CURVE_WITH_KNOTS('',3,(#70923,#70924,#70925,#70926),
 .UNSPECIFIED.,.F.,.F.,(4,4),(0.,0.0458781805671103),.UNSPECIFIED.);
#9784=B_SPLINE_CURVE_WITH_KNOTS('',3,(#70932,#70933,#70934,#70935,#70936,
#70937,#70938,#70939,#70940,#70941,#70942,#70943,#70944,#70945),
 .UNSPECIFIED.,.F.,.F.,(4,2,2,2,2,2,4),(-0.112045619239963,-0.11061169371515,
-0.0954349222053134,-0.0802581506954769,-0.0677819987765259,-0.0615439228170504,
-0.0553058468575749),.UNSPECIFIED.);
#9785=B_SPLINE_CURVE_WITH_KNOTS('',3,(#70959,#70960,#70961,#70962),
 .UNSPECIFIED.,.F.,.F.,(4,4),(-0.045878180566425,0.),.UNSPECIFIED.);
#9786=B_SPLINE_CURVE_WITH_KNOTS('',3,(#71001,#71002,#71003,#71004),
 .UNSPECIFIED.,.F.,.F.,(4,4),(-0.0458781805671206,0.),.UNSPECIFIED.);
#9787=B_SPLINE_CURVE_WITH_KNOTS('',3,(#71006,#71007,#71008,#71009),
 .UNSPECIFIED.,.F.,.F.,(4,4),(0.,0.0458781805671206),.UNSPECIFIED.);
#9788=B_SPLINE_CURVE_WITH_KNOTS('',3,(#71015,#71016,#71017,#71018,#71019,
#71020,#71021,#71022,#71023,#71024,#71025,#71026,#71027,#71028),
 .UNSPECIFIED.,.F.,.F.,(4,2,2,2,2,2,4),(-0.11204561923996,-0.110611693715147,
-0.0954349222053108,-0.0802581506954743,-0.067781998776524,-0.0615439228170489,
-0.0553058468575738),.UNSPECIFIED.);
#9789=B_SPLINE_CURVE_WITH_KNOTS('',3,(#71042,#71043,#71044,#71045),
 .UNSPECIFIED.,.F.,.F.,(4,4),(-0.0458781805665616,0.),.UNSPECIFIED.);
#9790=B_SPLINE_CURVE_WITH_KNOTS('',3,(#71078,#71079,#71080,#71081),
 .UNSPECIFIED.,.F.,.F.,(4,4),(0.,0.0458781805665721),.UNSPECIFIED.);
#9791=B_SPLINE_CURVE_WITH_KNOTS('',3,(#71095,#71096,#71097,#71098,#71099,
#71100),.UNSPECIFIED.,.F.,.F.,(4,2,4),(0.022217000993734,0.0333260526322429,
0.0444418875612835),.UNSPECIFIED.);
#9792=B_SPLINE_CURVE_WITH_KNOTS('',3,(#71132,#71133,#71134,#71135),
 .UNSPECIFIED.,.F.,.F.,(4,4),(-0.0458781805671148,0.),.UNSPECIFIED.);
#9793=B_SPLINE_CURVE_WITH_KNOTS('',3,(#71137,#71138,#71139,#71140),
 .UNSPECIFIED.,.F.,.F.,(4,4),(0.,0.0458781805671148),.UNSPECIFIED.);
#9794=B_SPLINE_CURVE_WITH_KNOTS('',3,(#71146,#71147,#71148,#71149,#71150,
#71151,#71152,#71153,#71154,#71155,#71156,#71157,#71158,#71159),
 .UNSPECIFIED.,.F.,.F.,(4,2,2,2,2,2,4),(-0.112045619239962,-0.110611693715149,
-0.0954349222053128,-0.080258150695477,-0.0677819987765257,-0.0615439228170501,
-0.0553058468575745),.UNSPECIFIED.);
#9795=B_SPLINE_CURVE_WITH_KNOTS('',3,(#71173,#71174,#71175,#71176),
 .UNSPECIFIED.,.F.,.F.,(4,4),(-0.0458781805667336,0.),.UNSPECIFIED.);
#9796=B_SPLINE_CURVE_WITH_KNOTS('',3,(#71209,#71210,#71211,#71212),
 .UNSPECIFIED.,.F.,.F.,(4,4),(0.,0.0458781805667336),.UNSPECIFIED.);
#9797=B_SPLINE_CURVE_WITH_KNOTS('',3,(#71226,#71227,#71228,#71229,#71230,
#71231),.UNSPECIFIED.,.F.,.F.,(4,2,4),(0.0222170009937314,0.0333260526322431,
0.0444418875612844),.UNSPECIFIED.);
#9798=B_SPLINE_CURVE_WITH_KNOTS('',3,(#71235,#71236,#71237,#71238,#71239,
#71240,#71241,#71242,#71243,#71244,#71245,#71246,#71247,#71248),
 .UNSPECIFIED.,.F.,.F.,(4,2,2,2,2,2,4),(0.0553058468575744,0.0615439228170501,
0.0677819987765257,0.080258150695477,0.0954349222053129,0.110611693715149,
0.112045606679734),.UNSPECIFIED.);
#9799=B_SPLINE_CURVE_WITH_KNOTS('',3,(#71253,#71254,#71255,#71256,#71257,
#71258),.UNSPECIFIED.,.F.,.F.,(4,2,4),(0.133326015406808,0.144441850335849,
0.155550901974359),.UNSPECIFIED.);
#9800=B_SPLINE_CURVE_WITH_KNOTS('',3,(#71292,#71293,#71294,#71295),
 .UNSPECIFIED.,.F.,.F.,(4,4),(-0.0458781805671248,0.),.UNSPECIFIED.);
#9801=B_SPLINE_CURVE_WITH_KNOTS('',3,(#71297,#71298,#71299,#71300),
 .UNSPECIFIED.,.F.,.F.,(4,4),(0.,0.0458781805671248),.UNSPECIFIED.);
#9802=B_SPLINE_CURVE_WITH_KNOTS('',3,(#71306,#71307,#71308,#71309,#71310,
#71311,#71312,#71313,#71314,#71315,#71316,#71317,#71318,#71319),
 .UNSPECIFIED.,.F.,.F.,(4,2,2,2,2,2,4),(-0.112045619239962,-0.110611693715148,
-0.0954349222053121,-0.0802581506954758,-0.0677819987765249,-0.0615439228170494,
-0.055305846857574),.UNSPECIFIED.);
#9803=B_SPLINE_CURVE_WITH_KNOTS('',3,(#71333,#71334,#71335,#71336),
 .UNSPECIFIED.,.F.,.F.,(4,4),(-0.0458781805667819,0.),.UNSPECIFIED.);
#9804=B_SPLINE_CURVE_WITH_KNOTS('',3,(#71375,#71376,#71377,#71378),
 .UNSPECIFIED.,.F.,.F.,(4,4),(-0.0458781805671175,0.),.UNSPECIFIED.);
#9805=B_SPLINE_CURVE_WITH_KNOTS('',3,(#71380,#71381,#71382,#71383),
 .UNSPECIFIED.,.F.,.F.,(4,4),(0.,0.0458781805671175),.UNSPECIFIED.);
#9806=B_SPLINE_CURVE_WITH_KNOTS('',3,(#71389,#71390,#71391,#71392,#71393,
#71394,#71395,#71396,#71397,#71398,#71399,#71400,#71401,#71402),
 .UNSPECIFIED.,.F.,.F.,(4,2,2,2,2,2,4),(-0.112045619239961,-0.110611693715148,
-0.095434922205312,-0.0802581506954759,-0.067781998776525,-0.0615439228170495,
-0.0553058468575741),.UNSPECIFIED.);
#9807=B_SPLINE_CURVE_WITH_KNOTS('',3,(#71416,#71417,#71418,#71419),
 .UNSPECIFIED.,.F.,.F.,(4,4),(-0.0458781805667752,0.),.UNSPECIFIED.);
#9808=B_SPLINE_CURVE_WITH_KNOTS('',3,(#71458,#71459,#71460,#71461),
 .UNSPECIFIED.,.F.,.F.,(4,4),(-0.0458781805671191,0.),.UNSPECIFIED.);
#9809=B_SPLINE_CURVE_WITH_KNOTS('',3,(#71463,#71464,#71465,#71466),
 .UNSPECIFIED.,.F.,.F.,(4,4),(0.,0.0458781805671191),.UNSPECIFIED.);
#9810=B_SPLINE_CURVE_WITH_KNOTS('',3,(#71472,#71473,#71474,#71475,#71476,
#71477,#71478,#71479,#71480,#71481,#71482,#71483,#71484,#71485),
 .UNSPECIFIED.,.F.,.F.,(4,2,2,2,2,2,4),(-0.11204561923996,-0.110611693715147,
-0.0954349222053112,-0.0802581506954753,-0.0677819987765244,-0.061543922817049,
-0.0553058468575736),.UNSPECIFIED.);
#9811=B_SPLINE_CURVE_WITH_KNOTS('',3,(#71499,#71500,#71501,#71502),
 .UNSPECIFIED.,.F.,.F.,(4,4),(-0.0458781805667294,0.),.UNSPECIFIED.);
#9812=B_SPLINE_CURVE_WITH_KNOTS('',3,(#71527,#71528,#71529,#71530),
 .UNSPECIFIED.,.F.,.F.,(4,4),(0.,0.0458781805665616),.UNSPECIFIED.);
#9813=B_SPLINE_CURVE_WITH_KNOTS('',3,(#71544,#71545,#71546,#71547,#71548,
#71549),.UNSPECIFIED.,.F.,.F.,(4,2,4),(0.0222170009937336,0.0333260526322425,
0.0444418875612836),.UNSPECIFIED.);
#9814=B_SPLINE_CURVE_WITH_KNOTS('',3,(#71575,#71576,#71577,#71578),
 .UNSPECIFIED.,.F.,.F.,(4,4),(0.,0.045878180566425),.UNSPECIFIED.);
#9815=B_SPLINE_CURVE_WITH_KNOTS('',3,(#71592,#71593,#71594,#71595,#71596,
#71597),.UNSPECIFIED.,.F.,.F.,(4,2,4),(0.0222170009937342,0.0333260526322429,
0.0444418875612842),.UNSPECIFIED.);
#9816=B_SPLINE_CURVE_WITH_KNOTS('',3,(#71629,#71630,#71631,#71632),
 .UNSPECIFIED.,.F.,.F.,(4,4),(-0.0458781805670893,0.),.UNSPECIFIED.);
#9817=B_SPLINE_CURVE_WITH_KNOTS('',3,(#71634,#71635,#71636,#71637),
 .UNSPECIFIED.,.F.,.F.,(4,4),(0.,0.0458781805670893),.UNSPECIFIED.);
#9818=B_SPLINE_CURVE_WITH_KNOTS('',3,(#71643,#71644,#71645,#71646,#71647,
#71648,#71649,#71650,#71651,#71652,#71653,#71654,#71655,#71656),
 .UNSPECIFIED.,.F.,.F.,(4,2,2,2,2,2,4),(-0.112045619239962,-0.110611693715149,
-0.0954349222053129,-0.0802581506954765,-0.0677819987765255,-0.06154392281705,
-0.0553058468575744),.UNSPECIFIED.);
#9819=B_SPLINE_CURVE_WITH_KNOTS('',3,(#71670,#71671,#71672,#71673),
 .UNSPECIFIED.,.F.,.F.,(4,4),(-0.0458781805664109,0.),.UNSPECIFIED.);
#9820=B_SPLINE_CURVE_WITH_KNOTS('',3,(#71706,#71707,#71708,#71709),
 .UNSPECIFIED.,.F.,.F.,(4,4),(0.,0.0458781805664109),.UNSPECIFIED.);
#9821=B_SPLINE_CURVE_WITH_KNOTS('',3,(#71723,#71724,#71725,#71726,#71727,
#71728),.UNSPECIFIED.,.F.,.F.,(4,2,4),(0.0222170009937338,0.0333260526322426,
0.0444418875612839),.UNSPECIFIED.);
#9822=B_SPLINE_CURVE_WITH_KNOTS('',3,(#71732,#71733,#71734,#71735,#71736,
#71737,#71738,#71739,#71740,#71741,#71742,#71743,#71744,#71745),
 .UNSPECIFIED.,.F.,.F.,(4,2,2,2,2,2,4),(0.0553058468575737,0.061543922817049,
0.0677819987765242,0.0802581506954747,0.0954349222053112,0.110611693715148,
0.112045606679731),.UNSPECIFIED.);
#9823=B_SPLINE_CURVE_WITH_KNOTS('',3,(#71750,#71751,#71752,#71753,#71754,
#71755),.UNSPECIFIED.,.F.,.F.,(4,2,4),(0.133326015406807,0.144441850335849,
0.155550901974357),.UNSPECIFIED.);
#9824=B_SPLINE_CURVE_WITH_KNOTS('',3,(#71761,#71762,#71763,#71764,#71765,
#71766,#71767,#71768,#71769,#71770,#71771,#71772,#71773,#71774),
 .UNSPECIFIED.,.F.,.F.,(4,2,2,2,2,2,4),(0.0553058468575747,0.0615439228170501,
0.0677819987765256,0.0802581506954765,0.095434922205313,0.11061169371515,
0.112045606679734),.UNSPECIFIED.);
#9825=B_SPLINE_CURVE_WITH_KNOTS('',3,(#71779,#71780,#71781,#71782,#71783,
#71784),.UNSPECIFIED.,.F.,.F.,(4,2,4),(0.133326015406808,0.144441850335849,
0.155550901974361),.UNSPECIFIED.);
#9826=B_SPLINE_CURVE_WITH_KNOTS('',3,(#71812,#71813,#71814,#71815),
 .UNSPECIFIED.,.F.,.F.,(4,4),(0.,0.0458781805667294),.UNSPECIFIED.);
#9827=B_SPLINE_CURVE_WITH_KNOTS('',3,(#71833,#71834,#71835,#71836,#71837,
#71838),.UNSPECIFIED.,.F.,.F.,(4,2,4),(0.0222170009937294,0.0333260526322426,
0.0444418875612829),.UNSPECIFIED.);
#9828=B_SPLINE_CURVE_WITH_KNOTS('',3,(#71864,#71865,#71866,#71867),
 .UNSPECIFIED.,.F.,.F.,(4,4),(0.,0.0458781805667752),.UNSPECIFIED.);
#9829=B_SPLINE_CURVE_WITH_KNOTS('',3,(#71881,#71882,#71883,#71884,#71885,
#71886),.UNSPECIFIED.,.F.,.F.,(4,2,4),(0.0222170009937318,0.0333260526322428,
0.0444418875612841),.UNSPECIFIED.);
#9830=B_SPLINE_CURVE_WITH_KNOTS('',3,(#71918,#71919,#71920,#71921),
 .UNSPECIFIED.,.F.,.F.,(4,4),(-0.0458781805671226,0.),.UNSPECIFIED.);
#9831=B_SPLINE_CURVE_WITH_KNOTS('',3,(#71923,#71924,#71925,#71926),
 .UNSPECIFIED.,.F.,.F.,(4,4),(0.,0.0458781805671226),.UNSPECIFIED.);
#9832=B_SPLINE_CURVE_WITH_KNOTS('',3,(#71932,#71933,#71934,#71935,#71936,
#71937,#71938,#71939,#71940,#71941,#71942,#71943,#71944,#71945),
 .UNSPECIFIED.,.F.,.F.,(4,2,2,2,2,2,4),(-0.112045619239962,-0.110611693715148,
-0.095434922205312,-0.0802581506954755,-0.0677819987765242,-0.0615439228170485,
-0.0553058468575729),.UNSPECIFIED.);
#9833=B_SPLINE_CURVE_WITH_KNOTS('',3,(#71959,#71960,#71961,#71962),
 .UNSPECIFIED.,.F.,.F.,(4,4),(-0.0458781805667781,0.),.UNSPECIFIED.);
#9834=B_SPLINE_CURVE_WITH_KNOTS('',3,(#71987,#71988,#71989,#71990),
 .UNSPECIFIED.,.F.,.F.,(4,4),(0.,0.0458781805667819),.UNSPECIFIED.);
#9835=B_SPLINE_CURVE_WITH_KNOTS('',3,(#72004,#72005,#72006,#72007,#72008,
#72009),.UNSPECIFIED.,.F.,.F.,(4,2,4),(0.0222170009937351,0.0333260526322426,
0.0444418875612842),.UNSPECIFIED.);
#9836=B_SPLINE_CURVE_WITH_KNOTS('',3,(#72041,#72042,#72043,#72044),
 .UNSPECIFIED.,.F.,.F.,(4,4),(-0.0458781805671222,0.),.UNSPECIFIED.);
#9837=B_SPLINE_CURVE_WITH_KNOTS('',3,(#72046,#72047,#72048,#72049),
 .UNSPECIFIED.,.F.,.F.,(4,4),(0.,0.0458781805671222),.UNSPECIFIED.);
#9838=B_SPLINE_CURVE_WITH_KNOTS('',3,(#72055,#72056,#72057,#72058,#72059,
#72060,#72061,#72062,#72063,#72064,#72065,#72066,#72067,#72068),
 .UNSPECIFIED.,.F.,.F.,(4,2,2,2,2,2,4),(-0.112045619239963,-0.110611693715148,
-0.0954349222053123,-0.0802581506954764,-0.0677819987765256,-0.0615439228170503,
-0.0553058468575749),.UNSPECIFIED.);
#9839=B_SPLINE_CURVE_WITH_KNOTS('',3,(#72082,#72083,#72084,#72085),
 .UNSPECIFIED.,.F.,.F.,(4,4),(-0.0458781805667355,0.),.UNSPECIFIED.);
#9840=B_SPLINE_CURVE_WITH_KNOTS('',3,(#72118,#72119,#72120,#72121),
 .UNSPECIFIED.,.F.,.F.,(4,4),(0.,0.0458781805667355),.UNSPECIFIED.);
#9841=B_SPLINE_CURVE_WITH_KNOTS('',3,(#72135,#72136,#72137,#72138,#72139,
#72140),.UNSPECIFIED.,.F.,.F.,(4,2,4),(0.0222170009937323,0.033326052632243,
0.0444418875612838),.UNSPECIFIED.);
#9842=B_SPLINE_CURVE_WITH_KNOTS('',3,(#72144,#72145,#72146,#72147,#72148,
#72149,#72150,#72151,#72152,#72153,#72154,#72155,#72156,#72157),
 .UNSPECIFIED.,.F.,.F.,(4,2,2,2,2,2,4),(0.0553058468575738,0.0615439228170493,
0.0677819987765247,0.0802581506954757,0.0954349222053123,0.110611693715149,
0.112045606679732),.UNSPECIFIED.);
#9843=B_SPLINE_CURVE_WITH_KNOTS('',3,(#72162,#72163,#72164,#72165,#72166,
#72167),.UNSPECIFIED.,.F.,.F.,(4,2,4),(0.133326015406808,0.144441850335849,
0.155550901974359),.UNSPECIFIED.);
#9844=B_SPLINE_CURVE_WITH_KNOTS('',3,(#72195,#72196,#72197,#72198),
 .UNSPECIFIED.,.F.,.F.,(4,4),(0.,0.0458781805667781),.UNSPECIFIED.);
#9845=B_SPLINE_CURVE_WITH_KNOTS('',3,(#72216,#72217,#72218,#72219,#72220,
#72221),.UNSPECIFIED.,.F.,.F.,(4,2,4),(0.0222170009937297,0.0333260526322422,
0.0444418875612833),.UNSPECIFIED.);
#9846=B_SPLINE_CURVE_WITH_KNOTS('',3,(#72225,#72226,#72227,#72228,#72229,
#72230,#72231,#72232,#72233,#72234,#72235,#72236,#72237,#72238),
 .UNSPECIFIED.,.F.,.F.,(4,2,2,2,2,2,4),(0.055305846857575,0.0615439228170507,
0.0677819987765264,0.0802581506954779,0.0954349222053137,0.11061169371515,
0.112045606679733),.UNSPECIFIED.);
#9847=B_SPLINE_CURVE_WITH_KNOTS('',3,(#72243,#72244,#72245,#72246,#72247,
#72248),.UNSPECIFIED.,.F.,.F.,(4,2,4),(0.133326015406807,0.144441850335848,
0.155550901974357),.UNSPECIFIED.);
#9848=B_SPLINE_CURVE_WITH_KNOTS('',3,(#72282,#72283,#72284,#72285),
 .UNSPECIFIED.,.F.,.F.,(4,4),(-0.045878180567112,0.),.UNSPECIFIED.);
#9849=B_SPLINE_CURVE_WITH_KNOTS('',3,(#72287,#72288,#72289,#72290),
 .UNSPECIFIED.,.F.,.F.,(4,4),(0.,0.045878180567112),.UNSPECIFIED.);
#9850=B_SPLINE_CURVE_WITH_KNOTS('',3,(#72296,#72297,#72298,#72299,#72300,
#72301,#72302,#72303,#72304,#72305,#72306,#72307,#72308,#72309),
 .UNSPECIFIED.,.F.,.F.,(4,2,2,2,2,2,4),(-0.112045619239962,-0.11061169371515,
-0.0954349222053132,-0.0802581506954765,-0.0677819987765257,-0.0615439228170503,
-0.0553058468575749),.UNSPECIFIED.);
#9851=B_SPLINE_CURVE_WITH_KNOTS('',3,(#72323,#72324,#72325,#72326),
 .UNSPECIFIED.,.F.,.F.,(4,4),(-0.0458781805664203,0.),.UNSPECIFIED.);
#9852=B_SPLINE_CURVE_WITH_KNOTS('',3,(#72365,#72366,#72367,#72368),
 .UNSPECIFIED.,.F.,.F.,(4,4),(-0.0458781805671177,0.),.UNSPECIFIED.);
#9853=B_SPLINE_CURVE_WITH_KNOTS('',3,(#72370,#72371,#72372,#72373),
 .UNSPECIFIED.,.F.,.F.,(4,4),(0.,0.0458781805671177),.UNSPECIFIED.);
#9854=B_SPLINE_CURVE_WITH_KNOTS('',3,(#72379,#72380,#72381,#72382,#72383,
#72384,#72385,#72386,#72387,#72388,#72389,#72390,#72391,#72392),
 .UNSPECIFIED.,.F.,.F.,(4,2,2,2,2,2,4),(-0.112045619239958,-0.110611693715147,
-0.0954349222053108,-0.0802581506954743,-0.067781998776524,-0.0615439228170488,
-0.0553058468575736),.UNSPECIFIED.);
#9855=B_SPLINE_CURVE_WITH_KNOTS('',3,(#72406,#72407,#72408,#72409),
 .UNSPECIFIED.,.F.,.F.,(4,4),(-0.0458781805665577,0.),.UNSPECIFIED.);
#9856=B_SPLINE_CURVE_WITH_KNOTS('',3,(#72448,#72449,#72450,#72451),
 .UNSPECIFIED.,.F.,.F.,(4,4),(-0.0458781805671118,0.),.UNSPECIFIED.);
#9857=B_SPLINE_CURVE_WITH_KNOTS('',3,(#72453,#72454,#72455,#72456),
 .UNSPECIFIED.,.F.,.F.,(4,4),(0.,0.0458781805671118),.UNSPECIFIED.);
#9858=B_SPLINE_CURVE_WITH_KNOTS('',3,(#72462,#72463,#72464,#72465,#72466,
#72467,#72468,#72469,#72470,#72471,#72472,#72473,#72474,#72475),
 .UNSPECIFIED.,.F.,.F.,(4,2,2,2,2,2,4),(-0.112045619239959,-0.110611693715147,
-0.0954349222053111,-0.0802581506954753,-0.0677819987765244,-0.0615439228170489,
-0.0553058468575734),.UNSPECIFIED.);
#9859=B_SPLINE_CURVE_WITH_KNOTS('',3,(#72489,#72490,#72491,#72492),
 .UNSPECIFIED.,.F.,.F.,(4,4),(-0.0458781805665584,0.),.UNSPECIFIED.);
#9860=B_SPLINE_CURVE_WITH_KNOTS('',3,(#72523,#72524,#72525,#72526),
 .UNSPECIFIED.,.F.,.F.,(4,4),(-0.0458781805671198,0.),.UNSPECIFIED.);
#9861=B_SPLINE_CURVE_WITH_KNOTS('',3,(#72528,#72529,#72530,#72531),
 .UNSPECIFIED.,.F.,.F.,(4,4),(0.,0.0458781805671198),.UNSPECIFIED.);
#9862=B_SPLINE_CURVE_WITH_KNOTS('',3,(#72537,#72538,#72539,#72540,#72541,
#72542,#72543,#72544,#72545,#72546,#72547,#72548,#72549,#72550),
 .UNSPECIFIED.,.F.,.F.,(4,2,2,2,2,2,4),(-0.112045619239961,-0.110611693715148,
-0.0954349222053111,-0.0802581506954746,-0.0677819987765242,-0.061543922817049,
-0.0553058468575738),.UNSPECIFIED.);
#9863=B_SPLINE_CURVE_WITH_KNOTS('',3,(#72564,#72565,#72566,#72567),
 .UNSPECIFIED.,.F.,.F.,(4,4),(-0.0458781805667331,0.),.UNSPECIFIED.);
#9864=B_SPLINE_CURVE_WITH_KNOTS('',3,(#72600,#72601,#72602,#72603),
 .UNSPECIFIED.,.F.,.F.,(4,4),(0.,0.0458781805667331),.UNSPECIFIED.);
#9865=B_SPLINE_CURVE_WITH_KNOTS('',3,(#72617,#72618,#72619,#72620,#72621,
#72622),.UNSPECIFIED.,.F.,.F.,(4,2,4),(0.0222170009937327,0.0333260526322426,
0.044441887561284),.UNSPECIFIED.);
#9866=B_SPLINE_CURVE_WITH_KNOTS('',3,(#72648,#72649,#72650,#72651),
 .UNSPECIFIED.,.F.,.F.,(4,4),(0.,0.0458781805665584),.UNSPECIFIED.);
#9867=B_SPLINE_CURVE_WITH_KNOTS('',3,(#72669,#72670,#72671,#72672,#72673,
#72674),.UNSPECIFIED.,.F.,.F.,(4,2,4),(0.0222170009937324,0.0333260526322424,
0.0444418875612831),.UNSPECIFIED.);
#9868=B_SPLINE_CURVE_WITH_KNOTS('',3,(#72706,#72707,#72708,#72709),
 .UNSPECIFIED.,.F.,.F.,(4,4),(-0.0458781805671227,0.),.UNSPECIFIED.);
#9869=B_SPLINE_CURVE_WITH_KNOTS('',3,(#72711,#72712,#72713,#72714),
 .UNSPECIFIED.,.F.,.F.,(4,4),(0.,0.0458781805671227),.UNSPECIFIED.);
#9870=B_SPLINE_CURVE_WITH_KNOTS('',3,(#72720,#72721,#72722,#72723,#72724,
#72725,#72726,#72727,#72728,#72729,#72730,#72731,#72732,#72733),
 .UNSPECIFIED.,.F.,.F.,(4,2,2,2,2,2,4),(-0.112045619239962,-0.11061169371515,
-0.0954349222053127,-0.0802581506954759,-0.0677819987765254,-0.0615439228170502,
-0.0553058468575749),.UNSPECIFIED.);
#9871=B_SPLINE_CURVE_WITH_KNOTS('',3,(#72747,#72748,#72749,#72750),
 .UNSPECIFIED.,.F.,.F.,(4,4),(-0.0458781805667359,0.),.UNSPECIFIED.);
#9872=B_SPLINE_CURVE_WITH_KNOTS('',3,(#72789,#72790,#72791,#72792),
 .UNSPECIFIED.,.F.,.F.,(4,4),(-0.0458781805671102,0.),.UNSPECIFIED.);
#9873=B_SPLINE_CURVE_WITH_KNOTS('',3,(#72794,#72795,#72796,#72797),
 .UNSPECIFIED.,.F.,.F.,(4,4),(0.,0.0458781805671102),.UNSPECIFIED.);
#9874=B_SPLINE_CURVE_WITH_KNOTS('',3,(#72803,#72804,#72805,#72806,#72807,
#72808,#72809,#72810,#72811,#72812,#72813,#72814,#72815,#72816),
 .UNSPECIFIED.,.F.,.F.,(4,2,2,2,2,2,4),(-0.112045619239961,-0.110611693715148,
-0.0954349222053117,-0.0802581506954758,-0.0677819987765249,-0.0615439228170493,
-0.0553058468575738),.UNSPECIFIED.);
#9875=B_SPLINE_CURVE_WITH_KNOTS('',3,(#72830,#72831,#72832,#72833),
 .UNSPECIFIED.,.F.,.F.,(4,4),(-0.0458781805667336,0.),.UNSPECIFIED.);
#9876=B_SPLINE_CURVE_WITH_KNOTS('',3,(#72858,#72859,#72860,#72861),
 .UNSPECIFIED.,.F.,.F.,(4,4),(0.,0.0458781805665577),.UNSPECIFIED.);
#9877=B_SPLINE_CURVE_WITH_KNOTS('',3,(#72875,#72876,#72877,#72878,#72879,
#72880),.UNSPECIFIED.,.F.,.F.,(4,2,4),(0.0222170009937346,0.0333260526322427,
0.0444418875612839),.UNSPECIFIED.);
#9878=B_SPLINE_CURVE_WITH_KNOTS('',3,(#72906,#72907,#72908,#72909),
 .UNSPECIFIED.,.F.,.F.,(4,4),(0.,0.0458781805664203),.UNSPECIFIED.);
#9879=B_SPLINE_CURVE_WITH_KNOTS('',3,(#72923,#72924,#72925,#72926,#72927,
#72928),.UNSPECIFIED.,.F.,.F.,(4,2,4),(0.0222170009937336,0.0333260526322428,
0.0444418875612842),.UNSPECIFIED.);
#9880=B_SPLINE_CURVE_WITH_KNOTS('',3,(#72960,#72961,#72962,#72963),
 .UNSPECIFIED.,.F.,.F.,(4,4),(-0.0458781805670802,0.),.UNSPECIFIED.);
#9881=B_SPLINE_CURVE_WITH_KNOTS('',3,(#72965,#72966,#72967,#72968),
 .UNSPECIFIED.,.F.,.F.,(4,4),(0.,0.0458781805670802),.UNSPECIFIED.);
#9882=B_SPLINE_CURVE_WITH_KNOTS('',3,(#72974,#72975,#72976,#72977,#72978,
#72979,#72980,#72981,#72982,#72983,#72984,#72985,#72986,#72987),
 .UNSPECIFIED.,.F.,.F.,(4,2,2,2,2,2,4),(-0.112045619239963,-0.110611693715149,
-0.0954349222053127,-0.0802581506954762,-0.0677819987765253,-0.0615439228170498,
-0.0553058468575744),.UNSPECIFIED.);
#9883=B_SPLINE_CURVE_WITH_KNOTS('',3,(#73001,#73002,#73003,#73004),
 .UNSPECIFIED.,.F.,.F.,(4,4),(-0.0458781805664058,0.),.UNSPECIFIED.);
#9884=B_SPLINE_CURVE_WITH_KNOTS('',3,(#73037,#73038,#73039,#73040),
 .UNSPECIFIED.,.F.,.F.,(4,4),(0.,0.0458781805665695),.UNSPECIFIED.);
#9885=B_SPLINE_CURVE_WITH_KNOTS('',3,(#73051,#73052,#73053,#73054,#73055,
#73056,#73057,#73058,#73059,#73060,#73061,#73062,#73063,#73064),
 .UNSPECIFIED.,.F.,.F.,(4,2,2,2,2,2,4),(0.0553058468575735,0.0615439228170487,
0.0677819987765239,0.0802581506954742,0.0954349222053109,0.110611693715148,
0.112045606679732),.UNSPECIFIED.);
#9886=B_SPLINE_CURVE_WITH_KNOTS('',3,(#73069,#73070,#73071,#73072,#73073,
#73074),.UNSPECIFIED.,.F.,.F.,(4,2,4),(0.133326015406808,0.144441850335849,
0.155550901974358),.UNSPECIFIED.);
#9887=B_SPLINE_CURVE_WITH_KNOTS('',3,(#73102,#73103,#73104,#73105),
 .UNSPECIFIED.,.F.,.F.,(4,4),(0.,0.0458781805664058),.UNSPECIFIED.);
#9888=B_SPLINE_CURVE_WITH_KNOTS('',3,(#73119,#73120,#73121,#73122,#73123,
#73124),.UNSPECIFIED.,.F.,.F.,(4,2,4),(0.0222170009937338,0.0333260526322426,
0.0444418875612839),.UNSPECIFIED.);
#9889=B_SPLINE_CURVE_WITH_KNOTS('',3,(#73128,#73129,#73130,#73131,#73132,
#73133,#73134,#73135,#73136,#73137,#73138,#73139,#73140,#73141),
 .UNSPECIFIED.,.F.,.F.,(4,2,2,2,2,2,4),(0.0553058468575736,0.0615439228170489,
0.0677819987765241,0.0802581506954747,0.0954349222053112,0.110611693715148,
0.112045606679731),.UNSPECIFIED.);
#9890=B_SPLINE_CURVE_WITH_KNOTS('',3,(#73146,#73147,#73148,#73149,#73150,
#73151),.UNSPECIFIED.,.F.,.F.,(4,2,4),(0.133326015406807,0.144441850335849,
0.155550901974357),.UNSPECIFIED.);
#9891=B_SPLINE_CURVE_WITH_KNOTS('',3,(#73157,#73158,#73159,#73160,#73161,
#73162,#73163,#73164,#73165,#73166,#73167,#73168,#73169,#73170),
 .UNSPECIFIED.,.F.,.F.,(4,2,2,2,2,2,4),(0.0553058468575749,0.0615439228170503,
0.0677819987765258,0.0802581506954767,0.0954349222053132,0.11061169371515,
0.112045606679735),.UNSPECIFIED.);
#9892=B_SPLINE_CURVE_WITH_KNOTS('',3,(#73175,#73176,#73177,#73178,#73179,
#73180),.UNSPECIFIED.,.F.,.F.,(4,2,4),(0.133326015406807,0.144441850335848,
0.155550901974357),.UNSPECIFIED.);
#9893=B_SPLINE_CURVE_WITH_KNOTS('',3,(#73208,#73209,#73210,#73211),
 .UNSPECIFIED.,.F.,.F.,(4,4),(0.,0.0458781805667336),.UNSPECIFIED.);
#9894=B_SPLINE_CURVE_WITH_KNOTS('',3,(#73229,#73230,#73231,#73232,#73233,
#73234),.UNSPECIFIED.,.F.,.F.,(4,2,4),(0.0222170009937288,0.0333260526322423,
0.044441887561283),.UNSPECIFIED.);
#9895=B_SPLINE_CURVE_WITH_KNOTS('',3,(#73260,#73261,#73262,#73263),
 .UNSPECIFIED.,.F.,.F.,(4,4),(0.,0.0458781805667359),.UNSPECIFIED.);
#9896=B_SPLINE_CURVE_WITH_KNOTS('',3,(#73277,#73278,#73279,#73280,#73281,
#73282),.UNSPECIFIED.,.F.,.F.,(4,2,4),(0.0222170009937317,0.033326052632243,
0.0444418875612838),.UNSPECIFIED.);
#9897=B_SPLINE_CURVE_WITH_KNOTS('',3,(#73314,#73315,#73316,#73317),
 .UNSPECIFIED.,.F.,.F.,(4,4),(-0.0458781805670993,0.),.UNSPECIFIED.);
#9898=B_SPLINE_CURVE_WITH_KNOTS('',3,(#73319,#73320,#73321,#73322),
 .UNSPECIFIED.,.F.,.F.,(4,4),(0.,0.0458781805670993),.UNSPECIFIED.);
#9899=B_SPLINE_CURVE_WITH_KNOTS('',3,(#73328,#73329,#73330,#73331,#73332,
#73333,#73334,#73335,#73336,#73337,#73338,#73339,#73340,#73341),
 .UNSPECIFIED.,.F.,.F.,(4,2,2,2,2,2,4),(-0.11204561923996,-0.110611693715147,
-0.0954349222053112,-0.0802581506954753,-0.0677819987765244,-0.0615439228170489,
-0.0553058468575734),.UNSPECIFIED.);
#9900=B_SPLINE_CURVE_WITH_KNOTS('',3,(#73355,#73356,#73357,#73358),
 .UNSPECIFIED.,.F.,.F.,(4,4),(-0.0458781805665721,0.),.UNSPECIFIED.);
#9901=B_SPLINE_CURVE_WITH_KNOTS('',3,(#73391,#73392,#73393,#73394),
 .UNSPECIFIED.,.F.,.F.,(4,4),(0.,0.0458781805667874),.UNSPECIFIED.);
#9902=B_SPLINE_CURVE_WITH_KNOTS('',3,(#73405,#73406,#73407,#73408,#73409,
#73410,#73411,#73412,#73413,#73414,#73415,#73416,#73417,#73418),
 .UNSPECIFIED.,.F.,.F.,(4,2,2,2,2,2,4),(0.0553058468575741,0.0615439228170497,
0.0677819987765252,0.0802581506954764,0.0954349222053128,0.110611693715149,
0.112045606679733),.UNSPECIFIED.);
#9903=B_SPLINE_CURVE_WITH_KNOTS('',3,(#73423,#73424,#73425,#73426,#73427,
#73428),.UNSPECIFIED.,.F.,.F.,(4,2,4),(0.133326015406808,0.144441850335849,
0.155550901974358),.UNSPECIFIED.);
#9904=B_SPLINE_CURVE_WITH_KNOTS('',3,(#73462,#73463,#73464,#73465),
 .UNSPECIFIED.,.F.,.F.,(4,4),(-0.0458781805671104,0.),.UNSPECIFIED.);
#9905=B_SPLINE_CURVE_WITH_KNOTS('',3,(#73467,#73468,#73469,#73470),
 .UNSPECIFIED.,.F.,.F.,(4,4),(0.,0.0458781805671104),.UNSPECIFIED.);
#9906=B_SPLINE_CURVE_WITH_KNOTS('',3,(#73476,#73477,#73478,#73479,#73480,
#73481,#73482,#73483,#73484,#73485,#73486,#73487,#73488,#73489),
 .UNSPECIFIED.,.F.,.F.,(4,2,2,2,2,2,4),(-0.11204561923996,-0.110611693715149,
-0.0954349222053131,-0.0802581506954772,-0.0677819987765258,-0.0615439228170501,
-0.0553058468575744),.UNSPECIFIED.);
#9907=B_SPLINE_CURVE_WITH_KNOTS('',3,(#73503,#73504,#73505,#73506),
 .UNSPECIFIED.,.F.,.F.,(4,4),(-0.0458781805664257,0.),.UNSPECIFIED.);
#9908=B_SPLINE_CURVE_WITH_KNOTS('',3,(#73545,#73546,#73547,#73548),
 .UNSPECIFIED.,.F.,.F.,(4,4),(-0.0458781805671196,0.),.UNSPECIFIED.);
#9909=B_SPLINE_CURVE_WITH_KNOTS('',3,(#73550,#73551,#73552,#73553),
 .UNSPECIFIED.,.F.,.F.,(4,4),(0.,0.0458781805671196),.UNSPECIFIED.);
#9910=B_SPLINE_CURVE_WITH_KNOTS('',3,(#73559,#73560,#73561,#73562,#73563,
#73564,#73565,#73566,#73567,#73568,#73569,#73570,#73571,#73572),
 .UNSPECIFIED.,.F.,.F.,(4,2,2,2,2,2,4),(-0.112045619239961,-0.110611693715147,
-0.0954349222053108,-0.0802581506954743,-0.0677819987765239,-0.0615439228170487,
-0.0553058468575735),.UNSPECIFIED.);
#9911=B_SPLINE_CURVE_WITH_KNOTS('',3,(#73586,#73587,#73588,#73589),
 .UNSPECIFIED.,.F.,.F.,(4,4),(-0.0458781805665626,0.),.UNSPECIFIED.);
#9912=B_SPLINE_CURVE_WITH_KNOTS('',3,(#73622,#73623,#73624,#73625),
 .UNSPECIFIED.,.F.,.F.,(4,4),(0.,0.0458781805665721),.UNSPECIFIED.);
#9913=B_SPLINE_CURVE_WITH_KNOTS('',3,(#73639,#73640,#73641,#73642,#73643,
#73644),.UNSPECIFIED.,.F.,.F.,(4,2,4),(0.0222170009937341,0.0333260526322432,
0.0444418875612838),.UNSPECIFIED.);
#9914=B_SPLINE_CURVE_WITH_KNOTS('',3,(#73676,#73677,#73678,#73679),
 .UNSPECIFIED.,.F.,.F.,(4,4),(-0.0458781805671142,0.),.UNSPECIFIED.);
#9915=B_SPLINE_CURVE_WITH_KNOTS('',3,(#73681,#73682,#73683,#73684),
 .UNSPECIFIED.,.F.,.F.,(4,4),(0.,0.0458781805671142),.UNSPECIFIED.);
#9916=B_SPLINE_CURVE_WITH_KNOTS('',3,(#73690,#73691,#73692,#73693,#73694,
#73695,#73696,#73697,#73698,#73699,#73700,#73701,#73702,#73703),
 .UNSPECIFIED.,.F.,.F.,(4,2,2,2,2,2,4),(-0.112045619239961,-0.110611693715149,
-0.095434922205313,-0.0802581506954771,-0.0677819987765258,-0.0615439228170502,
-0.0553058468575746),.UNSPECIFIED.);
#9917=B_SPLINE_CURVE_WITH_KNOTS('',3,(#73717,#73718,#73719,#73720),
 .UNSPECIFIED.,.F.,.F.,(4,4),(-0.0458781805665558,0.),.UNSPECIFIED.);
#9918=B_SPLINE_CURVE_WITH_KNOTS('',3,(#73751,#73752,#73753,#73754),
 .UNSPECIFIED.,.F.,.F.,(4,4),(-0.0458781805671177,0.),.UNSPECIFIED.);
#9919=B_SPLINE_CURVE_WITH_KNOTS('',3,(#73756,#73757,#73758,#73759),
 .UNSPECIFIED.,.F.,.F.,(4,4),(0.,0.0458781805671177),.UNSPECIFIED.);
#9920=B_SPLINE_CURVE_WITH_KNOTS('',3,(#73765,#73766,#73767,#73768,#73769,
#73770,#73771,#73772,#73773,#73774,#73775,#73776,#73777,#73778),
 .UNSPECIFIED.,.F.,.F.,(4,2,2,2,2,2,4),(-0.112045619239961,-0.110611693715147,
-0.0954349222053108,-0.0802581506954744,-0.0677819987765238,-0.0615439228170485,
-0.0553058468575731),.UNSPECIFIED.);
#9921=B_SPLINE_CURVE_WITH_KNOTS('',3,(#73792,#73793,#73794,#73795),
 .UNSPECIFIED.,.F.,.F.,(4,4),(-0.0458781805667322,0.),.UNSPECIFIED.);
#9922=B_SPLINE_CURVE_WITH_KNOTS('',3,(#73861,#73862,#73863,#73864),
 .UNSPECIFIED.,.F.,.F.,(4,4),(-0.04587818056712,0.),.UNSPECIFIED.);
#9923=B_SPLINE_CURVE_WITH_KNOTS('',3,(#73866,#73867,#73868,#73869),
 .UNSPECIFIED.,.F.,.F.,(4,4),(0.,0.04587818056712),.UNSPECIFIED.);
#9924=B_SPLINE_CURVE_WITH_KNOTS('',3,(#73875,#73876,#73877,#73878,#73879,
#73880,#73881,#73882,#73883,#73884,#73885,#73886,#73887,#73888),
 .UNSPECIFIED.,.F.,.F.,(4,2,2,2,2,2,4),(-0.112045619239957,-0.110611693715148,
-0.0954349222053112,-0.0802581506954748,-0.0677819987765241,-0.0615439228170488,
-0.0553058468575735),.UNSPECIFIED.);
#9925=B_SPLINE_CURVE_WITH_KNOTS('',3,(#73902,#73903,#73904,#73905),
 .UNSPECIFIED.,.F.,.F.,(4,4),(-0.0458781805667838,0.),.UNSPECIFIED.);
#9926=B_SPLINE_CURVE_WITH_KNOTS('',3,(#73930,#73931,#73932,#73933),
 .UNSPECIFIED.,.F.,.F.,(4,4),(0.,0.0458781805667838),.UNSPECIFIED.);
#9927=B_SPLINE_CURVE_WITH_KNOTS('',3,(#73951,#73952,#73953,#73954,#73955,
#73956),.UNSPECIFIED.,.F.,.F.,(4,2,4),(0.0222170009937294,0.0333260526322421,
0.0444418875612831),.UNSPECIFIED.);
#9928=B_SPLINE_CURVE_WITH_KNOTS('',3,(#73982,#73983,#73984,#73985),
 .UNSPECIFIED.,.F.,.F.,(4,4),(0.,0.0458781805667322),.UNSPECIFIED.);
#9929=B_SPLINE_CURVE_WITH_KNOTS('',3,(#73999,#74000,#74001,#74002,#74003,
#74004),.UNSPECIFIED.,.F.,.F.,(4,2,4),(0.0222170009937333,0.0333260526322436,
0.044441887561284),.UNSPECIFIED.);
#9930=B_SPLINE_CURVE_WITH_KNOTS('',3,(#74030,#74031,#74032,#74033),
 .UNSPECIFIED.,.F.,.F.,(4,4),(0.,0.0458781805665558),.UNSPECIFIED.);
#9931=B_SPLINE_CURVE_WITH_KNOTS('',3,(#74051,#74052,#74053,#74054,#74055,
#74056),.UNSPECIFIED.,.F.,.F.,(4,2,4),(0.0222170009937317,0.0333260526322426,
0.0444418875612832),.UNSPECIFIED.);
#9932=B_SPLINE_CURVE_WITH_KNOTS('',3,(#74060,#74061,#74062,#74063,#74064,
#74065,#74066,#74067,#74068,#74069,#74070,#74071,#74072,#74073),
 .UNSPECIFIED.,.F.,.F.,(4,2,2,2,2,2,4),(0.0553058468575744,0.0615439228170499,
0.0677819987765254,0.0802581506954764,0.0954349222053129,0.110611693715149,
0.112045606679733),.UNSPECIFIED.);
#9933=B_SPLINE_CURVE_WITH_KNOTS('',3,(#74078,#74079,#74080,#74081,#74082,
#74083),.UNSPECIFIED.,.F.,.F.,(4,2,4),(0.133326015406808,0.144441850335849,
0.155550901974359),.UNSPECIFIED.);
#9934=B_SPLINE_CURVE_WITH_KNOTS('',3,(#74111,#74112,#74113,#74114),
 .UNSPECIFIED.,.F.,.F.,(4,4),(0.,0.0458781805665626),.UNSPECIFIED.);
#9935=B_SPLINE_CURVE_WITH_KNOTS('',3,(#74128,#74129,#74130,#74131,#74132,
#74133),.UNSPECIFIED.,.F.,.F.,(4,2,4),(0.0222170009937308,0.0333260526322429,
0.0444418875612833),.UNSPECIFIED.);
#9936=B_SPLINE_CURVE_WITH_KNOTS('',3,(#74159,#74160,#74161,#74162),
 .UNSPECIFIED.,.F.,.F.,(4,4),(0.,0.0458781805664257),.UNSPECIFIED.);
#9937=B_SPLINE_CURVE_WITH_KNOTS('',3,(#74176,#74177,#74178,#74179,#74180,
#74181),.UNSPECIFIED.,.F.,.F.,(4,2,4),(0.0222170009937338,0.0333260526322428,
0.0444418875612842),.UNSPECIFIED.);
#9938=B_SPLINE_CURVE_WITH_KNOTS('',3,(#74213,#74214,#74215,#74216),
 .UNSPECIFIED.,.F.,.F.,(4,4),(-0.0458781805670871,0.),.UNSPECIFIED.);
#9939=B_SPLINE_CURVE_WITH_KNOTS('',3,(#74218,#74219,#74220,#74221),
 .UNSPECIFIED.,.F.,.F.,(4,4),(0.,0.0458781805670871),.UNSPECIFIED.);
#9940=B_SPLINE_CURVE_WITH_KNOTS('',3,(#74227,#74228,#74229,#74230,#74231,
#74232,#74233,#74234,#74235,#74236,#74237,#74238,#74239,#74240),
 .UNSPECIFIED.,.F.,.F.,(4,2,2,2,2,2,4),(-0.112045619239962,-0.110611693715149,
-0.0954349222053129,-0.0802581506954765,-0.0677819987765255,-0.06154392281705,
-0.0553058468575744),.UNSPECIFIED.);
#9941=B_SPLINE_CURVE_WITH_KNOTS('',3,(#74254,#74255,#74256,#74257),
 .UNSPECIFIED.,.F.,.F.,(4,4),(-0.0458781805664109,0.),.UNSPECIFIED.);
#9942=B_SPLINE_CURVE_WITH_KNOTS('',3,(#74290,#74291,#74292,#74293),
 .UNSPECIFIED.,.F.,.F.,(4,4),(0.,0.0458781805664109),.UNSPECIFIED.);
#9943=B_SPLINE_CURVE_WITH_KNOTS('',3,(#74307,#74308,#74309,#74310,#74311,
#74312),.UNSPECIFIED.,.F.,.F.,(4,2,4),(0.0222170009937338,0.0333260526322426,
0.0444418875612839),.UNSPECIFIED.);
#9944=B_SPLINE_CURVE_WITH_KNOTS('',3,(#74316,#74317,#74318,#74319,#74320,
#74321,#74322,#74323,#74324,#74325,#74326,#74327,#74328,#74329),
 .UNSPECIFIED.,.F.,.F.,(4,2,2,2,2,2,4),(0.0553058468575736,0.0615439228170488,
0.0677819987765241,0.0802581506954746,0.0954349222053112,0.110611693715148,
0.112045606679732),.UNSPECIFIED.);
#9945=B_SPLINE_CURVE_WITH_KNOTS('',3,(#74334,#74335,#74336,#74337,#74338,
#74339),.UNSPECIFIED.,.F.,.F.,(4,2,4),(0.133326015406807,0.144441850335848,
0.155550901974356),.UNSPECIFIED.);
#9946=B_SPLINE_CURVE_WITH_KNOTS('',3,(#74345,#74346,#74347,#74348,#74349,
#74350,#74351,#74352,#74353,#74354,#74355,#74356,#74357,#74358),
 .UNSPECIFIED.,.F.,.F.,(4,2,2,2,2,2,4),(0.0553058468575751,0.0615439228170507,
0.0677819987765263,0.0802581506954776,0.0954349222053135,0.110611693715149,
0.112045606679735),.UNSPECIFIED.);
#9947=B_SPLINE_CURVE_WITH_KNOTS('',3,(#74363,#74364,#74365,#74366,#74367,
#74368),.UNSPECIFIED.,.F.,.F.,(4,2,4),(0.133326015406807,0.144441850335849,
0.15555090197436),.UNSPECIFIED.);
#9948=B_SPLINE_CURVE_WITH_KNOTS('',3,(#74402,#74403,#74404,#74405),
 .UNSPECIFIED.,.F.,.F.,(4,4),(-0.0458781805671202,0.),.UNSPECIFIED.);
#9949=B_SPLINE_CURVE_WITH_KNOTS('',3,(#74407,#74408,#74409,#74410),
 .UNSPECIFIED.,.F.,.F.,(4,4),(0.,0.0458781805671202),.UNSPECIFIED.);
#9950=B_SPLINE_CURVE_WITH_KNOTS('',3,(#74416,#74417,#74418,#74419,#74420,
#74421,#74422,#74423,#74424,#74425,#74426,#74427,#74428,#74429),
 .UNSPECIFIED.,.F.,.F.,(4,2,2,2,2,2,4),(-0.112045619239962,-0.11061169371515,
-0.0954349222053137,-0.0802581506954778,-0.0677819987765266,-0.0615439228170509,
-0.0553058468575753),.UNSPECIFIED.);
#9951=B_SPLINE_CURVE_WITH_KNOTS('',3,(#74443,#74444,#74445,#74446),
 .UNSPECIFIED.,.F.,.F.,(4,4),(-0.0458781805667708,0.),.UNSPECIFIED.);
#9952=B_SPLINE_CURVE_WITH_KNOTS('',3,(#74485,#74486,#74487,#74488),
 .UNSPECIFIED.,.F.,.F.,(4,4),(-0.045878180567117,0.),.UNSPECIFIED.);
#9953=B_SPLINE_CURVE_WITH_KNOTS('',3,(#74490,#74491,#74492,#74493),
 .UNSPECIFIED.,.F.,.F.,(4,4),(0.,0.045878180567117),.UNSPECIFIED.);
#9954=B_SPLINE_CURVE_WITH_KNOTS('',3,(#74499,#74500,#74501,#74502,#74503,
#74504,#74505,#74506,#74507,#74508,#74509,#74510,#74511,#74512),
 .UNSPECIFIED.,.F.,.F.,(4,2,2,2,2,2,4),(-0.112045619239961,-0.110611693715149,
-0.0954349222053133,-0.0802581506954775,-0.0677819987765261,-0.0615439228170503,
-0.0553058468575746),.UNSPECIFIED.);
#9955=B_SPLINE_CURVE_WITH_KNOTS('',3,(#74526,#74527,#74528,#74529),
 .UNSPECIFIED.,.F.,.F.,(4,4),(-0.045878180566557,0.),.UNSPECIFIED.);
#9956=B_SPLINE_CURVE_WITH_KNOTS('',3,(#74560,#74561,#74562,#74563),
 .UNSPECIFIED.,.F.,.F.,(4,4),(-0.0458781805671145,0.),.UNSPECIFIED.);
#9957=B_SPLINE_CURVE_WITH_KNOTS('',3,(#74565,#74566,#74567,#74568),
 .UNSPECIFIED.,.F.,.F.,(4,4),(0.,0.0458781805671145),.UNSPECIFIED.);
#9958=B_SPLINE_CURVE_WITH_KNOTS('',3,(#74574,#74575,#74576,#74577,#74578,
#74579,#74580,#74581,#74582,#74583,#74584,#74585,#74586,#74587),
 .UNSPECIFIED.,.F.,.F.,(4,2,2,2,2,2,4),(-0.11204561923996,-0.110611693715147,
-0.0954349222053113,-0.0802581506954755,-0.0677819987765246,-0.0615439228170492,
-0.0553058468575738),.UNSPECIFIED.);
#9959=B_SPLINE_CURVE_WITH_KNOTS('',3,(#74601,#74602,#74603,#74604),
 .UNSPECIFIED.,.F.,.F.,(4,4),(-0.0458781805667346,0.),.UNSPECIFIED.);
#9960=B_SPLINE_CURVE_WITH_KNOTS('',3,(#74643,#74644,#74645,#74646),
 .UNSPECIFIED.,.F.,.F.,(4,4),(-0.0458781805671221,0.),.UNSPECIFIED.);
#9961=B_SPLINE_CURVE_WITH_KNOTS('',3,(#74648,#74649,#74650,#74651),
 .UNSPECIFIED.,.F.,.F.,(4,4),(0.,0.0458781805671221),.UNSPECIFIED.);
#9962=B_SPLINE_CURVE_WITH_KNOTS('',3,(#74657,#74658,#74659,#74660,#74661,
#74662,#74663,#74664,#74665,#74666,#74667,#74668,#74669,#74670),
 .UNSPECIFIED.,.F.,.F.,(4,2,2,2,2,2,4),(-0.112045619239961,-0.110611693715149,
-0.0954349222053122,-0.080258150695475,-0.0677819987765244,-0.0615439228170491,
-0.0553058468575737),.UNSPECIFIED.);
#9963=B_SPLINE_CURVE_WITH_KNOTS('',3,(#74684,#74685,#74686,#74687),
 .UNSPECIFIED.,.F.,.F.,(4,4),(-0.0458781805667396,0.),.UNSPECIFIED.);
#9964=B_SPLINE_CURVE_WITH_KNOTS('',3,(#74726,#74727,#74728,#74729),
 .UNSPECIFIED.,.F.,.F.,(4,4),(-0.045878180567114,0.),.UNSPECIFIED.);
#9965=B_SPLINE_CURVE_WITH_KNOTS('',3,(#74731,#74732,#74733,#74734),
 .UNSPECIFIED.,.F.,.F.,(4,4),(0.,0.045878180567114),.UNSPECIFIED.);
#9966=B_SPLINE_CURVE_WITH_KNOTS('',3,(#74740,#74741,#74742,#74743,#74744,
#74745,#74746,#74747,#74748,#74749,#74750,#74751,#74752,#74753),
 .UNSPECIFIED.,.F.,.F.,(4,2,2,2,2,2,4),(-0.11204561923996,-0.110611693715147,
-0.0954349222053111,-0.0802581506954753,-0.0677819987765242,-0.0615439228170486,
-0.055305846857573),.UNSPECIFIED.);
#9967=B_SPLINE_CURVE_WITH_KNOTS('',3,(#74767,#74768,#74769,#74770),
 .UNSPECIFIED.,.F.,.F.,(4,4),(-0.045878180566732,0.),.UNSPECIFIED.);
#9968=B_SPLINE_CURVE_WITH_KNOTS('',3,(#74795,#74796,#74797,#74798),
 .UNSPECIFIED.,.F.,.F.,(4,4),(0.,0.045878180566732),.UNSPECIFIED.);
#9969=B_SPLINE_CURVE_WITH_KNOTS('',3,(#74816,#74817,#74818,#74819,#74820,
#74821),.UNSPECIFIED.,.F.,.F.,(4,2,4),(0.0222170009937299,0.0333260526322421,
0.0444418875612832),.UNSPECIFIED.);
#9970=B_SPLINE_CURVE_WITH_KNOTS('',3,(#74847,#74848,#74849,#74850),
 .UNSPECIFIED.,.F.,.F.,(4,4),(0.,0.0458781805667396),.UNSPECIFIED.);
#9971=B_SPLINE_CURVE_WITH_KNOTS('',3,(#74864,#74865,#74866,#74867,#74868,
#74869),.UNSPECIFIED.,.F.,.F.,(4,2,4),(0.0222170009937325,0.0333260526322431,
0.0444418875612845),.UNSPECIFIED.);
#9972=B_SPLINE_CURVE_WITH_KNOTS('',3,(#74895,#74896,#74897,#74898),
 .UNSPECIFIED.,.F.,.F.,(4,4),(0.,0.0458781805667346),.UNSPECIFIED.);
#9973=B_SPLINE_CURVE_WITH_KNOTS('',3,(#74912,#74913,#74914,#74915,#74916,
#74917),.UNSPECIFIED.,.F.,.F.,(4,2,4),(0.0222170009937307,0.0333260526322433,
0.0444418875612841),.UNSPECIFIED.);
#9974=B_SPLINE_CURVE_WITH_KNOTS('',3,(#74943,#74944,#74945,#74946),
 .UNSPECIFIED.,.F.,.F.,(4,4),(0.,0.045878180566557),.UNSPECIFIED.);
#9975=B_SPLINE_CURVE_WITH_KNOTS('',3,(#74964,#74965,#74966,#74967,#74968,
#74969),.UNSPECIFIED.,.F.,.F.,(4,2,4),(0.0222170009937318,0.0333260526322424,
0.0444418875612825),.UNSPECIFIED.);
#9976=B_SPLINE_CURVE_WITH_KNOTS('',3,(#74974,#74975,#74976,#74977,#74978,
#74979,#74980,#74981,#74982,#74983,#74984,#74985,#74986,#74987),
 .UNSPECIFIED.,.F.,.F.,(4,2,2,2,2,2,4),(-0.112045619239963,-0.110611693715149,
-0.0954349222053129,-0.0802581506954765,-0.0677819987765254,-0.0615439228170499,
-0.0553058468575743),.UNSPECIFIED.);
#9977=B_SPLINE_CURVE_WITH_KNOTS('',3,(#74991,#74992,#74993,#74994,#74995,
#74996,#74997,#74998,#74999,#75000,#75001,#75002,#75003,#75004),
 .UNSPECIFIED.,.F.,.F.,(4,2,2,2,2,2,4),(0.0553058468575743,0.0615439228170499,
0.0677819987765254,0.0802581506954765,0.0954349222053129,0.110611693715149,
0.112045606679732),.UNSPECIFIED.);
#9978=B_SPLINE_CURVE_WITH_KNOTS('',3,(#75014,#75015,#75016,#75017,#75018,
#75019,#75020,#75021,#75022,#75023,#75024,#75025,#75026,#75027),
 .UNSPECIFIED.,.F.,.F.,(4,2,2,2,2,2,4),(0.0553058468575735,0.061543922817049,
0.0677819987765245,0.0802581506954754,0.0954349222053113,0.110611693715147,
0.112045606679731),.UNSPECIFIED.);
#9979=B_SPLINE_CURVE_WITH_KNOTS('',3,(#75032,#75033,#75034,#75035,#75036,
#75037),.UNSPECIFIED.,.F.,.F.,(4,2,4),(0.133326015406808,0.144441850335849,
0.155550901974358),.UNSPECIFIED.);
#9980=B_SPLINE_CURVE_WITH_KNOTS('',3,(#75043,#75044,#75045,#75046,#75047,
#75048),.UNSPECIFIED.,.F.,.F.,(4,2,4),(0.0222170009937292,0.0333260526322429,
0.0444418875612827),.UNSPECIFIED.);
#9981=B_SPLINE_CURVE_WITH_KNOTS('',3,(#75073,#75074,#75075,#75076),
 .UNSPECIFIED.,.F.,.F.,(4,4),(0.,0.0458781805667708),.UNSPECIFIED.);
#9982=B_SPLINE_CURVE_WITH_KNOTS('',3,(#75090,#75091,#75092,#75093,#75094,
#75095),.UNSPECIFIED.,.F.,.F.,(4,2,4),(0.0222170009937321,0.033326052632243,
0.0444418875612839),.UNSPECIFIED.);
#9983=B_SPLINE_CURVE_WITH_KNOTS('',3,(#75127,#75128,#75129,#75130),
 .UNSPECIFIED.,.F.,.F.,(4,4),(-0.0458781805671245,0.),.UNSPECIFIED.);
#9984=B_SPLINE_CURVE_WITH_KNOTS('',3,(#75132,#75133,#75134,#75135),
 .UNSPECIFIED.,.F.,.F.,(4,4),(0.,0.0458781805671245),.UNSPECIFIED.);
#9985=B_SPLINE_CURVE_WITH_KNOTS('',3,(#75141,#75142,#75143,#75144,#75145,
#75146,#75147,#75148,#75149,#75150,#75151,#75152,#75153,#75154),
 .UNSPECIFIED.,.F.,.F.,(4,2,2,2,2,2,4),(-0.112045619239962,-0.110611693715149,
-0.0954349222053127,-0.0802581506954767,-0.0677819987765257,-0.0615439228170502,
-0.0553058468575746),.UNSPECIFIED.);
#9986=B_SPLINE_CURVE_WITH_KNOTS('',3,(#75168,#75169,#75170,#75171),
 .UNSPECIFIED.,.F.,.F.,(4,4),(-0.0458781805667809,0.),.UNSPECIFIED.);
#9987=B_SPLINE_CURVE_WITH_KNOTS('',3,(#75223,#75224,#75225,#75226),
 .UNSPECIFIED.,.F.,.F.,(4,4),(0.,0.0458781805667809),.UNSPECIFIED.);
#9988=B_SPLINE_CURVE_WITH_KNOTS('',3,(#75244,#75245,#75246,#75247,#75248,
#75249),.UNSPECIFIED.,.F.,.F.,(4,2,4),(0.0222170009937322,0.0333260526322429,
0.0444418875612822),.UNSPECIFIED.);
#9989=B_SPLINE_CURVE_WITH_KNOTS('',3,(#75253,#75254,#75255,#75256,#75257,
#75258,#75259,#75260,#75261,#75262,#75263,#75264,#75265,#75266),
 .UNSPECIFIED.,.F.,.F.,(4,2,2,2,2,2,4),(0.0553058468575756,0.0615439228170508,
0.0677819987765261,0.0802581506954766,0.0954349222053132,0.11061169371515,
0.112045606679733),.UNSPECIFIED.);
#9990=B_SPLINE_CURVE_WITH_KNOTS('',3,(#75271,#75272,#75273,#75274,#75275,
#75276),.UNSPECIFIED.,.F.,.F.,(4,2,4),(0.133326015406808,0.144441850335848,
0.15555090197436),.UNSPECIFIED.);
#9991=B_SPLINE_CURVE_WITH_KNOTS('',3,(#75282,#75283,#75284,#75285,#75286,
#75287),.UNSPECIFIED.,.F.,.F.,(4,2,4),(0.0222170009937338,0.0333260526322426,
0.0444418875612839),.UNSPECIFIED.);
#9992=B_SPLINE_CURVE_WITH_KNOTS('',3,(#75320,#75321,#75322,#75323),
 .UNSPECIFIED.,.F.,.F.,(4,4),(0.0848913392683917,0.130769519836251),
 .UNSPECIFIED.);
#9993=B_SPLINE_CURVE_WITH_KNOTS('',3,(#75326,#75327,#75328,#75329),
 .UNSPECIFIED.,.F.,.F.,(4,4),(-0.130769519836251,-0.0848913392683917),
 .UNSPECIFIED.);
#9994=B_SPLINE_CURVE_WITH_KNOTS('',3,(#75336,#75337,#75338,#75339),
 .UNSPECIFIED.,.F.,.F.,(4,4),(0.,0.0458781805664131),.UNSPECIFIED.);
#9995=B_SPLINE_CURVE_WITH_KNOTS('',3,(#75343,#75344,#75345,#75346,#75347,
#75348),.UNSPECIFIED.,.F.,.F.,(4,2,4),(0.0222170009937356,0.0333260526322432,
0.0444418875612838),.UNSPECIFIED.);
#9996=B_SPLINE_CURVE_WITH_KNOTS('',3,(#75361,#75362,#75363,#75364,#75365,
#75366),.UNSPECIFIED.,.F.,.F.,(4,2,4),(0.133326015406807,0.144441850335847,
0.155550901974362),.UNSPECIFIED.);
#9997=B_SPLINE_CURVE_WITH_KNOTS('',3,(#75370,#75371,#75372,#75373,#75374,
#75375,#75376,#75377,#75378,#75379,#75380,#75381,#75382,#75383),
 .UNSPECIFIED.,.F.,.F.,(4,2,2,2,2,2,4),(0.055305846857574,0.0615439228170492,
0.0677819987765245,0.0802581506954751,0.0954349222053116,0.110611693715148,
0.11204560667973),.UNSPECIFIED.);
#9998=B_SPLINE_CURVE_WITH_KNOTS('',3,(#75388,#75389,#75390,#75391,#75392,
#75393),.UNSPECIFIED.,.F.,.F.,(4,2,4),(0.133326015406808,0.144441850335849,
0.155550901974361),.UNSPECIFIED.);
#9999=B_SPLINE_CURVE_WITH_KNOTS('',3,(#75416,#75417,#75418,#75419,#75420,
#75421),.UNSPECIFIED.,.F.,.F.,(4,2,4),(0.133326015406807,0.144441850335846,
0.155550901974357),.UNSPECIFIED.);
#10000=B_SPLINE_CURVE_WITH_KNOTS('',3,(#75426,#75427,#75428,#75429,#75430,
#75431),.UNSPECIFIED.,.F.,.F.,(4,2,4),(0.0222170009937315,0.0333260526322426,
0.0444418875612843),.UNSPECIFIED.);
#10001=B_SPLINE_CURVE_WITH_KNOTS('',3,(#75438,#75439,#75440,#75441,#75442,
#75443,#75444,#75445,#75446,#75447,#75448,#75449,#75450,#75451),
 .UNSPECIFIED.,.F.,.F.,(4,2,2,2,2,2,4),(0.0553058468575743,0.0615439228170494,
0.0677819987765245,0.0802581506954748,0.095434922205311,0.110611693715147,
0.112045606679731),.UNSPECIFIED.);
#10002=B_SPLINE_CURVE_WITH_KNOTS('',3,(#75456,#75457,#75458,#75459,#75460,
#75461),.UNSPECIFIED.,.F.,.F.,(4,2,4),(0.133326015406808,0.144441850335849,
0.155550901974359),.UNSPECIFIED.);
#10003=B_SPLINE_CURVE_WITH_KNOTS('',3,(#75478,#75479,#75480,#75481,#75482,
#75483),.UNSPECIFIED.,.F.,.F.,(4,2,4),(0.133326015406806,0.144441850335847,
0.15555090197436),.UNSPECIFIED.);
#10004=B_SPLINE_CURVE_WITH_KNOTS('',3,(#75495,#75496,#75497,#75498,#75499,
#75500,#75501,#75502,#75503,#75504,#75505,#75506,#75507,#75508),
 .UNSPECIFIED.,.F.,.F.,(4,2,2,2,2,2,4),(0.0553058468575742,0.0615439228170496,
0.067781998776525,0.0802581506954758,0.0954349222053118,0.110611693715148,
0.112045606679732),.UNSPECIFIED.);
#10005=B_SPLINE_CURVE_WITH_KNOTS('',3,(#75513,#75514,#75515,#75516,#75517,
#75518),.UNSPECIFIED.,.F.,.F.,(4,2,4),(0.133326015406809,0.144441850335849,
0.155550901974358),.UNSPECIFIED.);
#10006=B_SPLINE_CURVE_WITH_KNOTS('',3,(#75546,#75547,#75548,#75549),
 .UNSPECIFIED.,.F.,.F.,(4,4),(0.,0.045878180566409),.UNSPECIFIED.);
#10007=B_SPLINE_CURVE_WITH_KNOTS('',3,(#75584,#75585,#75586,#75587,#75588,
#75589),.UNSPECIFIED.,.F.,.F.,(4,2,4),(0.133326015406807,0.144441850335848,
0.15555090197436),.UNSPECIFIED.);
#10008=B_SPLINE_CURVE_WITH_KNOTS('',3,(#75593,#75594,#75595,#75596,#75597,
#75598,#75599,#75600,#75601,#75602,#75603,#75604,#75605,#75606),
 .UNSPECIFIED.,.F.,.F.,(4,2,2,2,2,2,4),(0.0553058468575746,0.0615439228170503,
0.067781998776526,0.0802581506954775,0.0954349222053132,0.110611693715149,
0.112045606679734),.UNSPECIFIED.);
#10009=B_SPLINE_CURVE_WITH_KNOTS('',3,(#75611,#75612,#75613,#75614,#75615,
#75616),.UNSPECIFIED.,.F.,.F.,(4,2,4),(0.133326015406808,0.144441850335849,
0.155550901974361),.UNSPECIFIED.);
#10010=B_SPLINE_CURVE_WITH_KNOTS('',3,(#75632,#75633,#75634,#75635,#75636,
#75637),.UNSPECIFIED.,.F.,.F.,(4,2,4),(0.0222170009937321,0.033326052632243,
0.0444418875612839),.UNSPECIFIED.);
#10011=B_SPLINE_CURVE_WITH_KNOTS('',3,(#75649,#75650,#75651,#75652,#75653,
#75654),.UNSPECIFIED.,.F.,.F.,(4,2,4),(0.133326015406807,0.144441850335848,
0.155550901974356),.UNSPECIFIED.);
#10012=B_SPLINE_CURVE_WITH_KNOTS('',3,(#75658,#75659,#75660,#75661,#75662,
#75663),.UNSPECIFIED.,.F.,.F.,(4,2,4),(0.0222170009937305,0.0333260526322427,
0.0444418875612838),.UNSPECIFIED.);
#10013=B_SPLINE_CURVE_WITH_KNOTS('',3,(#75671,#75672,#75673,#75674,#75675,
#75676,#75677,#75678,#75679,#75680,#75681,#75682,#75683,#75684),
 .UNSPECIFIED.,.F.,.F.,(4,2,2,2,2,2,4),(0.0553058468575755,0.0615439228170512,
0.0677819987765268,0.0802581506954781,0.0954349222053139,0.11061169371515,
0.112045606679733),.UNSPECIFIED.);
#10014=B_SPLINE_CURVE_WITH_KNOTS('',3,(#75689,#75690,#75691,#75692,#75693,
#75694),.UNSPECIFIED.,.F.,.F.,(4,2,4),(0.133326015406808,0.144441850335849,
0.155550901974359),.UNSPECIFIED.);
#10015=B_SPLINE_CURVE_WITH_KNOTS('',3,(#75711,#75712,#75713,#75714,#75715,
#75716),.UNSPECIFIED.,.F.,.F.,(4,2,4),(0.133326015406807,0.144441850335847,
0.15555090197436),.UNSPECIFIED.);
#10016=B_SPLINE_CURVE_WITH_KNOTS('',3,(#75728,#75729,#75730,#75731,#75732,
#75733,#75734,#75735,#75736,#75737,#75738,#75739,#75740,#75741),
 .UNSPECIFIED.,.F.,.F.,(4,2,2,2,2,2,4),(0.0553058468575741,0.0615439228170494,
0.0677819987765246,0.0802581506954752,0.0954349222053117,0.110611693715148,
0.112045606679732),.UNSPECIFIED.);
#10017=B_SPLINE_CURVE_WITH_KNOTS('',3,(#75746,#75747,#75748,#75749,#75750,
#75751),.UNSPECIFIED.,.F.,.F.,(4,2,4),(0.133326015406808,0.14444185033585,
0.155550901974359),.UNSPECIFIED.);
#10018=B_SPLINE_CURVE_WITH_KNOTS('',3,(#75779,#75780,#75781,#75782),
 .UNSPECIFIED.,.F.,.F.,(4,4),(0.,0.0458781805664144),.UNSPECIFIED.);
#10019=B_SPLINE_CURVE_WITH_KNOTS('',3,(#75809,#75810,#75811,#75812,#75813,
#75814),.UNSPECIFIED.,.F.,.F.,(4,2,4),(0.0222170009937364,0.0333260526322433,
0.044441887561284),.UNSPECIFIED.);
#10020=B_SPLINE_CURVE_WITH_KNOTS('',3,(#75827,#75828,#75829,#75830,#75831,
#75832),.UNSPECIFIED.,.F.,.F.,(4,2,4),(0.133326015406808,0.144441850335847,
0.155550901974361),.UNSPECIFIED.);
#10021=B_SPLINE_CURVE_WITH_KNOTS('',3,(#75836,#75837,#75838,#75839,#75840,
#75841,#75842,#75843,#75844,#75845,#75846,#75847,#75848,#75849),
 .UNSPECIFIED.,.F.,.F.,(4,2,2,2,2,2,4),(0.0553058468575744,0.0615439228170498,
0.0677819987765252,0.0802581506954761,0.0954349222053126,0.110611693715149,
0.112045606679734),.UNSPECIFIED.);
#10022=B_SPLINE_CURVE_WITH_KNOTS('',3,(#75854,#75855,#75856,#75857,#75858,
#75859),.UNSPECIFIED.,.F.,.F.,(4,2,4),(0.133326015406808,0.144441850335849,
0.155550901974361),.UNSPECIFIED.);
#10023=B_SPLINE_CURVE_WITH_KNOTS('',3,(#75882,#75883,#75884,#75885,#75886,
#75887),.UNSPECIFIED.,.F.,.F.,(4,2,4),(0.133326015406808,0.144441850335848,
0.15555090197436),.UNSPECIFIED.);
#10024=B_SPLINE_CURVE_WITH_KNOTS('',3,(#75897,#75898,#75899,#75900,#75901,
#75902,#75903,#75904,#75905,#75906,#75907,#75908,#75909,#75910),
 .UNSPECIFIED.,.F.,.F.,(4,2,2,2,2,2,4),(0.0553058468575734,0.0615439228170488,
0.0677819987765242,0.0802581506954749,0.0954349222053108,0.110611693715147,
0.112045606679731),.UNSPECIFIED.);
#10025=B_SPLINE_CURVE_WITH_KNOTS('',3,(#75915,#75916,#75917,#75918,#75919,
#75920),.UNSPECIFIED.,.F.,.F.,(4,2,4),(0.133326015406808,0.144441850335849,
0.155550901974358),.UNSPECIFIED.);
#10026=B_SPLINE_CURVE_WITH_KNOTS('',3,(#75937,#75938,#75939,#75940,#75941,
#75942),.UNSPECIFIED.,.F.,.F.,(4,2,4),(0.133326015406807,0.144441850335846,
0.155550901974359),.UNSPECIFIED.);
#10027=B_SPLINE_CURVE_WITH_KNOTS('',3,(#75954,#75955,#75956,#75957,#75958,
#75959,#75960,#75961,#75962,#75963,#75964,#75965,#75966,#75967),
 .UNSPECIFIED.,.F.,.F.,(4,2,2,2,2,2,4),(0.0553058468575744,0.0615439228170499,
0.0677819987765254,0.0802581506954763,0.0954349222053129,0.110611693715149,
0.112045606679734),.UNSPECIFIED.);
#10028=B_SPLINE_CURVE_WITH_KNOTS('',3,(#75972,#75973,#75974,#75975,#75976,
#75977),.UNSPECIFIED.,.F.,.F.,(4,2,4),(0.133326015406808,0.14444185033585,
0.155550901974361),.UNSPECIFIED.);
#10029=B_SPLINE_CURVE_WITH_KNOTS('',3,(#76005,#76006,#76007,#76008),
 .UNSPECIFIED.,.F.,.F.,(4,4),(0.,0.045878180566409),.UNSPECIFIED.);
#10030=B_SPLINE_CURVE_WITH_KNOTS('',3,(#76034,#76035,#76036,#76037,#76038,
#76039,#76040,#76041,#76042,#76043,#76044,#76045,#76046,#76047),
 .UNSPECIFIED.,.F.,.F.,(4,2,2,2,2,2,4),(0.0553058468575743,0.06154392281705,
0.0677819987765257,0.0802581506954771,0.0954349222053129,0.110611693715149,
0.112045606679733),.UNSPECIFIED.);
#10031=B_SPLINE_CURVE_WITH_KNOTS('',3,(#76052,#76053,#76054,#76055,#76056,
#76057),.UNSPECIFIED.,.F.,.F.,(4,2,4),(0.133326015406808,0.144441850335849,
0.155550901974357),.UNSPECIFIED.);
#10032=B_SPLINE_CURVE_WITH_KNOTS('',3,(#76085,#76086,#76087,#76088),
 .UNSPECIFIED.,.F.,.F.,(4,4),(0.,0.0458781805665586),.UNSPECIFIED.);
#10033=B_SPLINE_CURVE_WITH_KNOTS('',3,(#76108,#76109,#76110,#76111,#76112,
#76113),.UNSPECIFIED.,.F.,.F.,(4,2,4),(0.0222170009937305,0.0333260526322418,
0.0444418875612824),.UNSPECIFIED.);
#10034=B_SPLINE_CURVE_WITH_KNOTS('',3,(#76120,#76121,#76122,#76123,#76124,
#76125),.UNSPECIFIED.,.F.,.F.,(4,2,4),(0.133326015406808,0.144441850335847,
0.155550901974361),.UNSPECIFIED.);
#10035=B_SPLINE_CURVE_WITH_KNOTS('',3,(#76148,#76149,#76150,#76151,#76152,
#76153),.UNSPECIFIED.,.F.,.F.,(4,2,4),(0.133326015406807,0.144441850335848,
0.155550901974362),.UNSPECIFIED.);
#10036=B_SPLINE_CURVE_WITH_KNOTS('',3,(#76157,#76158,#76159,#76160,#76161,
#76162),.UNSPECIFIED.,.F.,.F.,(4,2,4),(0.0222170009937301,0.0333260526322426,
0.0444418875612843),.UNSPECIFIED.);
#10037=B_SPLINE_CURVE_WITH_KNOTS('',3,(#76166,#76167,#76168,#76169,#76170,
#76171,#76172,#76173,#76174,#76175,#76176,#76177,#76178,#76179),
 .UNSPECIFIED.,.F.,.F.,(4,2,2,2,2,2,4),(0.0553058468575755,0.061543922817051,
0.0677819987765266,0.0802581506954776,0.0954349222053134,0.110611693715149,
0.112045606679735),.UNSPECIFIED.);
#10038=B_SPLINE_CURVE_WITH_KNOTS('',3,(#76184,#76185,#76186,#76187,#76188,
#76189),.UNSPECIFIED.,.F.,.F.,(4,2,4),(0.133326015406808,0.144441850335849,
0.15555090197436),.UNSPECIFIED.);
#10039=B_SPLINE_CURVE_WITH_KNOTS('',3,(#76210,#76211,#76212,#76213,#76214,
#76215),.UNSPECIFIED.,.F.,.F.,(4,2,4),(0.133326015406807,0.144441850335848,
0.155550901974361),.UNSPECIFIED.);
#10040=B_SPLINE_CURVE_WITH_KNOTS('',3,(#76247,#76248,#76249,#76250),
 .UNSPECIFIED.,.F.,.F.,(4,4),(-0.0458781805670896,0.),.UNSPECIFIED.);
#10041=B_SPLINE_CURVE_WITH_KNOTS('',3,(#76252,#76253,#76254,#76255),
 .UNSPECIFIED.,.F.,.F.,(4,4),(0.,0.0458781805670896),.UNSPECIFIED.);
#10042=B_SPLINE_CURVE_WITH_KNOTS('',3,(#76266,#76267,#76268,#76269,#76270,
#76271,#76272,#76273,#76274,#76275),.UNSPECIFIED.,.F.,.F.,(4,2,2,2,4),(0.108010287307675,
0.109444200272932,0.124620971782768,0.139797743292605,0.139840101164973),
 .UNSPECIFIED.);
#10043=B_SPLINE_CURVE_WITH_KNOTS('',3,(#76276,#76277,#76278,#76279,#76280,
#76281,#76282,#76283),.UNSPECIFIED.,.F.,.F.,(4,2,2,4),(-0.0323450549294852,
-0.0153026771617381,0.,0.000347076601513913),.UNSPECIFIED.);
#10044=B_SPLINE_CURVE_WITH_KNOTS('',3,(#76300,#76301,#76302,#76303),
 .UNSPECIFIED.,.F.,.F.,(4,4),(-0.0458781805664131,0.),.UNSPECIFIED.);
#10045=B_SPLINE_CURVE_WITH_KNOTS('',3,(#76348,#76349,#76350,#76351),
 .UNSPECIFIED.,.F.,.F.,(4,4),(-0.0458781805670864,0.),.UNSPECIFIED.);
#10046=B_SPLINE_CURVE_WITH_KNOTS('',3,(#76353,#76354,#76355,#76356),
 .UNSPECIFIED.,.F.,.F.,(4,4),(0.,0.0458781805670864),.UNSPECIFIED.);
#10047=B_SPLINE_CURVE_WITH_KNOTS('',3,(#76367,#76368,#76369,#76370,#76371,
#76372,#76373,#76374),.UNSPECIFIED.,.F.,.F.,(4,2,2,4),(-0.000347076601507095,
0.,0.0153026771617058,0.032345054929495),.UNSPECIFIED.);
#10048=B_SPLINE_CURVE_WITH_KNOTS('',3,(#76381,#76382,#76383,#76384,#76385,
#76386,#76387,#76388,#76389,#76390),.UNSPECIFIED.,.F.,.F.,(4,2,2,2,4),(-0.112045606680405,
-0.110611693715149,-0.0954349222053128,-0.0802581506954763,-0.0802157928231077),
 .UNSPECIFIED.);
#10049=B_SPLINE_CURVE_WITH_KNOTS('',3,(#76416,#76417,#76418,#76419),
 .UNSPECIFIED.,.F.,.F.,(4,4),(-0.0458781805664134,0.),.UNSPECIFIED.);
#10050=B_SPLINE_CURVE_WITH_KNOTS('',3,(#76421,#76422,#76423,#76424),
 .UNSPECIFIED.,.F.,.F.,(4,4),(0.,0.0458781805664134),.UNSPECIFIED.);
#10051=B_SPLINE_CURVE_WITH_KNOTS('',3,(#76441,#76442,#76443,#76444),
 .UNSPECIFIED.,.F.,.F.,(4,4),(0.,0.0883236961657942),.UNSPECIFIED.);
#10052=B_SPLINE_CURVE_WITH_KNOTS('',3,(#76448,#76449,#76450,#76451,#76452,
#76453),.UNSPECIFIED.,.F.,.F.,(4,2,4),(0.0222170009937288,0.0333260526322424,
0.044441887561283),.UNSPECIFIED.);
#10053=B_SPLINE_CURVE_WITH_KNOTS('',3,(#76459,#76460,#76461,#76462,#76463,
#76464,#76465,#76466),.UNSPECIFIED.,.F.,.F.,(4,2,2,4),(-0.0311981661884286,
-0.0308963070644515,-0.0149763680894757,0.),.UNSPECIFIED.);
#10054=B_SPLINE_CURVE_WITH_KNOTS('',3,(#76488,#76489,#76490,#76491),
 .UNSPECIFIED.,.F.,.F.,(4,4),(-0.0458781805671567,0.),.UNSPECIFIED.);
#10055=B_SPLINE_CURVE_WITH_KNOTS('',3,(#76544,#76545,#76546,#76547,#76548,
#76549,#76550,#76551),.UNSPECIFIED.,.F.,.F.,(4,2,2,4),(-0.0311981661886286,
-0.0308963070644535,-0.0149763680894719,0.),.UNSPECIFIED.);
#10056=B_SPLINE_CURVE_WITH_KNOTS('',3,(#76573,#76574,#76575,#76576),
 .UNSPECIFIED.,.F.,.F.,(4,4),(-0.0458781805671511,0.),.UNSPECIFIED.);
#10057=B_SPLINE_CURVE_WITH_KNOTS('',3,(#76585,#76586,#76587,#76588,#76589,
#76590,#76591,#76592),.UNSPECIFIED.,.F.,.F.,(4,2,2,4),(-0.0311981661875462,
-0.0308963070636882,-0.0149763680894736,0.),.UNSPECIFIED.);
#10058=B_SPLINE_CURVE_WITH_KNOTS('',3,(#76614,#76615,#76616,#76617),
 .UNSPECIFIED.,.F.,.F.,(4,4),(-0.0458781805671518,0.),.UNSPECIFIED.);
#10059=B_SPLINE_CURVE_WITH_KNOTS('',3,(#76654,#76655,#76656,#76657,#76658,
#76659,#76660,#76661,#76662,#76663,#76664,#76665,#76666,#76667),
 .UNSPECIFIED.,.F.,.F.,(4,2,2,2,2,2,4),(0.0553058468575744,0.0615439228170497,
0.0677819987765251,0.0802581506954758,0.0954349222053117,0.110611693715148,
0.112045606679733),.UNSPECIFIED.);
#10060=B_SPLINE_CURVE_WITH_KNOTS('',3,(#76685,#76686,#76687,#76688,#76689,
#76690,#76691,#76692,#76693,#76694,#76695,#76696,#76697,#76698),
 .UNSPECIFIED.,.F.,.F.,(4,2,2,2,2,2,4),(0.0553058468575743,0.0615439228170501,
0.0677819987765258,0.0802581506954773,0.0954349222053131,0.110611693715149,
0.112045606679733),.UNSPECIFIED.);
#10061=B_SPLINE_CURVE_WITH_KNOTS('',3,(#76711,#76712,#76713,#76714,#76715,
#76716,#76717,#76718,#76719,#76720,#76721,#76722,#76723,#76724),
 .UNSPECIFIED.,.F.,.F.,(4,2,2,2,2,2,4),(0.0553058468575743,0.0615439228170499,
0.0677819987765255,0.0802581506954768,0.0954349222053127,0.110611693715149,
0.112045606679732),.UNSPECIFIED.);
#10062=B_SPLINE_CURVE_WITH_KNOTS('',3,(#76749,#76750,#76751,#76752,#76753,
#76754,#76755,#76756,#76757,#76758,#76759,#76760,#76761,#76762),
 .UNSPECIFIED.,.F.,.F.,(4,2,2,2,2,2,4),(0.0553058468575743,0.0615439228170498,
0.0677819987765253,0.0802581506954762,0.0954349222053121,0.110611693715148,
0.112045606679733),.UNSPECIFIED.);
#10063=B_SPLINE_CURVE_WITH_KNOTS('',3,(#76775,#76776,#76777,#76778,#76779,
#76780,#76781,#76782,#76783,#76784,#76785,#76786,#76787,#76788),
 .UNSPECIFIED.,.F.,.F.,(4,2,2,2,2,2,4),(0.0553058468575731,0.0615439228170486,
0.067781998776524,0.0802581506954749,0.0954349222053116,0.110611693715148,
0.112045606679732),.UNSPECIFIED.);
#10064=B_SPLINE_CURVE_WITH_KNOTS('',3,(#76801,#76802,#76803,#76804,#76805,
#76806,#76807,#76808,#76809,#76810,#76811,#76812,#76813,#76814),
 .UNSPECIFIED.,.F.,.F.,(4,2,2,2,2,2,4),(0.0553058468575733,0.0615439228170484,
0.0677819987765236,0.0802581506954739,0.0954349222053105,0.110611693715147,
0.112045606679735),.UNSPECIFIED.);
#10065=B_SPLINE_CURVE_WITH_KNOTS('',3,(#76839,#76840,#76841,#76842,#76843,
#76844,#76845,#76846,#76847,#76848,#76849,#76850,#76851,#76852),
 .UNSPECIFIED.,.F.,.F.,(4,2,2,2,2,2,4),(0.0553058468575745,0.0615439228170501,
0.0677819987765257,0.0802581506954769,0.0954349222053128,0.110611693715149,
0.112045606679734),.UNSPECIFIED.);
#10066=B_SPLINE_CURVE_WITH_KNOTS('',3,(#76870,#76871,#76872,#76873,#76874,
#76875,#76876,#76877,#76878,#76879,#76880,#76881,#76882,#76883),
 .UNSPECIFIED.,.F.,.F.,(4,2,2,2,2,2,4),(0.0553058468575747,0.0615439228170501,
0.0677819987765255,0.0802581506954763,0.0954349222053129,0.110611693715149,
0.112045606679733),.UNSPECIFIED.);
#10067=B_SPLINE_CURVE_WITH_KNOTS('',3,(#76898,#76899,#76900,#76901,#76902,
#76903,#76904,#76905,#76906,#76907,#76908,#76909,#76910,#76911),
 .UNSPECIFIED.,.F.,.F.,(4,2,2,2,2,2,4),(0.0553058468575749,0.0615439228170505,
0.067781998776526,0.080258150695477,0.0954349222053134,0.11061169371515,
0.112045606679733),.UNSPECIFIED.);
#10068=B_SPLINE_CURVE_WITH_KNOTS('',3,(#76934,#76935,#76936,#76937,#76938,
#76939,#76940,#76941,#76942,#76943,#76944,#76945,#76946,#76947),
 .UNSPECIFIED.,.F.,.F.,(4,2,2,2,2,2,4),(0.0553058468575743,0.0615439228170499,
0.0677819987765255,0.0802581506954767,0.0954349222053127,0.110611693715149,
0.112045606679733),.UNSPECIFIED.);
#10069=B_SPLINE_CURVE_WITH_KNOTS('',3,(#76965,#76966,#76967,#76968,#76969,
#76970,#76971,#76972,#76973,#76974,#76975,#76976,#76977,#76978),
 .UNSPECIFIED.,.F.,.F.,(4,2,2,2,2,2,4),(0.0553058468575747,0.0615439228170501,
0.0677819987765255,0.0802581506954763,0.0954349222053129,0.110611693715149,
0.112045606679733),.UNSPECIFIED.);
#10070=B_SPLINE_CURVE_WITH_KNOTS('',3,(#76991,#76992,#76993,#76994,#76995,
#76996,#76997,#76998,#76999,#77000,#77001,#77002,#77003,#77004),
 .UNSPECIFIED.,.F.,.F.,(4,2,2,2,2,2,4),(0.0553058468575747,0.0615439228170503,
0.0677819987765259,0.0802581506954771,0.095434922205313,0.110611693715149,
0.112045606679732),.UNSPECIFIED.);
#10071=B_SPLINE_CURVE_WITH_KNOTS('',3,(#77014,#77015,#77016,#77017,#77018,
#77019),.UNSPECIFIED.,.F.,.F.,(4,2,4),(0.133326015406807,0.144441850335848,
0.15555090197436),.UNSPECIFIED.);
#10072=B_SPLINE_CURVE_WITH_KNOTS('',3,(#77036,#77037,#77038,#77039,#77040,
#77041,#77042,#77043,#77044,#77045,#77046,#77047,#77048,#77049),
 .UNSPECIFIED.,.F.,.F.,(4,2,2,2,2,2,4),(-0.112045606679732,-0.110611693715147,
-0.0954349222053114,-0.0802581506954755,-0.0677819987765245,-0.061543922817049,
-0.0553058468575735),.UNSPECIFIED.);
#10531=LINE('',#68022,#13025);
#10532=LINE('',#68025,#13026);
#10533=LINE('',#68066,#13027);
#10534=LINE('',#68069,#13028);
#10535=LINE('',#68088,#13029);
#10536=LINE('',#68091,#13030);
#10537=LINE('',#68142,#13031);
#10538=LINE('',#68146,#13032);
#10539=LINE('',#68154,#13033);
#10540=LINE('',#68157,#13034);
#10541=LINE('',#68161,#13035);
#10542=LINE('',#68163,#13036);
#10543=LINE('',#68165,#13037);
#10544=LINE('',#68169,#13038);
#10545=LINE('',#68171,#13039);
#10546=LINE('',#68173,#13040);
#10547=LINE('',#68177,#13041);
#10548=LINE('',#68179,#13042);
#10549=LINE('',#68181,#13043);
#10550=LINE('',#68185,#13044);
#10551=LINE('',#68187,#13045);
#10552=LINE('',#68189,#13046);
#10553=LINE('',#68193,#13047);
#10554=LINE('',#68195,#13048);
#10555=LINE('',#68197,#13049);
#10556=LINE('',#68201,#13050);
#10557=LINE('',#68203,#13051);
#10558=LINE('',#68205,#13052);
#10559=LINE('',#68209,#13053);
#10560=LINE('',#68211,#13054);
#10561=LINE('',#68213,#13055);
#10562=LINE('',#68217,#13056);
#10563=LINE('',#68219,#13057);
#10564=LINE('',#68221,#13058);
#10565=LINE('',#68225,#13059);
#10566=LINE('',#68227,#13060);
#10567=LINE('',#68229,#13061);
#10568=LINE('',#68233,#13062);
#10569=LINE('',#68235,#13063);
#10570=LINE('',#68237,#13064);
#10571=LINE('',#68241,#13065);
#10572=LINE('',#68243,#13066);
#10573=LINE('',#68245,#13067);
#10574=LINE('',#68249,#13068);
#10575=LINE('',#68251,#13069);
#10576=LINE('',#68253,#13070);
#10577=LINE('',#68257,#13071);
#10578=LINE('',#68259,#13072);
#10579=LINE('',#68261,#13073);
#10580=LINE('',#68265,#13074);
#10581=LINE('',#68267,#13075);
#10582=LINE('',#68269,#13076);
#10583=LINE('',#68273,#13077);
#10584=LINE('',#68275,#13078);
#10585=LINE('',#68277,#13079);
#10586=LINE('',#68281,#13080);
#10587=LINE('',#68283,#13081);
#10588=LINE('',#68285,#13082);
#10589=LINE('',#68289,#13083);
#10590=LINE('',#68291,#13084);
#10591=LINE('',#68293,#13085);
#10592=LINE('',#68297,#13086);
#10593=LINE('',#68299,#13087);
#10594=LINE('',#68301,#13088);
#10595=LINE('',#68305,#13089);
#10596=LINE('',#68307,#13090);
#10597=LINE('',#68309,#13091);
#10598=LINE('',#68313,#13092);
#10599=LINE('',#68315,#13093);
#10600=LINE('',#68317,#13094);
#10601=LINE('',#68321,#13095);
#10602=LINE('',#68323,#13096);
#10603=LINE('',#68325,#13097);
#10604=LINE('',#68329,#13098);
#10605=LINE('',#68331,#13099);
#10606=LINE('',#68333,#13100);
#10607=LINE('',#68337,#13101);
#10608=LINE('',#68339,#13102);
#10609=LINE('',#68341,#13103);
#10610=LINE('',#68345,#13104);
#10611=LINE('',#68347,#13105);
#10612=LINE('',#68349,#13106);
#10613=LINE('',#68353,#13107);
#10614=LINE('',#68355,#13108);
#10615=LINE('',#68357,#13109);
#10616=LINE('',#68361,#13110);
#10617=LINE('',#68363,#13111);
#10618=LINE('',#68365,#13112);
#10619=LINE('',#68369,#13113);
#10620=LINE('',#68371,#13114);
#10621=LINE('',#68373,#13115);
#10622=LINE('',#68377,#13116);
#10623=LINE('',#68379,#13117);
#10624=LINE('',#68381,#13118);
#10625=LINE('',#68385,#13119);
#10626=LINE('',#68387,#13120);
#10627=LINE('',#68389,#13121);
#10628=LINE('',#68393,#13122);
#10629=LINE('',#68395,#13123);
#10630=LINE('',#68397,#13124);
#10631=LINE('',#68401,#13125);
#10632=LINE('',#68403,#13126);
#10633=LINE('',#68405,#13127);
#10634=LINE('',#68409,#13128);
#10635=LINE('',#68411,#13129);
#10636=LINE('',#68413,#13130);
#10637=LINE('',#68417,#13131);
#10638=LINE('',#68419,#13132);
#10639=LINE('',#68421,#13133);
#10640=LINE('',#68425,#13134);
#10641=LINE('',#68427,#13135);
#10642=LINE('',#68429,#13136);
#10643=LINE('',#68433,#13137);
#10644=LINE('',#68435,#13138);
#10645=LINE('',#68437,#13139);
#10646=LINE('',#68441,#13140);
#10647=LINE('',#68443,#13141);
#10648=LINE('',#68445,#13142);
#10649=LINE('',#68469,#13143);
#10650=LINE('',#68471,#13144);
#10651=LINE('',#68473,#13145);
#10652=LINE('',#68497,#13146);
#10653=LINE('',#68499,#13147);
#10654=LINE('',#68501,#13148);
#10655=LINE('',#68525,#13149);
#10656=LINE('',#68527,#13150);
#10657=LINE('',#68529,#13151);
#10658=LINE('',#68533,#13152);
#10659=LINE('',#68535,#13153);
#10660=LINE('',#68537,#13154);
#10661=LINE('',#68541,#13155);
#10662=LINE('',#68543,#13156);
#10663=LINE('',#68545,#13157);
#10664=LINE('',#68549,#13158);
#10665=LINE('',#68551,#13159);
#10666=LINE('',#68553,#13160);
#10667=LINE('',#68557,#13161);
#10668=LINE('',#68559,#13162);
#10669=LINE('',#68561,#13163);
#10670=LINE('',#68565,#13164);
#10671=LINE('',#68567,#13165);
#10672=LINE('',#68569,#13166);
#10673=LINE('',#68573,#13167);
#10674=LINE('',#68575,#13168);
#10675=LINE('',#68577,#13169);
#10676=LINE('',#68581,#13170);
#10677=LINE('',#68583,#13171);
#10678=LINE('',#68585,#13172);
#10679=LINE('',#68589,#13173);
#10680=LINE('',#68591,#13174);
#10681=LINE('',#68593,#13175);
#10682=LINE('',#68596,#13176);
#10683=LINE('',#68615,#13177);
#10684=LINE('',#68621,#13178);
#10685=LINE('',#68662,#13179);
#10686=LINE('',#68665,#13180);
#10687=LINE('',#68684,#13181);
#10688=LINE('',#68687,#13182);
#10689=LINE('',#68738,#13183);
#10690=LINE('',#68742,#13184);
#10691=LINE('',#68750,#13185);
#10692=LINE('',#68767,#13186);
#10693=LINE('',#68773,#13187);
#10694=LINE('',#68814,#13188);
#10695=LINE('',#68817,#13189);
#10696=LINE('',#68836,#13190);
#10697=LINE('',#68839,#13191);
#10698=LINE('',#68890,#13192);
#10699=LINE('',#68894,#13193);
#10700=LINE('',#68902,#13194);
#10701=LINE('',#68919,#13195);
#10702=LINE('',#68925,#13196);
#10703=LINE('',#68928,#13197);
#10704=LINE('',#68982,#13198);
#10705=LINE('',#68985,#13199);
#10706=LINE('',#69003,#13200);
#10707=LINE('',#69058,#13201);
#10708=LINE('',#69061,#13202);
#10709=LINE('',#69065,#13203);
#10710=LINE('',#69067,#13204);
#10711=LINE('',#69077,#13205);
#10712=LINE('',#69080,#13206);
#10713=LINE('',#69134,#13207);
#10714=LINE('',#69137,#13208);
#10715=LINE('',#69155,#13209);
#10716=LINE('',#69210,#13210);
#10717=LINE('',#69213,#13211);
#10718=LINE('',#69217,#13212);
#10719=LINE('',#69219,#13213);
#10720=LINE('',#69229,#13214);
#10721=LINE('',#69232,#13215);
#10722=LINE('',#69286,#13216);
#10723=LINE('',#69288,#13217);
#10724=LINE('',#69294,#13218);
#10725=LINE('',#69296,#13219);
#10726=LINE('',#69300,#13220);
#10727=LINE('',#69302,#13221);
#10728=LINE('',#69304,#13222);
#10729=LINE('',#69308,#13223);
#10730=LINE('',#69310,#13224);
#10731=LINE('',#69312,#13225);
#10732=LINE('',#69316,#13226);
#10733=LINE('',#69318,#13227);
#10734=LINE('',#69320,#13228);
#10735=LINE('',#69324,#13229);
#10736=LINE('',#69326,#13230);
#10737=LINE('',#69328,#13231);
#10738=LINE('',#69332,#13232);
#10739=LINE('',#69334,#13233);
#10740=LINE('',#69336,#13234);
#10741=LINE('',#69340,#13235);
#10742=LINE('',#69342,#13236);
#10743=LINE('',#69344,#13237);
#10744=LINE('',#69348,#13238);
#10745=LINE('',#69350,#13239);
#10746=LINE('',#69352,#13240);
#10747=LINE('',#69356,#13241);
#10748=LINE('',#69358,#13242);
#10749=LINE('',#69360,#13243);
#10750=LINE('',#69364,#13244);
#10751=LINE('',#69366,#13245);
#10752=LINE('',#69368,#13246);
#10753=LINE('',#69372,#13247);
#10754=LINE('',#69374,#13248);
#10755=LINE('',#69376,#13249);
#10756=LINE('',#69380,#13250);
#10757=LINE('',#69382,#13251);
#10758=LINE('',#69384,#13252);
#10759=LINE('',#69388,#13253);
#10760=LINE('',#69390,#13254);
#10761=LINE('',#69392,#13255);
#10762=LINE('',#69396,#13256);
#10763=LINE('',#69398,#13257);
#10764=LINE('',#69400,#13258);
#10765=LINE('',#69404,#13259);
#10766=LINE('',#69406,#13260);
#10767=LINE('',#69408,#13261);
#10768=LINE('',#69412,#13262);
#10769=LINE('',#69414,#13263);
#10770=LINE('',#69416,#13264);
#10771=LINE('',#69420,#13265);
#10772=LINE('',#69422,#13266);
#10773=LINE('',#69424,#13267);
#10774=LINE('',#69428,#13268);
#10775=LINE('',#69430,#13269);
#10776=LINE('',#69432,#13270);
#10777=LINE('',#69436,#13271);
#10778=LINE('',#69437,#13272);
#10779=LINE('',#69439,#13273);
#10780=LINE('',#69441,#13274);
#10781=LINE('',#69443,#13275);
#10782=LINE('',#69447,#13276);
#10783=LINE('',#69449,#13277);
#10784=LINE('',#69451,#13278);
#10785=LINE('',#69455,#13279);
#10786=LINE('',#69457,#13280);
#10787=LINE('',#69459,#13281);
#10788=LINE('',#69463,#13282);
#10789=LINE('',#69465,#13283);
#10790=LINE('',#69467,#13284);
#10791=LINE('',#69471,#13285);
#10792=LINE('',#69472,#13286);
#10793=LINE('',#69475,#13287);
#10794=LINE('',#69477,#13288);
#10795=LINE('',#69481,#13289);
#10796=LINE('',#69483,#13290);
#10797=LINE('',#69485,#13291);
#10798=LINE('',#69489,#13292);
#10799=LINE('',#69491,#13293);
#10800=LINE('',#69493,#13294);
#10801=LINE('',#69497,#13295);
#10802=LINE('',#69499,#13296);
#10803=LINE('',#69501,#13297);
#10804=LINE('',#69505,#13298);
#10805=LINE('',#69506,#13299);
#10806=LINE('',#69508,#13300);
#10807=LINE('',#69510,#13301);
#10808=LINE('',#69512,#13302);
#10809=LINE('',#69516,#13303);
#10810=LINE('',#69517,#13304);
#10811=LINE('',#69521,#13305);
#10812=LINE('',#69523,#13306);
#10813=LINE('',#69525,#13307);
#10814=LINE('',#69529,#13308);
#10815=LINE('',#69531,#13309);
#10816=LINE('',#69533,#13310);
#10817=LINE('',#69537,#13311);
#10818=LINE('',#69539,#13312);
#10819=LINE('',#69541,#13313);
#10820=LINE('',#69545,#13314);
#10821=LINE('',#69547,#13315);
#10822=LINE('',#69549,#13316);
#10823=LINE('',#69553,#13317);
#10824=LINE('',#69554,#13318);
#10825=LINE('',#69557,#13319);
#10826=LINE('',#69559,#13320);
#10827=LINE('',#69563,#13321);
#10828=LINE('',#69565,#13322);
#10829=LINE('',#69567,#13323);
#10830=LINE('',#69571,#13324);
#10831=LINE('',#69573,#13325);
#10832=LINE('',#69575,#13326);
#10833=LINE('',#69579,#13327);
#10834=LINE('',#69581,#13328);
#10835=LINE('',#69583,#13329);
#10836=LINE('',#69587,#13330);
#10837=LINE('',#69589,#13331);
#10838=LINE('',#69591,#13332);
#10839=LINE('',#69595,#13333);
#10840=LINE('',#69597,#13334);
#10841=LINE('',#69599,#13335);
#10842=LINE('',#69603,#13336);
#10843=LINE('',#69605,#13337);
#10844=LINE('',#69607,#13338);
#10845=LINE('',#69611,#13339);
#10846=LINE('',#69613,#13340);
#10847=LINE('',#69615,#13341);
#10848=LINE('',#69619,#13342);
#10849=LINE('',#69621,#13343);
#10850=LINE('',#69623,#13344);
#10851=LINE('',#69627,#13345);
#10852=LINE('',#69629,#13346);
#10853=LINE('',#69631,#13347);
#10854=LINE('',#69635,#13348);
#10855=LINE('',#69637,#13349);
#10856=LINE('',#69639,#13350);
#10857=LINE('',#69643,#13351);
#10858=LINE('',#69644,#13352);
#10859=LINE('',#69665,#13353);
#10860=LINE('',#69671,#13354);
#10861=LINE('',#69725,#13355);
#10862=LINE('',#69727,#13356);
#10863=LINE('',#69748,#13357);
#10864=LINE('',#69754,#13358);
#10865=LINE('',#69808,#13359);
#10866=LINE('',#69810,#13360);
#10867=LINE('',#69831,#13361);
#10868=LINE('',#69837,#13362);
#10869=LINE('',#69843,#13363);
#10870=LINE('',#69897,#13364);
#10871=LINE('',#69900,#13365);
#10872=LINE('',#69951,#13366);
#10873=LINE('',#69955,#13367);
#10874=LINE('',#69959,#13368);
#10875=LINE('',#69975,#13369);
#10876=LINE('',#69981,#13370);
#10877=LINE('',#70035,#13371);
#10878=LINE('',#70037,#13372);
#10879=LINE('',#70058,#13373);
#10880=LINE('',#70064,#13374);
#10881=LINE('',#70118,#13375);
#10882=LINE('',#70120,#13376);
#10883=LINE('',#70141,#13377);
#10884=LINE('',#70147,#13378);
#10885=LINE('',#70201,#13379);
#10886=LINE('',#70203,#13380);
#10887=LINE('',#70222,#13381);
#10888=LINE('',#70228,#13382);
#10889=LINE('',#70282,#13383);
#10890=LINE('',#70285,#13384);
#10891=LINE('',#70336,#13385);
#10892=LINE('',#70340,#13386);
#10893=LINE('',#70344,#13387);
#10894=LINE('',#70360,#13388);
#10895=LINE('',#70398,#13389);
#10896=LINE('',#70403,#13390);
#10897=LINE('',#70412,#13391);
#10898=LINE('',#70444,#13392);
#10899=LINE('',#70451,#13393);
#10900=LINE('',#70460,#13394);
#10901=LINE('',#70466,#13395);
#10902=LINE('',#70520,#13396);
#10903=LINE('',#70522,#13397);
#10904=LINE('',#70543,#13398);
#10905=LINE('',#70575,#13399);
#10906=LINE('',#70582,#13400);
#10907=LINE('',#70591,#13401);
#10908=LINE('',#70597,#13402);
#10909=LINE('',#70651,#13403);
#10910=LINE('',#70653,#13404);
#10911=LINE('',#70698,#13405);
#10912=LINE('',#70719,#13406);
#10913=LINE('',#70722,#13407);
#10914=LINE('',#70731,#13408);
#10915=LINE('',#70769,#13409);
#10916=LINE('',#70774,#13410);
#10917=LINE('',#70783,#13411);
#10918=LINE('',#70800,#13412);
#10919=LINE('',#70803,#13413);
#10920=LINE('',#70812,#13414);
#10921=LINE('',#70818,#13415);
#10922=LINE('',#70872,#13416);
#10923=LINE('',#70874,#13417);
#10924=LINE('',#70893,#13418);
#10925=LINE('',#70947,#13419);
#10926=LINE('',#70949,#13420);
#10927=LINE('',#70970,#13421);
#10928=LINE('',#70976,#13422);
#10929=LINE('',#71030,#13423);
#10930=LINE('',#71032,#13424);
#10931=LINE('',#71053,#13425);
#10932=LINE('',#71085,#13426);
#10933=LINE('',#71092,#13427);
#10934=LINE('',#71101,#13428);
#10935=LINE('',#71107,#13429);
#10936=LINE('',#71161,#13430);
#10937=LINE('',#71163,#13431);
#10938=LINE('',#71184,#13432);
#10939=LINE('',#71216,#13433);
#10940=LINE('',#71223,#13434);
#10941=LINE('',#71232,#13435);
#10942=LINE('',#71249,#13436);
#10943=LINE('',#71252,#13437);
#10944=LINE('',#71261,#13438);
#10945=LINE('',#71267,#13439);
#10946=LINE('',#71321,#13440);
#10947=LINE('',#71323,#13441);
#10948=LINE('',#71344,#13442);
#10949=LINE('',#71350,#13443);
#10950=LINE('',#71404,#13444);
#10951=LINE('',#71406,#13445);
#10952=LINE('',#71427,#13446);
#10953=LINE('',#71433,#13447);
#10954=LINE('',#71487,#13448);
#10955=LINE('',#71489,#13449);
#10956=LINE('',#71534,#13450);
#10957=LINE('',#71541,#13451);
#10958=LINE('',#71550,#13452);
#10959=LINE('',#71582,#13453);
#10960=LINE('',#71589,#13454);
#10961=LINE('',#71598,#13455);
#10962=LINE('',#71604,#13456);
#10963=LINE('',#71658,#13457);
#10964=LINE('',#71660,#13458);
#10965=LINE('',#71681,#13459);
#10966=LINE('',#71713,#13460);
#10967=LINE('',#71720,#13461);
#10968=LINE('',#71729,#13462);
#10969=LINE('',#71746,#13463);
#10970=LINE('',#71749,#13464);
#10971=LINE('',#71758,#13465);
#10972=LINE('',#71775,#13466);
#10973=LINE('',#71778,#13467);
#10974=LINE('',#71787,#13468);
#10975=LINE('',#71825,#13469);
#10976=LINE('',#71830,#13470);
#10977=LINE('',#71839,#13471);
#10978=LINE('',#71871,#13472);
#10979=LINE('',#71878,#13473);
#10980=LINE('',#71887,#13474);
#10981=LINE('',#71893,#13475);
#10982=LINE('',#71947,#13476);
#10983=LINE('',#71949,#13477);
#10984=LINE('',#71994,#13478);
#10985=LINE('',#72001,#13479);
#10986=LINE('',#72010,#13480);
#10987=LINE('',#72016,#13481);
#10988=LINE('',#72070,#13482);
#10989=LINE('',#72072,#13483);
#10990=LINE('',#72093,#13484);
#10991=LINE('',#72125,#13485);
#10992=LINE('',#72132,#13486);
#10993=LINE('',#72141,#13487);
#10994=LINE('',#72158,#13488);
#10995=LINE('',#72161,#13489);
#10996=LINE('',#72170,#13490);
#10997=LINE('',#72208,#13491);
#10998=LINE('',#72213,#13492);
#10999=LINE('',#72222,#13493);
#11000=LINE('',#72239,#13494);
#11001=LINE('',#72242,#13495);
#11002=LINE('',#72251,#13496);
#11003=LINE('',#72257,#13497);
#11004=LINE('',#72311,#13498);
#11005=LINE('',#72313,#13499);
#11006=LINE('',#72334,#13500);
#11007=LINE('',#72340,#13501);
#11008=LINE('',#72394,#13502);
#11009=LINE('',#72396,#13503);
#11010=LINE('',#72417,#13504);
#11011=LINE('',#72423,#13505);
#11012=LINE('',#72477,#13506);
#11013=LINE('',#72479,#13507);
#11014=LINE('',#72498,#13508);
#11015=LINE('',#72552,#13509);
#11016=LINE('',#72554,#13510);
#11017=LINE('',#72575,#13511);
#11018=LINE('',#72607,#13512);
#11019=LINE('',#72614,#13513);
#11020=LINE('',#72623,#13514);
#11021=LINE('',#72661,#13515);
#11022=LINE('',#72666,#13516);
#11023=LINE('',#72675,#13517);
#11024=LINE('',#72681,#13518);
#11025=LINE('',#72735,#13519);
#11026=LINE('',#72737,#13520);
#11027=LINE('',#72758,#13521);
#11028=LINE('',#72764,#13522);
#11029=LINE('',#72818,#13523);
#11030=LINE('',#72820,#13524);
#11031=LINE('',#72865,#13525);
#11032=LINE('',#72872,#13526);
#11033=LINE('',#72881,#13527);
#11034=LINE('',#72913,#13528);
#11035=LINE('',#72920,#13529);
#11036=LINE('',#72929,#13530);
#11037=LINE('',#72935,#13531);
#11038=LINE('',#72989,#13532);
#11039=LINE('',#72991,#13533);
#11040=LINE('',#73012,#13534);
#11041=LINE('',#73044,#13535);
#11042=LINE('',#73065,#13536);
#11043=LINE('',#73068,#13537);
#11044=LINE('',#73077,#13538);
#11045=LINE('',#73109,#13539);
#11046=LINE('',#73116,#13540);
#11047=LINE('',#73125,#13541);
#11048=LINE('',#73142,#13542);
#11049=LINE('',#73145,#13543);
#11050=LINE('',#73154,#13544);
#11051=LINE('',#73171,#13545);
#11052=LINE('',#73174,#13546);
#11053=LINE('',#73183,#13547);
#11054=LINE('',#73221,#13548);
#11055=LINE('',#73226,#13549);
#11056=LINE('',#73235,#13550);
#11057=LINE('',#73267,#13551);
#11058=LINE('',#73274,#13552);
#11059=LINE('',#73283,#13553);
#11060=LINE('',#73289,#13554);
#11061=LINE('',#73343,#13555);
#11062=LINE('',#73345,#13556);
#11063=LINE('',#73366,#13557);
#11064=LINE('',#73398,#13558);
#11065=LINE('',#73419,#13559);
#11066=LINE('',#73422,#13560);
#11067=LINE('',#73431,#13561);
#11068=LINE('',#73437,#13562);
#11069=LINE('',#73491,#13563);
#11070=LINE('',#73493,#13564);
#11071=LINE('',#73514,#13565);
#11072=LINE('',#73520,#13566);
#11073=LINE('',#73574,#13567);
#11074=LINE('',#73576,#13568);
#11075=LINE('',#73597,#13569);
#11076=LINE('',#73629,#13570);
#11077=LINE('',#73636,#13571);
#11078=LINE('',#73645,#13572);
#11079=LINE('',#73651,#13573);
#11080=LINE('',#73705,#13574);
#11081=LINE('',#73707,#13575);
#11082=LINE('',#73726,#13576);
#11083=LINE('',#73780,#13577);
#11084=LINE('',#73782,#13578);
#11085=LINE('',#73803,#13579);
#11086=LINE('',#73836,#13580);
#11087=LINE('',#73890,#13581);
#11088=LINE('',#73892,#13582);
#11089=LINE('',#73943,#13583);
#11090=LINE('',#73948,#13584);
#11091=LINE('',#73957,#13585);
#11092=LINE('',#73989,#13586);
#11093=LINE('',#73996,#13587);
#11094=LINE('',#74005,#13588);
#11095=LINE('',#74043,#13589);
#11096=LINE('',#74048,#13590);
#11097=LINE('',#74057,#13591);
#11098=LINE('',#74074,#13592);
#11099=LINE('',#74077,#13593);
#11100=LINE('',#74086,#13594);
#11101=LINE('',#74118,#13595);
#11102=LINE('',#74125,#13596);
#11103=LINE('',#74134,#13597);
#11104=LINE('',#74166,#13598);
#11105=LINE('',#74173,#13599);
#11106=LINE('',#74182,#13600);
#11107=LINE('',#74188,#13601);
#11108=LINE('',#74242,#13602);
#11109=LINE('',#74244,#13603);
#11110=LINE('',#74265,#13604);
#11111=LINE('',#74297,#13605);
#11112=LINE('',#74304,#13606);
#11113=LINE('',#74313,#13607);
#11114=LINE('',#74330,#13608);
#11115=LINE('',#74333,#13609);
#11116=LINE('',#74342,#13610);
#11117=LINE('',#74359,#13611);
#11118=LINE('',#74362,#13612);
#11119=LINE('',#74371,#13613);
#11120=LINE('',#74377,#13614);
#11121=LINE('',#74431,#13615);
#11122=LINE('',#74433,#13616);
#11123=LINE('',#74454,#13617);
#11124=LINE('',#74460,#13618);
#11125=LINE('',#74514,#13619);
#11126=LINE('',#74516,#13620);
#11127=LINE('',#74535,#13621);
#11128=LINE('',#74589,#13622);
#11129=LINE('',#74591,#13623);
#11130=LINE('',#74612,#13624);
#11131=LINE('',#74618,#13625);
#11132=LINE('',#74672,#13626);
#11133=LINE('',#74674,#13627);
#11134=LINE('',#74695,#13628);
#11135=LINE('',#74701,#13629);
#11136=LINE('',#74755,#13630);
#11137=LINE('',#74757,#13631);
#11138=LINE('',#74808,#13632);
#11139=LINE('',#74813,#13633);
#11140=LINE('',#74822,#13634);
#11141=LINE('',#74854,#13635);
#11142=LINE('',#74861,#13636);
#11143=LINE('',#74870,#13637);
#11144=LINE('',#74902,#13638);
#11145=LINE('',#74909,#13639);
#11146=LINE('',#74918,#13640);
#11147=LINE('',#74956,#13641);
#11148=LINE('',#74961,#13642);
#11149=LINE('',#74970,#13643);
#11150=LINE('',#74989,#13644);
#11151=LINE('',#75005,#13645);
#11152=LINE('',#75008,#13646);
#11153=LINE('',#75012,#13647);
#11154=LINE('',#75031,#13648);
#11155=LINE('',#75041,#13649);
#11156=LINE('',#75080,#13650);
#11157=LINE('',#75087,#13651);
#11158=LINE('',#75096,#13652);
#11159=LINE('',#75102,#13653);
#11160=LINE('',#75156,#13654);
#11161=LINE('',#75158,#13655);
#11162=LINE('',#75236,#13656);
#11163=LINE('',#75241,#13657);
#11164=LINE('',#75250,#13658);
#11165=LINE('',#75267,#13659);
#11166=LINE('',#75270,#13660);
#11167=LINE('',#75279,#13661);
#11168=LINE('',#75296,#13662);
#11169=LINE('',#75332,#13663);
#11170=LINE('',#75334,#13664);
#11171=LINE('',#75340,#13665);
#11172=LINE('',#75351,#13666);
#11173=LINE('',#75354,#13667);
#11174=LINE('',#75355,#13668);
#11175=LINE('',#75358,#13669);
#11176=LINE('',#75360,#13670);
#11177=LINE('',#75384,#13671);
#11178=LINE('',#75387,#13672);
#11179=LINE('',#75396,#13673);
#11180=LINE('',#75400,#13674);
#11181=LINE('',#75402,#13675);
#11182=LINE('',#75406,#13676);
#11183=LINE('',#75409,#13677);
#11184=LINE('',#75410,#13678);
#11185=LINE('',#75413,#13679);
#11186=LINE('',#75415,#13680);
#11187=LINE('',#75433,#13681);
#11188=LINE('',#75435,#13682);
#11189=LINE('',#75452,#13683);
#11190=LINE('',#75455,#13684);
#11191=LINE('',#75464,#13685);
#11192=LINE('',#75468,#13686);
#11193=LINE('',#75471,#13687);
#11194=LINE('',#75472,#13688);
#11195=LINE('',#75475,#13689);
#11196=LINE('',#75477,#13690);
#11197=LINE('',#75488,#13691);
#11198=LINE('',#75490,#13692);
#11199=LINE('',#75509,#13693);
#11200=LINE('',#75512,#13694);
#11201=LINE('',#75521,#13695);
#11202=LINE('',#75555,#13696);
#11203=LINE('',#75559,#13697);
#11204=LINE('',#75561,#13698);
#11205=LINE('',#75562,#13699);
#11206=LINE('',#75564,#13700);
#11207=LINE('',#75568,#13701);
#11208=LINE('',#75570,#13702);
#11209=LINE('',#75574,#13703);
#11210=LINE('',#75577,#13704);
#11211=LINE('',#75578,#13705);
#11212=LINE('',#75581,#13706);
#11213=LINE('',#75583,#13707);
#11214=LINE('',#75607,#13708);
#11215=LINE('',#75610,#13709);
#11216=LINE('',#75619,#13710);
#11217=LINE('',#75625,#13711);
#11218=LINE('',#75627,#13712);
#11219=LINE('',#75628,#13713);
#11220=LINE('',#75639,#13714);
#11221=LINE('',#75642,#13715);
#11222=LINE('',#75643,#13716);
#11223=LINE('',#75646,#13717);
#11224=LINE('',#75648,#13718);
#11225=LINE('',#75666,#13719);
#11226=LINE('',#75668,#13720);
#11227=LINE('',#75685,#13721);
#11228=LINE('',#75688,#13722);
#11229=LINE('',#75697,#13723);
#11230=LINE('',#75701,#13724);
#11231=LINE('',#75704,#13725);
#11232=LINE('',#75705,#13726);
#11233=LINE('',#75708,#13727);
#11234=LINE('',#75710,#13728);
#11235=LINE('',#75721,#13729);
#11236=LINE('',#75723,#13730);
#11237=LINE('',#75742,#13731);
#11238=LINE('',#75745,#13732);
#11239=LINE('',#75754,#13733);
#11240=LINE('',#75788,#13734);
#11241=LINE('',#75792,#13735);
#11242=LINE('',#75794,#13736);
#11243=LINE('',#75795,#13737);
#11244=LINE('',#75797,#13738);
#11245=LINE('',#75803,#13739);
#11246=LINE('',#75805,#13740);
#11247=LINE('',#75806,#13741);
#11248=LINE('',#75817,#13742);
#11249=LINE('',#75820,#13743);
#11250=LINE('',#75821,#13744);
#11251=LINE('',#75824,#13745);
#11252=LINE('',#75826,#13746);
#11253=LINE('',#75850,#13747);
#11254=LINE('',#75853,#13748);
#11255=LINE('',#75862,#13749);
#11256=LINE('',#75866,#13750);
#11257=LINE('',#75868,#13751);
#11258=LINE('',#75872,#13752);
#11259=LINE('',#75875,#13753);
#11260=LINE('',#75876,#13754);
#11261=LINE('',#75879,#13755);
#11262=LINE('',#75881,#13756);
#11263=LINE('',#75892,#13757);
#11264=LINE('',#75894,#13758);
#11265=LINE('',#75911,#13759);
#11266=LINE('',#75914,#13760);
#11267=LINE('',#75923,#13761);
#11268=LINE('',#75927,#13762);
#11269=LINE('',#75930,#13763);
#11270=LINE('',#75931,#13764);
#11271=LINE('',#75934,#13765);
#11272=LINE('',#75936,#13766);
#11273=LINE('',#75947,#13767);
#11274=LINE('',#75949,#13768);
#11275=LINE('',#75968,#13769);
#11276=LINE('',#75971,#13770);
#11277=LINE('',#75980,#13771);
#11278=LINE('',#76014,#13772);
#11279=LINE('',#76018,#13773);
#11280=LINE('',#76020,#13774);
#11281=LINE('',#76021,#13775);
#11282=LINE('',#76023,#13776);
#11283=LINE('',#76027,#13777);
#11284=LINE('',#76029,#13778);
#11285=LINE('',#76048,#13779);
#11286=LINE('',#76051,#13780);
#11287=LINE('',#76060,#13781);
#11288=LINE('',#76098,#13782);
#11289=LINE('',#76101,#13783);
#11290=LINE('',#76105,#13784);
#11291=LINE('',#76114,#13785);
#11292=LINE('',#76117,#13786);
#11293=LINE('',#76119,#13787);
#11294=LINE('',#76128,#13788);
#11295=LINE('',#76132,#13789);
#11296=LINE('',#76134,#13790);
#11297=LINE('',#76138,#13791);
#11298=LINE('',#76141,#13792);
#11299=LINE('',#76142,#13793);
#11300=LINE('',#76145,#13794);
#11301=LINE('',#76147,#13795);
#11302=LINE('',#76180,#13796);
#11303=LINE('',#76183,#13797);
#11304=LINE('',#76192,#13798);
#11305=LINE('',#76194,#13799);
#11306=LINE('',#76196,#13800);
#11307=LINE('',#76200,#13801);
#11308=LINE('',#76203,#13802);
#11309=LINE('',#76204,#13803);
#11310=LINE('',#76207,#13804);
#11311=LINE('',#76209,#13805);
#11312=LINE('',#76222,#13806);
#11313=LINE('',#76261,#13807);
#11314=LINE('',#76264,#13808);
#11315=LINE('',#76309,#13809);
#11316=LINE('',#76317,#13810);
#11317=LINE('',#76323,#13811);
#11318=LINE('',#76377,#13812);
#11319=LINE('',#76380,#13813);
#11320=LINE('',#76431,#13814);
#11321=LINE('',#76435,#13815);
#11322=LINE('',#76439,#13816);
#11323=LINE('',#76455,#13817);
#11324=LINE('',#76500,#13818);
#11325=LINE('',#76537,#13819);
#11326=LINE('',#76625,#13820);
#11327=LINE('',#76628,#13821);
#11328=LINE('',#76629,#13822);
#11329=LINE('',#76632,#13823);
#11330=LINE('',#76635,#13824);
#11331=LINE('',#76636,#13825);
#11332=LINE('',#76642,#13826);
#11333=LINE('',#76644,#13827);
#11334=LINE('',#76645,#13828);
#11335=LINE('',#76653,#13829);
#11336=LINE('',#76669,#13830);
#11337=LINE('',#76671,#13831);
#11338=LINE('',#76679,#13832);
#11339=LINE('',#76681,#13833);
#11340=LINE('',#76684,#13834);
#11341=LINE('',#76700,#13835);
#11342=LINE('',#76702,#13836);
#11343=LINE('',#76710,#13837);
#11344=LINE('',#76726,#13838);
#11345=LINE('',#76728,#13839);
#11346=LINE('',#76733,#13840);
#11347=LINE('',#76738,#13841);
#11348=LINE('',#76740,#13842);
#11349=LINE('',#76748,#13843);
#11350=LINE('',#76764,#13844);
#11351=LINE('',#76766,#13845);
#11352=LINE('',#76774,#13846);
#11353=LINE('',#76790,#13847);
#11354=LINE('',#76792,#13848);
#11355=LINE('',#76800,#13849);
#11356=LINE('',#76816,#13850);
#11357=LINE('',#76818,#13851);
#11358=LINE('',#76824,#13852);
#11359=LINE('',#76828,#13853);
#11360=LINE('',#76830,#13854);
#11361=LINE('',#76838,#13855);
#11362=LINE('',#76854,#13856);
#11363=LINE('',#76856,#13857);
#11364=LINE('',#76864,#13858);
#11365=LINE('',#76866,#13859);
#11366=LINE('',#76869,#13860);
#11367=LINE('',#76885,#13861);
#11368=LINE('',#76887,#13862);
#11369=LINE('',#76893,#13863);
#11370=LINE('',#76897,#13864);
#11371=LINE('',#76913,#13865);
#11372=LINE('',#76915,#13866);
#11373=LINE('',#76923,#13867);
#11374=LINE('',#76925,#13868);
#11375=LINE('',#76933,#13869);
#11376=LINE('',#76949,#13870);
#11377=LINE('',#76951,#13871);
#11378=LINE('',#76959,#13872);
#11379=LINE('',#76961,#13873);
#11380=LINE('',#76964,#13874);
#11381=LINE('',#76980,#13875);
#11382=LINE('',#76982,#13876);
#11383=LINE('',#76990,#13877);
#11384=LINE('',#77006,#13878);
#11385=LINE('',#77008,#13879);
#11386=LINE('',#77022,#13880);
#11387=LINE('',#77023,#13881);
#11388=LINE('',#77027,#13882);
#11389=LINE('',#77030,#13883);
#11390=LINE('',#77032,#13884);
#11391=LINE('',#77050,#13885);
#11392=LINE('',#77124,#13886);
#13025=VECTOR('',#46183,10.);
#13026=VECTOR('',#46186,10.);
#13027=VECTOR('',#46199,10.);
#13028=VECTOR('',#46202,10.);
#13029=VECTOR('',#46213,10.);
#13030=VECTOR('',#46216,10.);
#13031=VECTOR('',#46235,10.);
#13032=VECTOR('',#46238,10.);
#13033=VECTOR('',#46239,10.);
#13034=VECTOR('',#46242,10.);
#13035=VECTOR('',#46245,10.);
#13036=VECTOR('',#46246,10.);
#13037=VECTOR('',#46247,10.);
#13038=VECTOR('',#46250,10.);
#13039=VECTOR('',#46251,10.);
#13040=VECTOR('',#46252,10.);
#13041=VECTOR('',#46255,10.);
#13042=VECTOR('',#46256,10.);
#13043=VECTOR('',#46257,10.);
#13044=VECTOR('',#46260,10.);
#13045=VECTOR('',#46261,10.);
#13046=VECTOR('',#46262,10.);
#13047=VECTOR('',#46265,10.);
#13048=VECTOR('',#46266,10.);
#13049=VECTOR('',#46267,10.);
#13050=VECTOR('',#46270,10.);
#13051=VECTOR('',#46271,10.);
#13052=VECTOR('',#46272,10.);
#13053=VECTOR('',#46275,10.);
#13054=VECTOR('',#46276,10.);
#13055=VECTOR('',#46277,10.);
#13056=VECTOR('',#46280,10.);
#13057=VECTOR('',#46281,10.);
#13058=VECTOR('',#46282,10.);
#13059=VECTOR('',#46285,10.);
#13060=VECTOR('',#46286,10.);
#13061=VECTOR('',#46287,10.);
#13062=VECTOR('',#46290,10.);
#13063=VECTOR('',#46291,10.);
#13064=VECTOR('',#46292,10.);
#13065=VECTOR('',#46295,10.);
#13066=VECTOR('',#46296,10.);
#13067=VECTOR('',#46297,10.);
#13068=VECTOR('',#46300,10.);
#13069=VECTOR('',#46301,10.);
#13070=VECTOR('',#46302,10.);
#13071=VECTOR('',#46305,10.);
#13072=VECTOR('',#46306,10.);
#13073=VECTOR('',#46307,10.);
#13074=VECTOR('',#46310,10.);
#13075=VECTOR('',#46311,10.);
#13076=VECTOR('',#46312,10.);
#13077=VECTOR('',#46315,10.);
#13078=VECTOR('',#46316,10.);
#13079=VECTOR('',#46317,10.);
#13080=VECTOR('',#46320,10.);
#13081=VECTOR('',#46321,10.);
#13082=VECTOR('',#46322,10.);
#13083=VECTOR('',#46325,10.);
#13084=VECTOR('',#46326,10.);
#13085=VECTOR('',#46327,10.);
#13086=VECTOR('',#46330,10.);
#13087=VECTOR('',#46331,10.);
#13088=VECTOR('',#46332,10.);
#13089=VECTOR('',#46335,10.);
#13090=VECTOR('',#46336,10.);
#13091=VECTOR('',#46337,10.);
#13092=VECTOR('',#46340,10.);
#13093=VECTOR('',#46341,10.);
#13094=VECTOR('',#46342,10.);
#13095=VECTOR('',#46345,10.);
#13096=VECTOR('',#46346,10.);
#13097=VECTOR('',#46347,10.);
#13098=VECTOR('',#46350,10.);
#13099=VECTOR('',#46351,10.);
#13100=VECTOR('',#46352,10.);
#13101=VECTOR('',#46355,10.);
#13102=VECTOR('',#46356,10.);
#13103=VECTOR('',#46357,10.);
#13104=VECTOR('',#46360,10.);
#13105=VECTOR('',#46361,10.);
#13106=VECTOR('',#46362,10.);
#13107=VECTOR('',#46365,10.);
#13108=VECTOR('',#46366,10.);
#13109=VECTOR('',#46367,10.);
#13110=VECTOR('',#46370,10.);
#13111=VECTOR('',#46371,10.);
#13112=VECTOR('',#46372,10.);
#13113=VECTOR('',#46375,10.);
#13114=VECTOR('',#46376,10.);
#13115=VECTOR('',#46377,10.);
#13116=VECTOR('',#46380,10.);
#13117=VECTOR('',#46381,10.);
#13118=VECTOR('',#46382,10.);
#13119=VECTOR('',#46385,10.);
#13120=VECTOR('',#46386,10.);
#13121=VECTOR('',#46387,10.);
#13122=VECTOR('',#46390,10.);
#13123=VECTOR('',#46391,10.);
#13124=VECTOR('',#46392,10.);
#13125=VECTOR('',#46395,10.);
#13126=VECTOR('',#46396,10.);
#13127=VECTOR('',#46397,10.);
#13128=VECTOR('',#46400,10.);
#13129=VECTOR('',#46401,10.);
#13130=VECTOR('',#46402,10.);
#13131=VECTOR('',#46405,10.);
#13132=VECTOR('',#46406,10.);
#13133=VECTOR('',#46407,10.);
#13134=VECTOR('',#46410,10.);
#13135=VECTOR('',#46411,10.);
#13136=VECTOR('',#46412,10.);
#13137=VECTOR('',#46415,10.);
#13138=VECTOR('',#46416,10.);
#13139=VECTOR('',#46417,10.);
#13140=VECTOR('',#46420,10.);
#13141=VECTOR('',#46421,10.);
#13142=VECTOR('',#46422,10.);
#13143=VECTOR('',#46425,10.);
#13144=VECTOR('',#46426,10.);
#13145=VECTOR('',#46427,10.);
#13146=VECTOR('',#46430,10.);
#13147=VECTOR('',#46431,10.);
#13148=VECTOR('',#46432,10.);
#13149=VECTOR('',#46435,10.);
#13150=VECTOR('',#46436,10.);
#13151=VECTOR('',#46437,10.);
#13152=VECTOR('',#46440,10.);
#13153=VECTOR('',#46441,10.);
#13154=VECTOR('',#46442,10.);
#13155=VECTOR('',#46445,10.);
#13156=VECTOR('',#46446,10.);
#13157=VECTOR('',#46447,10.);
#13158=VECTOR('',#46450,10.);
#13159=VECTOR('',#46451,10.);
#13160=VECTOR('',#46452,10.);
#13161=VECTOR('',#46455,10.);
#13162=VECTOR('',#46456,10.);
#13163=VECTOR('',#46457,10.);
#13164=VECTOR('',#46460,10.);
#13165=VECTOR('',#46461,10.);
#13166=VECTOR('',#46462,10.);
#13167=VECTOR('',#46465,10.);
#13168=VECTOR('',#46466,10.);
#13169=VECTOR('',#46467,10.);
#13170=VECTOR('',#46470,10.);
#13171=VECTOR('',#46471,10.);
#13172=VECTOR('',#46472,10.);
#13173=VECTOR('',#46475,10.);
#13174=VECTOR('',#46476,10.);
#13175=VECTOR('',#46477,10.);
#13176=VECTOR('',#46480,10.);
#13177=VECTOR('',#46501,10.);
#13178=VECTOR('',#46508,10.);
#13179=VECTOR('',#46521,10.);
#13180=VECTOR('',#46524,10.);
#13181=VECTOR('',#46535,10.);
#13182=VECTOR('',#46538,10.);
#13183=VECTOR('',#46557,10.);
#13184=VECTOR('',#46560,10.);
#13185=VECTOR('',#46561,10.);
#13186=VECTOR('',#46580,10.);
#13187=VECTOR('',#46587,10.);
#13188=VECTOR('',#46600,10.);
#13189=VECTOR('',#46603,10.);
#13190=VECTOR('',#46614,10.);
#13191=VECTOR('',#46617,10.);
#13192=VECTOR('',#46636,10.);
#13193=VECTOR('',#46639,10.);
#13194=VECTOR('',#46640,10.);
#13195=VECTOR('',#46659,10.);
#13196=VECTOR('',#46664,10.);
#13197=VECTOR('',#46667,10.);
#13198=VECTOR('',#46686,10.);
#13199=VECTOR('',#46689,10.);
#13200=VECTOR('',#46700,10.);
#13201=VECTOR('',#46733,10.);
#13202=VECTOR('',#46736,10.);
#13203=VECTOR('',#46741,10.);
#13204=VECTOR('',#46742,10.);
#13205=VECTOR('',#46747,10.);
#13206=VECTOR('',#46750,10.);
#13207=VECTOR('',#46769,10.);
#13208=VECTOR('',#46772,10.);
#13209=VECTOR('',#46783,10.);
#13210=VECTOR('',#46816,10.);
#13211=VECTOR('',#46819,10.);
#13212=VECTOR('',#46824,10.);
#13213=VECTOR('',#46825,10.);
#13214=VECTOR('',#46830,10.);
#13215=VECTOR('',#46833,10.);
#13216=VECTOR('',#46844,10.);
#13217=VECTOR('',#46847,10.);
#13218=VECTOR('',#46856,10.);
#13219=VECTOR('',#46857,10.);
#13220=VECTOR('',#46860,10.);
#13221=VECTOR('',#46861,10.);
#13222=VECTOR('',#46862,10.);
#13223=VECTOR('',#46865,10.);
#13224=VECTOR('',#46866,10.);
#13225=VECTOR('',#46867,10.);
#13226=VECTOR('',#46870,10.);
#13227=VECTOR('',#46871,10.);
#13228=VECTOR('',#46872,10.);
#13229=VECTOR('',#46875,10.);
#13230=VECTOR('',#46876,10.);
#13231=VECTOR('',#46877,10.);
#13232=VECTOR('',#46880,10.);
#13233=VECTOR('',#46881,10.);
#13234=VECTOR('',#46882,10.);
#13235=VECTOR('',#46885,10.);
#13236=VECTOR('',#46886,10.);
#13237=VECTOR('',#46887,10.);
#13238=VECTOR('',#46890,10.);
#13239=VECTOR('',#46891,10.);
#13240=VECTOR('',#46892,10.);
#13241=VECTOR('',#46895,10.);
#13242=VECTOR('',#46896,10.);
#13243=VECTOR('',#46897,10.);
#13244=VECTOR('',#46900,10.);
#13245=VECTOR('',#46901,10.);
#13246=VECTOR('',#46902,10.);
#13247=VECTOR('',#46905,10.);
#13248=VECTOR('',#46906,10.);
#13249=VECTOR('',#46907,10.);
#13250=VECTOR('',#46910,10.);
#13251=VECTOR('',#46911,10.);
#13252=VECTOR('',#46912,10.);
#13253=VECTOR('',#46915,10.);
#13254=VECTOR('',#46916,10.);
#13255=VECTOR('',#46917,10.);
#13256=VECTOR('',#46920,10.);
#13257=VECTOR('',#46921,10.);
#13258=VECTOR('',#46922,10.);
#13259=VECTOR('',#46925,10.);
#13260=VECTOR('',#46926,10.);
#13261=VECTOR('',#46927,10.);
#13262=VECTOR('',#46930,10.);
#13263=VECTOR('',#46931,10.);
#13264=VECTOR('',#46932,10.);
#13265=VECTOR('',#46935,10.);
#13266=VECTOR('',#46936,10.);
#13267=VECTOR('',#46937,10.);
#13268=VECTOR('',#46940,10.);
#13269=VECTOR('',#46941,10.);
#13270=VECTOR('',#46942,10.);
#13271=VECTOR('',#46945,10.);
#13272=VECTOR('',#46946,10.);
#13273=VECTOR('',#46947,10.);
#13274=VECTOR('',#46948,10.);
#13275=VECTOR('',#46949,10.);
#13276=VECTOR('',#46952,10.);
#13277=VECTOR('',#46953,10.);
#13278=VECTOR('',#46954,10.);
#13279=VECTOR('',#46957,10.);
#13280=VECTOR('',#46958,10.);
#13281=VECTOR('',#46959,10.);
#13282=VECTOR('',#46962,10.);
#13283=VECTOR('',#46963,10.);
#13284=VECTOR('',#46964,10.);
#13285=VECTOR('',#46967,10.);
#13286=VECTOR('',#46968,10.);
#13287=VECTOR('',#46971,10.);
#13288=VECTOR('',#46972,10.);
#13289=VECTOR('',#46975,10.);
#13290=VECTOR('',#46976,10.);
#13291=VECTOR('',#46977,10.);
#13292=VECTOR('',#46980,10.);
#13293=VECTOR('',#46981,10.);
#13294=VECTOR('',#46982,10.);
#13295=VECTOR('',#46985,10.);
#13296=VECTOR('',#46986,10.);
#13297=VECTOR('',#46987,10.);
#13298=VECTOR('',#46990,10.);
#13299=VECTOR('',#46991,10.);
#13300=VECTOR('',#46992,10.);
#13301=VECTOR('',#46993,10.);
#13302=VECTOR('',#46994,10.);
#13303=VECTOR('',#46997,10.);
#13304=VECTOR('',#46998,10.);
#13305=VECTOR('',#47001,10.);
#13306=VECTOR('',#47002,10.);
#13307=VECTOR('',#47003,10.);
#13308=VECTOR('',#47006,10.);
#13309=VECTOR('',#47007,10.);
#13310=VECTOR('',#47008,10.);
#13311=VECTOR('',#47011,10.);
#13312=VECTOR('',#47012,10.);
#13313=VECTOR('',#47013,10.);
#13314=VECTOR('',#47016,10.);
#13315=VECTOR('',#47017,10.);
#13316=VECTOR('',#47018,10.);
#13317=VECTOR('',#47021,10.);
#13318=VECTOR('',#47022,10.);
#13319=VECTOR('',#47025,10.);
#13320=VECTOR('',#47026,10.);
#13321=VECTOR('',#47029,10.);
#13322=VECTOR('',#47030,10.);
#13323=VECTOR('',#47031,10.);
#13324=VECTOR('',#47034,10.);
#13325=VECTOR('',#47035,10.);
#13326=VECTOR('',#47036,10.);
#13327=VECTOR('',#47039,10.);
#13328=VECTOR('',#47040,10.);
#13329=VECTOR('',#47041,10.);
#13330=VECTOR('',#47044,10.);
#13331=VECTOR('',#47045,10.);
#13332=VECTOR('',#47046,10.);
#13333=VECTOR('',#47049,10.);
#13334=VECTOR('',#47050,10.);
#13335=VECTOR('',#47051,10.);
#13336=VECTOR('',#47054,10.);
#13337=VECTOR('',#47055,10.);
#13338=VECTOR('',#47056,10.);
#13339=VECTOR('',#47059,10.);
#13340=VECTOR('',#47060,10.);
#13341=VECTOR('',#47061,10.);
#13342=VECTOR('',#47064,10.);
#13343=VECTOR('',#47065,10.);
#13344=VECTOR('',#47066,10.);
#13345=VECTOR('',#47069,10.);
#13346=VECTOR('',#47070,10.);
#13347=VECTOR('',#47071,10.);
#13348=VECTOR('',#47074,10.);
#13349=VECTOR('',#47075,10.);
#13350=VECTOR('',#47076,10.);
#13351=VECTOR('',#47079,10.);
#13352=VECTOR('',#47080,10.);
#13353=VECTOR('',#47103,10.);
#13354=VECTOR('',#47110,10.);
#13355=VECTOR('',#47121,10.);
#13356=VECTOR('',#47124,10.);
#13357=VECTOR('',#47149,10.);
#13358=VECTOR('',#47156,10.);
#13359=VECTOR('',#47167,10.);
#13360=VECTOR('',#47170,10.);
#13361=VECTOR('',#47195,10.);
#13362=VECTOR('',#47202,10.);
#13363=VECTOR('',#47209,10.);
#13364=VECTOR('',#47228,10.);
#13365=VECTOR('',#47231,10.);
#13366=VECTOR('',#47250,10.);
#13367=VECTOR('',#47255,10.);
#13368=VECTOR('',#47260,10.);
#13369=VECTOR('',#47269,10.);
#13370=VECTOR('',#47276,10.);
#13371=VECTOR('',#47287,10.);
#13372=VECTOR('',#47290,10.);
#13373=VECTOR('',#47315,10.);
#13374=VECTOR('',#47322,10.);
#13375=VECTOR('',#47333,10.);
#13376=VECTOR('',#47336,10.);
#13377=VECTOR('',#47361,10.);
#13378=VECTOR('',#47368,10.);
#13379=VECTOR('',#47379,10.);
#13380=VECTOR('',#47382,10.);
#13381=VECTOR('',#47403,10.);
#13382=VECTOR('',#47410,10.);
#13383=VECTOR('',#47429,10.);
#13384=VECTOR('',#47432,10.);
#13385=VECTOR('',#47451,10.);
#13386=VECTOR('',#47456,10.);
#13387=VECTOR('',#47461,10.);
#13388=VECTOR('',#47470,10.);
#13389=VECTOR('',#47489,10.);
#13390=VECTOR('',#47496,10.);
#13391=VECTOR('',#47499,10.);
#13392=VECTOR('',#47508,10.);
#13393=VECTOR('',#47519,10.);
#13394=VECTOR('',#47522,10.);
#13395=VECTOR('',#47529,10.);
#13396=VECTOR('',#47540,10.);
#13397=VECTOR('',#47543,10.);
#13398=VECTOR('',#47568,10.);
#13399=VECTOR('',#47577,10.);
#13400=VECTOR('',#47588,10.);
#13401=VECTOR('',#47591,10.);
#13402=VECTOR('',#47598,10.);
#13403=VECTOR('',#47609,10.);
#13404=VECTOR('',#47612,10.);
#13405=VECTOR('',#47635,10.);
#13406=VECTOR('',#47646,10.);
#13407=VECTOR('',#47649,10.);
#13408=VECTOR('',#47652,10.);
#13409=VECTOR('',#47671,10.);
#13410=VECTOR('',#47678,10.);
#13411=VECTOR('',#47681,10.);
#13412=VECTOR('',#47684,10.);
#13413=VECTOR('',#47687,10.);
#13414=VECTOR('',#47690,10.);
#13415=VECTOR('',#47697,10.);
#13416=VECTOR('',#47708,10.);
#13417=VECTOR('',#47711,10.);
#13418=VECTOR('',#47732,10.);
#13419=VECTOR('',#47743,10.);
#13420=VECTOR('',#47746,10.);
#13421=VECTOR('',#47771,10.);
#13422=VECTOR('',#47778,10.);
#13423=VECTOR('',#47789,10.);
#13424=VECTOR('',#47792,10.);
#13425=VECTOR('',#47817,10.);
#13426=VECTOR('',#47826,10.);
#13427=VECTOR('',#47837,10.);
#13428=VECTOR('',#47840,10.);
#13429=VECTOR('',#47847,10.);
#13430=VECTOR('',#47858,10.);
#13431=VECTOR('',#47861,10.);
#13432=VECTOR('',#47886,10.);
#13433=VECTOR('',#47895,10.);
#13434=VECTOR('',#47906,10.);
#13435=VECTOR('',#47909,10.);
#13436=VECTOR('',#47912,10.);
#13437=VECTOR('',#47915,10.);
#13438=VECTOR('',#47918,10.);
#13439=VECTOR('',#47925,10.);
#13440=VECTOR('',#47936,10.);
#13441=VECTOR('',#47939,10.);
#13442=VECTOR('',#47964,10.);
#13443=VECTOR('',#47971,10.);
#13444=VECTOR('',#47982,10.);
#13445=VECTOR('',#47985,10.);
#13446=VECTOR('',#48010,10.);
#13447=VECTOR('',#48017,10.);
#13448=VECTOR('',#48028,10.);
#13449=VECTOR('',#48031,10.);
#13450=VECTOR('',#48054,10.);
#13451=VECTOR('',#48065,10.);
#13452=VECTOR('',#48068,10.);
#13453=VECTOR('',#48077,10.);
#13454=VECTOR('',#48088,10.);
#13455=VECTOR('',#48091,10.);
#13456=VECTOR('',#48098,10.);
#13457=VECTOR('',#48109,10.);
#13458=VECTOR('',#48112,10.);
#13459=VECTOR('',#48137,10.);
#13460=VECTOR('',#48146,10.);
#13461=VECTOR('',#48157,10.);
#13462=VECTOR('',#48160,10.);
#13463=VECTOR('',#48163,10.);
#13464=VECTOR('',#48166,10.);
#13465=VECTOR('',#48169,10.);
#13466=VECTOR('',#48172,10.);
#13467=VECTOR('',#48175,10.);
#13468=VECTOR('',#48178,10.);
#13469=VECTOR('',#48197,10.);
#13470=VECTOR('',#48204,10.);
#13471=VECTOR('',#48207,10.);
#13472=VECTOR('',#48216,10.);
#13473=VECTOR('',#48227,10.);
#13474=VECTOR('',#48230,10.);
#13475=VECTOR('',#48237,10.);
#13476=VECTOR('',#48248,10.);
#13477=VECTOR('',#48251,10.);
#13478=VECTOR('',#48274,10.);
#13479=VECTOR('',#48285,10.);
#13480=VECTOR('',#48288,10.);
#13481=VECTOR('',#48295,10.);
#13482=VECTOR('',#48306,10.);
#13483=VECTOR('',#48309,10.);
#13484=VECTOR('',#48334,10.);
#13485=VECTOR('',#48343,10.);
#13486=VECTOR('',#48354,10.);
#13487=VECTOR('',#48357,10.);
#13488=VECTOR('',#48360,10.);
#13489=VECTOR('',#48363,10.);
#13490=VECTOR('',#48366,10.);
#13491=VECTOR('',#48385,10.);
#13492=VECTOR('',#48392,10.);
#13493=VECTOR('',#48395,10.);
#13494=VECTOR('',#48398,10.);
#13495=VECTOR('',#48401,10.);
#13496=VECTOR('',#48404,10.);
#13497=VECTOR('',#48411,10.);
#13498=VECTOR('',#48422,10.);
#13499=VECTOR('',#48425,10.);
#13500=VECTOR('',#48450,10.);
#13501=VECTOR('',#48457,10.);
#13502=VECTOR('',#48468,10.);
#13503=VECTOR('',#48471,10.);
#13504=VECTOR('',#48496,10.);
#13505=VECTOR('',#48503,10.);
#13506=VECTOR('',#48514,10.);
#13507=VECTOR('',#48517,10.);
#13508=VECTOR('',#48538,10.);
#13509=VECTOR('',#48549,10.);
#13510=VECTOR('',#48552,10.);
#13511=VECTOR('',#48577,10.);
#13512=VECTOR('',#48586,10.);
#13513=VECTOR('',#48597,10.);
#13514=VECTOR('',#48600,10.);
#13515=VECTOR('',#48619,10.);
#13516=VECTOR('',#48626,10.);
#13517=VECTOR('',#48629,10.);
#13518=VECTOR('',#48636,10.);
#13519=VECTOR('',#48647,10.);
#13520=VECTOR('',#48650,10.);
#13521=VECTOR('',#48675,10.);
#13522=VECTOR('',#48682,10.);
#13523=VECTOR('',#48693,10.);
#13524=VECTOR('',#48696,10.);
#13525=VECTOR('',#48719,10.);
#13526=VECTOR('',#48730,10.);
#13527=VECTOR('',#48733,10.);
#13528=VECTOR('',#48742,10.);
#13529=VECTOR('',#48753,10.);
#13530=VECTOR('',#48756,10.);
#13531=VECTOR('',#48763,10.);
#13532=VECTOR('',#48774,10.);
#13533=VECTOR('',#48777,10.);
#13534=VECTOR('',#48802,10.);
#13535=VECTOR('',#48811,10.);
#13536=VECTOR('',#48822,10.);
#13537=VECTOR('',#48825,10.);
#13538=VECTOR('',#48828,10.);
#13539=VECTOR('',#48837,10.);
#13540=VECTOR('',#48848,10.);
#13541=VECTOR('',#48851,10.);
#13542=VECTOR('',#48854,10.);
#13543=VECTOR('',#48857,10.);
#13544=VECTOR('',#48860,10.);
#13545=VECTOR('',#48863,10.);
#13546=VECTOR('',#48866,10.);
#13547=VECTOR('',#48869,10.);
#13548=VECTOR('',#48888,10.);
#13549=VECTOR('',#48895,10.);
#13550=VECTOR('',#48898,10.);
#13551=VECTOR('',#48907,10.);
#13552=VECTOR('',#48918,10.);
#13553=VECTOR('',#48921,10.);
#13554=VECTOR('',#48928,10.);
#13555=VECTOR('',#48939,10.);
#13556=VECTOR('',#48942,10.);
#13557=VECTOR('',#48967,10.);
#13558=VECTOR('',#48976,10.);
#13559=VECTOR('',#48987,10.);
#13560=VECTOR('',#48990,10.);
#13561=VECTOR('',#48993,10.);
#13562=VECTOR('',#49000,10.);
#13563=VECTOR('',#49011,10.);
#13564=VECTOR('',#49014,10.);
#13565=VECTOR('',#49039,10.);
#13566=VECTOR('',#49046,10.);
#13567=VECTOR('',#49057,10.);
#13568=VECTOR('',#49060,10.);
#13569=VECTOR('',#49085,10.);
#13570=VECTOR('',#49094,10.);
#13571=VECTOR('',#49105,10.);
#13572=VECTOR('',#49108,10.);
#13573=VECTOR('',#49115,10.);
#13574=VECTOR('',#49126,10.);
#13575=VECTOR('',#49129,10.);
#13576=VECTOR('',#49150,10.);
#13577=VECTOR('',#49161,10.);
#13578=VECTOR('',#49164,10.);
#13579=VECTOR('',#49189,10.);
#13580=VECTOR('',#49210,10.);
#13581=VECTOR('',#49221,10.);
#13582=VECTOR('',#49224,10.);
#13583=VECTOR('',#49257,10.);
#13584=VECTOR('',#49264,10.);
#13585=VECTOR('',#49267,10.);
#13586=VECTOR('',#49276,10.);
#13587=VECTOR('',#49287,10.);
#13588=VECTOR('',#49290,10.);
#13589=VECTOR('',#49309,10.);
#13590=VECTOR('',#49316,10.);
#13591=VECTOR('',#49319,10.);
#13592=VECTOR('',#49322,10.);
#13593=VECTOR('',#49325,10.);
#13594=VECTOR('',#49328,10.);
#13595=VECTOR('',#49337,10.);
#13596=VECTOR('',#49348,10.);
#13597=VECTOR('',#49351,10.);
#13598=VECTOR('',#49360,10.);
#13599=VECTOR('',#49371,10.);
#13600=VECTOR('',#49374,10.);
#13601=VECTOR('',#49381,10.);
#13602=VECTOR('',#49392,10.);
#13603=VECTOR('',#49395,10.);
#13604=VECTOR('',#49420,10.);
#13605=VECTOR('',#49429,10.);
#13606=VECTOR('',#49440,10.);
#13607=VECTOR('',#49443,10.);
#13608=VECTOR('',#49446,10.);
#13609=VECTOR('',#49449,10.);
#13610=VECTOR('',#49452,10.);
#13611=VECTOR('',#49455,10.);
#13612=VECTOR('',#49458,10.);
#13613=VECTOR('',#49461,10.);
#13614=VECTOR('',#49468,10.);
#13615=VECTOR('',#49479,10.);
#13616=VECTOR('',#49482,10.);
#13617=VECTOR('',#49507,10.);
#13618=VECTOR('',#49514,10.);
#13619=VECTOR('',#49525,10.);
#13620=VECTOR('',#49528,10.);
#13621=VECTOR('',#49549,10.);
#13622=VECTOR('',#49560,10.);
#13623=VECTOR('',#49563,10.);
#13624=VECTOR('',#49588,10.);
#13625=VECTOR('',#49595,10.);
#13626=VECTOR('',#49606,10.);
#13627=VECTOR('',#49609,10.);
#13628=VECTOR('',#49634,10.);
#13629=VECTOR('',#49641,10.);
#13630=VECTOR('',#49652,10.);
#13631=VECTOR('',#49655,10.);
#13632=VECTOR('',#49688,10.);
#13633=VECTOR('',#49695,10.);
#13634=VECTOR('',#49698,10.);
#13635=VECTOR('',#49707,10.);
#13636=VECTOR('',#49718,10.);
#13637=VECTOR('',#49721,10.);
#13638=VECTOR('',#49730,10.);
#13639=VECTOR('',#49741,10.);
#13640=VECTOR('',#49744,10.);
#13641=VECTOR('',#49763,10.);
#13642=VECTOR('',#49770,10.);
#13643=VECTOR('',#49773,10.);
#13644=VECTOR('',#49776,10.);
#13645=VECTOR('',#49777,10.);
#13646=VECTOR('',#49780,10.);
#13647=VECTOR('',#49783,10.);
#13648=VECTOR('',#49788,10.);
#13649=VECTOR('',#49791,10.);
#13650=VECTOR('',#49802,10.);
#13651=VECTOR('',#49813,10.);
#13652=VECTOR('',#49816,10.);
#13653=VECTOR('',#49823,10.);
#13654=VECTOR('',#49834,10.);
#13655=VECTOR('',#49837,10.);
#13656=VECTOR('',#49884,10.);
#13657=VECTOR('',#49891,10.);
#13658=VECTOR('',#49894,10.);
#13659=VECTOR('',#49897,10.);
#13660=VECTOR('',#49900,10.);
#13661=VECTOR('',#49903,10.);
#13662=VECTOR('',#49916,10.);
#13663=VECTOR('',#49925,10.);
#13664=VECTOR('',#49926,10.);
#13665=VECTOR('',#49927,10.);
#13666=VECTOR('',#49934,10.);
#13667=VECTOR('',#49937,10.);
#13668=VECTOR('',#49938,10.);
#13669=VECTOR('',#49941,10.);
#13670=VECTOR('',#49942,10.);
#13671=VECTOR('',#49947,10.);
#13672=VECTOR('',#49950,10.);
#13673=VECTOR('',#49953,10.);
#13674=VECTOR('',#49960,10.);
#13675=VECTOR('',#49963,10.);
#13676=VECTOR('',#49970,10.);
#13677=VECTOR('',#49973,10.);
#13678=VECTOR('',#49974,10.);
#13679=VECTOR('',#49977,10.);
#13680=VECTOR('',#49978,10.);
#13681=VECTOR('',#49987,10.);
#13682=VECTOR('',#49990,10.);
#13683=VECTOR('',#49993,10.);
#13684=VECTOR('',#49996,10.);
#13685=VECTOR('',#49999,10.);
#13686=VECTOR('',#50006,10.);
#13687=VECTOR('',#50009,10.);
#13688=VECTOR('',#50010,10.);
#13689=VECTOR('',#50013,10.);
#13690=VECTOR('',#50014,10.);
#13691=VECTOR('',#50023,10.);
#13692=VECTOR('',#50026,10.);
#13693=VECTOR('',#50033,10.);
#13694=VECTOR('',#50036,10.);
#13695=VECTOR('',#50039,10.);
#13696=VECTOR('',#50052,10.);
#13697=VECTOR('',#50059,10.);
#13698=VECTOR('',#50062,10.);
#13699=VECTOR('',#50063,10.);
#13700=VECTOR('',#50066,10.);
#13701=VECTOR('',#50073,10.);
#13702=VECTOR('',#50076,10.);
#13703=VECTOR('',#50083,10.);
#13704=VECTOR('',#50086,10.);
#13705=VECTOR('',#50087,10.);
#13706=VECTOR('',#50090,10.);
#13707=VECTOR('',#50091,10.);
#13708=VECTOR('',#50096,10.);
#13709=VECTOR('',#50099,10.);
#13710=VECTOR('',#50102,10.);
#13711=VECTOR('',#50111,10.);
#13712=VECTOR('',#50114,10.);
#13713=VECTOR('',#50115,10.);
#13714=VECTOR('',#50122,10.);
#13715=VECTOR('',#50125,10.);
#13716=VECTOR('',#50126,10.);
#13717=VECTOR('',#50129,10.);
#13718=VECTOR('',#50130,10.);
#13719=VECTOR('',#50139,10.);
#13720=VECTOR('',#50142,10.);
#13721=VECTOR('',#50145,10.);
#13722=VECTOR('',#50148,10.);
#13723=VECTOR('',#50151,10.);
#13724=VECTOR('',#50158,10.);
#13725=VECTOR('',#50161,10.);
#13726=VECTOR('',#50162,10.);
#13727=VECTOR('',#50165,10.);
#13728=VECTOR('',#50166,10.);
#13729=VECTOR('',#50175,10.);
#13730=VECTOR('',#50178,10.);
#13731=VECTOR('',#50185,10.);
#13732=VECTOR('',#50188,10.);
#13733=VECTOR('',#50191,10.);
#13734=VECTOR('',#50204,10.);
#13735=VECTOR('',#50211,10.);
#13736=VECTOR('',#50214,10.);
#13737=VECTOR('',#50215,10.);
#13738=VECTOR('',#50218,10.);
#13739=VECTOR('',#50227,10.);
#13740=VECTOR('',#50230,10.);
#13741=VECTOR('',#50231,10.);
#13742=VECTOR('',#50238,10.);
#13743=VECTOR('',#50241,10.);
#13744=VECTOR('',#50242,10.);
#13745=VECTOR('',#50245,10.);
#13746=VECTOR('',#50246,10.);
#13747=VECTOR('',#50251,10.);
#13748=VECTOR('',#50254,10.);
#13749=VECTOR('',#50257,10.);
#13750=VECTOR('',#50264,10.);
#13751=VECTOR('',#50267,10.);
#13752=VECTOR('',#50274,10.);
#13753=VECTOR('',#50277,10.);
#13754=VECTOR('',#50278,10.);
#13755=VECTOR('',#50281,10.);
#13756=VECTOR('',#50282,10.);
#13757=VECTOR('',#50291,10.);
#13758=VECTOR('',#50294,10.);
#13759=VECTOR('',#50297,10.);
#13760=VECTOR('',#50300,10.);
#13761=VECTOR('',#50303,10.);
#13762=VECTOR('',#50310,10.);
#13763=VECTOR('',#50313,10.);
#13764=VECTOR('',#50314,10.);
#13765=VECTOR('',#50317,10.);
#13766=VECTOR('',#50318,10.);
#13767=VECTOR('',#50327,10.);
#13768=VECTOR('',#50330,10.);
#13769=VECTOR('',#50337,10.);
#13770=VECTOR('',#50340,10.);
#13771=VECTOR('',#50343,10.);
#13772=VECTOR('',#50356,10.);
#13773=VECTOR('',#50363,10.);
#13774=VECTOR('',#50366,10.);
#13775=VECTOR('',#50367,10.);
#13776=VECTOR('',#50370,10.);
#13777=VECTOR('',#50377,10.);
#13778=VECTOR('',#50380,10.);
#13779=VECTOR('',#50387,10.);
#13780=VECTOR('',#50390,10.);
#13781=VECTOR('',#50393,10.);
#13782=VECTOR('',#50412,10.);
#13783=VECTOR('',#50417,10.);
#13784=VECTOR('',#50422,10.);
#13785=VECTOR('',#50425,10.);
#13786=VECTOR('',#50428,10.);
#13787=VECTOR('',#50429,10.);
#13788=VECTOR('',#50432,10.);
#13789=VECTOR('',#50439,10.);
#13790=VECTOR('',#50442,10.);
#13791=VECTOR('',#50449,10.);
#13792=VECTOR('',#50452,10.);
#13793=VECTOR('',#50453,10.);
#13794=VECTOR('',#50456,10.);
#13795=VECTOR('',#50457,10.);
#13796=VECTOR('',#50466,10.);
#13797=VECTOR('',#50469,10.);
#13798=VECTOR('',#50472,10.);
#13799=VECTOR('',#50475,10.);
#13800=VECTOR('',#50478,10.);
#13801=VECTOR('',#50485,10.);
#13802=VECTOR('',#50488,10.);
#13803=VECTOR('',#50489,10.);
#13804=VECTOR('',#50492,10.);
#13805=VECTOR('',#50493,10.);
#13806=VECTOR('',#50502,10.);
#13807=VECTOR('',#50513,10.);
#13808=VECTOR('',#50516,10.);
#13809=VECTOR('',#50551,10.);
#13810=VECTOR('',#50562,10.);
#13811=VECTOR('',#50569,10.);
#13812=VECTOR('',#50588,10.);
#13813=VECTOR('',#50591,10.);
#13814=VECTOR('',#50610,10.);
#13815=VECTOR('',#50615,10.);
#13816=VECTOR('',#50620,10.);
#13817=VECTOR('',#50629,10.);
#13818=VECTOR('',#50648,10.);
#13819=VECTOR('',#50675,33.);
#13820=VECTOR('',#50712,10.);
#13821=VECTOR('',#50715,10.);
#13822=VECTOR('',#50716,10.);
#13823=VECTOR('',#50721,10.);
#13824=VECTOR('',#50724,10.);
#13825=VECTOR('',#50725,10.);
#13826=VECTOR('',#50734,10.);
#13827=VECTOR('',#50737,10.);
#13828=VECTOR('',#50738,10.);
#13829=VECTOR('',#50751,10.);
#13830=VECTOR('',#50754,10.);
#13831=VECTOR('',#50757,10.);
#13832=VECTOR('',#50770,10.);
#13833=VECTOR('',#50773,10.);
#13834=VECTOR('',#50776,10.);
#13835=VECTOR('',#50779,10.);
#13836=VECTOR('',#50782,10.);
#13837=VECTOR('',#50795,10.);
#13838=VECTOR('',#50798,10.);
#13839=VECTOR('',#50801,10.);
#13840=VECTOR('',#50810,10.);
#13841=VECTOR('',#50819,10.);
#13842=VECTOR('',#50822,10.);
#13843=VECTOR('',#50835,10.);
#13844=VECTOR('',#50838,10.);
#13845=VECTOR('',#50841,10.);
#13846=VECTOR('',#50854,10.);
#13847=VECTOR('',#50857,10.);
#13848=VECTOR('',#50860,10.);
#13849=VECTOR('',#50873,10.);
#13850=VECTOR('',#50876,10.);
#13851=VECTOR('',#50879,10.);
#13852=VECTOR('',#50890,10.);
#13853=VECTOR('',#50897,10.);
#13854=VECTOR('',#50900,10.);
#13855=VECTOR('',#50913,10.);
#13856=VECTOR('',#50916,10.);
#13857=VECTOR('',#50919,10.);
#13858=VECTOR('',#50932,10.);
#13859=VECTOR('',#50935,10.);
#13860=VECTOR('',#50938,10.);
#13861=VECTOR('',#50941,10.);
#13862=VECTOR('',#50944,10.);
#13863=VECTOR('',#50955,10.);
#13864=VECTOR('',#50960,10.);
#13865=VECTOR('',#50963,10.);
#13866=VECTOR('',#50966,10.);
#13867=VECTOR('',#50981,10.);
#13868=VECTOR('',#50984,10.);
#13869=VECTOR('',#50997,10.);
#13870=VECTOR('',#51000,10.);
#13871=VECTOR('',#51003,10.);
#13872=VECTOR('',#51016,10.);
#13873=VECTOR('',#51019,10.);
#13874=VECTOR('',#51022,10.);
#13875=VECTOR('',#51025,10.);
#13876=VECTOR('',#51028,10.);
#13877=VECTOR('',#51041,10.);
#13878=VECTOR('',#51044,10.);
#13879=VECTOR('',#51047,10.);
#13880=VECTOR('',#51060,10.);
#13881=VECTOR('',#51061,10.);
#13882=VECTOR('',#51064,10.);
#13883=VECTOR('',#51069,10.);
#13884=VECTOR('',#51072,10.);
#13885=VECTOR('',#51077,10.);
#13886=VECTOR('',#51224,10.);
#15741=VERTEX_POINT('',#68018);
#15742=VERTEX_POINT('',#68019);
#15743=VERTEX_POINT('',#68021);
#15744=VERTEX_POINT('',#68023);
#15745=VERTEX_POINT('',#68046);
#15746=VERTEX_POINT('',#68047);
#15747=VERTEX_POINT('',#68049);
#15748=VERTEX_POINT('',#68062);
#15749=VERTEX_POINT('',#68063);
#15750=VERTEX_POINT('',#68065);
#15751=VERTEX_POINT('',#68067);
#15752=VERTEX_POINT('',#68071);
#15753=VERTEX_POINT('',#68072);
#15754=VERTEX_POINT('',#68074);
#15755=VERTEX_POINT('',#68076);
#15756=VERTEX_POINT('',#68087);
#15757=VERTEX_POINT('',#68090);
#15758=VERTEX_POINT('',#68122);
#15759=VERTEX_POINT('',#68124);
#15760=VERTEX_POINT('',#68141);
#15761=VERTEX_POINT('',#68143);
#15762=VERTEX_POINT('',#68145);
#15763=VERTEX_POINT('',#68147);
#15764=VERTEX_POINT('',#68156);
#15765=VERTEX_POINT('',#68158);
#15766=VERTEX_POINT('',#68160);
#15767=VERTEX_POINT('',#68162);
#15768=VERTEX_POINT('',#68164);
#15769=VERTEX_POINT('',#68166);
#15770=VERTEX_POINT('',#68168);
#15771=VERTEX_POINT('',#68170);
#15772=VERTEX_POINT('',#68172);
#15773=VERTEX_POINT('',#68174);
#15774=VERTEX_POINT('',#68176);
#15775=VERTEX_POINT('',#68178);
#15776=VERTEX_POINT('',#68180);
#15777=VERTEX_POINT('',#68182);
#15778=VERTEX_POINT('',#68184);
#15779=VERTEX_POINT('',#68186);
#15780=VERTEX_POINT('',#68188);
#15781=VERTEX_POINT('',#68190);
#15782=VERTEX_POINT('',#68192);
#15783=VERTEX_POINT('',#68194);
#15784=VERTEX_POINT('',#68196);
#15785=VERTEX_POINT('',#68198);
#15786=VERTEX_POINT('',#68200);
#15787=VERTEX_POINT('',#68202);
#15788=VERTEX_POINT('',#68204);
#15789=VERTEX_POINT('',#68206);
#15790=VERTEX_POINT('',#68208);
#15791=VERTEX_POINT('',#68210);
#15792=VERTEX_POINT('',#68212);
#15793=VERTEX_POINT('',#68214);
#15794=VERTEX_POINT('',#68216);
#15795=VERTEX_POINT('',#68218);
#15796=VERTEX_POINT('',#68220);
#15797=VERTEX_POINT('',#68222);
#15798=VERTEX_POINT('',#68224);
#15799=VERTEX_POINT('',#68226);
#15800=VERTEX_POINT('',#68228);
#15801=VERTEX_POINT('',#68230);
#15802=VERTEX_POINT('',#68232);
#15803=VERTEX_POINT('',#68234);
#15804=VERTEX_POINT('',#68236);
#15805=VERTEX_POINT('',#68238);
#15806=VERTEX_POINT('',#68240);
#15807=VERTEX_POINT('',#68242);
#15808=VERTEX_POINT('',#68244);
#15809=VERTEX_POINT('',#68246);
#15810=VERTEX_POINT('',#68248);
#15811=VERTEX_POINT('',#68250);
#15812=VERTEX_POINT('',#68252);
#15813=VERTEX_POINT('',#68254);
#15814=VERTEX_POINT('',#68256);
#15815=VERTEX_POINT('',#68258);
#15816=VERTEX_POINT('',#68260);
#15817=VERTEX_POINT('',#68262);
#15818=VERTEX_POINT('',#68264);
#15819=VERTEX_POINT('',#68266);
#15820=VERTEX_POINT('',#68268);
#15821=VERTEX_POINT('',#68270);
#15822=VERTEX_POINT('',#68272);
#15823=VERTEX_POINT('',#68274);
#15824=VERTEX_POINT('',#68276);
#15825=VERTEX_POINT('',#68278);
#15826=VERTEX_POINT('',#68280);
#15827=VERTEX_POINT('',#68282);
#15828=VERTEX_POINT('',#68284);
#15829=VERTEX_POINT('',#68286);
#15830=VERTEX_POINT('',#68288);
#15831=VERTEX_POINT('',#68290);
#15832=VERTEX_POINT('',#68292);
#15833=VERTEX_POINT('',#68294);
#15834=VERTEX_POINT('',#68296);
#15835=VERTEX_POINT('',#68298);
#15836=VERTEX_POINT('',#68300);
#15837=VERTEX_POINT('',#68302);
#15838=VERTEX_POINT('',#68304);
#15839=VERTEX_POINT('',#68306);
#15840=VERTEX_POINT('',#68308);
#15841=VERTEX_POINT('',#68310);
#15842=VERTEX_POINT('',#68312);
#15843=VERTEX_POINT('',#68314);
#15844=VERTEX_POINT('',#68316);
#15845=VERTEX_POINT('',#68318);
#15846=VERTEX_POINT('',#68320);
#15847=VERTEX_POINT('',#68322);
#15848=VERTEX_POINT('',#68324);
#15849=VERTEX_POINT('',#68326);
#15850=VERTEX_POINT('',#68328);
#15851=VERTEX_POINT('',#68330);
#15852=VERTEX_POINT('',#68332);
#15853=VERTEX_POINT('',#68334);
#15854=VERTEX_POINT('',#68336);
#15855=VERTEX_POINT('',#68338);
#15856=VERTEX_POINT('',#68340);
#15857=VERTEX_POINT('',#68342);
#15858=VERTEX_POINT('',#68344);
#15859=VERTEX_POINT('',#68346);
#15860=VERTEX_POINT('',#68348);
#15861=VERTEX_POINT('',#68350);
#15862=VERTEX_POINT('',#68352);
#15863=VERTEX_POINT('',#68354);
#15864=VERTEX_POINT('',#68356);
#15865=VERTEX_POINT('',#68358);
#15866=VERTEX_POINT('',#68360);
#15867=VERTEX_POINT('',#68362);
#15868=VERTEX_POINT('',#68364);
#15869=VERTEX_POINT('',#68366);
#15870=VERTEX_POINT('',#68368);
#15871=VERTEX_POINT('',#68370);
#15872=VERTEX_POINT('',#68372);
#15873=VERTEX_POINT('',#68374);
#15874=VERTEX_POINT('',#68376);
#15875=VERTEX_POINT('',#68378);
#15876=VERTEX_POINT('',#68380);
#15877=VERTEX_POINT('',#68382);
#15878=VERTEX_POINT('',#68384);
#15879=VERTEX_POINT('',#68386);
#15880=VERTEX_POINT('',#68388);
#15881=VERTEX_POINT('',#68390);
#15882=VERTEX_POINT('',#68392);
#15883=VERTEX_POINT('',#68394);
#15884=VERTEX_POINT('',#68396);
#15885=VERTEX_POINT('',#68398);
#15886=VERTEX_POINT('',#68400);
#15887=VERTEX_POINT('',#68402);
#15888=VERTEX_POINT('',#68404);
#15889=VERTEX_POINT('',#68406);
#15890=VERTEX_POINT('',#68408);
#15891=VERTEX_POINT('',#68410);
#15892=VERTEX_POINT('',#68412);
#15893=VERTEX_POINT('',#68414);
#15894=VERTEX_POINT('',#68416);
#15895=VERTEX_POINT('',#68418);
#15896=VERTEX_POINT('',#68420);
#15897=VERTEX_POINT('',#68422);
#15898=VERTEX_POINT('',#68424);
#15899=VERTEX_POINT('',#68426);
#15900=VERTEX_POINT('',#68428);
#15901=VERTEX_POINT('',#68430);
#15902=VERTEX_POINT('',#68432);
#15903=VERTEX_POINT('',#68434);
#15904=VERTEX_POINT('',#68436);
#15905=VERTEX_POINT('',#68438);
#15906=VERTEX_POINT('',#68440);
#15907=VERTEX_POINT('',#68442);
#15908=VERTEX_POINT('',#68444);
#15909=VERTEX_POINT('',#68446);
#15910=VERTEX_POINT('',#68448);
#15911=VERTEX_POINT('',#68468);
#15912=VERTEX_POINT('',#68470);
#15913=VERTEX_POINT('',#68472);
#15914=VERTEX_POINT('',#68474);
#15915=VERTEX_POINT('',#68476);
#15916=VERTEX_POINT('',#68496);
#15917=VERTEX_POINT('',#68498);
#15918=VERTEX_POINT('',#68500);
#15919=VERTEX_POINT('',#68502);
#15920=VERTEX_POINT('',#68504);
#15921=VERTEX_POINT('',#68524);
#15922=VERTEX_POINT('',#68526);
#15923=VERTEX_POINT('',#68528);
#15924=VERTEX_POINT('',#68530);
#15925=VERTEX_POINT('',#68532);
#15926=VERTEX_POINT('',#68534);
#15927=VERTEX_POINT('',#68536);
#15928=VERTEX_POINT('',#68538);
#15929=VERTEX_POINT('',#68540);
#15930=VERTEX_POINT('',#68542);
#15931=VERTEX_POINT('',#68544);
#15932=VERTEX_POINT('',#68546);
#15933=VERTEX_POINT('',#68548);
#15934=VERTEX_POINT('',#68550);
#15935=VERTEX_POINT('',#68552);
#15936=VERTEX_POINT('',#68554);
#15937=VERTEX_POINT('',#68556);
#15938=VERTEX_POINT('',#68558);
#15939=VERTEX_POINT('',#68560);
#15940=VERTEX_POINT('',#68562);
#15941=VERTEX_POINT('',#68564);
#15942=VERTEX_POINT('',#68566);
#15943=VERTEX_POINT('',#68568);
#15944=VERTEX_POINT('',#68570);
#15945=VERTEX_POINT('',#68572);
#15946=VERTEX_POINT('',#68574);
#15947=VERTEX_POINT('',#68576);
#15948=VERTEX_POINT('',#68578);
#15949=VERTEX_POINT('',#68580);
#15950=VERTEX_POINT('',#68582);
#15951=VERTEX_POINT('',#68584);
#15952=VERTEX_POINT('',#68586);
#15953=VERTEX_POINT('',#68588);
#15954=VERTEX_POINT('',#68590);
#15955=VERTEX_POINT('',#68592);
#15956=VERTEX_POINT('',#68594);
#15957=VERTEX_POINT('',#68597);
#15958=VERTEX_POINT('',#68600);
#15959=VERTEX_POINT('',#68604);
#15960=VERTEX_POINT('',#68611);
#15961=VERTEX_POINT('',#68617);
#15962=VERTEX_POINT('',#68619);
#15963=VERTEX_POINT('',#68642);
#15964=VERTEX_POINT('',#68643);
#15965=VERTEX_POINT('',#68645);
#15966=VERTEX_POINT('',#68658);
#15967=VERTEX_POINT('',#68659);
#15968=VERTEX_POINT('',#68661);
#15969=VERTEX_POINT('',#68663);
#15970=VERTEX_POINT('',#68667);
#15971=VERTEX_POINT('',#68668);
#15972=VERTEX_POINT('',#68670);
#15973=VERTEX_POINT('',#68672);
#15974=VERTEX_POINT('',#68683);
#15975=VERTEX_POINT('',#68686);
#15976=VERTEX_POINT('',#68718);
#15977=VERTEX_POINT('',#68720);
#15978=VERTEX_POINT('',#68737);
#15979=VERTEX_POINT('',#68739);
#15980=VERTEX_POINT('',#68741);
#15981=VERTEX_POINT('',#68743);
#15982=VERTEX_POINT('',#68752);
#15983=VERTEX_POINT('',#68756);
#15984=VERTEX_POINT('',#68763);
#15985=VERTEX_POINT('',#68769);
#15986=VERTEX_POINT('',#68771);
#15987=VERTEX_POINT('',#68794);
#15988=VERTEX_POINT('',#68795);
#15989=VERTEX_POINT('',#68797);
#15990=VERTEX_POINT('',#68810);
#15991=VERTEX_POINT('',#68811);
#15992=VERTEX_POINT('',#68813);
#15993=VERTEX_POINT('',#68815);
#15994=VERTEX_POINT('',#68819);
#15995=VERTEX_POINT('',#68820);
#15996=VERTEX_POINT('',#68822);
#15997=VERTEX_POINT('',#68824);
#15998=VERTEX_POINT('',#68835);
#15999=VERTEX_POINT('',#68838);
#16000=VERTEX_POINT('',#68870);
#16001=VERTEX_POINT('',#68872);
#16002=VERTEX_POINT('',#68889);
#16003=VERTEX_POINT('',#68891);
#16004=VERTEX_POINT('',#68893);
#16005=VERTEX_POINT('',#68895);
#16006=VERTEX_POINT('',#68904);
#16007=VERTEX_POINT('',#68908);
#16008=VERTEX_POINT('',#68915);
#16009=VERTEX_POINT('',#68921);
#16010=VERTEX_POINT('',#68922);
#16011=VERTEX_POINT('',#68924);
#16012=VERTEX_POINT('',#68926);
#16013=VERTEX_POINT('',#68949);
#16014=VERTEX_POINT('',#68950);
#16015=VERTEX_POINT('',#68952);
#16016=VERTEX_POINT('',#68965);
#16017=VERTEX_POINT('',#68966);
#16018=VERTEX_POINT('',#68968);
#16019=VERTEX_POINT('',#68970);
#16020=VERTEX_POINT('',#68981);
#16021=VERTEX_POINT('',#68984);
#16022=VERTEX_POINT('',#68999);
#16023=VERTEX_POINT('',#69001);
#16024=VERTEX_POINT('',#69024);
#16025=VERTEX_POINT('',#69026);
#16026=VERTEX_POINT('',#69041);
#16027=VERTEX_POINT('',#69043);
#16028=VERTEX_POINT('',#69047);
#16029=VERTEX_POINT('',#69054);
#16030=VERTEX_POINT('',#69060);
#16031=VERTEX_POINT('',#69064);
#16032=VERTEX_POINT('',#69066);
#16033=VERTEX_POINT('',#69073);
#16034=VERTEX_POINT('',#69074);
#16035=VERTEX_POINT('',#69076);
#16036=VERTEX_POINT('',#69078);
#16037=VERTEX_POINT('',#69101);
#16038=VERTEX_POINT('',#69102);
#16039=VERTEX_POINT('',#69104);
#16040=VERTEX_POINT('',#69117);
#16041=VERTEX_POINT('',#69118);
#16042=VERTEX_POINT('',#69120);
#16043=VERTEX_POINT('',#69122);
#16044=VERTEX_POINT('',#69133);
#16045=VERTEX_POINT('',#69136);
#16046=VERTEX_POINT('',#69151);
#16047=VERTEX_POINT('',#69153);
#16048=VERTEX_POINT('',#69176);
#16049=VERTEX_POINT('',#69178);
#16050=VERTEX_POINT('',#69193);
#16051=VERTEX_POINT('',#69195);
#16052=VERTEX_POINT('',#69199);
#16053=VERTEX_POINT('',#69206);
#16054=VERTEX_POINT('',#69212);
#16055=VERTEX_POINT('',#69216);
#16056=VERTEX_POINT('',#69218);
#16057=VERTEX_POINT('',#69225);
#16058=VERTEX_POINT('',#69226);
#16059=VERTEX_POINT('',#69228);
#16060=VERTEX_POINT('',#69230);
#16061=VERTEX_POINT('',#69253);
#16062=VERTEX_POINT('',#69254);
#16063=VERTEX_POINT('',#69256);
#16064=VERTEX_POINT('',#69269);
#16065=VERTEX_POINT('',#69270);
#16066=VERTEX_POINT('',#69285);
#16067=VERTEX_POINT('',#69293);
#16068=VERTEX_POINT('',#69295);
#16069=VERTEX_POINT('',#69297);
#16070=VERTEX_POINT('',#69299);
#16071=VERTEX_POINT('',#69301);
#16072=VERTEX_POINT('',#69303);
#16073=VERTEX_POINT('',#69305);
#16074=VERTEX_POINT('',#69307);
#16075=VERTEX_POINT('',#69309);
#16076=VERTEX_POINT('',#69311);
#16077=VERTEX_POINT('',#69313);
#16078=VERTEX_POINT('',#69315);
#16079=VERTEX_POINT('',#69317);
#16080=VERTEX_POINT('',#69319);
#16081=VERTEX_POINT('',#69321);
#16082=VERTEX_POINT('',#69323);
#16083=VERTEX_POINT('',#69325);
#16084=VERTEX_POINT('',#69327);
#16085=VERTEX_POINT('',#69329);
#16086=VERTEX_POINT('',#69331);
#16087=VERTEX_POINT('',#69333);
#16088=VERTEX_POINT('',#69335);
#16089=VERTEX_POINT('',#69337);
#16090=VERTEX_POINT('',#69339);
#16091=VERTEX_POINT('',#69341);
#16092=VERTEX_POINT('',#69343);
#16093=VERTEX_POINT('',#69345);
#16094=VERTEX_POINT('',#69347);
#16095=VERTEX_POINT('',#69349);
#16096=VERTEX_POINT('',#69351);
#16097=VERTEX_POINT('',#69353);
#16098=VERTEX_POINT('',#69355);
#16099=VERTEX_POINT('',#69357);
#16100=VERTEX_POINT('',#69359);
#16101=VERTEX_POINT('',#69361);
#16102=VERTEX_POINT('',#69363);
#16103=VERTEX_POINT('',#69365);
#16104=VERTEX_POINT('',#69367);
#16105=VERTEX_POINT('',#69369);
#16106=VERTEX_POINT('',#69371);
#16107=VERTEX_POINT('',#69373);
#16108=VERTEX_POINT('',#69375);
#16109=VERTEX_POINT('',#69377);
#16110=VERTEX_POINT('',#69379);
#16111=VERTEX_POINT('',#69381);
#16112=VERTEX_POINT('',#69383);
#16113=VERTEX_POINT('',#69385);
#16114=VERTEX_POINT('',#69387);
#16115=VERTEX_POINT('',#69389);
#16116=VERTEX_POINT('',#69391);
#16117=VERTEX_POINT('',#69393);
#16118=VERTEX_POINT('',#69395);
#16119=VERTEX_POINT('',#69397);
#16120=VERTEX_POINT('',#69399);
#16121=VERTEX_POINT('',#69401);
#16122=VERTEX_POINT('',#69403);
#16123=VERTEX_POINT('',#69405);
#16124=VERTEX_POINT('',#69407);
#16125=VERTEX_POINT('',#69409);
#16126=VERTEX_POINT('',#69411);
#16127=VERTEX_POINT('',#69413);
#16128=VERTEX_POINT('',#69415);
#16129=VERTEX_POINT('',#69417);
#16130=VERTEX_POINT('',#69419);
#16131=VERTEX_POINT('',#69421);
#16132=VERTEX_POINT('',#69423);
#16133=VERTEX_POINT('',#69425);
#16134=VERTEX_POINT('',#69427);
#16135=VERTEX_POINT('',#69429);
#16136=VERTEX_POINT('',#69431);
#16137=VERTEX_POINT('',#69433);
#16138=VERTEX_POINT('',#69435);
#16139=VERTEX_POINT('',#69438);
#16140=VERTEX_POINT('',#69440);
#16141=VERTEX_POINT('',#69442);
#16142=VERTEX_POINT('',#69444);
#16143=VERTEX_POINT('',#69446);
#16144=VERTEX_POINT('',#69448);
#16145=VERTEX_POINT('',#69450);
#16146=VERTEX_POINT('',#69452);
#16147=VERTEX_POINT('',#69454);
#16148=VERTEX_POINT('',#69456);
#16149=VERTEX_POINT('',#69458);
#16150=VERTEX_POINT('',#69460);
#16151=VERTEX_POINT('',#69462);
#16152=VERTEX_POINT('',#69464);
#16153=VERTEX_POINT('',#69466);
#16154=VERTEX_POINT('',#69468);
#16155=VERTEX_POINT('',#69470);
#16156=VERTEX_POINT('',#69474);
#16157=VERTEX_POINT('',#69476);
#16158=VERTEX_POINT('',#69478);
#16159=VERTEX_POINT('',#69480);
#16160=VERTEX_POINT('',#69482);
#16161=VERTEX_POINT('',#69484);
#16162=VERTEX_POINT('',#69486);
#16163=VERTEX_POINT('',#69488);
#16164=VERTEX_POINT('',#69490);
#16165=VERTEX_POINT('',#69492);
#16166=VERTEX_POINT('',#69494);
#16167=VERTEX_POINT('',#69496);
#16168=VERTEX_POINT('',#69498);
#16169=VERTEX_POINT('',#69500);
#16170=VERTEX_POINT('',#69502);
#16171=VERTEX_POINT('',#69504);
#16172=VERTEX_POINT('',#69507);
#16173=VERTEX_POINT('',#69509);
#16174=VERTEX_POINT('',#69511);
#16175=VERTEX_POINT('',#69513);
#16176=VERTEX_POINT('',#69515);
#16177=VERTEX_POINT('',#69518);
#16178=VERTEX_POINT('',#69520);
#16179=VERTEX_POINT('',#69522);
#16180=VERTEX_POINT('',#69524);
#16181=VERTEX_POINT('',#69526);
#16182=VERTEX_POINT('',#69528);
#16183=VERTEX_POINT('',#69530);
#16184=VERTEX_POINT('',#69532);
#16185=VERTEX_POINT('',#69534);
#16186=VERTEX_POINT('',#69536);
#16187=VERTEX_POINT('',#69538);
#16188=VERTEX_POINT('',#69540);
#16189=VERTEX_POINT('',#69542);
#16190=VERTEX_POINT('',#69544);
#16191=VERTEX_POINT('',#69546);
#16192=VERTEX_POINT('',#69548);
#16193=VERTEX_POINT('',#69550);
#16194=VERTEX_POINT('',#69552);
#16195=VERTEX_POINT('',#69556);
#16196=VERTEX_POINT('',#69558);
#16197=VERTEX_POINT('',#69560);
#16198=VERTEX_POINT('',#69562);
#16199=VERTEX_POINT('',#69564);
#16200=VERTEX_POINT('',#69566);
#16201=VERTEX_POINT('',#69568);
#16202=VERTEX_POINT('',#69570);
#16203=VERTEX_POINT('',#69572);
#16204=VERTEX_POINT('',#69574);
#16205=VERTEX_POINT('',#69576);
#16206=VERTEX_POINT('',#69578);
#16207=VERTEX_POINT('',#69580);
#16208=VERTEX_POINT('',#69582);
#16209=VERTEX_POINT('',#69584);
#16210=VERTEX_POINT('',#69586);
#16211=VERTEX_POINT('',#69588);
#16212=VERTEX_POINT('',#69590);
#16213=VERTEX_POINT('',#69592);
#16214=VERTEX_POINT('',#69594);
#16215=VERTEX_POINT('',#69596);
#16216=VERTEX_POINT('',#69598);
#16217=VERTEX_POINT('',#69600);
#16218=VERTEX_POINT('',#69602);
#16219=VERTEX_POINT('',#69604);
#16220=VERTEX_POINT('',#69606);
#16221=VERTEX_POINT('',#69608);
#16222=VERTEX_POINT('',#69610);
#16223=VERTEX_POINT('',#69612);
#16224=VERTEX_POINT('',#69614);
#16225=VERTEX_POINT('',#69616);
#16226=VERTEX_POINT('',#69618);
#16227=VERTEX_POINT('',#69620);
#16228=VERTEX_POINT('',#69622);
#16229=VERTEX_POINT('',#69624);
#16230=VERTEX_POINT('',#69626);
#16231=VERTEX_POINT('',#69628);
#16232=VERTEX_POINT('',#69630);
#16233=VERTEX_POINT('',#69632);
#16234=VERTEX_POINT('',#69634);
#16235=VERTEX_POINT('',#69636);
#16236=VERTEX_POINT('',#69638);
#16237=VERTEX_POINT('',#69640);
#16238=VERTEX_POINT('',#69642);
#16239=VERTEX_POINT('',#69645);
#16240=VERTEX_POINT('',#69648);
#16241=VERTEX_POINT('',#69652);
#16242=VERTEX_POINT('',#69659);
#16243=VERTEX_POINT('',#69663);
#16244=VERTEX_POINT('',#69667);
#16245=VERTEX_POINT('',#69669);
#16246=VERTEX_POINT('',#69692);
#16247=VERTEX_POINT('',#69693);
#16248=VERTEX_POINT('',#69695);
#16249=VERTEX_POINT('',#69708);
#16250=VERTEX_POINT('',#69709);
#16251=VERTEX_POINT('',#69724);
#16252=VERTEX_POINT('',#69731);
#16253=VERTEX_POINT('',#69735);
#16254=VERTEX_POINT('',#69742);
#16255=VERTEX_POINT('',#69746);
#16256=VERTEX_POINT('',#69750);
#16257=VERTEX_POINT('',#69752);
#16258=VERTEX_POINT('',#69775);
#16259=VERTEX_POINT('',#69776);
#16260=VERTEX_POINT('',#69778);
#16261=VERTEX_POINT('',#69791);
#16262=VERTEX_POINT('',#69792);
#16263=VERTEX_POINT('',#69807);
#16264=VERTEX_POINT('',#69814);
#16265=VERTEX_POINT('',#69818);
#16266=VERTEX_POINT('',#69825);
#16267=VERTEX_POINT('',#69829);
#16268=VERTEX_POINT('',#69833);
#16269=VERTEX_POINT('',#69835);
#16270=VERTEX_POINT('',#69839);
#16271=VERTEX_POINT('',#69841);
#16272=VERTEX_POINT('',#69864);
#16273=VERTEX_POINT('',#69865);
#16274=VERTEX_POINT('',#69867);
#16275=VERTEX_POINT('',#69880);
#16276=VERTEX_POINT('',#69881);
#16277=VERTEX_POINT('',#69883);
#16278=VERTEX_POINT('',#69885);
#16279=VERTEX_POINT('',#69896);
#16280=VERTEX_POINT('',#69899);
#16281=VERTEX_POINT('',#69933);
#16282=VERTEX_POINT('',#69935);
#16283=VERTEX_POINT('',#69950);
#16284=VERTEX_POINT('',#69954);
#16285=VERTEX_POINT('',#69958);
#16286=VERTEX_POINT('',#69966);
#16287=VERTEX_POINT('',#69977);
#16288=VERTEX_POINT('',#69979);
#16289=VERTEX_POINT('',#70002);
#16290=VERTEX_POINT('',#70003);
#16291=VERTEX_POINT('',#70005);
#16292=VERTEX_POINT('',#70018);
#16293=VERTEX_POINT('',#70019);
#16294=VERTEX_POINT('',#70034);
#16295=VERTEX_POINT('',#70041);
#16296=VERTEX_POINT('',#70045);
#16297=VERTEX_POINT('',#70052);
#16298=VERTEX_POINT('',#70056);
#16299=VERTEX_POINT('',#70060);
#16300=VERTEX_POINT('',#70062);
#16301=VERTEX_POINT('',#70085);
#16302=VERTEX_POINT('',#70086);
#16303=VERTEX_POINT('',#70088);
#16304=VERTEX_POINT('',#70101);
#16305=VERTEX_POINT('',#70102);
#16306=VERTEX_POINT('',#70117);
#16307=VERTEX_POINT('',#70124);
#16308=VERTEX_POINT('',#70128);
#16309=VERTEX_POINT('',#70135);
#16310=VERTEX_POINT('',#70139);
#16311=VERTEX_POINT('',#70143);
#16312=VERTEX_POINT('',#70145);
#16313=VERTEX_POINT('',#70168);
#16314=VERTEX_POINT('',#70169);
#16315=VERTEX_POINT('',#70171);
#16316=VERTEX_POINT('',#70184);
#16317=VERTEX_POINT('',#70185);
#16318=VERTEX_POINT('',#70200);
#16319=VERTEX_POINT('',#70207);
#16320=VERTEX_POINT('',#70211);
#16321=VERTEX_POINT('',#70218);
#16322=VERTEX_POINT('',#70220);
#16323=VERTEX_POINT('',#70224);
#16324=VERTEX_POINT('',#70226);
#16325=VERTEX_POINT('',#70249);
#16326=VERTEX_POINT('',#70250);
#16327=VERTEX_POINT('',#70252);
#16328=VERTEX_POINT('',#70265);
#16329=VERTEX_POINT('',#70266);
#16330=VERTEX_POINT('',#70268);
#16331=VERTEX_POINT('',#70270);
#16332=VERTEX_POINT('',#70281);
#16333=VERTEX_POINT('',#70284);
#16334=VERTEX_POINT('',#70318);
#16335=VERTEX_POINT('',#70320);
#16336=VERTEX_POINT('',#70335);
#16337=VERTEX_POINT('',#70339);
#16338=VERTEX_POINT('',#70343);
#16339=VERTEX_POINT('',#70351);
#16340=VERTEX_POINT('',#70381);
#16341=VERTEX_POINT('',#70383);
#16342=VERTEX_POINT('',#70390);
#16343=VERTEX_POINT('',#70397);
#16344=VERTEX_POINT('',#70402);
#16345=VERTEX_POINT('',#70405);
#16346=VERTEX_POINT('',#70433);
#16347=VERTEX_POINT('',#70435);
#16348=VERTEX_POINT('',#70443);
#16349=VERTEX_POINT('',#70450);
#16350=VERTEX_POINT('',#70453);
#16351=VERTEX_POINT('',#70462);
#16352=VERTEX_POINT('',#70464);
#16353=VERTEX_POINT('',#70487);
#16354=VERTEX_POINT('',#70488);
#16355=VERTEX_POINT('',#70490);
#16356=VERTEX_POINT('',#70503);
#16357=VERTEX_POINT('',#70504);
#16358=VERTEX_POINT('',#70519);
#16359=VERTEX_POINT('',#70526);
#16360=VERTEX_POINT('',#70530);
#16361=VERTEX_POINT('',#70537);
#16362=VERTEX_POINT('',#70541);
#16363=VERTEX_POINT('',#70564);
#16364=VERTEX_POINT('',#70566);
#16365=VERTEX_POINT('',#70574);
#16366=VERTEX_POINT('',#70581);
#16367=VERTEX_POINT('',#70584);
#16368=VERTEX_POINT('',#70593);
#16369=VERTEX_POINT('',#70595);
#16370=VERTEX_POINT('',#70618);
#16371=VERTEX_POINT('',#70619);
#16372=VERTEX_POINT('',#70621);
#16373=VERTEX_POINT('',#70634);
#16374=VERTEX_POINT('',#70635);
#16375=VERTEX_POINT('',#70650);
#16376=VERTEX_POINT('',#70657);
#16377=VERTEX_POINT('',#70661);
#16378=VERTEX_POINT('',#70687);
#16379=VERTEX_POINT('',#70689);
#16380=VERTEX_POINT('',#70697);
#16381=VERTEX_POINT('',#70704);
#16382=VERTEX_POINT('',#70721);
#16383=VERTEX_POINT('',#70729);
#16384=VERTEX_POINT('',#70752);
#16385=VERTEX_POINT('',#70754);
#16386=VERTEX_POINT('',#70761);
#16387=VERTEX_POINT('',#70768);
#16388=VERTEX_POINT('',#70773);
#16389=VERTEX_POINT('',#70776);
#16390=VERTEX_POINT('',#70785);
#16391=VERTEX_POINT('',#70802);
#16392=VERTEX_POINT('',#70810);
#16393=VERTEX_POINT('',#70814);
#16394=VERTEX_POINT('',#70816);
#16395=VERTEX_POINT('',#70839);
#16396=VERTEX_POINT('',#70840);
#16397=VERTEX_POINT('',#70842);
#16398=VERTEX_POINT('',#70855);
#16399=VERTEX_POINT('',#70856);
#16400=VERTEX_POINT('',#70871);
#16401=VERTEX_POINT('',#70878);
#16402=VERTEX_POINT('',#70882);
#16403=VERTEX_POINT('',#70889);
#16404=VERTEX_POINT('',#70891);
#16405=VERTEX_POINT('',#70914);
#16406=VERTEX_POINT('',#70915);
#16407=VERTEX_POINT('',#70917);
#16408=VERTEX_POINT('',#70930);
#16409=VERTEX_POINT('',#70931);
#16410=VERTEX_POINT('',#70946);
#16411=VERTEX_POINT('',#70953);
#16412=VERTEX_POINT('',#70957);
#16413=VERTEX_POINT('',#70964);
#16414=VERTEX_POINT('',#70968);
#16415=VERTEX_POINT('',#70972);
#16416=VERTEX_POINT('',#70974);
#16417=VERTEX_POINT('',#70997);
#16418=VERTEX_POINT('',#70998);
#16419=VERTEX_POINT('',#71000);
#16420=VERTEX_POINT('',#71013);
#16421=VERTEX_POINT('',#71014);
#16422=VERTEX_POINT('',#71029);
#16423=VERTEX_POINT('',#71036);
#16424=VERTEX_POINT('',#71040);
#16425=VERTEX_POINT('',#71047);
#16426=VERTEX_POINT('',#71051);
#16427=VERTEX_POINT('',#71074);
#16428=VERTEX_POINT('',#71076);
#16429=VERTEX_POINT('',#71084);
#16430=VERTEX_POINT('',#71091);
#16431=VERTEX_POINT('',#71094);
#16432=VERTEX_POINT('',#71103);
#16433=VERTEX_POINT('',#71105);
#16434=VERTEX_POINT('',#71128);
#16435=VERTEX_POINT('',#71129);
#16436=VERTEX_POINT('',#71131);
#16437=VERTEX_POINT('',#71144);
#16438=VERTEX_POINT('',#71145);
#16439=VERTEX_POINT('',#71160);
#16440=VERTEX_POINT('',#71167);
#16441=VERTEX_POINT('',#71171);
#16442=VERTEX_POINT('',#71178);
#16443=VERTEX_POINT('',#71182);
#16444=VERTEX_POINT('',#71205);
#16445=VERTEX_POINT('',#71207);
#16446=VERTEX_POINT('',#71215);
#16447=VERTEX_POINT('',#71222);
#16448=VERTEX_POINT('',#71225);
#16449=VERTEX_POINT('',#71234);
#16450=VERTEX_POINT('',#71251);
#16451=VERTEX_POINT('',#71259);
#16452=VERTEX_POINT('',#71263);
#16453=VERTEX_POINT('',#71265);
#16454=VERTEX_POINT('',#71288);
#16455=VERTEX_POINT('',#71289);
#16456=VERTEX_POINT('',#71291);
#16457=VERTEX_POINT('',#71304);
#16458=VERTEX_POINT('',#71305);
#16459=VERTEX_POINT('',#71320);
#16460=VERTEX_POINT('',#71327);
#16461=VERTEX_POINT('',#71331);
#16462=VERTEX_POINT('',#71338);
#16463=VERTEX_POINT('',#71342);
#16464=VERTEX_POINT('',#71346);
#16465=VERTEX_POINT('',#71348);
#16466=VERTEX_POINT('',#71371);
#16467=VERTEX_POINT('',#71372);
#16468=VERTEX_POINT('',#71374);
#16469=VERTEX_POINT('',#71387);
#16470=VERTEX_POINT('',#71388);
#16471=VERTEX_POINT('',#71403);
#16472=VERTEX_POINT('',#71410);
#16473=VERTEX_POINT('',#71414);
#16474=VERTEX_POINT('',#71421);
#16475=VERTEX_POINT('',#71425);
#16476=VERTEX_POINT('',#71429);
#16477=VERTEX_POINT('',#71431);
#16478=VERTEX_POINT('',#71454);
#16479=VERTEX_POINT('',#71455);
#16480=VERTEX_POINT('',#71457);
#16481=VERTEX_POINT('',#71470);
#16482=VERTEX_POINT('',#71471);
#16483=VERTEX_POINT('',#71486);
#16484=VERTEX_POINT('',#71493);
#16485=VERTEX_POINT('',#71497);
#16486=VERTEX_POINT('',#71523);
#16487=VERTEX_POINT('',#71525);
#16488=VERTEX_POINT('',#71533);
#16489=VERTEX_POINT('',#71540);
#16490=VERTEX_POINT('',#71543);
#16491=VERTEX_POINT('',#71571);
#16492=VERTEX_POINT('',#71573);
#16493=VERTEX_POINT('',#71581);
#16494=VERTEX_POINT('',#71588);
#16495=VERTEX_POINT('',#71591);
#16496=VERTEX_POINT('',#71600);
#16497=VERTEX_POINT('',#71602);
#16498=VERTEX_POINT('',#71625);
#16499=VERTEX_POINT('',#71626);
#16500=VERTEX_POINT('',#71628);
#16501=VERTEX_POINT('',#71641);
#16502=VERTEX_POINT('',#71642);
#16503=VERTEX_POINT('',#71657);
#16504=VERTEX_POINT('',#71664);
#16505=VERTEX_POINT('',#71668);
#16506=VERTEX_POINT('',#71675);
#16507=VERTEX_POINT('',#71679);
#16508=VERTEX_POINT('',#71702);
#16509=VERTEX_POINT('',#71704);
#16510=VERTEX_POINT('',#71712);
#16511=VERTEX_POINT('',#71719);
#16512=VERTEX_POINT('',#71722);
#16513=VERTEX_POINT('',#71731);
#16514=VERTEX_POINT('',#71748);
#16515=VERTEX_POINT('',#71756);
#16516=VERTEX_POINT('',#71760);
#16517=VERTEX_POINT('',#71777);
#16518=VERTEX_POINT('',#71785);
#16519=VERTEX_POINT('',#71808);
#16520=VERTEX_POINT('',#71810);
#16521=VERTEX_POINT('',#71817);
#16522=VERTEX_POINT('',#71824);
#16523=VERTEX_POINT('',#71829);
#16524=VERTEX_POINT('',#71832);
#16525=VERTEX_POINT('',#71860);
#16526=VERTEX_POINT('',#71862);
#16527=VERTEX_POINT('',#71870);
#16528=VERTEX_POINT('',#71877);
#16529=VERTEX_POINT('',#71880);
#16530=VERTEX_POINT('',#71889);
#16531=VERTEX_POINT('',#71891);
#16532=VERTEX_POINT('',#71914);
#16533=VERTEX_POINT('',#71915);
#16534=VERTEX_POINT('',#71917);
#16535=VERTEX_POINT('',#71930);
#16536=VERTEX_POINT('',#71931);
#16537=VERTEX_POINT('',#71946);
#16538=VERTEX_POINT('',#71953);
#16539=VERTEX_POINT('',#71957);
#16540=VERTEX_POINT('',#71983);
#16541=VERTEX_POINT('',#71985);
#16542=VERTEX_POINT('',#71993);
#16543=VERTEX_POINT('',#72000);
#16544=VERTEX_POINT('',#72003);
#16545=VERTEX_POINT('',#72012);
#16546=VERTEX_POINT('',#72014);
#16547=VERTEX_POINT('',#72037);
#16548=VERTEX_POINT('',#72038);
#16549=VERTEX_POINT('',#72040);
#16550=VERTEX_POINT('',#72053);
#16551=VERTEX_POINT('',#72054);
#16552=VERTEX_POINT('',#72069);
#16553=VERTEX_POINT('',#72076);
#16554=VERTEX_POINT('',#72080);
#16555=VERTEX_POINT('',#72087);
#16556=VERTEX_POINT('',#72091);
#16557=VERTEX_POINT('',#72114);
#16558=VERTEX_POINT('',#72116);
#16559=VERTEX_POINT('',#72124);
#16560=VERTEX_POINT('',#72131);
#16561=VERTEX_POINT('',#72134);
#16562=VERTEX_POINT('',#72143);
#16563=VERTEX_POINT('',#72160);
#16564=VERTEX_POINT('',#72168);
#16565=VERTEX_POINT('',#72191);
#16566=VERTEX_POINT('',#72193);
#16567=VERTEX_POINT('',#72200);
#16568=VERTEX_POINT('',#72207);
#16569=VERTEX_POINT('',#72212);
#16570=VERTEX_POINT('',#72215);
#16571=VERTEX_POINT('',#72224);
#16572=VERTEX_POINT('',#72241);
#16573=VERTEX_POINT('',#72249);
#16574=VERTEX_POINT('',#72253);
#16575=VERTEX_POINT('',#72255);
#16576=VERTEX_POINT('',#72278);
#16577=VERTEX_POINT('',#72279);
#16578=VERTEX_POINT('',#72281);
#16579=VERTEX_POINT('',#72294);
#16580=VERTEX_POINT('',#72295);
#16581=VERTEX_POINT('',#72310);
#16582=VERTEX_POINT('',#72317);
#16583=VERTEX_POINT('',#72321);
#16584=VERTEX_POINT('',#72328);
#16585=VERTEX_POINT('',#72332);
#16586=VERTEX_POINT('',#72336);
#16587=VERTEX_POINT('',#72338);
#16588=VERTEX_POINT('',#72361);
#16589=VERTEX_POINT('',#72362);
#16590=VERTEX_POINT('',#72364);
#16591=VERTEX_POINT('',#72377);
#16592=VERTEX_POINT('',#72378);
#16593=VERTEX_POINT('',#72393);
#16594=VERTEX_POINT('',#72400);
#16595=VERTEX_POINT('',#72404);
#16596=VERTEX_POINT('',#72411);
#16597=VERTEX_POINT('',#72415);
#16598=VERTEX_POINT('',#72419);
#16599=VERTEX_POINT('',#72421);
#16600=VERTEX_POINT('',#72444);
#16601=VERTEX_POINT('',#72445);
#16602=VERTEX_POINT('',#72447);
#16603=VERTEX_POINT('',#72460);
#16604=VERTEX_POINT('',#72461);
#16605=VERTEX_POINT('',#72476);
#16606=VERTEX_POINT('',#72483);
#16607=VERTEX_POINT('',#72487);
#16608=VERTEX_POINT('',#72494);
#16609=VERTEX_POINT('',#72496);
#16610=VERTEX_POINT('',#72519);
#16611=VERTEX_POINT('',#72520);
#16612=VERTEX_POINT('',#72522);
#16613=VERTEX_POINT('',#72535);
#16614=VERTEX_POINT('',#72536);
#16615=VERTEX_POINT('',#72551);
#16616=VERTEX_POINT('',#72558);
#16617=VERTEX_POINT('',#72562);
#16618=VERTEX_POINT('',#72569);
#16619=VERTEX_POINT('',#72573);
#16620=VERTEX_POINT('',#72596);
#16621=VERTEX_POINT('',#72598);
#16622=VERTEX_POINT('',#72606);
#16623=VERTEX_POINT('',#72613);
#16624=VERTEX_POINT('',#72616);
#16625=VERTEX_POINT('',#72644);
#16626=VERTEX_POINT('',#72646);
#16627=VERTEX_POINT('',#72653);
#16628=VERTEX_POINT('',#72660);
#16629=VERTEX_POINT('',#72665);
#16630=VERTEX_POINT('',#72668);
#16631=VERTEX_POINT('',#72677);
#16632=VERTEX_POINT('',#72679);
#16633=VERTEX_POINT('',#72702);
#16634=VERTEX_POINT('',#72703);
#16635=VERTEX_POINT('',#72705);
#16636=VERTEX_POINT('',#72718);
#16637=VERTEX_POINT('',#72719);
#16638=VERTEX_POINT('',#72734);
#16639=VERTEX_POINT('',#72741);
#16640=VERTEX_POINT('',#72745);
#16641=VERTEX_POINT('',#72752);
#16642=VERTEX_POINT('',#72756);
#16643=VERTEX_POINT('',#72760);
#16644=VERTEX_POINT('',#72762);
#16645=VERTEX_POINT('',#72785);
#16646=VERTEX_POINT('',#72786);
#16647=VERTEX_POINT('',#72788);
#16648=VERTEX_POINT('',#72801);
#16649=VERTEX_POINT('',#72802);
#16650=VERTEX_POINT('',#72817);
#16651=VERTEX_POINT('',#72824);
#16652=VERTEX_POINT('',#72828);
#16653=VERTEX_POINT('',#72854);
#16654=VERTEX_POINT('',#72856);
#16655=VERTEX_POINT('',#72864);
#16656=VERTEX_POINT('',#72871);
#16657=VERTEX_POINT('',#72874);
#16658=VERTEX_POINT('',#72902);
#16659=VERTEX_POINT('',#72904);
#16660=VERTEX_POINT('',#72912);
#16661=VERTEX_POINT('',#72919);
#16662=VERTEX_POINT('',#72922);
#16663=VERTEX_POINT('',#72931);
#16664=VERTEX_POINT('',#72933);
#16665=VERTEX_POINT('',#72956);
#16666=VERTEX_POINT('',#72957);
#16667=VERTEX_POINT('',#72959);
#16668=VERTEX_POINT('',#72972);
#16669=VERTEX_POINT('',#72973);
#16670=VERTEX_POINT('',#72988);
#16671=VERTEX_POINT('',#72995);
#16672=VERTEX_POINT('',#72999);
#16673=VERTEX_POINT('',#73006);
#16674=VERTEX_POINT('',#73010);
#16675=VERTEX_POINT('',#73033);
#16676=VERTEX_POINT('',#73035);
#16677=VERTEX_POINT('',#73043);
#16678=VERTEX_POINT('',#73050);
#16679=VERTEX_POINT('',#73067);
#16680=VERTEX_POINT('',#73075);
#16681=VERTEX_POINT('',#73098);
#16682=VERTEX_POINT('',#73100);
#16683=VERTEX_POINT('',#73108);
#16684=VERTEX_POINT('',#73115);
#16685=VERTEX_POINT('',#73118);
#16686=VERTEX_POINT('',#73127);
#16687=VERTEX_POINT('',#73144);
#16688=VERTEX_POINT('',#73152);
#16689=VERTEX_POINT('',#73156);
#16690=VERTEX_POINT('',#73173);
#16691=VERTEX_POINT('',#73181);
#16692=VERTEX_POINT('',#73204);
#16693=VERTEX_POINT('',#73206);
#16694=VERTEX_POINT('',#73213);
#16695=VERTEX_POINT('',#73220);
#16696=VERTEX_POINT('',#73225);
#16697=VERTEX_POINT('',#73228);
#16698=VERTEX_POINT('',#73256);
#16699=VERTEX_POINT('',#73258);
#16700=VERTEX_POINT('',#73266);
#16701=VERTEX_POINT('',#73273);
#16702=VERTEX_POINT('',#73276);
#16703=VERTEX_POINT('',#73285);
#16704=VERTEX_POINT('',#73287);
#16705=VERTEX_POINT('',#73310);
#16706=VERTEX_POINT('',#73311);
#16707=VERTEX_POINT('',#73313);
#16708=VERTEX_POINT('',#73326);
#16709=VERTEX_POINT('',#73327);
#16710=VERTEX_POINT('',#73342);
#16711=VERTEX_POINT('',#73349);
#16712=VERTEX_POINT('',#73353);
#16713=VERTEX_POINT('',#73360);
#16714=VERTEX_POINT('',#73364);
#16715=VERTEX_POINT('',#73387);
#16716=VERTEX_POINT('',#73389);
#16717=VERTEX_POINT('',#73397);
#16718=VERTEX_POINT('',#73404);
#16719=VERTEX_POINT('',#73421);
#16720=VERTEX_POINT('',#73429);
#16721=VERTEX_POINT('',#73433);
#16722=VERTEX_POINT('',#73435);
#16723=VERTEX_POINT('',#73458);
#16724=VERTEX_POINT('',#73459);
#16725=VERTEX_POINT('',#73461);
#16726=VERTEX_POINT('',#73474);
#16727=VERTEX_POINT('',#73475);
#16728=VERTEX_POINT('',#73490);
#16729=VERTEX_POINT('',#73497);
#16730=VERTEX_POINT('',#73501);
#16731=VERTEX_POINT('',#73508);
#16732=VERTEX_POINT('',#73512);
#16733=VERTEX_POINT('',#73516);
#16734=VERTEX_POINT('',#73518);
#16735=VERTEX_POINT('',#73541);
#16736=VERTEX_POINT('',#73542);
#16737=VERTEX_POINT('',#73544);
#16738=VERTEX_POINT('',#73557);
#16739=VERTEX_POINT('',#73558);
#16740=VERTEX_POINT('',#73573);
#16741=VERTEX_POINT('',#73580);
#16742=VERTEX_POINT('',#73584);
#16743=VERTEX_POINT('',#73591);
#16744=VERTEX_POINT('',#73595);
#16745=VERTEX_POINT('',#73618);
#16746=VERTEX_POINT('',#73620);
#16747=VERTEX_POINT('',#73628);
#16748=VERTEX_POINT('',#73635);
#16749=VERTEX_POINT('',#73638);
#16750=VERTEX_POINT('',#73647);
#16751=VERTEX_POINT('',#73649);
#16752=VERTEX_POINT('',#73672);
#16753=VERTEX_POINT('',#73673);
#16754=VERTEX_POINT('',#73675);
#16755=VERTEX_POINT('',#73688);
#16756=VERTEX_POINT('',#73689);
#16757=VERTEX_POINT('',#73704);
#16758=VERTEX_POINT('',#73711);
#16759=VERTEX_POINT('',#73715);
#16760=VERTEX_POINT('',#73722);
#16761=VERTEX_POINT('',#73724);
#16762=VERTEX_POINT('',#73747);
#16763=VERTEX_POINT('',#73748);
#16764=VERTEX_POINT('',#73750);
#16765=VERTEX_POINT('',#73763);
#16766=VERTEX_POINT('',#73764);
#16767=VERTEX_POINT('',#73779);
#16768=VERTEX_POINT('',#73786);
#16769=VERTEX_POINT('',#73790);
#16770=VERTEX_POINT('',#73797);
#16771=VERTEX_POINT('',#73801);
#16772=VERTEX_POINT('',#73832);
#16773=VERTEX_POINT('',#73834);
#16774=VERTEX_POINT('',#73857);
#16775=VERTEX_POINT('',#73858);
#16776=VERTEX_POINT('',#73860);
#16777=VERTEX_POINT('',#73873);
#16778=VERTEX_POINT('',#73874);
#16779=VERTEX_POINT('',#73889);
#16780=VERTEX_POINT('',#73896);
#16781=VERTEX_POINT('',#73900);
#16782=VERTEX_POINT('',#73926);
#16783=VERTEX_POINT('',#73928);
#16784=VERTEX_POINT('',#73935);
#16785=VERTEX_POINT('',#73942);
#16786=VERTEX_POINT('',#73947);
#16787=VERTEX_POINT('',#73950);
#16788=VERTEX_POINT('',#73978);
#16789=VERTEX_POINT('',#73980);
#16790=VERTEX_POINT('',#73988);
#16791=VERTEX_POINT('',#73995);
#16792=VERTEX_POINT('',#73998);
#16793=VERTEX_POINT('',#74026);
#16794=VERTEX_POINT('',#74028);
#16795=VERTEX_POINT('',#74035);
#16796=VERTEX_POINT('',#74042);
#16797=VERTEX_POINT('',#74047);
#16798=VERTEX_POINT('',#74050);
#16799=VERTEX_POINT('',#74059);
#16800=VERTEX_POINT('',#74076);
#16801=VERTEX_POINT('',#74084);
#16802=VERTEX_POINT('',#74107);
#16803=VERTEX_POINT('',#74109);
#16804=VERTEX_POINT('',#74117);
#16805=VERTEX_POINT('',#74124);
#16806=VERTEX_POINT('',#74127);
#16807=VERTEX_POINT('',#74155);
#16808=VERTEX_POINT('',#74157);
#16809=VERTEX_POINT('',#74165);
#16810=VERTEX_POINT('',#74172);
#16811=VERTEX_POINT('',#74175);
#16812=VERTEX_POINT('',#74184);
#16813=VERTEX_POINT('',#74186);
#16814=VERTEX_POINT('',#74209);
#16815=VERTEX_POINT('',#74210);
#16816=VERTEX_POINT('',#74212);
#16817=VERTEX_POINT('',#74225);
#16818=VERTEX_POINT('',#74226);
#16819=VERTEX_POINT('',#74241);
#16820=VERTEX_POINT('',#74248);
#16821=VERTEX_POINT('',#74252);
#16822=VERTEX_POINT('',#74259);
#16823=VERTEX_POINT('',#74263);
#16824=VERTEX_POINT('',#74286);
#16825=VERTEX_POINT('',#74288);
#16826=VERTEX_POINT('',#74296);
#16827=VERTEX_POINT('',#74303);
#16828=VERTEX_POINT('',#74306);
#16829=VERTEX_POINT('',#74315);
#16830=VERTEX_POINT('',#74332);
#16831=VERTEX_POINT('',#74340);
#16832=VERTEX_POINT('',#74344);
#16833=VERTEX_POINT('',#74361);
#16834=VERTEX_POINT('',#74369);
#16835=VERTEX_POINT('',#74373);
#16836=VERTEX_POINT('',#74375);
#16837=VERTEX_POINT('',#74398);
#16838=VERTEX_POINT('',#74399);
#16839=VERTEX_POINT('',#74401);
#16840=VERTEX_POINT('',#74414);
#16841=VERTEX_POINT('',#74415);
#16842=VERTEX_POINT('',#74430);
#16843=VERTEX_POINT('',#74437);
#16844=VERTEX_POINT('',#74441);
#16845=VERTEX_POINT('',#74448);
#16846=VERTEX_POINT('',#74452);
#16847=VERTEX_POINT('',#74456);
#16848=VERTEX_POINT('',#74458);
#16849=VERTEX_POINT('',#74481);
#16850=VERTEX_POINT('',#74482);
#16851=VERTEX_POINT('',#74484);
#16852=VERTEX_POINT('',#74497);
#16853=VERTEX_POINT('',#74498);
#16854=VERTEX_POINT('',#74513);
#16855=VERTEX_POINT('',#74520);
#16856=VERTEX_POINT('',#74524);
#16857=VERTEX_POINT('',#74531);
#16858=VERTEX_POINT('',#74533);
#16859=VERTEX_POINT('',#74556);
#16860=VERTEX_POINT('',#74557);
#16861=VERTEX_POINT('',#74559);
#16862=VERTEX_POINT('',#74572);
#16863=VERTEX_POINT('',#74573);
#16864=VERTEX_POINT('',#74588);
#16865=VERTEX_POINT('',#74595);
#16866=VERTEX_POINT('',#74599);
#16867=VERTEX_POINT('',#74606);
#16868=VERTEX_POINT('',#74610);
#16869=VERTEX_POINT('',#74614);
#16870=VERTEX_POINT('',#74616);
#16871=VERTEX_POINT('',#74639);
#16872=VERTEX_POINT('',#74640);
#16873=VERTEX_POINT('',#74642);
#16874=VERTEX_POINT('',#74655);
#16875=VERTEX_POINT('',#74656);
#16876=VERTEX_POINT('',#74671);
#16877=VERTEX_POINT('',#74678);
#16878=VERTEX_POINT('',#74682);
#16879=VERTEX_POINT('',#74689);
#16880=VERTEX_POINT('',#74693);
#16881=VERTEX_POINT('',#74697);
#16882=VERTEX_POINT('',#74699);
#16883=VERTEX_POINT('',#74722);
#16884=VERTEX_POINT('',#74723);
#16885=VERTEX_POINT('',#74725);
#16886=VERTEX_POINT('',#74738);
#16887=VERTEX_POINT('',#74739);
#16888=VERTEX_POINT('',#74754);
#16889=VERTEX_POINT('',#74761);
#16890=VERTEX_POINT('',#74765);
#16891=VERTEX_POINT('',#74791);
#16892=VERTEX_POINT('',#74793);
#16893=VERTEX_POINT('',#74800);
#16894=VERTEX_POINT('',#74807);
#16895=VERTEX_POINT('',#74812);
#16896=VERTEX_POINT('',#74815);
#16897=VERTEX_POINT('',#74843);
#16898=VERTEX_POINT('',#74845);
#16899=VERTEX_POINT('',#74853);
#16900=VERTEX_POINT('',#74860);
#16901=VERTEX_POINT('',#74863);
#16902=VERTEX_POINT('',#74891);
#16903=VERTEX_POINT('',#74893);
#16904=VERTEX_POINT('',#74901);
#16905=VERTEX_POINT('',#74908);
#16906=VERTEX_POINT('',#74911);
#16907=VERTEX_POINT('',#74939);
#16908=VERTEX_POINT('',#74941);
#16909=VERTEX_POINT('',#74948);
#16910=VERTEX_POINT('',#74955);
#16911=VERTEX_POINT('',#74960);
#16912=VERTEX_POINT('',#74963);
#16913=VERTEX_POINT('',#74972);
#16914=VERTEX_POINT('',#74973);
#16915=VERTEX_POINT('',#74988);
#16916=VERTEX_POINT('',#74990);
#16917=VERTEX_POINT('',#75007);
#16918=VERTEX_POINT('',#75009);
#16919=VERTEX_POINT('',#75011);
#16920=VERTEX_POINT('',#75013);
#16921=VERTEX_POINT('',#75030);
#16922=VERTEX_POINT('',#75038);
#16923=VERTEX_POINT('',#75040);
#16924=VERTEX_POINT('',#75069);
#16925=VERTEX_POINT('',#75071);
#16926=VERTEX_POINT('',#75079);
#16927=VERTEX_POINT('',#75086);
#16928=VERTEX_POINT('',#75089);
#16929=VERTEX_POINT('',#75098);
#16930=VERTEX_POINT('',#75100);
#16931=VERTEX_POINT('',#75123);
#16932=VERTEX_POINT('',#75124);
#16933=VERTEX_POINT('',#75126);
#16934=VERTEX_POINT('',#75139);
#16935=VERTEX_POINT('',#75140);
#16936=VERTEX_POINT('',#75155);
#16937=VERTEX_POINT('',#75162);
#16938=VERTEX_POINT('',#75166);
#16939=VERTEX_POINT('',#75219);
#16940=VERTEX_POINT('',#75221);
#16941=VERTEX_POINT('',#75228);
#16942=VERTEX_POINT('',#75235);
#16943=VERTEX_POINT('',#75240);
#16944=VERTEX_POINT('',#75243);
#16945=VERTEX_POINT('',#75252);
#16946=VERTEX_POINT('',#75269);
#16947=VERTEX_POINT('',#75277);
#16948=VERTEX_POINT('',#75281);
#16949=VERTEX_POINT('',#75288);
#16950=VERTEX_POINT('',#75292);
#16951=VERTEX_POINT('',#75294);
#16952=VERTEX_POINT('',#75319);
#16953=VERTEX_POINT('',#75324);
#16954=VERTEX_POINT('',#75331);
#16955=VERTEX_POINT('',#75333);
#16956=VERTEX_POINT('',#75335);
#16957=VERTEX_POINT('',#75342);
#16958=VERTEX_POINT('',#75353);
#16959=VERTEX_POINT('',#75357);
#16960=VERTEX_POINT('',#75359);
#16961=VERTEX_POINT('',#75369);
#16962=VERTEX_POINT('',#75386);
#16963=VERTEX_POINT('',#75394);
#16964=VERTEX_POINT('',#75408);
#16965=VERTEX_POINT('',#75412);
#16966=VERTEX_POINT('',#75414);
#16967=VERTEX_POINT('',#75424);
#16968=VERTEX_POINT('',#75437);
#16969=VERTEX_POINT('',#75454);
#16970=VERTEX_POINT('',#75462);
#16971=VERTEX_POINT('',#75470);
#16972=VERTEX_POINT('',#75474);
#16973=VERTEX_POINT('',#75476);
#16974=VERTEX_POINT('',#75494);
#16975=VERTEX_POINT('',#75511);
#16976=VERTEX_POINT('',#75519);
#16977=VERTEX_POINT('',#75542);
#16978=VERTEX_POINT('',#75544);
#16979=VERTEX_POINT('',#75554);
#16980=VERTEX_POINT('',#75576);
#16981=VERTEX_POINT('',#75580);
#16982=VERTEX_POINT('',#75582);
#16983=VERTEX_POINT('',#75592);
#16984=VERTEX_POINT('',#75609);
#16985=VERTEX_POINT('',#75617);
#16986=VERTEX_POINT('',#75623);
#16987=VERTEX_POINT('',#75630);
#16988=VERTEX_POINT('',#75641);
#16989=VERTEX_POINT('',#75645);
#16990=VERTEX_POINT('',#75647);
#16991=VERTEX_POINT('',#75657);
#16992=VERTEX_POINT('',#75670);
#16993=VERTEX_POINT('',#75687);
#16994=VERTEX_POINT('',#75695);
#16995=VERTEX_POINT('',#75703);
#16996=VERTEX_POINT('',#75707);
#16997=VERTEX_POINT('',#75709);
#16998=VERTEX_POINT('',#75727);
#16999=VERTEX_POINT('',#75744);
#17000=VERTEX_POINT('',#75752);
#17001=VERTEX_POINT('',#75775);
#17002=VERTEX_POINT('',#75777);
#17003=VERTEX_POINT('',#75787);
#17004=VERTEX_POINT('',#75801);
#17005=VERTEX_POINT('',#75808);
#17006=VERTEX_POINT('',#75819);
#17007=VERTEX_POINT('',#75823);
#17008=VERTEX_POINT('',#75825);
#17009=VERTEX_POINT('',#75835);
#17010=VERTEX_POINT('',#75852);
#17011=VERTEX_POINT('',#75860);
#17012=VERTEX_POINT('',#75874);
#17013=VERTEX_POINT('',#75878);
#17014=VERTEX_POINT('',#75880);
#17015=VERTEX_POINT('',#75896);
#17016=VERTEX_POINT('',#75913);
#17017=VERTEX_POINT('',#75921);
#17018=VERTEX_POINT('',#75929);
#17019=VERTEX_POINT('',#75933);
#17020=VERTEX_POINT('',#75935);
#17021=VERTEX_POINT('',#75953);
#17022=VERTEX_POINT('',#75970);
#17023=VERTEX_POINT('',#75978);
#17024=VERTEX_POINT('',#76001);
#17025=VERTEX_POINT('',#76003);
#17026=VERTEX_POINT('',#76013);
#17027=VERTEX_POINT('',#76033);
#17028=VERTEX_POINT('',#76050);
#17029=VERTEX_POINT('',#76058);
#17030=VERTEX_POINT('',#76081);
#17031=VERTEX_POINT('',#76083);
#17032=VERTEX_POINT('',#76090);
#17033=VERTEX_POINT('',#76097);
#17034=VERTEX_POINT('',#76104);
#17035=VERTEX_POINT('',#76107);
#17036=VERTEX_POINT('',#76116);
#17037=VERTEX_POINT('',#76118);
#17038=VERTEX_POINT('',#76126);
#17039=VERTEX_POINT('',#76140);
#17040=VERTEX_POINT('',#76144);
#17041=VERTEX_POINT('',#76146);
#17042=VERTEX_POINT('',#76156);
#17043=VERTEX_POINT('',#76165);
#17044=VERTEX_POINT('',#76182);
#17045=VERTEX_POINT('',#76190);
#17046=VERTEX_POINT('',#76202);
#17047=VERTEX_POINT('',#76206);
#17048=VERTEX_POINT('',#76208);
#17049=VERTEX_POINT('',#76218);
#17050=VERTEX_POINT('',#76220);
#17051=VERTEX_POINT('',#76243);
#17052=VERTEX_POINT('',#76244);
#17053=VERTEX_POINT('',#76246);
#17054=VERTEX_POINT('',#76259);
#17055=VERTEX_POINT('',#76260);
#17056=VERTEX_POINT('',#76263);
#17057=VERTEX_POINT('',#76265);
#17058=VERTEX_POINT('',#76286);
#17059=VERTEX_POINT('',#76294);
#17060=VERTEX_POINT('',#76298);
#17061=VERTEX_POINT('',#76305);
#17062=VERTEX_POINT('',#76313);
#17063=VERTEX_POINT('',#76315);
#17064=VERTEX_POINT('',#76319);
#17065=VERTEX_POINT('',#76321);
#17066=VERTEX_POINT('',#76344);
#17067=VERTEX_POINT('',#76345);
#17068=VERTEX_POINT('',#76347);
#17069=VERTEX_POINT('',#76360);
#17070=VERTEX_POINT('',#76361);
#17071=VERTEX_POINT('',#76363);
#17072=VERTEX_POINT('',#76365);
#17073=VERTEX_POINT('',#76376);
#17074=VERTEX_POINT('',#76379);
#17075=VERTEX_POINT('',#76413);
#17076=VERTEX_POINT('',#76415);
#17077=VERTEX_POINT('',#76430);
#17078=VERTEX_POINT('',#76434);
#17079=VERTEX_POINT('',#76438);
#17080=VERTEX_POINT('',#76446);
#17081=VERTEX_POINT('',#76457);
#17082=VERTEX_POINT('',#76487);
#17083=VERTEX_POINT('',#76499);
#17084=VERTEX_POINT('',#76530);
#17085=VERTEX_POINT('',#76531);
#17086=VERTEX_POINT('',#76536);
#17087=VERTEX_POINT('',#76538);
#17088=VERTEX_POINT('',#76542);
#17089=VERTEX_POINT('',#76572);
#17090=VERTEX_POINT('',#76583);
#17091=VERTEX_POINT('',#76613);
#17092=VERTEX_POINT('',#76627);
#17093=VERTEX_POINT('',#76634);
#17094=VERTEX_POINT('',#76640);
#17095=VERTEX_POINT('',#76652);
#17096=VERTEX_POINT('',#76678);
#17097=VERTEX_POINT('',#76683);
#17098=VERTEX_POINT('',#76709);
#17099=VERTEX_POINT('',#76747);
#17100=VERTEX_POINT('',#76773);
#17101=VERTEX_POINT('',#76799);
#17102=VERTEX_POINT('',#76837);
#17103=VERTEX_POINT('',#76863);
#17104=VERTEX_POINT('',#76868);
#17105=VERTEX_POINT('',#76896);
#17106=VERTEX_POINT('',#76932);
#17107=VERTEX_POINT('',#76958);
#17108=VERTEX_POINT('',#76963);
#17109=VERTEX_POINT('',#76989);
#17110=VERTEX_POINT('',#77021);
#17111=VERTEX_POINT('',#77024);
#17112=VERTEX_POINT('',#77026);
#17113=VERTEX_POINT('',#77035);
#19678=EDGE_CURVE('',#15741,#15742,#7194,.T.);
#19679=EDGE_CURVE('',#15742,#15743,#10531,.T.);
#19680=EDGE_CURVE('',#15743,#15744,#111,.F.);
#19681=EDGE_CURVE('',#15744,#15741,#10532,.T.);
#19682=EDGE_CURVE('',#15745,#15746,#7195,.T.);
#19683=EDGE_CURVE('',#15746,#15747,#9674,.T.);
#19684=EDGE_CURVE('',#15747,#15741,#7196,.T.);
#19685=EDGE_CURVE('',#15741,#15745,#9675,.T.);
#19686=EDGE_CURVE('',#15747,#15742,#7197,.T.);
#19687=EDGE_CURVE('',#15748,#15749,#7198,.T.);
#19688=EDGE_CURVE('',#15749,#15750,#10533,.T.);
#19689=EDGE_CURVE('',#15750,#15751,#112,.F.);
#19690=EDGE_CURVE('',#15751,#15748,#10534,.T.);
#19691=EDGE_CURVE('',#15752,#15753,#7199,.T.);
#19692=EDGE_CURVE('',#15753,#15754,#7200,.T.);
#19693=EDGE_CURVE('',#15754,#15755,#7201,.T.);
#19694=EDGE_CURVE('',#15755,#15752,#9676,.T.);
#19695=EDGE_CURVE('',#15755,#15756,#10535,.T.);
#19696=EDGE_CURVE('',#15756,#15745,#7202,.T.);
#19697=EDGE_CURVE('',#15745,#15757,#10536,.T.);
#19698=EDGE_CURVE('',#15757,#15752,#9677,.T.);
#19699=EDGE_CURVE('',#15758,#15753,#7203,.T.);
#19700=EDGE_CURVE('',#15753,#15759,#9678,.T.);
#19701=EDGE_CURVE('',#15759,#15748,#7204,.T.);
#19702=EDGE_CURVE('',#15748,#15758,#9679,.T.);
#19703=EDGE_CURVE('',#15758,#15754,#7205,.T.);
#19704=EDGE_CURVE('',#15759,#15749,#7206,.T.);
#19705=EDGE_CURVE('',#15756,#15746,#7207,.T.);
#19706=EDGE_CURVE('',#15760,#15744,#10537,.T.);
#19707=EDGE_CURVE('',#15761,#15760,#7208,.F.);
#19708=EDGE_CURVE('',#15762,#15761,#10538,.T.);
#19709=EDGE_CURVE('',#15763,#15762,#9680,.T.);
#19710=EDGE_CURVE('',#15757,#15763,#10539,.T.);
#19711=EDGE_CURVE('',#15743,#15764,#10540,.T.);
#19712=EDGE_CURVE('',#15765,#15742,#7209,.T.);
#19713=EDGE_CURVE('',#15766,#15765,#10541,.T.);
#19714=EDGE_CURVE('',#15767,#15766,#10542,.T.);
#19715=EDGE_CURVE('',#15767,#15768,#10543,.T.);
#19716=EDGE_CURVE('',#15769,#15768,#7210,.T.);
#19717=EDGE_CURVE('',#15769,#15770,#10544,.T.);
#19718=EDGE_CURVE('',#15771,#15770,#10545,.T.);
#19719=EDGE_CURVE('',#15771,#15772,#10546,.T.);
#19720=EDGE_CURVE('',#15773,#15772,#7211,.T.);
#19721=EDGE_CURVE('',#15773,#15774,#10547,.T.);
#19722=EDGE_CURVE('',#15775,#15774,#10548,.T.);
#19723=EDGE_CURVE('',#15776,#15775,#10549,.T.);
#19724=EDGE_CURVE('',#15777,#15776,#7212,.T.);
#19725=EDGE_CURVE('',#15778,#15777,#10550,.T.);
#19726=EDGE_CURVE('',#15779,#15778,#10551,.T.);
#19727=EDGE_CURVE('',#15779,#15780,#10552,.T.);
#19728=EDGE_CURVE('',#15781,#15780,#7213,.T.);
#19729=EDGE_CURVE('',#15781,#15782,#10553,.T.);
#19730=EDGE_CURVE('',#15783,#15782,#10554,.T.);
#19731=EDGE_CURVE('',#15783,#15784,#10555,.T.);
#19732=EDGE_CURVE('',#15785,#15784,#7214,.T.);
#19733=EDGE_CURVE('',#15785,#15786,#10556,.T.);
#19734=EDGE_CURVE('',#15787,#15786,#10557,.T.);
#19735=EDGE_CURVE('',#15788,#15787,#10558,.T.);
#19736=EDGE_CURVE('',#15789,#15788,#7215,.T.);
#19737=EDGE_CURVE('',#15790,#15789,#10559,.T.);
#19738=EDGE_CURVE('',#15791,#15790,#10560,.T.);
#19739=EDGE_CURVE('',#15791,#15792,#10561,.T.);
#19740=EDGE_CURVE('',#15793,#15792,#7216,.T.);
#19741=EDGE_CURVE('',#15793,#15794,#10562,.T.);
#19742=EDGE_CURVE('',#15795,#15794,#10563,.T.);
#19743=EDGE_CURVE('',#15795,#15796,#10564,.T.);
#19744=EDGE_CURVE('',#15797,#15796,#7217,.T.);
#19745=EDGE_CURVE('',#15797,#15798,#10565,.T.);
#19746=EDGE_CURVE('',#15799,#15798,#10566,.T.);
#19747=EDGE_CURVE('',#15800,#15799,#10567,.T.);
#19748=EDGE_CURVE('',#15801,#15800,#7218,.T.);
#19749=EDGE_CURVE('',#15802,#15801,#10568,.T.);
#19750=EDGE_CURVE('',#15803,#15802,#10569,.T.);
#19751=EDGE_CURVE('',#15803,#15804,#10570,.T.);
#19752=EDGE_CURVE('',#15805,#15804,#7219,.T.);
#19753=EDGE_CURVE('',#15805,#15806,#10571,.T.);
#19754=EDGE_CURVE('',#15807,#15806,#10572,.T.);
#19755=EDGE_CURVE('',#15807,#15808,#10573,.T.);
#19756=EDGE_CURVE('',#15809,#15808,#7220,.T.);
#19757=EDGE_CURVE('',#15809,#15810,#10574,.T.);
#19758=EDGE_CURVE('',#15811,#15810,#10575,.T.);
#19759=EDGE_CURVE('',#15812,#15811,#10576,.T.);
#19760=EDGE_CURVE('',#15813,#15812,#7221,.T.);
#19761=EDGE_CURVE('',#15814,#15813,#10577,.T.);
#19762=EDGE_CURVE('',#15815,#15814,#10578,.T.);
#19763=EDGE_CURVE('',#15815,#15816,#10579,.T.);
#19764=EDGE_CURVE('',#15817,#15816,#7222,.T.);
#19765=EDGE_CURVE('',#15817,#15818,#10580,.T.);
#19766=EDGE_CURVE('',#15819,#15818,#10581,.T.);
#19767=EDGE_CURVE('',#15819,#15820,#10582,.T.);
#19768=EDGE_CURVE('',#15821,#15820,#7223,.T.);
#19769=EDGE_CURVE('',#15821,#15822,#10583,.T.);
#19770=EDGE_CURVE('',#15823,#15822,#10584,.T.);
#19771=EDGE_CURVE('',#15824,#15823,#10585,.T.);
#19772=EDGE_CURVE('',#15825,#15824,#7224,.T.);
#19773=EDGE_CURVE('',#15826,#15825,#10586,.T.);
#19774=EDGE_CURVE('',#15827,#15826,#10587,.T.);
#19775=EDGE_CURVE('',#15827,#15828,#10588,.T.);
#19776=EDGE_CURVE('',#15829,#15828,#7225,.T.);
#19777=EDGE_CURVE('',#15829,#15830,#10589,.T.);
#19778=EDGE_CURVE('',#15831,#15830,#10590,.T.);
#19779=EDGE_CURVE('',#15831,#15832,#10591,.T.);
#19780=EDGE_CURVE('',#15833,#15832,#7226,.T.);
#19781=EDGE_CURVE('',#15833,#15834,#10592,.T.);
#19782=EDGE_CURVE('',#15835,#15834,#10593,.T.);
#19783=EDGE_CURVE('',#15836,#15835,#10594,.T.);
#19784=EDGE_CURVE('',#15837,#15836,#7227,.T.);
#19785=EDGE_CURVE('',#15838,#15837,#10595,.T.);
#19786=EDGE_CURVE('',#15839,#15838,#10596,.T.);
#19787=EDGE_CURVE('',#15840,#15839,#10597,.T.);
#19788=EDGE_CURVE('',#15841,#15840,#7228,.T.);
#19789=EDGE_CURVE('',#15841,#15842,#10598,.T.);
#19790=EDGE_CURVE('',#15843,#15842,#10599,.T.);
#19791=EDGE_CURVE('',#15843,#15844,#10600,.T.);
#19792=EDGE_CURVE('',#15845,#15844,#7229,.T.);
#19793=EDGE_CURVE('',#15845,#15846,#10601,.T.);
#19794=EDGE_CURVE('',#15847,#15846,#10602,.T.);
#19795=EDGE_CURVE('',#15848,#15847,#10603,.T.);
#19796=EDGE_CURVE('',#15849,#15848,#7230,.T.);
#19797=EDGE_CURVE('',#15850,#15849,#10604,.T.);
#19798=EDGE_CURVE('',#15851,#15850,#10605,.T.);
#19799=EDGE_CURVE('',#15851,#15852,#10606,.T.);
#19800=EDGE_CURVE('',#15853,#15852,#7231,.T.);
#19801=EDGE_CURVE('',#15853,#15854,#10607,.T.);
#19802=EDGE_CURVE('',#15855,#15854,#10608,.T.);
#19803=EDGE_CURVE('',#15855,#15856,#10609,.T.);
#19804=EDGE_CURVE('',#15857,#15856,#7232,.T.);
#19805=EDGE_CURVE('',#15857,#15858,#10610,.T.);
#19806=EDGE_CURVE('',#15859,#15858,#10611,.T.);
#19807=EDGE_CURVE('',#15860,#15859,#10612,.T.);
#19808=EDGE_CURVE('',#15861,#15860,#7233,.T.);
#19809=EDGE_CURVE('',#15862,#15861,#10613,.T.);
#19810=EDGE_CURVE('',#15863,#15862,#10614,.T.);
#19811=EDGE_CURVE('',#15863,#15864,#10615,.T.);
#19812=EDGE_CURVE('',#15865,#15864,#7234,.T.);
#19813=EDGE_CURVE('',#15865,#15866,#10616,.T.);
#19814=EDGE_CURVE('',#15867,#15866,#10617,.T.);
#19815=EDGE_CURVE('',#15867,#15868,#10618,.T.);
#19816=EDGE_CURVE('',#15869,#15868,#7235,.T.);
#19817=EDGE_CURVE('',#15869,#15870,#10619,.T.);
#19818=EDGE_CURVE('',#15871,#15870,#10620,.T.);
#19819=EDGE_CURVE('',#15872,#15871,#10621,.T.);
#19820=EDGE_CURVE('',#15873,#15872,#7236,.T.);
#19821=EDGE_CURVE('',#15874,#15873,#10622,.T.);
#19822=EDGE_CURVE('',#15875,#15874,#10623,.T.);
#19823=EDGE_CURVE('',#15875,#15876,#10624,.T.);
#19824=EDGE_CURVE('',#15877,#15876,#7237,.T.);
#19825=EDGE_CURVE('',#15877,#15878,#10625,.T.);
#19826=EDGE_CURVE('',#15879,#15878,#10626,.T.);
#19827=EDGE_CURVE('',#15880,#15879,#10627,.T.);
#19828=EDGE_CURVE('',#15881,#15880,#7238,.T.);
#19829=EDGE_CURVE('',#15881,#15882,#10628,.T.);
#19830=EDGE_CURVE('',#15883,#15882,#10629,.T.);
#19831=EDGE_CURVE('',#15884,#15883,#10630,.T.);
#19832=EDGE_CURVE('',#15885,#15884,#7239,.T.);
#19833=EDGE_CURVE('',#15886,#15885,#10631,.T.);
#19834=EDGE_CURVE('',#15887,#15886,#10632,.T.);
#19835=EDGE_CURVE('',#15887,#15888,#10633,.T.);
#19836=EDGE_CURVE('',#15889,#15888,#7240,.T.);
#19837=EDGE_CURVE('',#15889,#15890,#10634,.T.);
#19838=EDGE_CURVE('',#15891,#15890,#10635,.T.);
#19839=EDGE_CURVE('',#15891,#15892,#10636,.T.);
#19840=EDGE_CURVE('',#15893,#15892,#7241,.T.);
#19841=EDGE_CURVE('',#15893,#15894,#10637,.T.);
#19842=EDGE_CURVE('',#15895,#15894,#10638,.T.);
#19843=EDGE_CURVE('',#15896,#15895,#10639,.T.);
#19844=EDGE_CURVE('',#15897,#15896,#7242,.T.);
#19845=EDGE_CURVE('',#15898,#15897,#10640,.T.);
#19846=EDGE_CURVE('',#15899,#15898,#10641,.T.);
#19847=EDGE_CURVE('',#15899,#15900,#10642,.T.);
#19848=EDGE_CURVE('',#15901,#15900,#7243,.T.);
#19849=EDGE_CURVE('',#15901,#15902,#10643,.T.);
#19850=EDGE_CURVE('',#15903,#15902,#10644,.T.);
#19851=EDGE_CURVE('',#15904,#15903,#10645,.T.);
#19852=EDGE_CURVE('',#15905,#15904,#7244,.T.);
#19853=EDGE_CURVE('',#15905,#15906,#10646,.T.);
#19854=EDGE_CURVE('',#15907,#15906,#10647,.T.);
#19855=EDGE_CURVE('',#15908,#15907,#10648,.T.);
#19856=EDGE_CURVE('',#15909,#15908,#7245,.T.);
#19857=EDGE_CURVE('',#15910,#15909,#9681,.T.);
#19858=EDGE_CURVE('',#15910,#15911,#10649,.T.);
#19859=EDGE_CURVE('',#15912,#15911,#10650,.T.);
#19860=EDGE_CURVE('',#15913,#15912,#10651,.T.);
#19861=EDGE_CURVE('',#15914,#15913,#7246,.T.);
#19862=EDGE_CURVE('',#15915,#15914,#9682,.T.);
#19863=EDGE_CURVE('',#15915,#15916,#10652,.T.);
#19864=EDGE_CURVE('',#15917,#15916,#10653,.T.);
#19865=EDGE_CURVE('',#15918,#15917,#10654,.T.);
#19866=EDGE_CURVE('',#15919,#15918,#7247,.T.);
#19867=EDGE_CURVE('',#15920,#15919,#9683,.T.);
#19868=EDGE_CURVE('',#15920,#15921,#10655,.T.);
#19869=EDGE_CURVE('',#15922,#15921,#10656,.T.);
#19870=EDGE_CURVE('',#15923,#15922,#10657,.T.);
#19871=EDGE_CURVE('',#15924,#15923,#7248,.T.);
#19872=EDGE_CURVE('',#15925,#15924,#10658,.T.);
#19873=EDGE_CURVE('',#15926,#15925,#10659,.T.);
#19874=EDGE_CURVE('',#15926,#15927,#10660,.T.);
#19875=EDGE_CURVE('',#15928,#15927,#7249,.T.);
#19876=EDGE_CURVE('',#15928,#15929,#10661,.T.);
#19877=EDGE_CURVE('',#15930,#15929,#10662,.T.);
#19878=EDGE_CURVE('',#15930,#15931,#10663,.T.);
#19879=EDGE_CURVE('',#15932,#15931,#7250,.T.);
#19880=EDGE_CURVE('',#15932,#15933,#10664,.T.);
#19881=EDGE_CURVE('',#15934,#15933,#10665,.T.);
#19882=EDGE_CURVE('',#15935,#15934,#10666,.T.);
#19883=EDGE_CURVE('',#15936,#15935,#7251,.T.);
#19884=EDGE_CURVE('',#15937,#15936,#10667,.T.);
#19885=EDGE_CURVE('',#15938,#15937,#10668,.T.);
#19886=EDGE_CURVE('',#15938,#15939,#10669,.T.);
#19887=EDGE_CURVE('',#15940,#15939,#7252,.T.);
#19888=EDGE_CURVE('',#15940,#15941,#10670,.T.);
#19889=EDGE_CURVE('',#15942,#15941,#10671,.T.);
#19890=EDGE_CURVE('',#15942,#15943,#10672,.T.);
#19891=EDGE_CURVE('',#15944,#15943,#7253,.T.);
#19892=EDGE_CURVE('',#15944,#15945,#10673,.T.);
#19893=EDGE_CURVE('',#15946,#15945,#10674,.T.);
#19894=EDGE_CURVE('',#15947,#15946,#10675,.T.);
#19895=EDGE_CURVE('',#15948,#15947,#7254,.T.);
#19896=EDGE_CURVE('',#15949,#15948,#10676,.T.);
#19897=EDGE_CURVE('',#15950,#15949,#10677,.T.);
#19898=EDGE_CURVE('',#15950,#15951,#10678,.T.);
#19899=EDGE_CURVE('',#15952,#15951,#7255,.T.);
#19900=EDGE_CURVE('',#15952,#15953,#10679,.T.);
#19901=EDGE_CURVE('',#15954,#15953,#10680,.T.);
#19902=EDGE_CURVE('',#15954,#15955,#10681,.T.);
#19903=EDGE_CURVE('',#15956,#15955,#7256,.T.);
#19904=EDGE_CURVE('',#15956,#15764,#10682,.T.);
#19905=EDGE_CURVE('',#15957,#15957,#7257,.T.);
#19906=EDGE_CURVE('',#15747,#15958,#7258,.T.);
#19907=EDGE_CURVE('',#15765,#15958,#7259,.T.);
#19908=EDGE_CURVE('',#15959,#15746,#7260,.T.);
#19909=EDGE_CURVE('',#15958,#15959,#9684,.T.);
#19910=EDGE_CURVE('',#15756,#15960,#7261,.T.);
#19911=EDGE_CURVE('',#15960,#15959,#7262,.T.);
#19912=EDGE_CURVE('',#15960,#15754,#10683,.T.);
#19913=EDGE_CURVE('',#15961,#15812,#7263,.T.);
#19914=EDGE_CURVE('',#15811,#15962,#113,.F.);
#19915=EDGE_CURVE('',#15962,#15961,#10684,.T.);
#19916=EDGE_CURVE('',#15963,#15964,#7264,.T.);
#19917=EDGE_CURVE('',#15964,#15965,#9685,.T.);
#19918=EDGE_CURVE('',#15965,#15961,#7265,.T.);
#19919=EDGE_CURVE('',#15961,#15963,#9686,.T.);
#19920=EDGE_CURVE('',#15965,#15812,#7266,.T.);
#19921=EDGE_CURVE('',#15966,#15967,#7267,.T.);
#19922=EDGE_CURVE('',#15967,#15968,#10685,.T.);
#19923=EDGE_CURVE('',#15968,#15969,#114,.F.);
#19924=EDGE_CURVE('',#15969,#15966,#10686,.T.);
#19925=EDGE_CURVE('',#15970,#15971,#7268,.T.);
#19926=EDGE_CURVE('',#15971,#15972,#7269,.T.);
#19927=EDGE_CURVE('',#15972,#15973,#7270,.T.);
#19928=EDGE_CURVE('',#15973,#15970,#9687,.T.);
#19929=EDGE_CURVE('',#15973,#15974,#10687,.T.);
#19930=EDGE_CURVE('',#15974,#15963,#7271,.T.);
#19931=EDGE_CURVE('',#15963,#15975,#10688,.T.);
#19932=EDGE_CURVE('',#15975,#15970,#9688,.T.);
#19933=EDGE_CURVE('',#15976,#15971,#7272,.T.);
#19934=EDGE_CURVE('',#15971,#15977,#9689,.T.);
#19935=EDGE_CURVE('',#15977,#15966,#7273,.T.);
#19936=EDGE_CURVE('',#15966,#15976,#9690,.T.);
#19937=EDGE_CURVE('',#15976,#15972,#7274,.T.);
#19938=EDGE_CURVE('',#15977,#15967,#7275,.T.);
#19939=EDGE_CURVE('',#15974,#15964,#7276,.T.);
#19940=EDGE_CURVE('',#15978,#15962,#10689,.T.);
#19941=EDGE_CURVE('',#15979,#15978,#7277,.F.);
#19942=EDGE_CURVE('',#15980,#15979,#10690,.T.);
#19943=EDGE_CURVE('',#15981,#15980,#9691,.T.);
#19944=EDGE_CURVE('',#15975,#15981,#10691,.T.);
#19945=EDGE_CURVE('',#15965,#15982,#7278,.T.);
#19946=EDGE_CURVE('',#15813,#15982,#7279,.T.);
#19947=EDGE_CURVE('',#15983,#15964,#7280,.T.);
#19948=EDGE_CURVE('',#15982,#15983,#9692,.T.);
#19949=EDGE_CURVE('',#15974,#15984,#7281,.T.);
#19950=EDGE_CURVE('',#15984,#15983,#7282,.T.);
#19951=EDGE_CURVE('',#15984,#15972,#10692,.T.);
#19952=EDGE_CURVE('',#15985,#15860,#7283,.T.);
#19953=EDGE_CURVE('',#15859,#15986,#115,.F.);
#19954=EDGE_CURVE('',#15986,#15985,#10693,.T.);
#19955=EDGE_CURVE('',#15987,#15988,#7284,.T.);
#19956=EDGE_CURVE('',#15988,#15989,#9693,.T.);
#19957=EDGE_CURVE('',#15989,#15985,#7285,.T.);
#19958=EDGE_CURVE('',#15985,#15987,#9694,.T.);
#19959=EDGE_CURVE('',#15989,#15860,#7286,.T.);
#19960=EDGE_CURVE('',#15990,#15991,#7287,.T.);
#19961=EDGE_CURVE('',#15991,#15992,#10694,.T.);
#19962=EDGE_CURVE('',#15992,#15993,#116,.F.);
#19963=EDGE_CURVE('',#15993,#15990,#10695,.T.);
#19964=EDGE_CURVE('',#15994,#15995,#7288,.T.);
#19965=EDGE_CURVE('',#15995,#15996,#7289,.T.);
#19966=EDGE_CURVE('',#15996,#15997,#7290,.T.);
#19967=EDGE_CURVE('',#15997,#15994,#9695,.T.);
#19968=EDGE_CURVE('',#15997,#15998,#10696,.T.);
#19969=EDGE_CURVE('',#15998,#15987,#7291,.T.);
#19970=EDGE_CURVE('',#15987,#15999,#10697,.T.);
#19971=EDGE_CURVE('',#15999,#15994,#9696,.T.);
#19972=EDGE_CURVE('',#16000,#15995,#7292,.T.);
#19973=EDGE_CURVE('',#15995,#16001,#9697,.T.);
#19974=EDGE_CURVE('',#16001,#15990,#7293,.T.);
#19975=EDGE_CURVE('',#15990,#16000,#9698,.T.);
#19976=EDGE_CURVE('',#16000,#15996,#7294,.T.);
#19977=EDGE_CURVE('',#16001,#15991,#7295,.T.);
#19978=EDGE_CURVE('',#15998,#15988,#7296,.T.);
#19979=EDGE_CURVE('',#16002,#15986,#10698,.T.);
#19980=EDGE_CURVE('',#16003,#16002,#7297,.F.);
#19981=EDGE_CURVE('',#16004,#16003,#10699,.T.);
#19982=EDGE_CURVE('',#16005,#16004,#9699,.T.);
#19983=EDGE_CURVE('',#15999,#16005,#10700,.T.);
#19984=EDGE_CURVE('',#15989,#16006,#7298,.T.);
#19985=EDGE_CURVE('',#15861,#16006,#7299,.T.);
#19986=EDGE_CURVE('',#16007,#15988,#7300,.T.);
#19987=EDGE_CURVE('',#16006,#16007,#9700,.T.);
#19988=EDGE_CURVE('',#15998,#16008,#7301,.T.);
#19989=EDGE_CURVE('',#16008,#16007,#7302,.T.);
#19990=EDGE_CURVE('',#16008,#15996,#10701,.T.);
#19991=EDGE_CURVE('',#16009,#16010,#7303,.T.);
#19992=EDGE_CURVE('',#16010,#16011,#10702,.T.);
#19993=EDGE_CURVE('',#16011,#16012,#117,.F.);
#19994=EDGE_CURVE('',#16012,#16009,#10703,.T.);
#19995=EDGE_CURVE('',#16013,#16014,#7304,.T.);
#19996=EDGE_CURVE('',#16014,#16015,#9701,.T.);
#19997=EDGE_CURVE('',#16015,#16009,#7305,.T.);
#19998=EDGE_CURVE('',#16009,#16013,#9702,.T.);
#19999=EDGE_CURVE('',#16015,#16010,#7306,.T.);
#20000=EDGE_CURVE('',#16016,#16017,#7307,.T.);
#20001=EDGE_CURVE('',#16017,#16018,#7308,.T.);
#20002=EDGE_CURVE('',#16018,#16019,#7309,.T.);
#20003=EDGE_CURVE('',#16019,#16016,#9703,.T.);
#20004=EDGE_CURVE('',#16019,#16020,#10704,.T.);
#20005=EDGE_CURVE('',#16020,#16013,#7310,.T.);
#20006=EDGE_CURVE('',#16013,#16021,#10705,.T.);
#20007=EDGE_CURVE('',#16021,#16016,#9704,.T.);
#20008=EDGE_CURVE('',#16020,#16014,#7311,.T.);
#20009=EDGE_CURVE('',#16022,#15880,#7312,.T.);
#20010=EDGE_CURVE('',#15879,#16023,#118,.F.);
#20011=EDGE_CURVE('',#16023,#16022,#10706,.T.);
#20012=EDGE_CURVE('',#16024,#16017,#7313,.T.);
#20013=EDGE_CURVE('',#16017,#16025,#9705,.T.);
#20014=EDGE_CURVE('',#16025,#16022,#7314,.T.);
#20015=EDGE_CURVE('',#16022,#16024,#9706,.T.);
#20016=EDGE_CURVE('',#16025,#15880,#7315,.T.);
#20017=EDGE_CURVE('',#16024,#16018,#7316,.T.);
#20018=EDGE_CURVE('',#16015,#16026,#7317,.T.);
#20019=EDGE_CURVE('',#16027,#16026,#7318,.T.);
#20020=EDGE_CURVE('',#16027,#16010,#7319,.T.);
#20021=EDGE_CURVE('',#16028,#16014,#7320,.T.);
#20022=EDGE_CURVE('',#16026,#16028,#9707,.T.);
#20023=EDGE_CURVE('',#16020,#16029,#7321,.T.);
#20024=EDGE_CURVE('',#16029,#16028,#7322,.T.);
#20025=EDGE_CURVE('',#16029,#16018,#10707,.T.);
#20026=EDGE_CURVE('',#16024,#16030,#10708,.T.);
#20027=EDGE_CURVE('',#16029,#16030,#7323,.T.);
#20028=EDGE_CURVE('',#16031,#16023,#10709,.T.);
#20029=EDGE_CURVE('',#16032,#16031,#10710,.T.);
#20030=EDGE_CURVE('',#16030,#16032,#9708,.T.);
#20031=EDGE_CURVE('',#16033,#16034,#7324,.T.);
#20032=EDGE_CURVE('',#16034,#16035,#10711,.T.);
#20033=EDGE_CURVE('',#16035,#16036,#119,.F.);
#20034=EDGE_CURVE('',#16036,#16033,#10712,.T.);
#20035=EDGE_CURVE('',#16037,#16038,#7325,.T.);
#20036=EDGE_CURVE('',#16038,#16039,#9709,.T.);
#20037=EDGE_CURVE('',#16039,#16033,#7326,.T.);
#20038=EDGE_CURVE('',#16033,#16037,#9710,.T.);
#20039=EDGE_CURVE('',#16039,#16034,#7327,.T.);
#20040=EDGE_CURVE('',#16040,#16041,#7328,.T.);
#20041=EDGE_CURVE('',#16041,#16042,#7329,.T.);
#20042=EDGE_CURVE('',#16042,#16043,#7330,.T.);
#20043=EDGE_CURVE('',#16043,#16040,#9711,.T.);
#20044=EDGE_CURVE('',#16043,#16044,#10713,.T.);
#20045=EDGE_CURVE('',#16044,#16037,#7331,.T.);
#20046=EDGE_CURVE('',#16037,#16045,#10714,.T.);
#20047=EDGE_CURVE('',#16045,#16040,#9712,.T.);
#20048=EDGE_CURVE('',#16044,#16038,#7332,.T.);
#20049=EDGE_CURVE('',#16046,#15840,#7333,.T.);
#20050=EDGE_CURVE('',#15839,#16047,#120,.F.);
#20051=EDGE_CURVE('',#16047,#16046,#10715,.T.);
#20052=EDGE_CURVE('',#16048,#16041,#7334,.T.);
#20053=EDGE_CURVE('',#16041,#16049,#9713,.T.);
#20054=EDGE_CURVE('',#16049,#16046,#7335,.T.);
#20055=EDGE_CURVE('',#16046,#16048,#9714,.T.);
#20056=EDGE_CURVE('',#16049,#15840,#7336,.T.);
#20057=EDGE_CURVE('',#16048,#16042,#7337,.T.);
#20058=EDGE_CURVE('',#16039,#16050,#7338,.T.);
#20059=EDGE_CURVE('',#16051,#16050,#7339,.T.);
#20060=EDGE_CURVE('',#16051,#16034,#7340,.T.);
#20061=EDGE_CURVE('',#16052,#16038,#7341,.T.);
#20062=EDGE_CURVE('',#16050,#16052,#9715,.T.);
#20063=EDGE_CURVE('',#16044,#16053,#7342,.T.);
#20064=EDGE_CURVE('',#16053,#16052,#7343,.T.);
#20065=EDGE_CURVE('',#16053,#16042,#10716,.T.);
#20066=EDGE_CURVE('',#16048,#16054,#10717,.T.);
#20067=EDGE_CURVE('',#16053,#16054,#7344,.T.);
#20068=EDGE_CURVE('',#16055,#16047,#10718,.T.);
#20069=EDGE_CURVE('',#16056,#16055,#10719,.T.);
#20070=EDGE_CURVE('',#16054,#16056,#9716,.T.);
#20071=EDGE_CURVE('',#16057,#16058,#7345,.T.);
#20072=EDGE_CURVE('',#16058,#16059,#10720,.T.);
#20073=EDGE_CURVE('',#16059,#16060,#121,.F.);
#20074=EDGE_CURVE('',#16060,#16057,#10721,.T.);
#20075=EDGE_CURVE('',#16061,#16062,#7346,.T.);
#20076=EDGE_CURVE('',#16062,#16063,#9717,.T.);
#20077=EDGE_CURVE('',#16063,#16057,#7347,.T.);
#20078=EDGE_CURVE('',#16057,#16061,#9718,.T.);
#20079=EDGE_CURVE('',#16063,#16058,#7348,.T.);
#20080=EDGE_CURVE('',#16064,#16065,#9719,.T.);
#20081=EDGE_CURVE('',#16065,#16066,#10722,.T.);
#20082=EDGE_CURVE('',#16066,#16061,#7349,.T.);
#20083=EDGE_CURVE('',#16061,#16064,#10723,.T.);
#20084=EDGE_CURVE('',#16066,#16062,#7350,.T.);
#20085=EDGE_CURVE('',#15762,#15749,#7351,.T.);
#20086=EDGE_CURVE('',#16067,#15761,#10724,.T.);
#20087=EDGE_CURVE('',#16068,#16067,#10725,.T.);
#20088=EDGE_CURVE('',#16069,#16068,#7352,.T.);
#20089=EDGE_CURVE('',#16070,#16069,#10726,.T.);
#20090=EDGE_CURVE('',#16071,#16070,#10727,.T.);
#20091=EDGE_CURVE('',#16072,#16071,#10728,.T.);
#20092=EDGE_CURVE('',#16073,#16072,#7353,.T.);
#20093=EDGE_CURVE('',#16074,#16073,#10729,.T.);
#20094=EDGE_CURVE('',#16075,#16074,#10730,.T.);
#20095=EDGE_CURVE('',#16075,#16076,#10731,.T.);
#20096=EDGE_CURVE('',#16077,#16076,#7354,.T.);
#20097=EDGE_CURVE('',#16077,#16078,#10732,.T.);
#20098=EDGE_CURVE('',#16079,#16078,#10733,.T.);
#20099=EDGE_CURVE('',#16080,#16079,#10734,.T.);
#20100=EDGE_CURVE('',#16081,#16080,#7355,.T.);
#20101=EDGE_CURVE('',#16082,#16081,#10735,.T.);
#20102=EDGE_CURVE('',#16083,#16082,#10736,.T.);
#20103=EDGE_CURVE('',#16084,#16083,#10737,.T.);
#20104=EDGE_CURVE('',#16085,#16084,#7356,.T.);
#20105=EDGE_CURVE('',#16086,#16085,#10738,.T.);
#20106=EDGE_CURVE('',#16087,#16086,#10739,.T.);
#20107=EDGE_CURVE('',#16087,#16088,#10740,.T.);
#20108=EDGE_CURVE('',#16089,#16088,#7357,.T.);
#20109=EDGE_CURVE('',#16089,#16090,#10741,.T.);
#20110=EDGE_CURVE('',#16091,#16090,#10742,.T.);
#20111=EDGE_CURVE('',#16092,#16091,#10743,.T.);
#20112=EDGE_CURVE('',#16093,#16092,#7358,.T.);
#20113=EDGE_CURVE('',#16094,#16093,#10744,.T.);
#20114=EDGE_CURVE('',#16095,#16094,#10745,.T.);
#20115=EDGE_CURVE('',#16096,#16095,#10746,.T.);
#20116=EDGE_CURVE('',#16097,#16096,#7359,.T.);
#20117=EDGE_CURVE('',#16098,#16097,#10747,.T.);
#20118=EDGE_CURVE('',#16099,#16098,#10748,.T.);
#20119=EDGE_CURVE('',#16099,#16100,#10749,.T.);
#20120=EDGE_CURVE('',#16101,#16100,#7360,.T.);
#20121=EDGE_CURVE('',#16101,#16102,#10750,.T.);
#20122=EDGE_CURVE('',#16103,#16102,#10751,.T.);
#20123=EDGE_CURVE('',#16104,#16103,#10752,.T.);
#20124=EDGE_CURVE('',#16105,#16104,#7361,.T.);
#20125=EDGE_CURVE('',#16105,#16106,#10753,.T.);
#20126=EDGE_CURVE('',#16107,#16106,#10754,.T.);
#20127=EDGE_CURVE('',#16108,#16107,#10755,.T.);
#20128=EDGE_CURVE('',#16109,#16108,#7362,.T.);
#20129=EDGE_CURVE('',#16109,#16110,#10756,.T.);
#20130=EDGE_CURVE('',#16111,#16110,#10757,.T.);
#20131=EDGE_CURVE('',#16112,#16111,#10758,.T.);
#20132=EDGE_CURVE('',#16113,#16112,#7363,.T.);
#20133=EDGE_CURVE('',#16113,#16114,#10759,.T.);
#20134=EDGE_CURVE('',#16115,#16114,#10760,.T.);
#20135=EDGE_CURVE('',#16116,#16115,#10761,.T.);
#20136=EDGE_CURVE('',#16117,#16116,#7364,.T.);
#20137=EDGE_CURVE('',#16118,#16117,#10762,.T.);
#20138=EDGE_CURVE('',#16119,#16118,#10763,.T.);
#20139=EDGE_CURVE('',#16119,#16120,#10764,.T.);
#20140=EDGE_CURVE('',#16121,#16120,#7365,.T.);
#20141=EDGE_CURVE('',#16121,#16122,#10765,.T.);
#20142=EDGE_CURVE('',#16123,#16122,#10766,.T.);
#20143=EDGE_CURVE('',#16123,#16124,#10767,.T.);
#20144=EDGE_CURVE('',#16125,#16124,#7366,.T.);
#20145=EDGE_CURVE('',#16125,#16126,#10768,.T.);
#20146=EDGE_CURVE('',#16127,#16126,#10769,.T.);
#20147=EDGE_CURVE('',#16128,#16127,#10770,.T.);
#20148=EDGE_CURVE('',#16129,#16128,#7367,.T.);
#20149=EDGE_CURVE('',#16130,#16129,#10771,.T.);
#20150=EDGE_CURVE('',#16131,#16130,#10772,.T.);
#20151=EDGE_CURVE('',#16132,#16131,#10773,.T.);
#20152=EDGE_CURVE('',#16133,#16132,#7368,.T.);
#20153=EDGE_CURVE('',#16134,#16133,#10774,.T.);
#20154=EDGE_CURVE('',#16135,#16134,#10775,.T.);
#20155=EDGE_CURVE('',#16135,#16136,#10776,.T.);
#20156=EDGE_CURVE('',#16137,#16136,#7369,.T.);
#20157=EDGE_CURVE('',#16137,#16138,#10777,.T.);
#20158=EDGE_CURVE('',#16011,#16138,#10778,.T.);
#20159=EDGE_CURVE('',#16139,#16027,#10779,.T.);
#20160=EDGE_CURVE('',#16140,#16139,#10780,.T.);
#20161=EDGE_CURVE('',#16141,#16140,#10781,.T.);
#20162=EDGE_CURVE('',#16142,#16141,#7370,.T.);
#20163=EDGE_CURVE('',#16143,#16142,#10782,.T.);
#20164=EDGE_CURVE('',#16144,#16143,#10783,.T.);
#20165=EDGE_CURVE('',#16144,#16145,#10784,.T.);
#20166=EDGE_CURVE('',#16146,#16145,#7371,.T.);
#20167=EDGE_CURVE('',#16146,#16147,#10785,.T.);
#20168=EDGE_CURVE('',#16148,#16147,#10786,.T.);
#20169=EDGE_CURVE('',#16149,#16148,#10787,.T.);
#20170=EDGE_CURVE('',#16150,#16149,#7372,.T.);
#20171=EDGE_CURVE('',#16151,#16150,#10788,.T.);
#20172=EDGE_CURVE('',#16152,#16151,#10789,.T.);
#20173=EDGE_CURVE('',#16153,#16152,#10790,.T.);
#20174=EDGE_CURVE('',#16154,#16153,#7373,.T.);
#20175=EDGE_CURVE('',#16155,#16154,#10791,.T.);
#20176=EDGE_CURVE('',#15992,#16155,#10792,.T.);
#20177=EDGE_CURVE('',#16004,#15991,#7374,.T.);
#20178=EDGE_CURVE('',#16156,#16003,#10793,.T.);
#20179=EDGE_CURVE('',#16157,#16156,#10794,.T.);
#20180=EDGE_CURVE('',#16158,#16157,#7375,.T.);
#20181=EDGE_CURVE('',#16159,#16158,#10795,.T.);
#20182=EDGE_CURVE('',#16160,#16159,#10796,.T.);
#20183=EDGE_CURVE('',#16161,#16160,#10797,.T.);
#20184=EDGE_CURVE('',#16162,#16161,#7376,.T.);
#20185=EDGE_CURVE('',#16163,#16162,#10798,.T.);
#20186=EDGE_CURVE('',#16164,#16163,#10799,.T.);
#20187=EDGE_CURVE('',#16164,#16165,#10800,.T.);
#20188=EDGE_CURVE('',#16166,#16165,#7377,.T.);
#20189=EDGE_CURVE('',#16166,#16167,#10801,.T.);
#20190=EDGE_CURVE('',#16168,#16167,#10802,.T.);
#20191=EDGE_CURVE('',#16169,#16168,#10803,.T.);
#20192=EDGE_CURVE('',#16170,#16169,#7378,.T.);
#20193=EDGE_CURVE('',#16171,#16170,#10804,.T.);
#20194=EDGE_CURVE('',#16035,#16171,#10805,.T.);
#20195=EDGE_CURVE('',#16172,#16051,#10806,.T.);
#20196=EDGE_CURVE('',#16173,#16172,#10807,.T.);
#20197=EDGE_CURVE('',#16173,#16174,#10808,.T.);
#20198=EDGE_CURVE('',#16175,#16174,#7379,.T.);
#20199=EDGE_CURVE('',#16175,#16176,#10809,.T.);
#20200=EDGE_CURVE('',#16059,#16176,#10810,.T.);
#20201=EDGE_CURVE('',#16177,#16058,#7380,.T.);
#20202=EDGE_CURVE('',#16178,#16177,#10811,.T.);
#20203=EDGE_CURVE('',#16179,#16178,#10812,.T.);
#20204=EDGE_CURVE('',#16180,#16179,#10813,.T.);
#20205=EDGE_CURVE('',#16181,#16180,#7381,.T.);
#20206=EDGE_CURVE('',#16182,#16181,#10814,.T.);
#20207=EDGE_CURVE('',#16183,#16182,#10815,.T.);
#20208=EDGE_CURVE('',#16183,#16184,#10816,.T.);
#20209=EDGE_CURVE('',#16185,#16184,#7382,.T.);
#20210=EDGE_CURVE('',#16185,#16186,#10817,.T.);
#20211=EDGE_CURVE('',#16187,#16186,#10818,.T.);
#20212=EDGE_CURVE('',#16188,#16187,#10819,.T.);
#20213=EDGE_CURVE('',#16189,#16188,#7383,.T.);
#20214=EDGE_CURVE('',#16190,#16189,#10820,.T.);
#20215=EDGE_CURVE('',#16191,#16190,#10821,.T.);
#20216=EDGE_CURVE('',#16192,#16191,#10822,.T.);
#20217=EDGE_CURVE('',#16193,#16192,#7384,.T.);
#20218=EDGE_CURVE('',#16194,#16193,#10823,.T.);
#20219=EDGE_CURVE('',#15968,#16194,#10824,.T.);
#20220=EDGE_CURVE('',#15980,#15967,#7385,.T.);
#20221=EDGE_CURVE('',#16195,#15979,#10825,.T.);
#20222=EDGE_CURVE('',#16196,#16195,#10826,.T.);
#20223=EDGE_CURVE('',#16197,#16196,#7386,.T.);
#20224=EDGE_CURVE('',#16198,#16197,#10827,.T.);
#20225=EDGE_CURVE('',#16199,#16198,#10828,.T.);
#20226=EDGE_CURVE('',#16200,#16199,#10829,.T.);
#20227=EDGE_CURVE('',#16201,#16200,#7387,.T.);
#20228=EDGE_CURVE('',#16202,#16201,#10830,.T.);
#20229=EDGE_CURVE('',#16203,#16202,#10831,.T.);
#20230=EDGE_CURVE('',#16203,#16204,#10832,.T.);
#20231=EDGE_CURVE('',#16205,#16204,#7388,.T.);
#20232=EDGE_CURVE('',#16205,#16206,#10833,.T.);
#20233=EDGE_CURVE('',#16207,#16206,#10834,.T.);
#20234=EDGE_CURVE('',#16208,#16207,#10835,.T.);
#20235=EDGE_CURVE('',#16209,#16208,#7389,.T.);
#20236=EDGE_CURVE('',#16210,#16209,#10836,.T.);
#20237=EDGE_CURVE('',#16211,#16210,#10837,.T.);
#20238=EDGE_CURVE('',#16212,#16211,#10838,.T.);
#20239=EDGE_CURVE('',#16213,#16212,#7390,.T.);
#20240=EDGE_CURVE('',#16214,#16213,#10839,.T.);
#20241=EDGE_CURVE('',#16215,#16214,#10840,.T.);
#20242=EDGE_CURVE('',#16215,#16216,#10841,.T.);
#20243=EDGE_CURVE('',#16217,#16216,#7391,.T.);
#20244=EDGE_CURVE('',#16217,#16218,#10842,.T.);
#20245=EDGE_CURVE('',#16219,#16218,#10843,.T.);
#20246=EDGE_CURVE('',#16220,#16219,#10844,.T.);
#20247=EDGE_CURVE('',#16221,#16220,#7392,.T.);
#20248=EDGE_CURVE('',#16222,#16221,#10845,.T.);
#20249=EDGE_CURVE('',#16223,#16222,#10846,.T.);
#20250=EDGE_CURVE('',#16224,#16223,#10847,.T.);
#20251=EDGE_CURVE('',#16225,#16224,#7393,.T.);
#20252=EDGE_CURVE('',#16226,#16225,#10848,.T.);
#20253=EDGE_CURVE('',#16227,#16226,#10849,.T.);
#20254=EDGE_CURVE('',#16227,#16228,#10850,.T.);
#20255=EDGE_CURVE('',#16229,#16228,#7394,.T.);
#20256=EDGE_CURVE('',#16229,#16230,#10851,.T.);
#20257=EDGE_CURVE('',#16231,#16230,#10852,.T.);
#20258=EDGE_CURVE('',#16232,#16231,#10853,.T.);
#20259=EDGE_CURVE('',#16233,#16232,#7395,.T.);
#20260=EDGE_CURVE('',#16234,#16233,#10854,.T.);
#20261=EDGE_CURVE('',#16235,#16234,#10855,.T.);
#20262=EDGE_CURVE('',#16236,#16235,#10856,.T.);
#20263=EDGE_CURVE('',#16237,#16236,#7396,.T.);
#20264=EDGE_CURVE('',#16238,#16237,#10857,.T.);
#20265=EDGE_CURVE('',#15750,#16238,#10858,.T.);
#20266=EDGE_CURVE('',#16239,#16239,#7397,.T.);
#20267=EDGE_CURVE('',#16063,#16240,#7398,.T.);
#20268=EDGE_CURVE('',#16177,#16240,#7399,.T.);
#20269=EDGE_CURVE('',#16241,#16062,#7400,.T.);
#20270=EDGE_CURVE('',#16240,#16241,#9720,.T.);
#20271=EDGE_CURVE('',#16066,#16242,#7401,.T.);
#20272=EDGE_CURVE('',#16242,#16241,#7402,.T.);
#20273=EDGE_CURVE('',#16243,#16065,#7403,.T.);
#20274=EDGE_CURVE('',#16242,#16243,#10859,.T.);
#20275=EDGE_CURVE('',#16244,#16200,#7404,.T.);
#20276=EDGE_CURVE('',#16199,#16245,#122,.F.);
#20277=EDGE_CURVE('',#16245,#16244,#10860,.T.);
#20278=EDGE_CURVE('',#16246,#16247,#7405,.T.);
#20279=EDGE_CURVE('',#16247,#16248,#9721,.T.);
#20280=EDGE_CURVE('',#16248,#16244,#7406,.T.);
#20281=EDGE_CURVE('',#16244,#16246,#9722,.T.);
#20282=EDGE_CURVE('',#16248,#16200,#7407,.T.);
#20283=EDGE_CURVE('',#16249,#16250,#9723,.T.);
#20284=EDGE_CURVE('',#16250,#16251,#10861,.T.);
#20285=EDGE_CURVE('',#16251,#16246,#7408,.T.);
#20286=EDGE_CURVE('',#16246,#16249,#10862,.T.);
#20287=EDGE_CURVE('',#16251,#16247,#7409,.T.);
#20288=EDGE_CURVE('',#16248,#16252,#7410,.T.);
#20289=EDGE_CURVE('',#16201,#16252,#7411,.T.);
#20290=EDGE_CURVE('',#16253,#16247,#7412,.T.);
#20291=EDGE_CURVE('',#16252,#16253,#9724,.T.);
#20292=EDGE_CURVE('',#16251,#16254,#7413,.T.);
#20293=EDGE_CURVE('',#16254,#16253,#7414,.T.);
#20294=EDGE_CURVE('',#16255,#16250,#7415,.T.);
#20295=EDGE_CURVE('',#16254,#16255,#10863,.T.);
#20296=EDGE_CURVE('',#16256,#16092,#7416,.T.);
#20297=EDGE_CURVE('',#16091,#16257,#123,.F.);
#20298=EDGE_CURVE('',#16257,#16256,#10864,.T.);
#20299=EDGE_CURVE('',#16258,#16259,#7417,.T.);
#20300=EDGE_CURVE('',#16259,#16260,#9725,.T.);
#20301=EDGE_CURVE('',#16260,#16256,#7418,.T.);
#20302=EDGE_CURVE('',#16256,#16258,#9726,.T.);
#20303=EDGE_CURVE('',#16260,#16092,#7419,.T.);
#20304=EDGE_CURVE('',#16261,#16262,#9727,.T.);
#20305=EDGE_CURVE('',#16262,#16263,#10865,.T.);
#20306=EDGE_CURVE('',#16263,#16258,#7420,.T.);
#20307=EDGE_CURVE('',#16258,#16261,#10866,.T.);
#20308=EDGE_CURVE('',#16263,#16259,#7421,.T.);
#20309=EDGE_CURVE('',#16260,#16264,#7422,.T.);
#20310=EDGE_CURVE('',#16093,#16264,#7423,.T.);
#20311=EDGE_CURVE('',#16265,#16259,#7424,.T.);
#20312=EDGE_CURVE('',#16264,#16265,#9728,.T.);
#20313=EDGE_CURVE('',#16263,#16266,#7425,.T.);
#20314=EDGE_CURVE('',#16266,#16265,#7426,.T.);
#20315=EDGE_CURVE('',#16267,#16262,#7427,.T.);
#20316=EDGE_CURVE('',#16266,#16267,#10867,.T.);
#20317=EDGE_CURVE('',#16268,#16104,#7428,.T.);
#20318=EDGE_CURVE('',#16103,#16269,#124,.F.);
#20319=EDGE_CURVE('',#16269,#16268,#10868,.T.);
#20320=EDGE_CURVE('',#16270,#15918,#7429,.T.);
#20321=EDGE_CURVE('',#15917,#16271,#125,.F.);
#20322=EDGE_CURVE('',#16271,#16270,#10869,.T.);
#20323=EDGE_CURVE('',#16272,#16273,#7430,.T.);
#20324=EDGE_CURVE('',#16273,#16274,#9729,.T.);
#20325=EDGE_CURVE('',#16274,#16270,#7431,.T.);
#20326=EDGE_CURVE('',#16270,#16272,#9730,.T.);
#20327=EDGE_CURVE('',#16274,#15918,#7432,.T.);
#20328=EDGE_CURVE('',#16275,#16276,#7433,.T.);
#20329=EDGE_CURVE('',#16276,#16277,#7434,.T.);
#20330=EDGE_CURVE('',#16277,#16278,#7435,.T.);
#20331=EDGE_CURVE('',#16278,#16275,#9731,.T.);
#20332=EDGE_CURVE('',#16278,#16279,#10870,.T.);
#20333=EDGE_CURVE('',#16279,#16272,#7436,.T.);
#20334=EDGE_CURVE('',#16272,#16280,#10871,.T.);
#20335=EDGE_CURVE('',#16280,#16275,#9732,.T.);
#20336=EDGE_CURVE('',#16279,#16273,#7437,.T.);
#20337=EDGE_CURVE('',#16281,#16276,#7438,.T.);
#20338=EDGE_CURVE('',#16276,#16282,#9733,.T.);
#20339=EDGE_CURVE('',#16282,#16268,#7439,.T.);
#20340=EDGE_CURVE('',#16268,#16281,#9734,.T.);
#20341=EDGE_CURVE('',#16281,#16277,#7440,.T.);
#20342=EDGE_CURVE('',#16282,#16104,#7441,.T.);
#20343=EDGE_CURVE('',#16283,#16277,#10872,.T.);
#20344=EDGE_CURVE('',#16279,#16283,#7442,.T.);
#20345=EDGE_CURVE('',#16281,#16284,#10873,.T.);
#20346=EDGE_CURVE('',#16283,#16284,#7443,.T.);
#20347=EDGE_CURVE('',#16285,#16269,#10874,.T.);
#20348=EDGE_CURVE('',#15921,#16285,#7444,.F.);
#20349=EDGE_CURVE('',#16284,#15920,#9735,.T.);
#20350=EDGE_CURVE('',#16282,#16286,#7445,.T.);
#20351=EDGE_CURVE('',#16286,#16105,#9736,.T.);
#20352=EDGE_CURVE('',#16280,#16286,#10875,.T.);
#20353=EDGE_CURVE('',#16287,#16084,#7446,.T.);
#20354=EDGE_CURVE('',#16083,#16288,#126,.F.);
#20355=EDGE_CURVE('',#16288,#16287,#10876,.T.);
#20356=EDGE_CURVE('',#16289,#16290,#7447,.T.);
#20357=EDGE_CURVE('',#16290,#16291,#9737,.T.);
#20358=EDGE_CURVE('',#16291,#16287,#7448,.T.);
#20359=EDGE_CURVE('',#16287,#16289,#9738,.T.);
#20360=EDGE_CURVE('',#16291,#16084,#7449,.T.);
#20361=EDGE_CURVE('',#16292,#16293,#9739,.T.);
#20362=EDGE_CURVE('',#16293,#16294,#10877,.T.);
#20363=EDGE_CURVE('',#16294,#16289,#7450,.T.);
#20364=EDGE_CURVE('',#16289,#16292,#10878,.T.);
#20365=EDGE_CURVE('',#16294,#16290,#7451,.T.);
#20366=EDGE_CURVE('',#16291,#16295,#7452,.T.);
#20367=EDGE_CURVE('',#16085,#16295,#7453,.T.);
#20368=EDGE_CURVE('',#16296,#16290,#7454,.T.);
#20369=EDGE_CURVE('',#16295,#16296,#9740,.T.);
#20370=EDGE_CURVE('',#16294,#16297,#7455,.T.);
#20371=EDGE_CURVE('',#16297,#16296,#7456,.T.);
#20372=EDGE_CURVE('',#16298,#16293,#7457,.T.);
#20373=EDGE_CURVE('',#16297,#16298,#10879,.T.);
#20374=EDGE_CURVE('',#16299,#16096,#7458,.T.);
#20375=EDGE_CURVE('',#16095,#16300,#127,.F.);
#20376=EDGE_CURVE('',#16300,#16299,#10880,.T.);
#20377=EDGE_CURVE('',#16301,#16302,#7459,.T.);
#20378=EDGE_CURVE('',#16302,#16303,#9741,.T.);
#20379=EDGE_CURVE('',#16303,#16299,#7460,.T.);
#20380=EDGE_CURVE('',#16299,#16301,#9742,.T.);
#20381=EDGE_CURVE('',#16303,#16096,#7461,.T.);
#20382=EDGE_CURVE('',#16304,#16305,#9743,.T.);
#20383=EDGE_CURVE('',#16305,#16306,#10881,.T.);
#20384=EDGE_CURVE('',#16306,#16301,#7462,.T.);
#20385=EDGE_CURVE('',#16301,#16304,#10882,.T.);
#20386=EDGE_CURVE('',#16306,#16302,#7463,.T.);
#20387=EDGE_CURVE('',#16303,#16307,#7464,.T.);
#20388=EDGE_CURVE('',#16097,#16307,#7465,.T.);
#20389=EDGE_CURVE('',#16308,#16302,#7466,.T.);
#20390=EDGE_CURVE('',#16307,#16308,#9744,.T.);
#20391=EDGE_CURVE('',#16306,#16309,#7467,.T.);
#20392=EDGE_CURVE('',#16309,#16308,#7468,.T.);
#20393=EDGE_CURVE('',#16310,#16305,#7469,.T.);
#20394=EDGE_CURVE('',#16309,#16310,#10883,.T.);
#20395=EDGE_CURVE('',#16311,#15923,#7470,.T.);
#20396=EDGE_CURVE('',#15922,#16312,#128,.F.);
#20397=EDGE_CURVE('',#16312,#16311,#10884,.T.);
#20398=EDGE_CURVE('',#16313,#16314,#7471,.T.);
#20399=EDGE_CURVE('',#16314,#16315,#9745,.T.);
#20400=EDGE_CURVE('',#16315,#16311,#7472,.T.);
#20401=EDGE_CURVE('',#16311,#16313,#9746,.T.);
#20402=EDGE_CURVE('',#16315,#15923,#7473,.T.);
#20403=EDGE_CURVE('',#16316,#16317,#9747,.T.);
#20404=EDGE_CURVE('',#16317,#16318,#10885,.T.);
#20405=EDGE_CURVE('',#16318,#16313,#7474,.T.);
#20406=EDGE_CURVE('',#16313,#16316,#10886,.T.);
#20407=EDGE_CURVE('',#16318,#16314,#7475,.T.);
#20408=EDGE_CURVE('',#16315,#16319,#7476,.T.);
#20409=EDGE_CURVE('',#15924,#16319,#7477,.T.);
#20410=EDGE_CURVE('',#16320,#16314,#7478,.T.);
#20411=EDGE_CURVE('',#16319,#16320,#9748,.T.);
#20412=EDGE_CURVE('',#16321,#16108,#7479,.T.);
#20413=EDGE_CURVE('',#16107,#16322,#129,.F.);
#20414=EDGE_CURVE('',#16322,#16321,#10887,.T.);
#20415=EDGE_CURVE('',#16323,#15913,#7480,.T.);
#20416=EDGE_CURVE('',#15912,#16324,#130,.F.);
#20417=EDGE_CURVE('',#16324,#16323,#10888,.T.);
#20418=EDGE_CURVE('',#16325,#16326,#7481,.T.);
#20419=EDGE_CURVE('',#16326,#16327,#9749,.T.);
#20420=EDGE_CURVE('',#16327,#16323,#7482,.T.);
#20421=EDGE_CURVE('',#16323,#16325,#9750,.T.);
#20422=EDGE_CURVE('',#16327,#15913,#7483,.T.);
#20423=EDGE_CURVE('',#16328,#16329,#7484,.T.);
#20424=EDGE_CURVE('',#16329,#16330,#7485,.T.);
#20425=EDGE_CURVE('',#16330,#16331,#7486,.T.);
#20426=EDGE_CURVE('',#16331,#16328,#9751,.T.);
#20427=EDGE_CURVE('',#16331,#16332,#10889,.T.);
#20428=EDGE_CURVE('',#16332,#16325,#7487,.T.);
#20429=EDGE_CURVE('',#16325,#16333,#10890,.T.);
#20430=EDGE_CURVE('',#16333,#16328,#9752,.T.);
#20431=EDGE_CURVE('',#16332,#16326,#7488,.T.);
#20432=EDGE_CURVE('',#16334,#16329,#7489,.T.);
#20433=EDGE_CURVE('',#16329,#16335,#9753,.T.);
#20434=EDGE_CURVE('',#16335,#16321,#7490,.T.);
#20435=EDGE_CURVE('',#16321,#16334,#9754,.T.);
#20436=EDGE_CURVE('',#16334,#16330,#7491,.T.);
#20437=EDGE_CURVE('',#16335,#16108,#7492,.T.);
#20438=EDGE_CURVE('',#16336,#16330,#10891,.T.);
#20439=EDGE_CURVE('',#16332,#16336,#7493,.T.);
#20440=EDGE_CURVE('',#16334,#16337,#10892,.T.);
#20441=EDGE_CURVE('',#16336,#16337,#7494,.T.);
#20442=EDGE_CURVE('',#16338,#16322,#10893,.T.);
#20443=EDGE_CURVE('',#15916,#16338,#7495,.F.);
#20444=EDGE_CURVE('',#16337,#15915,#9755,.T.);
#20445=EDGE_CURVE('',#16335,#16339,#7496,.T.);
#20446=EDGE_CURVE('',#16339,#16109,#9756,.T.);
#20447=EDGE_CURVE('',#16333,#16339,#10894,.T.);
#20448=EDGE_CURVE('',#16340,#16319,#7497,.T.);
#20449=EDGE_CURVE('',#16320,#16341,#7498,.T.);
#20450=EDGE_CURVE('',#16341,#16340,#9757,.T.);
#20451=EDGE_CURVE('',#16318,#16342,#7499,.T.);
#20452=EDGE_CURVE('',#16342,#16320,#7500,.T.);
#20453=EDGE_CURVE('',#16342,#16341,#7501,.T.);
#20454=EDGE_CURVE('',#15924,#16340,#7502,.T.);
#20455=EDGE_CURVE('',#16340,#16343,#10895,.T.);
#20456=EDGE_CURVE('',#16343,#15925,#131,.F.);
#20457=EDGE_CURVE('',#16344,#16312,#10896,.T.);
#20458=EDGE_CURVE('',#16102,#16344,#7503,.F.);
#20459=EDGE_CURVE('',#16345,#16101,#9758,.T.);
#20460=EDGE_CURVE('',#16316,#16345,#10897,.T.);
#20461=EDGE_CURVE('',#16346,#16307,#7504,.T.);
#20462=EDGE_CURVE('',#16308,#16347,#7505,.T.);
#20463=EDGE_CURVE('',#16347,#16346,#9759,.T.);
#20464=EDGE_CURVE('',#16097,#16346,#7506,.T.);
#20465=EDGE_CURVE('',#16346,#16348,#10898,.T.);
#20466=EDGE_CURVE('',#16348,#16098,#132,.F.);
#20467=EDGE_CURVE('',#16309,#16347,#7507,.T.);
#20468=EDGE_CURVE('',#16349,#16300,#10899,.T.);
#20469=EDGE_CURVE('',#15929,#16349,#7508,.F.);
#20470=EDGE_CURVE('',#16350,#15928,#9760,.T.);
#20471=EDGE_CURVE('',#16304,#16350,#10900,.T.);
#20472=EDGE_CURVE('',#16351,#16072,#7509,.T.);
#20473=EDGE_CURVE('',#16071,#16352,#133,.F.);
#20474=EDGE_CURVE('',#16352,#16351,#10901,.T.);
#20475=EDGE_CURVE('',#16353,#16354,#7510,.T.);
#20476=EDGE_CURVE('',#16354,#16355,#9761,.T.);
#20477=EDGE_CURVE('',#16355,#16351,#7511,.T.);
#20478=EDGE_CURVE('',#16351,#16353,#9762,.T.);
#20479=EDGE_CURVE('',#16355,#16072,#7512,.T.);
#20480=EDGE_CURVE('',#16356,#16357,#9763,.T.);
#20481=EDGE_CURVE('',#16357,#16358,#10902,.T.);
#20482=EDGE_CURVE('',#16358,#16353,#7513,.T.);
#20483=EDGE_CURVE('',#16353,#16356,#10903,.T.);
#20484=EDGE_CURVE('',#16358,#16354,#7514,.T.);
#20485=EDGE_CURVE('',#16355,#16359,#7515,.T.);
#20486=EDGE_CURVE('',#16073,#16359,#7516,.T.);
#20487=EDGE_CURVE('',#16360,#16354,#7517,.T.);
#20488=EDGE_CURVE('',#16359,#16360,#9764,.T.);
#20489=EDGE_CURVE('',#16358,#16361,#7518,.T.);
#20490=EDGE_CURVE('',#16361,#16360,#7519,.T.);
#20491=EDGE_CURVE('',#16362,#16357,#7520,.T.);
#20492=EDGE_CURVE('',#16361,#16362,#10904,.T.);
#20493=EDGE_CURVE('',#16363,#16295,#7521,.T.);
#20494=EDGE_CURVE('',#16296,#16364,#7522,.T.);
#20495=EDGE_CURVE('',#16364,#16363,#9765,.T.);
#20496=EDGE_CURVE('',#16085,#16363,#7523,.T.);
#20497=EDGE_CURVE('',#16363,#16365,#10905,.T.);
#20498=EDGE_CURVE('',#16365,#16086,#134,.F.);
#20499=EDGE_CURVE('',#16297,#16364,#7524,.T.);
#20500=EDGE_CURVE('',#16366,#16288,#10906,.T.);
#20501=EDGE_CURVE('',#15941,#16366,#7525,.F.);
#20502=EDGE_CURVE('',#16367,#15940,#9766,.T.);
#20503=EDGE_CURVE('',#16292,#16367,#10907,.T.);
#20504=EDGE_CURVE('',#16368,#15935,#7526,.T.);
#20505=EDGE_CURVE('',#15934,#16369,#135,.F.);
#20506=EDGE_CURVE('',#16369,#16368,#10908,.T.);
#20507=EDGE_CURVE('',#16370,#16371,#7527,.T.);
#20508=EDGE_CURVE('',#16371,#16372,#9767,.T.);
#20509=EDGE_CURVE('',#16372,#16368,#7528,.T.);
#20510=EDGE_CURVE('',#16368,#16370,#9768,.T.);
#20511=EDGE_CURVE('',#16372,#15935,#7529,.T.);
#20512=EDGE_CURVE('',#16373,#16374,#9769,.T.);
#20513=EDGE_CURVE('',#16374,#16375,#10909,.T.);
#20514=EDGE_CURVE('',#16375,#16370,#7530,.T.);
#20515=EDGE_CURVE('',#16370,#16373,#10910,.T.);
#20516=EDGE_CURVE('',#16375,#16371,#7531,.T.);
#20517=EDGE_CURVE('',#16372,#16376,#7532,.T.);
#20518=EDGE_CURVE('',#15936,#16376,#7533,.T.);
#20519=EDGE_CURVE('',#16377,#16371,#7534,.T.);
#20520=EDGE_CURVE('',#16376,#16377,#9770,.T.);
#20521=EDGE_CURVE('',#16378,#16264,#7535,.T.);
#20522=EDGE_CURVE('',#16265,#16379,#7536,.T.);
#20523=EDGE_CURVE('',#16379,#16378,#9771,.T.);
#20524=EDGE_CURVE('',#16093,#16378,#7537,.T.);
#20525=EDGE_CURVE('',#16378,#16380,#10911,.T.);
#20526=EDGE_CURVE('',#16380,#16094,#136,.F.);
#20527=EDGE_CURVE('',#16266,#16379,#7538,.T.);
#20528=EDGE_CURVE('',#16267,#16381,#9772,.T.);
#20529=EDGE_CURVE('',#16381,#16379,#10912,.T.);
#20530=EDGE_CURVE('',#16382,#16381,#10913,.T.);
#20531=EDGE_CURVE('',#15931,#16382,#9773,.T.);
#20532=EDGE_CURVE('',#16383,#15930,#7539,.F.);
#20533=EDGE_CURVE('',#16380,#16383,#10914,.T.);
#20534=EDGE_CURVE('',#16384,#16376,#7540,.T.);
#20535=EDGE_CURVE('',#16377,#16385,#7541,.T.);
#20536=EDGE_CURVE('',#16385,#16384,#9774,.T.);
#20537=EDGE_CURVE('',#16375,#16386,#7542,.T.);
#20538=EDGE_CURVE('',#16386,#16377,#7543,.T.);
#20539=EDGE_CURVE('',#16386,#16385,#7544,.T.);
#20540=EDGE_CURVE('',#15936,#16384,#7545,.T.);
#20541=EDGE_CURVE('',#16384,#16387,#10915,.T.);
#20542=EDGE_CURVE('',#16387,#15937,#137,.F.);
#20543=EDGE_CURVE('',#16388,#16369,#10916,.T.);
#20544=EDGE_CURVE('',#16090,#16388,#7546,.F.);
#20545=EDGE_CURVE('',#16389,#16089,#9775,.T.);
#20546=EDGE_CURVE('',#16373,#16389,#10917,.T.);
#20547=EDGE_CURVE('',#16298,#16390,#9776,.T.);
#20548=EDGE_CURVE('',#16390,#16364,#10918,.T.);
#20549=EDGE_CURVE('',#16391,#16390,#10919,.T.);
#20550=EDGE_CURVE('',#15939,#16391,#9777,.T.);
#20551=EDGE_CURVE('',#16392,#15938,#7547,.F.);
#20552=EDGE_CURVE('',#16365,#16392,#10920,.T.);
#20553=EDGE_CURVE('',#16393,#15947,#7548,.T.);
#20554=EDGE_CURVE('',#15946,#16394,#138,.F.);
#20555=EDGE_CURVE('',#16394,#16393,#10921,.T.);
#20556=EDGE_CURVE('',#16395,#16396,#7549,.T.);
#20557=EDGE_CURVE('',#16396,#16397,#9778,.T.);
#20558=EDGE_CURVE('',#16397,#16393,#7550,.T.);
#20559=EDGE_CURVE('',#16393,#16395,#9779,.T.);
#20560=EDGE_CURVE('',#16397,#15947,#7551,.T.);
#20561=EDGE_CURVE('',#16398,#16399,#9780,.T.);
#20562=EDGE_CURVE('',#16399,#16400,#10922,.T.);
#20563=EDGE_CURVE('',#16400,#16395,#7552,.T.);
#20564=EDGE_CURVE('',#16395,#16398,#10923,.T.);
#20565=EDGE_CURVE('',#16400,#16396,#7553,.T.);
#20566=EDGE_CURVE('',#16397,#16401,#7554,.T.);
#20567=EDGE_CURVE('',#15948,#16401,#7555,.T.);
#20568=EDGE_CURVE('',#16402,#16396,#7556,.T.);
#20569=EDGE_CURVE('',#16401,#16402,#9781,.T.);
#20570=EDGE_CURVE('',#16403,#16236,#7557,.T.);
#20571=EDGE_CURVE('',#16235,#16404,#139,.F.);
#20572=EDGE_CURVE('',#16404,#16403,#10924,.T.);
#20573=EDGE_CURVE('',#16405,#16406,#7558,.T.);
#20574=EDGE_CURVE('',#16406,#16407,#9782,.T.);
#20575=EDGE_CURVE('',#16407,#16403,#7559,.T.);
#20576=EDGE_CURVE('',#16403,#16405,#9783,.T.);
#20577=EDGE_CURVE('',#16407,#16236,#7560,.T.);
#20578=EDGE_CURVE('',#16408,#16409,#9784,.T.);
#20579=EDGE_CURVE('',#16409,#16410,#10925,.T.);
#20580=EDGE_CURVE('',#16410,#16405,#7561,.T.);
#20581=EDGE_CURVE('',#16405,#16408,#10926,.T.);
#20582=EDGE_CURVE('',#16410,#16406,#7562,.T.);
#20583=EDGE_CURVE('',#16407,#16411,#7563,.T.);
#20584=EDGE_CURVE('',#16237,#16411,#7564,.T.);
#20585=EDGE_CURVE('',#16412,#16406,#7565,.T.);
#20586=EDGE_CURVE('',#16411,#16412,#9785,.T.);
#20587=EDGE_CURVE('',#16410,#16413,#7566,.T.);
#20588=EDGE_CURVE('',#16413,#16412,#7567,.T.);
#20589=EDGE_CURVE('',#16414,#16409,#7568,.T.);
#20590=EDGE_CURVE('',#16413,#16414,#10927,.T.);
#20591=EDGE_CURVE('',#16415,#16232,#7569,.T.);
#20592=EDGE_CURVE('',#16231,#16416,#140,.F.);
#20593=EDGE_CURVE('',#16416,#16415,#10928,.T.);
#20594=EDGE_CURVE('',#16417,#16418,#7570,.T.);
#20595=EDGE_CURVE('',#16418,#16419,#9786,.T.);
#20596=EDGE_CURVE('',#16419,#16415,#7571,.T.);
#20597=EDGE_CURVE('',#16415,#16417,#9787,.T.);
#20598=EDGE_CURVE('',#16419,#16232,#7572,.T.);
#20599=EDGE_CURVE('',#16420,#16421,#9788,.T.);
#20600=EDGE_CURVE('',#16421,#16422,#10929,.T.);
#20601=EDGE_CURVE('',#16422,#16417,#7573,.T.);
#20602=EDGE_CURVE('',#16417,#16420,#10930,.T.);
#20603=EDGE_CURVE('',#16422,#16418,#7574,.T.);
#20604=EDGE_CURVE('',#16419,#16423,#7575,.T.);
#20605=EDGE_CURVE('',#16233,#16423,#7576,.T.);
#20606=EDGE_CURVE('',#16424,#16418,#7577,.T.);
#20607=EDGE_CURVE('',#16423,#16424,#9789,.T.);
#20608=EDGE_CURVE('',#16422,#16425,#7578,.T.);
#20609=EDGE_CURVE('',#16425,#16424,#7579,.T.);
#20610=EDGE_CURVE('',#16426,#16421,#7580,.T.);
#20611=EDGE_CURVE('',#16425,#16426,#10931,.T.);
#20612=EDGE_CURVE('',#16427,#16359,#7581,.T.);
#20613=EDGE_CURVE('',#16360,#16428,#7582,.T.);
#20614=EDGE_CURVE('',#16428,#16427,#9790,.T.);
#20615=EDGE_CURVE('',#16073,#16427,#7583,.T.);
#20616=EDGE_CURVE('',#16427,#16429,#10932,.T.);
#20617=EDGE_CURVE('',#16429,#16074,#141,.F.);
#20618=EDGE_CURVE('',#16361,#16428,#7584,.T.);
#20619=EDGE_CURVE('',#16430,#16352,#10933,.T.);
#20620=EDGE_CURVE('',#15953,#16430,#7585,.F.);
#20621=EDGE_CURVE('',#16431,#15952,#9791,.T.);
#20622=EDGE_CURVE('',#16356,#16431,#10934,.T.);
#20623=EDGE_CURVE('',#16432,#16080,#7586,.T.);
#20624=EDGE_CURVE('',#16079,#16433,#142,.F.);
#20625=EDGE_CURVE('',#16433,#16432,#10935,.T.);
#20626=EDGE_CURVE('',#16434,#16435,#7587,.T.);
#20627=EDGE_CURVE('',#16435,#16436,#9792,.T.);
#20628=EDGE_CURVE('',#16436,#16432,#7588,.T.);
#20629=EDGE_CURVE('',#16432,#16434,#9793,.T.);
#20630=EDGE_CURVE('',#16436,#16080,#7589,.T.);
#20631=EDGE_CURVE('',#16437,#16438,#9794,.T.);
#20632=EDGE_CURVE('',#16438,#16439,#10936,.T.);
#20633=EDGE_CURVE('',#16439,#16434,#7590,.T.);
#20634=EDGE_CURVE('',#16434,#16437,#10937,.T.);
#20635=EDGE_CURVE('',#16439,#16435,#7591,.T.);
#20636=EDGE_CURVE('',#16436,#16440,#7592,.T.);
#20637=EDGE_CURVE('',#16081,#16440,#7593,.T.);
#20638=EDGE_CURVE('',#16441,#16435,#7594,.T.);
#20639=EDGE_CURVE('',#16440,#16441,#9795,.T.);
#20640=EDGE_CURVE('',#16439,#16442,#7595,.T.);
#20641=EDGE_CURVE('',#16442,#16441,#7596,.T.);
#20642=EDGE_CURVE('',#16443,#16438,#7597,.T.);
#20643=EDGE_CURVE('',#16442,#16443,#10938,.T.);
#20644=EDGE_CURVE('',#16444,#16440,#7598,.T.);
#20645=EDGE_CURVE('',#16441,#16445,#7599,.T.);
#20646=EDGE_CURVE('',#16445,#16444,#9796,.T.);
#20647=EDGE_CURVE('',#16081,#16444,#7600,.T.);
#20648=EDGE_CURVE('',#16444,#16446,#10939,.T.);
#20649=EDGE_CURVE('',#16446,#16082,#143,.F.);
#20650=EDGE_CURVE('',#16442,#16445,#7601,.T.);
#20651=EDGE_CURVE('',#16447,#16433,#10940,.T.);
#20652=EDGE_CURVE('',#15945,#16447,#7602,.F.);
#20653=EDGE_CURVE('',#16448,#15944,#9797,.T.);
#20654=EDGE_CURVE('',#16437,#16448,#10941,.T.);
#20655=EDGE_CURVE('',#16362,#16449,#9798,.T.);
#20656=EDGE_CURVE('',#16449,#16428,#10942,.T.);
#20657=EDGE_CURVE('',#16450,#16449,#10943,.T.);
#20658=EDGE_CURVE('',#15951,#16450,#9799,.T.);
#20659=EDGE_CURVE('',#16451,#15950,#7603,.F.);
#20660=EDGE_CURVE('',#16429,#16451,#10944,.T.);
#20661=EDGE_CURVE('',#16452,#16220,#7604,.T.);
#20662=EDGE_CURVE('',#16219,#16453,#144,.F.);
#20663=EDGE_CURVE('',#16453,#16452,#10945,.T.);
#20664=EDGE_CURVE('',#16454,#16455,#7605,.T.);
#20665=EDGE_CURVE('',#16455,#16456,#9800,.T.);
#20666=EDGE_CURVE('',#16456,#16452,#7606,.T.);
#20667=EDGE_CURVE('',#16452,#16454,#9801,.T.);
#20668=EDGE_CURVE('',#16456,#16220,#7607,.T.);
#20669=EDGE_CURVE('',#16457,#16458,#9802,.T.);
#20670=EDGE_CURVE('',#16458,#16459,#10946,.T.);
#20671=EDGE_CURVE('',#16459,#16454,#7608,.T.);
#20672=EDGE_CURVE('',#16454,#16457,#10947,.T.);
#20673=EDGE_CURVE('',#16459,#16455,#7609,.T.);
#20674=EDGE_CURVE('',#16456,#16460,#7610,.T.);
#20675=EDGE_CURVE('',#16221,#16460,#7611,.T.);
#20676=EDGE_CURVE('',#16461,#16455,#7612,.T.);
#20677=EDGE_CURVE('',#16460,#16461,#9803,.T.);
#20678=EDGE_CURVE('',#16459,#16462,#7613,.T.);
#20679=EDGE_CURVE('',#16462,#16461,#7614,.T.);
#20680=EDGE_CURVE('',#16463,#16458,#7615,.T.);
#20681=EDGE_CURVE('',#16462,#16463,#10948,.T.);
#20682=EDGE_CURVE('',#16464,#16212,#7616,.T.);
#20683=EDGE_CURVE('',#16211,#16465,#145,.F.);
#20684=EDGE_CURVE('',#16465,#16464,#10949,.T.);
#20685=EDGE_CURVE('',#16466,#16467,#7617,.T.);
#20686=EDGE_CURVE('',#16467,#16468,#9804,.T.);
#20687=EDGE_CURVE('',#16468,#16464,#7618,.T.);
#20688=EDGE_CURVE('',#16464,#16466,#9805,.T.);
#20689=EDGE_CURVE('',#16468,#16212,#7619,.T.);
#20690=EDGE_CURVE('',#16469,#16470,#9806,.T.);
#20691=EDGE_CURVE('',#16470,#16471,#10950,.T.);
#20692=EDGE_CURVE('',#16471,#16466,#7620,.T.);
#20693=EDGE_CURVE('',#16466,#16469,#10951,.T.);
#20694=EDGE_CURVE('',#16471,#16467,#7621,.T.);
#20695=EDGE_CURVE('',#16468,#16472,#7622,.T.);
#20696=EDGE_CURVE('',#16213,#16472,#7623,.T.);
#20697=EDGE_CURVE('',#16473,#16467,#7624,.T.);
#20698=EDGE_CURVE('',#16472,#16473,#9807,.T.);
#20699=EDGE_CURVE('',#16471,#16474,#7625,.T.);
#20700=EDGE_CURVE('',#16474,#16473,#7626,.T.);
#20701=EDGE_CURVE('',#16475,#16470,#7627,.T.);
#20702=EDGE_CURVE('',#16474,#16475,#10952,.T.);
#20703=EDGE_CURVE('',#16476,#15776,#7628,.T.);
#20704=EDGE_CURVE('',#15775,#16477,#146,.F.);
#20705=EDGE_CURVE('',#16477,#16476,#10953,.T.);
#20706=EDGE_CURVE('',#16478,#16479,#7629,.T.);
#20707=EDGE_CURVE('',#16479,#16480,#9808,.T.);
#20708=EDGE_CURVE('',#16480,#16476,#7630,.T.);
#20709=EDGE_CURVE('',#16476,#16478,#9809,.T.);
#20710=EDGE_CURVE('',#16480,#15776,#7631,.T.);
#20711=EDGE_CURVE('',#16481,#16482,#9810,.T.);
#20712=EDGE_CURVE('',#16482,#16483,#10954,.T.);
#20713=EDGE_CURVE('',#16483,#16478,#7632,.T.);
#20714=EDGE_CURVE('',#16478,#16481,#10955,.T.);
#20715=EDGE_CURVE('',#16483,#16479,#7633,.T.);
#20716=EDGE_CURVE('',#16480,#16484,#7634,.T.);
#20717=EDGE_CURVE('',#15777,#16484,#7635,.T.);
#20718=EDGE_CURVE('',#16485,#16479,#7636,.T.);
#20719=EDGE_CURVE('',#16484,#16485,#9811,.T.);
#20720=EDGE_CURVE('',#16486,#16423,#7637,.T.);
#20721=EDGE_CURVE('',#16424,#16487,#7638,.T.);
#20722=EDGE_CURVE('',#16487,#16486,#9812,.T.);
#20723=EDGE_CURVE('',#16233,#16486,#7639,.T.);
#20724=EDGE_CURVE('',#16486,#16488,#10956,.T.);
#20725=EDGE_CURVE('',#16488,#16234,#147,.F.);
#20726=EDGE_CURVE('',#16425,#16487,#7640,.T.);
#20727=EDGE_CURVE('',#16489,#16416,#10957,.T.);
#20728=EDGE_CURVE('',#15774,#16489,#7641,.F.);
#20729=EDGE_CURVE('',#16490,#15773,#9813,.T.);
#20730=EDGE_CURVE('',#16420,#16490,#10958,.T.);
#20731=EDGE_CURVE('',#16491,#16411,#7642,.T.);
#20732=EDGE_CURVE('',#16412,#16492,#7643,.T.);
#20733=EDGE_CURVE('',#16492,#16491,#9814,.T.);
#20734=EDGE_CURVE('',#16237,#16491,#7644,.T.);
#20735=EDGE_CURVE('',#16491,#16493,#10959,.T.);
#20736=EDGE_CURVE('',#16493,#16238,#148,.F.);
#20737=EDGE_CURVE('',#16413,#16492,#7645,.T.);
#20738=EDGE_CURVE('',#16494,#16404,#10960,.T.);
#20739=EDGE_CURVE('',#15770,#16494,#7646,.F.);
#20740=EDGE_CURVE('',#16495,#15769,#9815,.T.);
#20741=EDGE_CURVE('',#16408,#16495,#10961,.T.);
#20742=EDGE_CURVE('',#16496,#16068,#7647,.T.);
#20743=EDGE_CURVE('',#16067,#16497,#149,.F.);
#20744=EDGE_CURVE('',#16497,#16496,#10962,.T.);
#20745=EDGE_CURVE('',#16498,#16499,#7648,.T.);
#20746=EDGE_CURVE('',#16499,#16500,#9816,.T.);
#20747=EDGE_CURVE('',#16500,#16496,#7649,.T.);
#20748=EDGE_CURVE('',#16496,#16498,#9817,.T.);
#20749=EDGE_CURVE('',#16500,#16068,#7650,.T.);
#20750=EDGE_CURVE('',#16501,#16502,#9818,.T.);
#20751=EDGE_CURVE('',#16502,#16503,#10963,.T.);
#20752=EDGE_CURVE('',#16503,#16498,#7651,.T.);
#20753=EDGE_CURVE('',#16498,#16501,#10964,.T.);
#20754=EDGE_CURVE('',#16503,#16499,#7652,.T.);
#20755=EDGE_CURVE('',#16500,#16504,#7653,.T.);
#20756=EDGE_CURVE('',#16069,#16504,#7654,.T.);
#20757=EDGE_CURVE('',#16505,#16499,#7655,.T.);
#20758=EDGE_CURVE('',#16504,#16505,#9819,.T.);
#20759=EDGE_CURVE('',#16503,#16506,#7656,.T.);
#20760=EDGE_CURVE('',#16506,#16505,#7657,.T.);
#20761=EDGE_CURVE('',#16507,#16502,#7658,.T.);
#20762=EDGE_CURVE('',#16506,#16507,#10965,.T.);
#20763=EDGE_CURVE('',#16508,#16504,#7659,.T.);
#20764=EDGE_CURVE('',#16505,#16509,#7660,.T.);
#20765=EDGE_CURVE('',#16509,#16508,#9820,.T.);
#20766=EDGE_CURVE('',#16069,#16508,#7661,.T.);
#20767=EDGE_CURVE('',#16508,#16510,#10966,.T.);
#20768=EDGE_CURVE('',#16510,#16070,#150,.F.);
#20769=EDGE_CURVE('',#16506,#16509,#7662,.T.);
#20770=EDGE_CURVE('',#16511,#16497,#10967,.T.);
#20771=EDGE_CURVE('',#15764,#16511,#7663,.F.);
#20772=EDGE_CURVE('',#16512,#15956,#9821,.T.);
#20773=EDGE_CURVE('',#16501,#16512,#10968,.T.);
#20774=EDGE_CURVE('',#16414,#16513,#9822,.T.);
#20775=EDGE_CURVE('',#16513,#16492,#10969,.T.);
#20776=EDGE_CURVE('',#16514,#16513,#10970,.T.);
#20777=EDGE_CURVE('',#15768,#16514,#9823,.T.);
#20778=EDGE_CURVE('',#16515,#15767,#7664,.F.);
#20779=EDGE_CURVE('',#16493,#16515,#10971,.T.);
#20780=EDGE_CURVE('',#16426,#16516,#9824,.T.);
#20781=EDGE_CURVE('',#16516,#16487,#10972,.T.);
#20782=EDGE_CURVE('',#16517,#16516,#10973,.T.);
#20783=EDGE_CURVE('',#15772,#16517,#9825,.T.);
#20784=EDGE_CURVE('',#16518,#15771,#7665,.F.);
#20785=EDGE_CURVE('',#16488,#16518,#10974,.T.);
#20786=EDGE_CURVE('',#16519,#16484,#7666,.T.);
#20787=EDGE_CURVE('',#16485,#16520,#7667,.T.);
#20788=EDGE_CURVE('',#16520,#16519,#9826,.T.);
#20789=EDGE_CURVE('',#16483,#16521,#7668,.T.);
#20790=EDGE_CURVE('',#16521,#16485,#7669,.T.);
#20791=EDGE_CURVE('',#16521,#16520,#7670,.T.);
#20792=EDGE_CURVE('',#15777,#16519,#7671,.T.);
#20793=EDGE_CURVE('',#16519,#16522,#10975,.T.);
#20794=EDGE_CURVE('',#16522,#15778,#151,.F.);
#20795=EDGE_CURVE('',#16523,#16477,#10976,.T.);
#20796=EDGE_CURVE('',#16230,#16523,#7672,.F.);
#20797=EDGE_CURVE('',#16524,#16229,#9827,.T.);
#20798=EDGE_CURVE('',#16481,#16524,#10977,.T.);
#20799=EDGE_CURVE('',#16525,#16472,#7673,.T.);
#20800=EDGE_CURVE('',#16473,#16526,#7674,.T.);
#20801=EDGE_CURVE('',#16526,#16525,#9828,.T.);
#20802=EDGE_CURVE('',#16213,#16525,#7675,.T.);
#20803=EDGE_CURVE('',#16525,#16527,#10978,.T.);
#20804=EDGE_CURVE('',#16527,#16214,#152,.F.);
#20805=EDGE_CURVE('',#16474,#16526,#7676,.T.);
#20806=EDGE_CURVE('',#16528,#16465,#10979,.T.);
#20807=EDGE_CURVE('',#15794,#16528,#7677,.F.);
#20808=EDGE_CURVE('',#16529,#15793,#9829,.T.);
#20809=EDGE_CURVE('',#16469,#16529,#10980,.T.);
#20810=EDGE_CURVE('',#16530,#15788,#7678,.T.);
#20811=EDGE_CURVE('',#15787,#16531,#153,.F.);
#20812=EDGE_CURVE('',#16531,#16530,#10981,.T.);
#20813=EDGE_CURVE('',#16532,#16533,#7679,.T.);
#20814=EDGE_CURVE('',#16533,#16534,#9830,.T.);
#20815=EDGE_CURVE('',#16534,#16530,#7680,.T.);
#20816=EDGE_CURVE('',#16530,#16532,#9831,.T.);
#20817=EDGE_CURVE('',#16534,#15788,#7681,.T.);
#20818=EDGE_CURVE('',#16535,#16536,#9832,.T.);
#20819=EDGE_CURVE('',#16536,#16537,#10982,.T.);
#20820=EDGE_CURVE('',#16537,#16532,#7682,.T.);
#20821=EDGE_CURVE('',#16532,#16535,#10983,.T.);
#20822=EDGE_CURVE('',#16537,#16533,#7683,.T.);
#20823=EDGE_CURVE('',#16534,#16538,#7684,.T.);
#20824=EDGE_CURVE('',#15789,#16538,#7685,.T.);
#20825=EDGE_CURVE('',#16539,#16533,#7686,.T.);
#20826=EDGE_CURVE('',#16538,#16539,#9833,.T.);
#20827=EDGE_CURVE('',#16540,#16460,#7687,.T.);
#20828=EDGE_CURVE('',#16461,#16541,#7688,.T.);
#20829=EDGE_CURVE('',#16541,#16540,#9834,.T.);
#20830=EDGE_CURVE('',#16221,#16540,#7689,.T.);
#20831=EDGE_CURVE('',#16540,#16542,#10984,.T.);
#20832=EDGE_CURVE('',#16542,#16222,#154,.F.);
#20833=EDGE_CURVE('',#16462,#16541,#7690,.T.);
#20834=EDGE_CURVE('',#16543,#16453,#10985,.T.);
#20835=EDGE_CURVE('',#15786,#16543,#7691,.F.);
#20836=EDGE_CURVE('',#16544,#15785,#9835,.T.);
#20837=EDGE_CURVE('',#16457,#16544,#10986,.T.);
#20838=EDGE_CURVE('',#16545,#16224,#7692,.T.);
#20839=EDGE_CURVE('',#16223,#16546,#155,.F.);
#20840=EDGE_CURVE('',#16546,#16545,#10987,.T.);
#20841=EDGE_CURVE('',#16547,#16548,#7693,.T.);
#20842=EDGE_CURVE('',#16548,#16549,#9836,.T.);
#20843=EDGE_CURVE('',#16549,#16545,#7694,.T.);
#20844=EDGE_CURVE('',#16545,#16547,#9837,.T.);
#20845=EDGE_CURVE('',#16549,#16224,#7695,.T.);
#20846=EDGE_CURVE('',#16550,#16551,#9838,.T.);
#20847=EDGE_CURVE('',#16551,#16552,#10988,.T.);
#20848=EDGE_CURVE('',#16552,#16547,#7696,.T.);
#20849=EDGE_CURVE('',#16547,#16550,#10989,.T.);
#20850=EDGE_CURVE('',#16552,#16548,#7697,.T.);
#20851=EDGE_CURVE('',#16549,#16553,#7698,.T.);
#20852=EDGE_CURVE('',#16225,#16553,#7699,.T.);
#20853=EDGE_CURVE('',#16554,#16548,#7700,.T.);
#20854=EDGE_CURVE('',#16553,#16554,#9839,.T.);
#20855=EDGE_CURVE('',#16552,#16555,#7701,.T.);
#20856=EDGE_CURVE('',#16555,#16554,#7702,.T.);
#20857=EDGE_CURVE('',#16556,#16551,#7703,.T.);
#20858=EDGE_CURVE('',#16555,#16556,#10990,.T.);
#20859=EDGE_CURVE('',#16557,#16553,#7704,.T.);
#20860=EDGE_CURVE('',#16554,#16558,#7705,.T.);
#20861=EDGE_CURVE('',#16558,#16557,#9840,.T.);
#20862=EDGE_CURVE('',#16225,#16557,#7706,.T.);
#20863=EDGE_CURVE('',#16557,#16559,#10991,.T.);
#20864=EDGE_CURVE('',#16559,#16226,#156,.F.);
#20865=EDGE_CURVE('',#16555,#16558,#7707,.T.);
#20866=EDGE_CURVE('',#16560,#16546,#10992,.T.);
#20867=EDGE_CURVE('',#15782,#16560,#7708,.F.);
#20868=EDGE_CURVE('',#16561,#15781,#9841,.T.);
#20869=EDGE_CURVE('',#16550,#16561,#10993,.T.);
#20870=EDGE_CURVE('',#16463,#16562,#9842,.T.);
#20871=EDGE_CURVE('',#16562,#16541,#10994,.T.);
#20872=EDGE_CURVE('',#16563,#16562,#10995,.T.);
#20873=EDGE_CURVE('',#15784,#16563,#9843,.T.);
#20874=EDGE_CURVE('',#16564,#15783,#7709,.F.);
#20875=EDGE_CURVE('',#16542,#16564,#10996,.T.);
#20876=EDGE_CURVE('',#16565,#16538,#7710,.T.);
#20877=EDGE_CURVE('',#16539,#16566,#7711,.T.);
#20878=EDGE_CURVE('',#16566,#16565,#9844,.T.);
#20879=EDGE_CURVE('',#16537,#16567,#7712,.T.);
#20880=EDGE_CURVE('',#16567,#16539,#7713,.T.);
#20881=EDGE_CURVE('',#16567,#16566,#7714,.T.);
#20882=EDGE_CURVE('',#15789,#16565,#7715,.T.);
#20883=EDGE_CURVE('',#16565,#16568,#10997,.T.);
#20884=EDGE_CURVE('',#16568,#15790,#157,.F.);
#20885=EDGE_CURVE('',#16569,#16531,#10998,.T.);
#20886=EDGE_CURVE('',#16218,#16569,#7716,.F.);
#20887=EDGE_CURVE('',#16570,#16217,#9845,.T.);
#20888=EDGE_CURVE('',#16535,#16570,#10999,.T.);
#20889=EDGE_CURVE('',#16475,#16571,#9846,.T.);
#20890=EDGE_CURVE('',#16571,#16526,#11000,.T.);
#20891=EDGE_CURVE('',#16572,#16571,#11001,.T.);
#20892=EDGE_CURVE('',#15792,#16572,#9847,.T.);
#20893=EDGE_CURVE('',#16573,#15791,#7717,.F.);
#20894=EDGE_CURVE('',#16527,#16573,#11002,.T.);
#20895=EDGE_CURVE('',#16574,#16192,#7718,.T.);
#20896=EDGE_CURVE('',#16191,#16575,#158,.F.);
#20897=EDGE_CURVE('',#16575,#16574,#11003,.T.);
#20898=EDGE_CURVE('',#16576,#16577,#7719,.T.);
#20899=EDGE_CURVE('',#16577,#16578,#9848,.T.);
#20900=EDGE_CURVE('',#16578,#16574,#7720,.T.);
#20901=EDGE_CURVE('',#16574,#16576,#9849,.T.);
#20902=EDGE_CURVE('',#16578,#16192,#7721,.T.);
#20903=EDGE_CURVE('',#16579,#16580,#9850,.T.);
#20904=EDGE_CURVE('',#16580,#16581,#11004,.T.);
#20905=EDGE_CURVE('',#16581,#16576,#7722,.T.);
#20906=EDGE_CURVE('',#16576,#16579,#11005,.T.);
#20907=EDGE_CURVE('',#16581,#16577,#7723,.T.);
#20908=EDGE_CURVE('',#16578,#16582,#7724,.T.);
#20909=EDGE_CURVE('',#16193,#16582,#7725,.T.);
#20910=EDGE_CURVE('',#16583,#16577,#7726,.T.);
#20911=EDGE_CURVE('',#16582,#16583,#9851,.T.);
#20912=EDGE_CURVE('',#16581,#16584,#7727,.T.);
#20913=EDGE_CURVE('',#16584,#16583,#7728,.T.);
#20914=EDGE_CURVE('',#16585,#16580,#7729,.T.);
#20915=EDGE_CURVE('',#16584,#16585,#11006,.T.);
#20916=EDGE_CURVE('',#16586,#16188,#7730,.T.);
#20917=EDGE_CURVE('',#16187,#16587,#159,.F.);
#20918=EDGE_CURVE('',#16587,#16586,#11007,.T.);
#20919=EDGE_CURVE('',#16588,#16589,#7731,.T.);
#20920=EDGE_CURVE('',#16589,#16590,#9852,.T.);
#20921=EDGE_CURVE('',#16590,#16586,#7732,.T.);
#20922=EDGE_CURVE('',#16586,#16588,#9853,.T.);
#20923=EDGE_CURVE('',#16590,#16188,#7733,.T.);
#20924=EDGE_CURVE('',#16591,#16592,#9854,.T.);
#20925=EDGE_CURVE('',#16592,#16593,#11008,.T.);
#20926=EDGE_CURVE('',#16593,#16588,#7734,.T.);
#20927=EDGE_CURVE('',#16588,#16591,#11009,.T.);
#20928=EDGE_CURVE('',#16593,#16589,#7735,.T.);
#20929=EDGE_CURVE('',#16590,#16594,#7736,.T.);
#20930=EDGE_CURVE('',#16189,#16594,#7737,.T.);
#20931=EDGE_CURVE('',#16595,#16589,#7738,.T.);
#20932=EDGE_CURVE('',#16594,#16595,#9855,.T.);
#20933=EDGE_CURVE('',#16593,#16596,#7739,.T.);
#20934=EDGE_CURVE('',#16596,#16595,#7740,.T.);
#20935=EDGE_CURVE('',#16597,#16592,#7741,.T.);
#20936=EDGE_CURVE('',#16596,#16597,#11010,.T.);
#20937=EDGE_CURVE('',#16598,#15800,#7742,.T.);
#20938=EDGE_CURVE('',#15799,#16599,#160,.F.);
#20939=EDGE_CURVE('',#16599,#16598,#11011,.T.);
#20940=EDGE_CURVE('',#16600,#16601,#7743,.T.);
#20941=EDGE_CURVE('',#16601,#16602,#9856,.T.);
#20942=EDGE_CURVE('',#16602,#16598,#7744,.T.);
#20943=EDGE_CURVE('',#16598,#16600,#9857,.T.);
#20944=EDGE_CURVE('',#16602,#15800,#7745,.T.);
#20945=EDGE_CURVE('',#16603,#16604,#9858,.T.);
#20946=EDGE_CURVE('',#16604,#16605,#11012,.T.);
#20947=EDGE_CURVE('',#16605,#16600,#7746,.T.);
#20948=EDGE_CURVE('',#16600,#16603,#11013,.T.);
#20949=EDGE_CURVE('',#16605,#16601,#7747,.T.);
#20950=EDGE_CURVE('',#16602,#16606,#7748,.T.);
#20951=EDGE_CURVE('',#15801,#16606,#7749,.T.);
#20952=EDGE_CURVE('',#16607,#16601,#7750,.T.);
#20953=EDGE_CURVE('',#16606,#16607,#9859,.T.);
#20954=EDGE_CURVE('',#16608,#16208,#7751,.T.);
#20955=EDGE_CURVE('',#16207,#16609,#161,.F.);
#20956=EDGE_CURVE('',#16609,#16608,#11014,.T.);
#20957=EDGE_CURVE('',#16610,#16611,#7752,.T.);
#20958=EDGE_CURVE('',#16611,#16612,#9860,.T.);
#20959=EDGE_CURVE('',#16612,#16608,#7753,.T.);
#20960=EDGE_CURVE('',#16608,#16610,#9861,.T.);
#20961=EDGE_CURVE('',#16612,#16208,#7754,.T.);
#20962=EDGE_CURVE('',#16613,#16614,#9862,.T.);
#20963=EDGE_CURVE('',#16614,#16615,#11015,.T.);
#20964=EDGE_CURVE('',#16615,#16610,#7755,.T.);
#20965=EDGE_CURVE('',#16610,#16613,#11016,.T.);
#20966=EDGE_CURVE('',#16615,#16611,#7756,.T.);
#20967=EDGE_CURVE('',#16612,#16616,#7757,.T.);
#20968=EDGE_CURVE('',#16209,#16616,#7758,.T.);
#20969=EDGE_CURVE('',#16617,#16611,#7759,.T.);
#20970=EDGE_CURVE('',#16616,#16617,#9863,.T.);
#20971=EDGE_CURVE('',#16615,#16618,#7760,.T.);
#20972=EDGE_CURVE('',#16618,#16617,#7761,.T.);
#20973=EDGE_CURVE('',#16619,#16614,#7762,.T.);
#20974=EDGE_CURVE('',#16618,#16619,#11017,.T.);
#20975=EDGE_CURVE('',#16620,#16616,#7763,.T.);
#20976=EDGE_CURVE('',#16617,#16621,#7764,.T.);
#20977=EDGE_CURVE('',#16621,#16620,#9864,.T.);
#20978=EDGE_CURVE('',#16209,#16620,#7765,.T.);
#20979=EDGE_CURVE('',#16620,#16622,#11018,.T.);
#20980=EDGE_CURVE('',#16622,#16210,#162,.F.);
#20981=EDGE_CURVE('',#16618,#16621,#7766,.T.);
#20982=EDGE_CURVE('',#16623,#16609,#11019,.T.);
#20983=EDGE_CURVE('',#15798,#16623,#7767,.F.);
#20984=EDGE_CURVE('',#16624,#15797,#9865,.T.);
#20985=EDGE_CURVE('',#16613,#16624,#11020,.T.);
#20986=EDGE_CURVE('',#16625,#16606,#7768,.T.);
#20987=EDGE_CURVE('',#16607,#16626,#7769,.T.);
#20988=EDGE_CURVE('',#16626,#16625,#9866,.T.);
#20989=EDGE_CURVE('',#16605,#16627,#7770,.T.);
#20990=EDGE_CURVE('',#16627,#16607,#7771,.T.);
#20991=EDGE_CURVE('',#16627,#16626,#7772,.T.);
#20992=EDGE_CURVE('',#15801,#16625,#7773,.T.);
#20993=EDGE_CURVE('',#16625,#16628,#11021,.T.);
#20994=EDGE_CURVE('',#16628,#15802,#163,.F.);
#20995=EDGE_CURVE('',#16629,#16599,#11022,.T.);
#20996=EDGE_CURVE('',#16206,#16629,#7774,.F.);
#20997=EDGE_CURVE('',#16630,#16205,#9867,.T.);
#20998=EDGE_CURVE('',#16603,#16630,#11023,.T.);
#20999=EDGE_CURVE('',#16631,#16180,#7775,.T.);
#21000=EDGE_CURVE('',#16179,#16632,#164,.F.);
#21001=EDGE_CURVE('',#16632,#16631,#11024,.T.);
#21002=EDGE_CURVE('',#16633,#16634,#7776,.T.);
#21003=EDGE_CURVE('',#16634,#16635,#9868,.T.);
#21004=EDGE_CURVE('',#16635,#16631,#7777,.T.);
#21005=EDGE_CURVE('',#16631,#16633,#9869,.T.);
#21006=EDGE_CURVE('',#16635,#16180,#7778,.T.);
#21007=EDGE_CURVE('',#16636,#16637,#9870,.T.);
#21008=EDGE_CURVE('',#16637,#16638,#11025,.T.);
#21009=EDGE_CURVE('',#16638,#16633,#7779,.T.);
#21010=EDGE_CURVE('',#16633,#16636,#11026,.T.);
#21011=EDGE_CURVE('',#16638,#16634,#7780,.T.);
#21012=EDGE_CURVE('',#16635,#16639,#7781,.T.);
#21013=EDGE_CURVE('',#16181,#16639,#7782,.T.);
#21014=EDGE_CURVE('',#16640,#16634,#7783,.T.);
#21015=EDGE_CURVE('',#16639,#16640,#9871,.T.);
#21016=EDGE_CURVE('',#16638,#16641,#7784,.T.);
#21017=EDGE_CURVE('',#16641,#16640,#7785,.T.);
#21018=EDGE_CURVE('',#16642,#16637,#7786,.T.);
#21019=EDGE_CURVE('',#16641,#16642,#11027,.T.);
#21020=EDGE_CURVE('',#16643,#15824,#7787,.T.);
#21021=EDGE_CURVE('',#15823,#16644,#165,.F.);
#21022=EDGE_CURVE('',#16644,#16643,#11028,.T.);
#21023=EDGE_CURVE('',#16645,#16646,#7788,.T.);
#21024=EDGE_CURVE('',#16646,#16647,#9872,.T.);
#21025=EDGE_CURVE('',#16647,#16643,#7789,.T.);
#21026=EDGE_CURVE('',#16643,#16645,#9873,.T.);
#21027=EDGE_CURVE('',#16647,#15824,#7790,.T.);
#21028=EDGE_CURVE('',#16648,#16649,#9874,.T.);
#21029=EDGE_CURVE('',#16649,#16650,#11029,.T.);
#21030=EDGE_CURVE('',#16650,#16645,#7791,.T.);
#21031=EDGE_CURVE('',#16645,#16648,#11030,.T.);
#21032=EDGE_CURVE('',#16650,#16646,#7792,.T.);
#21033=EDGE_CURVE('',#16647,#16651,#7793,.T.);
#21034=EDGE_CURVE('',#15825,#16651,#7794,.T.);
#21035=EDGE_CURVE('',#16652,#16646,#7795,.T.);
#21036=EDGE_CURVE('',#16651,#16652,#9875,.T.);
#21037=EDGE_CURVE('',#16653,#16594,#7796,.T.);
#21038=EDGE_CURVE('',#16595,#16654,#7797,.T.);
#21039=EDGE_CURVE('',#16654,#16653,#9876,.T.);
#21040=EDGE_CURVE('',#16189,#16653,#7798,.T.);
#21041=EDGE_CURVE('',#16653,#16655,#11031,.T.);
#21042=EDGE_CURVE('',#16655,#16190,#166,.F.);
#21043=EDGE_CURVE('',#16596,#16654,#7799,.T.);
#21044=EDGE_CURVE('',#16656,#16587,#11032,.T.);
#21045=EDGE_CURVE('',#15822,#16656,#7800,.F.);
#21046=EDGE_CURVE('',#16657,#15821,#9877,.T.);
#21047=EDGE_CURVE('',#16591,#16657,#11033,.T.);
#21048=EDGE_CURVE('',#16658,#16582,#7801,.T.);
#21049=EDGE_CURVE('',#16583,#16659,#7802,.T.);
#21050=EDGE_CURVE('',#16659,#16658,#9878,.T.);
#21051=EDGE_CURVE('',#16193,#16658,#7803,.T.);
#21052=EDGE_CURVE('',#16658,#16660,#11034,.T.);
#21053=EDGE_CURVE('',#16660,#16194,#167,.F.);
#21054=EDGE_CURVE('',#16584,#16659,#7804,.T.);
#21055=EDGE_CURVE('',#16661,#16575,#11035,.T.);
#21056=EDGE_CURVE('',#15818,#16661,#7805,.F.);
#21057=EDGE_CURVE('',#16662,#15817,#9879,.T.);
#21058=EDGE_CURVE('',#16579,#16662,#11036,.T.);
#21059=EDGE_CURVE('',#16663,#16196,#7806,.T.);
#21060=EDGE_CURVE('',#16195,#16664,#168,.F.);
#21061=EDGE_CURVE('',#16664,#16663,#11037,.T.);
#21062=EDGE_CURVE('',#16665,#16666,#7807,.T.);
#21063=EDGE_CURVE('',#16666,#16667,#9880,.T.);
#21064=EDGE_CURVE('',#16667,#16663,#7808,.T.);
#21065=EDGE_CURVE('',#16663,#16665,#9881,.T.);
#21066=EDGE_CURVE('',#16667,#16196,#7809,.T.);
#21067=EDGE_CURVE('',#16668,#16669,#9882,.T.);
#21068=EDGE_CURVE('',#16669,#16670,#11038,.T.);
#21069=EDGE_CURVE('',#16670,#16665,#7810,.T.);
#21070=EDGE_CURVE('',#16665,#16668,#11039,.T.);
#21071=EDGE_CURVE('',#16670,#16666,#7811,.T.);
#21072=EDGE_CURVE('',#16667,#16671,#7812,.T.);
#21073=EDGE_CURVE('',#16197,#16671,#7813,.T.);
#21074=EDGE_CURVE('',#16672,#16666,#7814,.T.);
#21075=EDGE_CURVE('',#16671,#16672,#9883,.T.);
#21076=EDGE_CURVE('',#16670,#16673,#7815,.T.);
#21077=EDGE_CURVE('',#16673,#16672,#7816,.T.);
#21078=EDGE_CURVE('',#16674,#16669,#7817,.T.);
#21079=EDGE_CURVE('',#16673,#16674,#11040,.T.);
#21080=EDGE_CURVE('',#16675,#16252,#7818,.T.);
#21081=EDGE_CURVE('',#16253,#16676,#7819,.T.);
#21082=EDGE_CURVE('',#16676,#16675,#9884,.T.);
#21083=EDGE_CURVE('',#16201,#16675,#7820,.T.);
#21084=EDGE_CURVE('',#16675,#16677,#11041,.T.);
#21085=EDGE_CURVE('',#16677,#16202,#169,.F.);
#21086=EDGE_CURVE('',#16254,#16676,#7821,.T.);
#21087=EDGE_CURVE('',#16255,#16678,#9885,.T.);
#21088=EDGE_CURVE('',#16678,#16676,#11042,.T.);
#21089=EDGE_CURVE('',#16679,#16678,#11043,.T.);
#21090=EDGE_CURVE('',#15804,#16679,#9886,.T.);
#21091=EDGE_CURVE('',#16680,#15803,#7822,.F.);
#21092=EDGE_CURVE('',#16677,#16680,#11044,.T.);
#21093=EDGE_CURVE('',#16681,#16671,#7823,.T.);
#21094=EDGE_CURVE('',#16672,#16682,#7824,.T.);
#21095=EDGE_CURVE('',#16682,#16681,#9887,.T.);
#21096=EDGE_CURVE('',#16197,#16681,#7825,.T.);
#21097=EDGE_CURVE('',#16681,#16683,#11045,.T.);
#21098=EDGE_CURVE('',#16683,#16198,#170,.F.);
#21099=EDGE_CURVE('',#16673,#16682,#7826,.T.);
#21100=EDGE_CURVE('',#16684,#16664,#11046,.T.);
#21101=EDGE_CURVE('',#15810,#16684,#7827,.F.);
#21102=EDGE_CURVE('',#16685,#15809,#9888,.T.);
#21103=EDGE_CURVE('',#16668,#16685,#11047,.T.);
#21104=EDGE_CURVE('',#16585,#16686,#9889,.T.);
#21105=EDGE_CURVE('',#16686,#16659,#11048,.T.);
#21106=EDGE_CURVE('',#16687,#16686,#11049,.T.);
#21107=EDGE_CURVE('',#15816,#16687,#9890,.T.);
#21108=EDGE_CURVE('',#16688,#15815,#7828,.F.);
#21109=EDGE_CURVE('',#16660,#16688,#11050,.T.);
#21110=EDGE_CURVE('',#16597,#16689,#9891,.T.);
#21111=EDGE_CURVE('',#16689,#16654,#11051,.T.);
#21112=EDGE_CURVE('',#16690,#16689,#11052,.T.);
#21113=EDGE_CURVE('',#15820,#16690,#9892,.T.);
#21114=EDGE_CURVE('',#16691,#15819,#7829,.F.);
#21115=EDGE_CURVE('',#16655,#16691,#11053,.T.);
#21116=EDGE_CURVE('',#16692,#16651,#7830,.T.);
#21117=EDGE_CURVE('',#16652,#16693,#7831,.T.);
#21118=EDGE_CURVE('',#16693,#16692,#9893,.T.);
#21119=EDGE_CURVE('',#16650,#16694,#7832,.T.);
#21120=EDGE_CURVE('',#16694,#16652,#7833,.T.);
#21121=EDGE_CURVE('',#16694,#16693,#7834,.T.);
#21122=EDGE_CURVE('',#15825,#16692,#7835,.T.);
#21123=EDGE_CURVE('',#16692,#16695,#11054,.T.);
#21124=EDGE_CURVE('',#16695,#15826,#171,.F.);
#21125=EDGE_CURVE('',#16696,#16644,#11055,.T.);
#21126=EDGE_CURVE('',#16186,#16696,#7836,.F.);
#21127=EDGE_CURVE('',#16697,#16185,#9894,.T.);
#21128=EDGE_CURVE('',#16648,#16697,#11056,.T.);
#21129=EDGE_CURVE('',#16698,#16639,#7837,.T.);
#21130=EDGE_CURVE('',#16640,#16699,#7838,.T.);
#21131=EDGE_CURVE('',#16699,#16698,#9895,.T.);
#21132=EDGE_CURVE('',#16181,#16698,#7839,.T.);
#21133=EDGE_CURVE('',#16698,#16700,#11057,.T.);
#21134=EDGE_CURVE('',#16700,#16182,#172,.F.);
#21135=EDGE_CURVE('',#16641,#16699,#7840,.T.);
#21136=EDGE_CURVE('',#16701,#16632,#11058,.T.);
#21137=EDGE_CURVE('',#15830,#16701,#7841,.F.);
#21138=EDGE_CURVE('',#16702,#15829,#9896,.T.);
#21139=EDGE_CURVE('',#16636,#16702,#11059,.T.);
#21140=EDGE_CURVE('',#16703,#16161,#7842,.T.);
#21141=EDGE_CURVE('',#16160,#16704,#173,.F.);
#21142=EDGE_CURVE('',#16704,#16703,#11060,.T.);
#21143=EDGE_CURVE('',#16705,#16706,#7843,.T.);
#21144=EDGE_CURVE('',#16706,#16707,#9897,.T.);
#21145=EDGE_CURVE('',#16707,#16703,#7844,.T.);
#21146=EDGE_CURVE('',#16703,#16705,#9898,.T.);
#21147=EDGE_CURVE('',#16707,#16161,#7845,.T.);
#21148=EDGE_CURVE('',#16708,#16709,#9899,.T.);
#21149=EDGE_CURVE('',#16709,#16710,#11061,.T.);
#21150=EDGE_CURVE('',#16710,#16705,#7846,.T.);
#21151=EDGE_CURVE('',#16705,#16708,#11062,.T.);
#21152=EDGE_CURVE('',#16710,#16706,#7847,.T.);
#21153=EDGE_CURVE('',#16707,#16711,#7848,.T.);
#21154=EDGE_CURVE('',#16162,#16711,#7849,.T.);
#21155=EDGE_CURVE('',#16712,#16706,#7850,.T.);
#21156=EDGE_CURVE('',#16711,#16712,#9900,.T.);
#21157=EDGE_CURVE('',#16710,#16713,#7851,.T.);
#21158=EDGE_CURVE('',#16713,#16712,#7852,.T.);
#21159=EDGE_CURVE('',#16714,#16709,#7853,.T.);
#21160=EDGE_CURVE('',#16713,#16714,#11063,.T.);
#21161=EDGE_CURVE('',#16715,#16240,#7854,.T.);
#21162=EDGE_CURVE('',#16241,#16716,#7855,.T.);
#21163=EDGE_CURVE('',#16716,#16715,#9901,.T.);
#21164=EDGE_CURVE('',#16177,#16715,#7856,.T.);
#21165=EDGE_CURVE('',#16715,#16717,#11064,.T.);
#21166=EDGE_CURVE('',#16717,#16178,#174,.F.);
#21167=EDGE_CURVE('',#16242,#16716,#7857,.T.);
#21168=EDGE_CURVE('',#16243,#16718,#9902,.T.);
#21169=EDGE_CURVE('',#16718,#16716,#11065,.T.);
#21170=EDGE_CURVE('',#16719,#16718,#11066,.T.);
#21171=EDGE_CURVE('',#15832,#16719,#9903,.T.);
#21172=EDGE_CURVE('',#16720,#15831,#7858,.F.);
#21173=EDGE_CURVE('',#16717,#16720,#11067,.T.);
#21174=EDGE_CURVE('',#16721,#16153,#7859,.T.);
#21175=EDGE_CURVE('',#16152,#16722,#175,.F.);
#21176=EDGE_CURVE('',#16722,#16721,#11068,.T.);
#21177=EDGE_CURVE('',#16723,#16724,#7860,.T.);
#21178=EDGE_CURVE('',#16724,#16725,#9904,.T.);
#21179=EDGE_CURVE('',#16725,#16721,#7861,.T.);
#21180=EDGE_CURVE('',#16721,#16723,#9905,.T.);
#21181=EDGE_CURVE('',#16725,#16153,#7862,.T.);
#21182=EDGE_CURVE('',#16726,#16727,#9906,.T.);
#21183=EDGE_CURVE('',#16727,#16728,#11069,.T.);
#21184=EDGE_CURVE('',#16728,#16723,#7863,.T.);
#21185=EDGE_CURVE('',#16723,#16726,#11070,.T.);
#21186=EDGE_CURVE('',#16728,#16724,#7864,.T.);
#21187=EDGE_CURVE('',#16725,#16729,#7865,.T.);
#21188=EDGE_CURVE('',#16154,#16729,#7866,.T.);
#21189=EDGE_CURVE('',#16730,#16724,#7867,.T.);
#21190=EDGE_CURVE('',#16729,#16730,#9907,.T.);
#21191=EDGE_CURVE('',#16728,#16731,#7868,.T.);
#21192=EDGE_CURVE('',#16731,#16730,#7869,.T.);
#21193=EDGE_CURVE('',#16732,#16727,#7870,.T.);
#21194=EDGE_CURVE('',#16731,#16732,#11071,.T.);
#21195=EDGE_CURVE('',#16733,#16149,#7871,.T.);
#21196=EDGE_CURVE('',#16148,#16734,#176,.F.);
#21197=EDGE_CURVE('',#16734,#16733,#11072,.T.);
#21198=EDGE_CURVE('',#16735,#16736,#7872,.T.);
#21199=EDGE_CURVE('',#16736,#16737,#9908,.T.);
#21200=EDGE_CURVE('',#16737,#16733,#7873,.T.);
#21201=EDGE_CURVE('',#16733,#16735,#9909,.T.);
#21202=EDGE_CURVE('',#16737,#16149,#7874,.T.);
#21203=EDGE_CURVE('',#16738,#16739,#9910,.T.);
#21204=EDGE_CURVE('',#16739,#16740,#11073,.T.);
#21205=EDGE_CURVE('',#16740,#16735,#7875,.T.);
#21206=EDGE_CURVE('',#16735,#16738,#11074,.T.);
#21207=EDGE_CURVE('',#16740,#16736,#7876,.T.);
#21208=EDGE_CURVE('',#16737,#16741,#7877,.T.);
#21209=EDGE_CURVE('',#16150,#16741,#7878,.T.);
#21210=EDGE_CURVE('',#16742,#16736,#7879,.T.);
#21211=EDGE_CURVE('',#16741,#16742,#9911,.T.);
#21212=EDGE_CURVE('',#16740,#16743,#7880,.T.);
#21213=EDGE_CURVE('',#16743,#16742,#7881,.T.);
#21214=EDGE_CURVE('',#16744,#16739,#7882,.T.);
#21215=EDGE_CURVE('',#16743,#16744,#11075,.T.);
#21216=EDGE_CURVE('',#16745,#16711,#7883,.T.);
#21217=EDGE_CURVE('',#16712,#16746,#7884,.T.);
#21218=EDGE_CURVE('',#16746,#16745,#9912,.T.);
#21219=EDGE_CURVE('',#16162,#16745,#7885,.T.);
#21220=EDGE_CURVE('',#16745,#16747,#11076,.T.);
#21221=EDGE_CURVE('',#16747,#16163,#177,.F.);
#21222=EDGE_CURVE('',#16713,#16746,#7886,.T.);
#21223=EDGE_CURVE('',#16748,#16704,#11077,.T.);
#21224=EDGE_CURVE('',#15854,#16748,#7887,.F.);
#21225=EDGE_CURVE('',#16749,#15853,#9913,.T.);
#21226=EDGE_CURVE('',#16708,#16749,#11078,.T.);
#21227=EDGE_CURVE('',#16750,#15848,#7888,.T.);
#21228=EDGE_CURVE('',#15847,#16751,#178,.F.);
#21229=EDGE_CURVE('',#16751,#16750,#11079,.T.);
#21230=EDGE_CURVE('',#16752,#16753,#7889,.T.);
#21231=EDGE_CURVE('',#16753,#16754,#9914,.T.);
#21232=EDGE_CURVE('',#16754,#16750,#7890,.T.);
#21233=EDGE_CURVE('',#16750,#16752,#9915,.T.);
#21234=EDGE_CURVE('',#16754,#15848,#7891,.T.);
#21235=EDGE_CURVE('',#16755,#16756,#9916,.T.);
#21236=EDGE_CURVE('',#16756,#16757,#11080,.T.);
#21237=EDGE_CURVE('',#16757,#16752,#7892,.T.);
#21238=EDGE_CURVE('',#16752,#16755,#11081,.T.);
#21239=EDGE_CURVE('',#16757,#16753,#7893,.T.);
#21240=EDGE_CURVE('',#16754,#16758,#7894,.T.);
#21241=EDGE_CURVE('',#15849,#16758,#7895,.T.);
#21242=EDGE_CURVE('',#16759,#16753,#7896,.T.);
#21243=EDGE_CURVE('',#16758,#16759,#9917,.T.);
#21244=EDGE_CURVE('',#16760,#16169,#7897,.T.);
#21245=EDGE_CURVE('',#16168,#16761,#179,.F.);
#21246=EDGE_CURVE('',#16761,#16760,#11082,.T.);
#21247=EDGE_CURVE('',#16762,#16763,#7898,.T.);
#21248=EDGE_CURVE('',#16763,#16764,#9918,.T.);
#21249=EDGE_CURVE('',#16764,#16760,#7899,.T.);
#21250=EDGE_CURVE('',#16760,#16762,#9919,.T.);
#21251=EDGE_CURVE('',#16764,#16169,#7900,.T.);
#21252=EDGE_CURVE('',#16765,#16766,#9920,.T.);
#21253=EDGE_CURVE('',#16766,#16767,#11083,.T.);
#21254=EDGE_CURVE('',#16767,#16762,#7901,.T.);
#21255=EDGE_CURVE('',#16762,#16765,#11084,.T.);
#21256=EDGE_CURVE('',#16767,#16763,#7902,.T.);
#21257=EDGE_CURVE('',#16764,#16768,#7903,.T.);
#21258=EDGE_CURVE('',#16170,#16768,#7904,.T.);
#21259=EDGE_CURVE('',#16769,#16763,#7905,.T.);
#21260=EDGE_CURVE('',#16768,#16769,#9921,.T.);
#21261=EDGE_CURVE('',#16767,#16770,#7906,.T.);
#21262=EDGE_CURVE('',#16770,#16769,#7907,.T.);
#21263=EDGE_CURVE('',#16771,#16766,#7908,.T.);
#21264=EDGE_CURVE('',#16770,#16771,#11085,.T.);
#21265=EDGE_CURVE('',#16056,#16050,#7909,.T.);
#21266=EDGE_CURVE('',#16052,#16054,#7910,.T.);
#21267=EDGE_CURVE('',#16051,#16056,#7911,.T.);
#21268=EDGE_CURVE('',#16055,#16172,#180,.F.);
#21269=EDGE_CURVE('',#16772,#15836,#7912,.T.);
#21270=EDGE_CURVE('',#15835,#16773,#181,.F.);
#21271=EDGE_CURVE('',#16773,#16772,#11086,.T.);
#21272=EDGE_CURVE('',#16774,#16775,#7913,.T.);
#21273=EDGE_CURVE('',#16775,#16776,#9922,.T.);
#21274=EDGE_CURVE('',#16776,#16772,#7914,.T.);
#21275=EDGE_CURVE('',#16772,#16774,#9923,.T.);
#21276=EDGE_CURVE('',#16776,#15836,#7915,.T.);
#21277=EDGE_CURVE('',#16777,#16778,#9924,.T.);
#21278=EDGE_CURVE('',#16778,#16779,#11087,.T.);
#21279=EDGE_CURVE('',#16779,#16774,#7916,.T.);
#21280=EDGE_CURVE('',#16774,#16777,#11088,.T.);
#21281=EDGE_CURVE('',#16779,#16775,#7917,.T.);
#21282=EDGE_CURVE('',#16776,#16780,#7918,.T.);
#21283=EDGE_CURVE('',#15837,#16780,#7919,.T.);
#21284=EDGE_CURVE('',#16781,#16775,#7920,.T.);
#21285=EDGE_CURVE('',#16780,#16781,#9925,.T.);
#21286=EDGE_CURVE('',#16782,#16780,#7921,.T.);
#21287=EDGE_CURVE('',#16781,#16783,#7922,.T.);
#21288=EDGE_CURVE('',#16783,#16782,#9926,.T.);
#21289=EDGE_CURVE('',#16779,#16784,#7923,.T.);
#21290=EDGE_CURVE('',#16784,#16781,#7924,.T.);
#21291=EDGE_CURVE('',#16784,#16783,#7925,.T.);
#21292=EDGE_CURVE('',#15837,#16782,#7926,.T.);
#21293=EDGE_CURVE('',#16782,#16785,#11089,.T.);
#21294=EDGE_CURVE('',#16785,#15838,#182,.F.);
#21295=EDGE_CURVE('',#16786,#16773,#11090,.T.);
#21296=EDGE_CURVE('',#16176,#16786,#7927,.F.);
#21297=EDGE_CURVE('',#16787,#16175,#9927,.T.);
#21298=EDGE_CURVE('',#16777,#16787,#11091,.T.);
#21299=EDGE_CURVE('',#16788,#16768,#7928,.T.);
#21300=EDGE_CURVE('',#16769,#16789,#7929,.T.);
#21301=EDGE_CURVE('',#16789,#16788,#9928,.T.);
#21302=EDGE_CURVE('',#16170,#16788,#7930,.T.);
#21303=EDGE_CURVE('',#16788,#16790,#11092,.T.);
#21304=EDGE_CURVE('',#16790,#16171,#183,.F.);
#21305=EDGE_CURVE('',#16770,#16789,#7931,.T.);
#21306=EDGE_CURVE('',#16791,#16761,#11093,.T.);
#21307=EDGE_CURVE('',#15846,#16791,#7932,.F.);
#21308=EDGE_CURVE('',#16792,#15845,#9929,.T.);
#21309=EDGE_CURVE('',#16765,#16792,#11094,.T.);
#21310=EDGE_CURVE('',#16793,#16758,#7933,.T.);
#21311=EDGE_CURVE('',#16759,#16794,#7934,.T.);
#21312=EDGE_CURVE('',#16794,#16793,#9930,.T.);
#21313=EDGE_CURVE('',#16757,#16795,#7935,.T.);
#21314=EDGE_CURVE('',#16795,#16759,#7936,.T.);
#21315=EDGE_CURVE('',#16795,#16794,#7937,.T.);
#21316=EDGE_CURVE('',#15849,#16793,#7938,.T.);
#21317=EDGE_CURVE('',#16793,#16796,#11095,.T.);
#21318=EDGE_CURVE('',#16796,#15850,#184,.F.);
#21319=EDGE_CURVE('',#16797,#16751,#11096,.T.);
#21320=EDGE_CURVE('',#16167,#16797,#7939,.F.);
#21321=EDGE_CURVE('',#16798,#16166,#9931,.T.);
#21322=EDGE_CURVE('',#16755,#16798,#11097,.T.);
#21323=EDGE_CURVE('',#16714,#16799,#9932,.T.);
#21324=EDGE_CURVE('',#16799,#16746,#11098,.T.);
#21325=EDGE_CURVE('',#16800,#16799,#11099,.T.);
#21326=EDGE_CURVE('',#15852,#16800,#9933,.T.);
#21327=EDGE_CURVE('',#16801,#15851,#7940,.F.);
#21328=EDGE_CURVE('',#16747,#16801,#11100,.T.);
#21329=EDGE_CURVE('',#16802,#16741,#7941,.T.);
#21330=EDGE_CURVE('',#16742,#16803,#7942,.T.);
#21331=EDGE_CURVE('',#16803,#16802,#9934,.T.);
#21332=EDGE_CURVE('',#16150,#16802,#7943,.T.);
#21333=EDGE_CURVE('',#16802,#16804,#11101,.T.);
#21334=EDGE_CURVE('',#16804,#16151,#185,.F.);
#21335=EDGE_CURVE('',#16743,#16803,#7944,.T.);
#21336=EDGE_CURVE('',#16805,#16734,#11102,.T.);
#21337=EDGE_CURVE('',#15870,#16805,#7945,.F.);
#21338=EDGE_CURVE('',#16806,#15869,#9935,.T.);
#21339=EDGE_CURVE('',#16738,#16806,#11103,.T.);
#21340=EDGE_CURVE('',#16807,#16729,#7946,.T.);
#21341=EDGE_CURVE('',#16730,#16808,#7947,.T.);
#21342=EDGE_CURVE('',#16808,#16807,#9936,.T.);
#21343=EDGE_CURVE('',#16154,#16807,#7948,.T.);
#21344=EDGE_CURVE('',#16807,#16809,#11104,.T.);
#21345=EDGE_CURVE('',#16809,#16155,#186,.F.);
#21346=EDGE_CURVE('',#16731,#16808,#7949,.T.);
#21347=EDGE_CURVE('',#16810,#16722,#11105,.T.);
#21348=EDGE_CURVE('',#15866,#16810,#7950,.F.);
#21349=EDGE_CURVE('',#16811,#15865,#9937,.T.);
#21350=EDGE_CURVE('',#16726,#16811,#11106,.T.);
#21351=EDGE_CURVE('',#16812,#16157,#7951,.T.);
#21352=EDGE_CURVE('',#16156,#16813,#187,.F.);
#21353=EDGE_CURVE('',#16813,#16812,#11107,.T.);
#21354=EDGE_CURVE('',#16814,#16815,#7952,.T.);
#21355=EDGE_CURVE('',#16815,#16816,#9938,.T.);
#21356=EDGE_CURVE('',#16816,#16812,#7953,.T.);
#21357=EDGE_CURVE('',#16812,#16814,#9939,.T.);
#21358=EDGE_CURVE('',#16816,#16157,#7954,.T.);
#21359=EDGE_CURVE('',#16817,#16818,#9940,.T.);
#21360=EDGE_CURVE('',#16818,#16819,#11108,.T.);
#21361=EDGE_CURVE('',#16819,#16814,#7955,.T.);
#21362=EDGE_CURVE('',#16814,#16817,#11109,.T.);
#21363=EDGE_CURVE('',#16819,#16815,#7956,.T.);
#21364=EDGE_CURVE('',#16816,#16820,#7957,.T.);
#21365=EDGE_CURVE('',#16158,#16820,#7958,.T.);
#21366=EDGE_CURVE('',#16821,#16815,#7959,.T.);
#21367=EDGE_CURVE('',#16820,#16821,#9941,.T.);
#21368=EDGE_CURVE('',#16819,#16822,#7960,.T.);
#21369=EDGE_CURVE('',#16822,#16821,#7961,.T.);
#21370=EDGE_CURVE('',#16823,#16818,#7962,.T.);
#21371=EDGE_CURVE('',#16822,#16823,#11110,.T.);
#21372=EDGE_CURVE('',#16824,#16820,#7963,.T.);
#21373=EDGE_CURVE('',#16821,#16825,#7964,.T.);
#21374=EDGE_CURVE('',#16825,#16824,#9942,.T.);
#21375=EDGE_CURVE('',#16158,#16824,#7965,.T.);
#21376=EDGE_CURVE('',#16824,#16826,#11111,.T.);
#21377=EDGE_CURVE('',#16826,#16159,#188,.F.);
#21378=EDGE_CURVE('',#16822,#16825,#7966,.T.);
#21379=EDGE_CURVE('',#16827,#16813,#11112,.T.);
#21380=EDGE_CURVE('',#15858,#16827,#7967,.F.);
#21381=EDGE_CURVE('',#16828,#15857,#9943,.T.);
#21382=EDGE_CURVE('',#16817,#16828,#11113,.T.);
#21383=EDGE_CURVE('',#16732,#16829,#9944,.T.);
#21384=EDGE_CURVE('',#16829,#16808,#11114,.T.);
#21385=EDGE_CURVE('',#16830,#16829,#11115,.T.);
#21386=EDGE_CURVE('',#15864,#16830,#9945,.T.);
#21387=EDGE_CURVE('',#16831,#15863,#7968,.F.);
#21388=EDGE_CURVE('',#16809,#16831,#11116,.T.);
#21389=EDGE_CURVE('',#16744,#16832,#9946,.T.);
#21390=EDGE_CURVE('',#16832,#16803,#11117,.T.);
#21391=EDGE_CURVE('',#16833,#16832,#11118,.T.);
#21392=EDGE_CURVE('',#15868,#16833,#9947,.T.);
#21393=EDGE_CURVE('',#16834,#15867,#7969,.F.);
#21394=EDGE_CURVE('',#16804,#16834,#11119,.T.);
#21395=EDGE_CURVE('',#16835,#16132,#7970,.T.);
#21396=EDGE_CURVE('',#16131,#16836,#189,.F.);
#21397=EDGE_CURVE('',#16836,#16835,#11120,.T.);
#21398=EDGE_CURVE('',#16837,#16838,#7971,.T.);
#21399=EDGE_CURVE('',#16838,#16839,#9948,.T.);
#21400=EDGE_CURVE('',#16839,#16835,#7972,.T.);
#21401=EDGE_CURVE('',#16835,#16837,#9949,.T.);
#21402=EDGE_CURVE('',#16839,#16132,#7973,.T.);
#21403=EDGE_CURVE('',#16840,#16841,#9950,.T.);
#21404=EDGE_CURVE('',#16841,#16842,#11121,.T.);
#21405=EDGE_CURVE('',#16842,#16837,#7974,.T.);
#21406=EDGE_CURVE('',#16837,#16840,#11122,.T.);
#21407=EDGE_CURVE('',#16842,#16838,#7975,.T.);
#21408=EDGE_CURVE('',#16839,#16843,#7976,.T.);
#21409=EDGE_CURVE('',#16133,#16843,#7977,.T.);
#21410=EDGE_CURVE('',#16844,#16838,#7978,.T.);
#21411=EDGE_CURVE('',#16843,#16844,#9951,.T.);
#21412=EDGE_CURVE('',#16842,#16845,#7979,.T.);
#21413=EDGE_CURVE('',#16845,#16844,#7980,.T.);
#21414=EDGE_CURVE('',#16846,#16841,#7981,.T.);
#21415=EDGE_CURVE('',#16845,#16846,#11123,.T.);
#21416=EDGE_CURVE('',#16847,#15896,#7982,.T.);
#21417=EDGE_CURVE('',#15895,#16848,#190,.F.);
#21418=EDGE_CURVE('',#16848,#16847,#11124,.T.);
#21419=EDGE_CURVE('',#16849,#16850,#7983,.T.);
#21420=EDGE_CURVE('',#16850,#16851,#9952,.T.);
#21421=EDGE_CURVE('',#16851,#16847,#7984,.T.);
#21422=EDGE_CURVE('',#16847,#16849,#9953,.T.);
#21423=EDGE_CURVE('',#16851,#15896,#7985,.T.);
#21424=EDGE_CURVE('',#16852,#16853,#9954,.T.);
#21425=EDGE_CURVE('',#16853,#16854,#11125,.T.);
#21426=EDGE_CURVE('',#16854,#16849,#7986,.T.);
#21427=EDGE_CURVE('',#16849,#16852,#11126,.T.);
#21428=EDGE_CURVE('',#16854,#16850,#7987,.T.);
#21429=EDGE_CURVE('',#16851,#16855,#7988,.T.);
#21430=EDGE_CURVE('',#15897,#16855,#7989,.T.);
#21431=EDGE_CURVE('',#16856,#16850,#7990,.T.);
#21432=EDGE_CURVE('',#16855,#16856,#9955,.T.);
#21433=EDGE_CURVE('',#16857,#16128,#7991,.T.);
#21434=EDGE_CURVE('',#16127,#16858,#191,.F.);
#21435=EDGE_CURVE('',#16858,#16857,#11127,.T.);
#21436=EDGE_CURVE('',#16859,#16860,#7992,.T.);
#21437=EDGE_CURVE('',#16860,#16861,#9956,.T.);
#21438=EDGE_CURVE('',#16861,#16857,#7993,.T.);
#21439=EDGE_CURVE('',#16857,#16859,#9957,.T.);
#21440=EDGE_CURVE('',#16861,#16128,#7994,.T.);
#21441=EDGE_CURVE('',#16862,#16863,#9958,.T.);
#21442=EDGE_CURVE('',#16863,#16864,#11128,.T.);
#21443=EDGE_CURVE('',#16864,#16859,#7995,.T.);
#21444=EDGE_CURVE('',#16859,#16862,#11129,.T.);
#21445=EDGE_CURVE('',#16864,#16860,#7996,.T.);
#21446=EDGE_CURVE('',#16861,#16865,#7997,.T.);
#21447=EDGE_CURVE('',#16129,#16865,#7998,.T.);
#21448=EDGE_CURVE('',#16866,#16860,#7999,.T.);
#21449=EDGE_CURVE('',#16865,#16866,#9959,.T.);
#21450=EDGE_CURVE('',#16864,#16867,#8000,.T.);
#21451=EDGE_CURVE('',#16867,#16866,#8001,.T.);
#21452=EDGE_CURVE('',#16868,#16863,#8002,.T.);
#21453=EDGE_CURVE('',#16867,#16868,#11130,.T.);
#21454=EDGE_CURVE('',#16869,#16141,#8003,.T.);
#21455=EDGE_CURVE('',#16140,#16870,#192,.F.);
#21456=EDGE_CURVE('',#16870,#16869,#11131,.T.);
#21457=EDGE_CURVE('',#16871,#16872,#8004,.T.);
#21458=EDGE_CURVE('',#16872,#16873,#9960,.T.);
#21459=EDGE_CURVE('',#16873,#16869,#8005,.T.);
#21460=EDGE_CURVE('',#16869,#16871,#9961,.T.);
#21461=EDGE_CURVE('',#16873,#16141,#8006,.T.);
#21462=EDGE_CURVE('',#16874,#16875,#9962,.T.);
#21463=EDGE_CURVE('',#16875,#16876,#11132,.T.);
#21464=EDGE_CURVE('',#16876,#16871,#8007,.T.);
#21465=EDGE_CURVE('',#16871,#16874,#11133,.T.);
#21466=EDGE_CURVE('',#16876,#16872,#8008,.T.);
#21467=EDGE_CURVE('',#16873,#16877,#8009,.T.);
#21468=EDGE_CURVE('',#16142,#16877,#8010,.T.);
#21469=EDGE_CURVE('',#16878,#16872,#8011,.T.);
#21470=EDGE_CURVE('',#16877,#16878,#9963,.T.);
#21471=EDGE_CURVE('',#16876,#16879,#8012,.T.);
#21472=EDGE_CURVE('',#16879,#16878,#8013,.T.);
#21473=EDGE_CURVE('',#16880,#16875,#8014,.T.);
#21474=EDGE_CURVE('',#16879,#16880,#11134,.T.);
#21475=EDGE_CURVE('',#16881,#15872,#8015,.T.);
#21476=EDGE_CURVE('',#15871,#16882,#193,.F.);
#21477=EDGE_CURVE('',#16882,#16881,#11135,.T.);
#21478=EDGE_CURVE('',#16883,#16884,#8016,.T.);
#21479=EDGE_CURVE('',#16884,#16885,#9964,.T.);
#21480=EDGE_CURVE('',#16885,#16881,#8017,.T.);
#21481=EDGE_CURVE('',#16881,#16883,#9965,.T.);
#21482=EDGE_CURVE('',#16885,#15872,#8018,.T.);
#21483=EDGE_CURVE('',#16886,#16887,#9966,.T.);
#21484=EDGE_CURVE('',#16887,#16888,#11136,.T.);
#21485=EDGE_CURVE('',#16888,#16883,#8019,.T.);
#21486=EDGE_CURVE('',#16883,#16886,#11137,.T.);
#21487=EDGE_CURVE('',#16888,#16884,#8020,.T.);
#21488=EDGE_CURVE('',#16885,#16889,#8021,.T.);
#21489=EDGE_CURVE('',#15873,#16889,#8022,.T.);
#21490=EDGE_CURVE('',#16890,#16884,#8023,.T.);
#21491=EDGE_CURVE('',#16889,#16890,#9967,.T.);
#21492=EDGE_CURVE('',#16891,#16889,#8024,.T.);
#21493=EDGE_CURVE('',#16890,#16892,#8025,.T.);
#21494=EDGE_CURVE('',#16892,#16891,#9968,.T.);
#21495=EDGE_CURVE('',#16888,#16893,#8026,.T.);
#21496=EDGE_CURVE('',#16893,#16890,#8027,.T.);
#21497=EDGE_CURVE('',#16893,#16892,#8028,.T.);
#21498=EDGE_CURVE('',#15873,#16891,#8029,.T.);
#21499=EDGE_CURVE('',#16891,#16894,#11138,.T.);
#21500=EDGE_CURVE('',#16894,#15874,#194,.F.);
#21501=EDGE_CURVE('',#16895,#16882,#11139,.T.);
#21502=EDGE_CURVE('',#16147,#16895,#8030,.F.);
#21503=EDGE_CURVE('',#16896,#16146,#9969,.T.);
#21504=EDGE_CURVE('',#16886,#16896,#11140,.T.);
#21505=EDGE_CURVE('',#16897,#16877,#8031,.T.);
#21506=EDGE_CURVE('',#16878,#16898,#8032,.T.);
#21507=EDGE_CURVE('',#16898,#16897,#9970,.T.);
#21508=EDGE_CURVE('',#16142,#16897,#8033,.T.);
#21509=EDGE_CURVE('',#16897,#16899,#11141,.T.);
#21510=EDGE_CURVE('',#16899,#16143,#195,.F.);
#21511=EDGE_CURVE('',#16879,#16898,#8034,.T.);
#21512=EDGE_CURVE('',#16900,#16870,#11142,.T.);
#21513=EDGE_CURVE('',#15878,#16900,#8035,.F.);
#21514=EDGE_CURVE('',#16901,#15877,#9971,.T.);
#21515=EDGE_CURVE('',#16874,#16901,#11143,.T.);
#21516=EDGE_CURVE('',#16902,#16865,#8036,.T.);
#21517=EDGE_CURVE('',#16866,#16903,#8037,.T.);
#21518=EDGE_CURVE('',#16903,#16902,#9972,.T.);
#21519=EDGE_CURVE('',#16129,#16902,#8038,.T.);
#21520=EDGE_CURVE('',#16902,#16904,#11144,.T.);
#21521=EDGE_CURVE('',#16904,#16130,#196,.F.);
#21522=EDGE_CURVE('',#16867,#16903,#8039,.T.);
#21523=EDGE_CURVE('',#16905,#16858,#11145,.T.);
#21524=EDGE_CURVE('',#15894,#16905,#8040,.F.);
#21525=EDGE_CURVE('',#16906,#15893,#9973,.T.);
#21526=EDGE_CURVE('',#16862,#16906,#11146,.T.);
#21527=EDGE_CURVE('',#16907,#16855,#8041,.T.);
#21528=EDGE_CURVE('',#16856,#16908,#8042,.T.);
#21529=EDGE_CURVE('',#16908,#16907,#9974,.T.);
#21530=EDGE_CURVE('',#16854,#16909,#8043,.T.);
#21531=EDGE_CURVE('',#16909,#16856,#8044,.T.);
#21532=EDGE_CURVE('',#16909,#16908,#8045,.T.);
#21533=EDGE_CURVE('',#15897,#16907,#8046,.T.);
#21534=EDGE_CURVE('',#16907,#16910,#11147,.T.);
#21535=EDGE_CURVE('',#16910,#15898,#197,.F.);
#21536=EDGE_CURVE('',#16911,#16848,#11148,.T.);
#21537=EDGE_CURVE('',#16126,#16911,#8047,.F.);
#21538=EDGE_CURVE('',#16912,#16125,#9975,.T.);
#21539=EDGE_CURVE('',#16852,#16912,#11149,.T.);
#21540=EDGE_CURVE('',#16913,#16914,#9976,.T.);
#21541=EDGE_CURVE('',#16914,#16915,#11150,.T.);
#21542=EDGE_CURVE('',#16915,#16916,#9977,.T.);
#21543=EDGE_CURVE('',#16916,#16913,#11151,.T.);
#21544=EDGE_CURVE('',#16913,#16917,#11152,.T.);
#21545=EDGE_CURVE('',#16918,#16917,#8048,.T.);
#21546=EDGE_CURVE('',#16918,#16919,#11153,.T.);
#21547=EDGE_CURVE('',#16920,#16919,#9978,.T.);
#21548=EDGE_CURVE('',#16914,#16920,#8049,.T.);
#21549=EDGE_CURVE('',#16921,#16916,#11154,.T.);
#21550=EDGE_CURVE('',#15900,#16921,#9979,.T.);
#21551=EDGE_CURVE('',#16922,#15899,#8050,.F.);
#21552=EDGE_CURVE('',#16923,#16922,#11155,.T.);
#21553=EDGE_CURVE('',#16122,#16923,#8051,.F.);
#21554=EDGE_CURVE('',#16917,#16121,#9980,.T.);
#21555=EDGE_CURVE('',#16924,#16843,#8052,.T.);
#21556=EDGE_CURVE('',#16844,#16925,#8053,.T.);
#21557=EDGE_CURVE('',#16925,#16924,#9981,.T.);
#21558=EDGE_CURVE('',#16133,#16924,#8054,.T.);
#21559=EDGE_CURVE('',#16924,#16926,#11156,.T.);
#21560=EDGE_CURVE('',#16926,#16134,#198,.F.);
#21561=EDGE_CURVE('',#16845,#16925,#8055,.T.);
#21562=EDGE_CURVE('',#16927,#16836,#11157,.T.);
#21563=EDGE_CURVE('',#15890,#16927,#8056,.F.);
#21564=EDGE_CURVE('',#16928,#15889,#9982,.T.);
#21565=EDGE_CURVE('',#16840,#16928,#11158,.T.);
#21566=EDGE_CURVE('',#16929,#15884,#8057,.T.);
#21567=EDGE_CURVE('',#15883,#16930,#199,.F.);
#21568=EDGE_CURVE('',#16930,#16929,#11159,.T.);
#21569=EDGE_CURVE('',#16931,#16932,#8058,.T.);
#21570=EDGE_CURVE('',#16932,#16933,#9983,.T.);
#21571=EDGE_CURVE('',#16933,#16929,#8059,.T.);
#21572=EDGE_CURVE('',#16929,#16931,#9984,.T.);
#21573=EDGE_CURVE('',#16933,#15884,#8060,.T.);
#21574=EDGE_CURVE('',#16934,#16935,#9985,.T.);
#21575=EDGE_CURVE('',#16935,#16936,#11160,.T.);
#21576=EDGE_CURVE('',#16936,#16931,#8061,.T.);
#21577=EDGE_CURVE('',#16931,#16934,#11161,.T.);
#21578=EDGE_CURVE('',#16936,#16932,#8062,.T.);
#21579=EDGE_CURVE('',#16933,#16937,#8063,.T.);
#21580=EDGE_CURVE('',#15885,#16937,#8064,.T.);
#21581=EDGE_CURVE('',#16938,#16932,#8065,.T.);
#21582=EDGE_CURVE('',#16937,#16938,#9986,.T.);
#21583=EDGE_CURVE('',#16032,#16026,#8066,.T.);
#21584=EDGE_CURVE('',#16028,#16030,#8067,.T.);
#21585=EDGE_CURVE('',#16027,#16032,#8068,.T.);
#21586=EDGE_CURVE('',#16031,#16139,#200,.F.);
#21587=EDGE_CURVE('',#16939,#16937,#8069,.T.);
#21588=EDGE_CURVE('',#16938,#16940,#8070,.T.);
#21589=EDGE_CURVE('',#16940,#16939,#9987,.T.);
#21590=EDGE_CURVE('',#16936,#16941,#8071,.T.);
#21591=EDGE_CURVE('',#16941,#16938,#8072,.T.);
#21592=EDGE_CURVE('',#16941,#16940,#8073,.T.);
#21593=EDGE_CURVE('',#15885,#16939,#8074,.T.);
#21594=EDGE_CURVE('',#16939,#16942,#11162,.T.);
#21595=EDGE_CURVE('',#16942,#15886,#201,.F.);
#21596=EDGE_CURVE('',#16943,#16930,#11163,.T.);
#21597=EDGE_CURVE('',#16138,#16943,#8075,.F.);
#21598=EDGE_CURVE('',#16944,#16137,#9988,.T.);
#21599=EDGE_CURVE('',#16934,#16944,#11164,.T.);
#21600=EDGE_CURVE('',#16846,#16945,#9989,.T.);
#21601=EDGE_CURVE('',#16945,#16925,#11165,.T.);
#21602=EDGE_CURVE('',#16946,#16945,#11166,.T.);
#21603=EDGE_CURVE('',#15888,#16946,#9990,.T.);
#21604=EDGE_CURVE('',#16947,#15887,#8076,.F.);
#21605=EDGE_CURVE('',#16926,#16947,#11167,.T.);
#21606=EDGE_CURVE('',#16948,#15905,#9991,.T.);
#21607=EDGE_CURVE('',#15904,#16949,#8077,.T.);
#21608=EDGE_CURVE('',#16949,#16948,#8078,.T.);
#21609=EDGE_CURVE('',#16950,#15904,#8079,.T.);
#21610=EDGE_CURVE('',#15903,#16951,#202,.F.);
#21611=EDGE_CURVE('',#16951,#16950,#11168,.T.);
#21612=EDGE_CURVE('',#16950,#16949,#8080,.T.);
#21613=EDGE_CURVE('',#16950,#16952,#9992,.T.);
#21614=EDGE_CURVE('',#16952,#16953,#8081,.T.);
#21615=EDGE_CURVE('',#16953,#16949,#9993,.T.);
#21616=EDGE_CURVE('',#16954,#16951,#11169,.T.);
#21617=EDGE_CURVE('',#16955,#16954,#11170,.T.);
#21618=EDGE_CURVE('',#16956,#16955,#9994,.T.);
#21619=EDGE_CURVE('',#16952,#16956,#11171,.T.);
#21620=EDGE_CURVE('',#16957,#15901,#9995,.T.);
#21621=EDGE_CURVE('',#16921,#16957,#8082,.T.);
#21622=EDGE_CURVE('',#16910,#16922,#11172,.T.);
#21623=EDGE_CURVE('',#16910,#16958,#11173,.T.);
#21624=EDGE_CURVE('',#16923,#16958,#11174,.T.);
#21625=EDGE_CURVE('',#16959,#16908,#11175,.T.);
#21626=EDGE_CURVE('',#16960,#16959,#11176,.T.);
#21627=EDGE_CURVE('',#16124,#16960,#9996,.T.);
#21628=EDGE_CURVE('',#16958,#16123,#8083,.F.);
#21629=EDGE_CURVE('',#16868,#16961,#9997,.T.);
#21630=EDGE_CURVE('',#16961,#16903,#11177,.T.);
#21631=EDGE_CURVE('',#16962,#16961,#11178,.T.);
#21632=EDGE_CURVE('',#15892,#16962,#9998,.T.);
#21633=EDGE_CURVE('',#16963,#15891,#8084,.F.);
#21634=EDGE_CURVE('',#16904,#16963,#11179,.T.);
#21635=EDGE_CURVE('',#16962,#16906,#8085,.T.);
#21636=EDGE_CURVE('',#16927,#16963,#11180,.T.);
#21637=EDGE_CURVE('',#16904,#16836,#11181,.T.);
#21638=EDGE_CURVE('',#16946,#16928,#8086,.T.);
#21639=EDGE_CURVE('',#16942,#16947,#11182,.T.);
#21640=EDGE_CURVE('',#16942,#16964,#11183,.T.);
#21641=EDGE_CURVE('',#16926,#16964,#11184,.T.);
#21642=EDGE_CURVE('',#16965,#16940,#11185,.T.);
#21643=EDGE_CURVE('',#16966,#16965,#11186,.T.);
#21644=EDGE_CURVE('',#16136,#16966,#9999,.T.);
#21645=EDGE_CURVE('',#16964,#16135,#8087,.F.);
#21646=EDGE_CURVE('',#16025,#16967,#8088,.T.);
#21647=EDGE_CURVE('',#16967,#15881,#10000,.T.);
#21648=EDGE_CURVE('',#16900,#16023,#11187,.T.);
#21649=EDGE_CURVE('',#16031,#16870,#11188,.T.);
#21650=EDGE_CURVE('',#16880,#16968,#10001,.T.);
#21651=EDGE_CURVE('',#16968,#16898,#11189,.T.);
#21652=EDGE_CURVE('',#16969,#16968,#11190,.T.);
#21653=EDGE_CURVE('',#15876,#16969,#10002,.T.);
#21654=EDGE_CURVE('',#16970,#15875,#8089,.F.);
#21655=EDGE_CURVE('',#16899,#16970,#11191,.T.);
#21656=EDGE_CURVE('',#16969,#16901,#8090,.T.);
#21657=EDGE_CURVE('',#16894,#16970,#11192,.T.);
#21658=EDGE_CURVE('',#16894,#16971,#11193,.T.);
#21659=EDGE_CURVE('',#16899,#16971,#11194,.T.);
#21660=EDGE_CURVE('',#16972,#16892,#11195,.T.);
#21661=EDGE_CURVE('',#16973,#16972,#11196,.T.);
#21662=EDGE_CURVE('',#16145,#16973,#10003,.T.);
#21663=EDGE_CURVE('',#16971,#16144,#8091,.F.);
#21664=EDGE_CURVE('',#16833,#16806,#8092,.T.);
#21665=EDGE_CURVE('',#16810,#16834,#11197,.T.);
#21666=EDGE_CURVE('',#16804,#16722,#11198,.T.);
#21667=EDGE_CURVE('',#16830,#16811,#8093,.T.);
#21668=EDGE_CURVE('',#16823,#16974,#10004,.T.);
#21669=EDGE_CURVE('',#16974,#16825,#11199,.T.);
#21670=EDGE_CURVE('',#16975,#16974,#11200,.T.);
#21671=EDGE_CURVE('',#15856,#16975,#10005,.T.);
#21672=EDGE_CURVE('',#16976,#15855,#8094,.F.);
#21673=EDGE_CURVE('',#16826,#16976,#11201,.T.);
#21674=EDGE_CURVE('',#16977,#16006,#8095,.T.);
#21675=EDGE_CURVE('',#16007,#16978,#8096,.T.);
#21676=EDGE_CURVE('',#16978,#16977,#10006,.T.);
#21677=EDGE_CURVE('',#16008,#16978,#8097,.T.);
#21678=EDGE_CURVE('',#15861,#16977,#8098,.T.);
#21679=EDGE_CURVE('',#16977,#16979,#11202,.T.);
#21680=EDGE_CURVE('',#16979,#15862,#203,.F.);
#21681=EDGE_CURVE('',#16979,#16831,#11203,.T.);
#21682=EDGE_CURVE('',#16979,#15993,#11204,.T.);
#21683=EDGE_CURVE('',#16809,#15993,#11205,.T.);
#21684=EDGE_CURVE('',#16000,#16978,#11206,.T.);
#21685=EDGE_CURVE('',#16975,#16828,#8099,.T.);
#21686=EDGE_CURVE('',#16748,#16976,#11207,.T.);
#21687=EDGE_CURVE('',#16826,#16704,#11208,.T.);
#21688=EDGE_CURVE('',#16800,#16749,#8100,.T.);
#21689=EDGE_CURVE('',#16796,#16801,#11209,.T.);
#21690=EDGE_CURVE('',#16796,#16980,#11210,.T.);
#21691=EDGE_CURVE('',#16747,#16980,#11211,.T.);
#21692=EDGE_CURVE('',#16981,#16794,#11212,.T.);
#21693=EDGE_CURVE('',#16982,#16981,#11213,.T.);
#21694=EDGE_CURVE('',#16165,#16982,#10007,.T.);
#21695=EDGE_CURVE('',#16980,#16164,#8101,.F.);
#21696=EDGE_CURVE('',#16771,#16983,#10008,.T.);
#21697=EDGE_CURVE('',#16983,#16789,#11214,.T.);
#21698=EDGE_CURVE('',#16984,#16983,#11215,.T.);
#21699=EDGE_CURVE('',#15844,#16984,#10009,.T.);
#21700=EDGE_CURVE('',#16985,#15843,#8102,.F.);
#21701=EDGE_CURVE('',#16790,#16985,#11216,.T.);
#21702=EDGE_CURVE('',#16984,#16792,#8103,.T.);
#21703=EDGE_CURVE('',#15842,#16986,#8104,.F.);
#21704=EDGE_CURVE('',#16986,#16985,#11217,.T.);
#21705=EDGE_CURVE('',#16986,#16036,#11218,.T.);
#21706=EDGE_CURVE('',#16790,#16036,#11219,.T.);
#21707=EDGE_CURVE('',#16049,#16987,#8105,.T.);
#21708=EDGE_CURVE('',#16987,#15841,#10010,.T.);
#21709=EDGE_CURVE('',#16785,#16047,#11220,.T.);
#21710=EDGE_CURVE('',#16785,#16988,#11221,.T.);
#21711=EDGE_CURVE('',#16055,#16988,#11222,.T.);
#21712=EDGE_CURVE('',#16989,#16783,#11223,.T.);
#21713=EDGE_CURVE('',#16990,#16989,#11224,.T.);
#21714=EDGE_CURVE('',#16174,#16990,#10011,.T.);
#21715=EDGE_CURVE('',#16988,#16173,#8106,.F.);
#21716=EDGE_CURVE('',#16991,#15833,#10012,.T.);
#21717=EDGE_CURVE('',#16719,#16991,#8107,.T.);
#21718=EDGE_CURVE('',#16701,#16720,#11225,.T.);
#21719=EDGE_CURVE('',#16717,#16632,#11226,.T.);
#21720=EDGE_CURVE('',#16642,#16992,#10013,.T.);
#21721=EDGE_CURVE('',#16992,#16699,#11227,.T.);
#21722=EDGE_CURVE('',#16993,#16992,#11228,.T.);
#21723=EDGE_CURVE('',#15828,#16993,#10014,.T.);
#21724=EDGE_CURVE('',#16994,#15827,#8108,.F.);
#21725=EDGE_CURVE('',#16700,#16994,#11229,.T.);
#21726=EDGE_CURVE('',#16993,#16702,#8109,.T.);
#21727=EDGE_CURVE('',#16695,#16994,#11230,.T.);
#21728=EDGE_CURVE('',#16695,#16995,#11231,.T.);
#21729=EDGE_CURVE('',#16700,#16995,#11232,.T.);
#21730=EDGE_CURVE('',#16996,#16693,#11233,.T.);
#21731=EDGE_CURVE('',#16997,#16996,#11234,.T.);
#21732=EDGE_CURVE('',#16184,#16997,#10015,.T.);
#21733=EDGE_CURVE('',#16995,#16183,#8110,.F.);
#21734=EDGE_CURVE('',#16690,#16657,#8111,.T.);
#21735=EDGE_CURVE('',#16661,#16691,#11235,.T.);
#21736=EDGE_CURVE('',#16655,#16575,#11236,.T.);
#21737=EDGE_CURVE('',#16687,#16662,#8112,.T.);
#21738=EDGE_CURVE('',#16674,#16998,#10016,.T.);
#21739=EDGE_CURVE('',#16998,#16682,#11237,.T.);
#21740=EDGE_CURVE('',#16999,#16998,#11238,.T.);
#21741=EDGE_CURVE('',#15808,#16999,#10017,.T.);
#21742=EDGE_CURVE('',#17000,#15807,#8113,.F.);
#21743=EDGE_CURVE('',#16683,#17000,#11239,.T.);
#21744=EDGE_CURVE('',#17001,#15982,#8114,.T.);
#21745=EDGE_CURVE('',#15983,#17002,#8115,.T.);
#21746=EDGE_CURVE('',#17002,#17001,#10018,.T.);
#21747=EDGE_CURVE('',#15984,#17002,#8116,.T.);
#21748=EDGE_CURVE('',#15813,#17001,#8117,.T.);
#21749=EDGE_CURVE('',#17001,#17003,#11240,.T.);
#21750=EDGE_CURVE('',#17003,#15814,#204,.F.);
#21751=EDGE_CURVE('',#17003,#16688,#11241,.T.);
#21752=EDGE_CURVE('',#17003,#15969,#11242,.T.);
#21753=EDGE_CURVE('',#16660,#15969,#11243,.T.);
#21754=EDGE_CURVE('',#15976,#17002,#11244,.T.);
#21755=EDGE_CURVE('',#16999,#16685,#8118,.T.);
#21756=EDGE_CURVE('',#15806,#17004,#8119,.F.);
#21757=EDGE_CURVE('',#17004,#17000,#11245,.T.);
#21758=EDGE_CURVE('',#17004,#16245,#11246,.T.);
#21759=EDGE_CURVE('',#16683,#16245,#11247,.T.);
#21760=EDGE_CURVE('',#17005,#15805,#10019,.T.);
#21761=EDGE_CURVE('',#16679,#17005,#8120,.T.);
#21762=EDGE_CURVE('',#16628,#16680,#11248,.T.);
#21763=EDGE_CURVE('',#16628,#17006,#11249,.T.);
#21764=EDGE_CURVE('',#16677,#17006,#11250,.T.);
#21765=EDGE_CURVE('',#17007,#16626,#11251,.T.);
#21766=EDGE_CURVE('',#17008,#17007,#11252,.T.);
#21767=EDGE_CURVE('',#16204,#17008,#10020,.T.);
#21768=EDGE_CURVE('',#17006,#16203,#8121,.F.);
#21769=EDGE_CURVE('',#16619,#17009,#10021,.T.);
#21770=EDGE_CURVE('',#17009,#16621,#11253,.T.);
#21771=EDGE_CURVE('',#17010,#17009,#11254,.T.);
#21772=EDGE_CURVE('',#15796,#17010,#10022,.T.);
#21773=EDGE_CURVE('',#17011,#15795,#8122,.F.);
#21774=EDGE_CURVE('',#16622,#17011,#11255,.T.);
#21775=EDGE_CURVE('',#17010,#16624,#8123,.T.);
#21776=EDGE_CURVE('',#16528,#17011,#11256,.T.);
#21777=EDGE_CURVE('',#16622,#16465,#11257,.T.);
#21778=EDGE_CURVE('',#16572,#16529,#8124,.T.);
#21779=EDGE_CURVE('',#16568,#16573,#11258,.T.);
#21780=EDGE_CURVE('',#16568,#17012,#11259,.T.);
#21781=EDGE_CURVE('',#16527,#17012,#11260,.T.);
#21782=EDGE_CURVE('',#17013,#16566,#11261,.T.);
#21783=EDGE_CURVE('',#17014,#17013,#11262,.T.);
#21784=EDGE_CURVE('',#16216,#17014,#10023,.T.);
#21785=EDGE_CURVE('',#17012,#16215,#8125,.F.);
#21786=EDGE_CURVE('',#16563,#16544,#8126,.T.);
#21787=EDGE_CURVE('',#16560,#16564,#11263,.T.);
#21788=EDGE_CURVE('',#16542,#16546,#11264,.T.);
#21789=EDGE_CURVE('',#16556,#17015,#10024,.T.);
#21790=EDGE_CURVE('',#17015,#16558,#11265,.T.);
#21791=EDGE_CURVE('',#17016,#17015,#11266,.T.);
#21792=EDGE_CURVE('',#15780,#17016,#10025,.T.);
#21793=EDGE_CURVE('',#17017,#15779,#8127,.F.);
#21794=EDGE_CURVE('',#16559,#17017,#11267,.T.);
#21795=EDGE_CURVE('',#17016,#16561,#8128,.T.);
#21796=EDGE_CURVE('',#16522,#17017,#11268,.T.);
#21797=EDGE_CURVE('',#16522,#17018,#11269,.T.);
#21798=EDGE_CURVE('',#16559,#17018,#11270,.T.);
#21799=EDGE_CURVE('',#17019,#16520,#11271,.T.);
#21800=EDGE_CURVE('',#17020,#17019,#11272,.T.);
#21801=EDGE_CURVE('',#16228,#17020,#10026,.T.);
#21802=EDGE_CURVE('',#17018,#16227,#8129,.F.);
#21803=EDGE_CURVE('',#16517,#16490,#8130,.T.);
#21804=EDGE_CURVE('',#16494,#16518,#11273,.T.);
#21805=EDGE_CURVE('',#16488,#16404,#11274,.T.);
#21806=EDGE_CURVE('',#16514,#16495,#8131,.T.);
#21807=EDGE_CURVE('',#16507,#17021,#10027,.T.);
#21808=EDGE_CURVE('',#17021,#16509,#11275,.T.);
#21809=EDGE_CURVE('',#17022,#17021,#11276,.T.);
#21810=EDGE_CURVE('',#15955,#17022,#10028,.T.);
#21811=EDGE_CURVE('',#17023,#15954,#8132,.F.);
#21812=EDGE_CURVE('',#16510,#17023,#11277,.T.);
#21813=EDGE_CURVE('',#17024,#15958,#8133,.T.);
#21814=EDGE_CURVE('',#15959,#17025,#8134,.T.);
#21815=EDGE_CURVE('',#17025,#17024,#10029,.T.);
#21816=EDGE_CURVE('',#15960,#17025,#8135,.T.);
#21817=EDGE_CURVE('',#15765,#17024,#8136,.T.);
#21818=EDGE_CURVE('',#17024,#17026,#11278,.T.);
#21819=EDGE_CURVE('',#17026,#15766,#205,.F.);
#21820=EDGE_CURVE('',#17026,#16515,#11279,.T.);
#21821=EDGE_CURVE('',#17026,#15751,#11280,.T.);
#21822=EDGE_CURVE('',#16493,#15751,#11281,.T.);
#21823=EDGE_CURVE('',#15758,#17025,#11282,.T.);
#21824=EDGE_CURVE('',#17022,#16512,#8137,.T.);
#21825=EDGE_CURVE('',#16430,#17023,#11283,.T.);
#21826=EDGE_CURVE('',#16510,#16352,#11284,.T.);
#21827=EDGE_CURVE('',#16450,#16431,#8138,.T.);
#21828=EDGE_CURVE('',#16443,#17027,#10030,.T.);
#21829=EDGE_CURVE('',#17027,#16445,#11285,.T.);
#21830=EDGE_CURVE('',#17028,#17027,#11286,.T.);
#21831=EDGE_CURVE('',#15943,#17028,#10031,.T.);
#21832=EDGE_CURVE('',#17029,#15942,#8139,.F.);
#21833=EDGE_CURVE('',#16446,#17029,#11287,.T.);
#21834=EDGE_CURVE('',#17030,#16401,#8140,.T.);
#21835=EDGE_CURVE('',#16402,#17031,#8141,.T.);
#21836=EDGE_CURVE('',#17031,#17030,#10032,.T.);
#21837=EDGE_CURVE('',#16400,#17032,#8142,.T.);
#21838=EDGE_CURVE('',#17032,#16402,#8143,.T.);
#21839=EDGE_CURVE('',#17032,#17031,#8144,.T.);
#21840=EDGE_CURVE('',#15948,#17030,#8145,.T.);
#21841=EDGE_CURVE('',#17030,#17033,#11288,.T.);
#21842=EDGE_CURVE('',#17033,#15949,#206,.T.);
#21843=EDGE_CURVE('',#17033,#16451,#11289,.T.);
#21844=EDGE_CURVE('',#17034,#16394,#11290,.T.);
#21845=EDGE_CURVE('',#16078,#17034,#8146,.F.);
#21846=EDGE_CURVE('',#17035,#16077,#10033,.T.);
#21847=EDGE_CURVE('',#16398,#17035,#11291,.T.);
#21848=EDGE_CURVE('',#17036,#17031,#11292,.T.);
#21849=EDGE_CURVE('',#17037,#17036,#11293,.T.);
#21850=EDGE_CURVE('',#16076,#17037,#10034,.T.);
#21851=EDGE_CURVE('',#17038,#16075,#8147,.F.);
#21852=EDGE_CURVE('',#17033,#17038,#11294,.T.);
#21853=EDGE_CURVE('',#17028,#16448,#8148,.T.);
#21854=EDGE_CURVE('',#16366,#17029,#11295,.T.);
#21855=EDGE_CURVE('',#16446,#16288,#11296,.T.);
#21856=EDGE_CURVE('',#16391,#16367,#8149,.T.);
#21857=EDGE_CURVE('',#16387,#16392,#11297,.T.);
#21858=EDGE_CURVE('',#16387,#17039,#11298,.T.);
#21859=EDGE_CURVE('',#16365,#17039,#11299,.T.);
#21860=EDGE_CURVE('',#17040,#16385,#11300,.T.);
#21861=EDGE_CURVE('',#17041,#17040,#11301,.T.);
#21862=EDGE_CURVE('',#16088,#17041,#10035,.T.);
#21863=EDGE_CURVE('',#17039,#16087,#8150,.F.);
#21864=EDGE_CURVE('',#17042,#15932,#10036,.T.);
#21865=EDGE_CURVE('',#16382,#17042,#8151,.T.);
#21866=EDGE_CURVE('',#16310,#17043,#10037,.T.);
#21867=EDGE_CURVE('',#17043,#16347,#11302,.T.);
#21868=EDGE_CURVE('',#17044,#17043,#11303,.T.);
#21869=EDGE_CURVE('',#15927,#17044,#10038,.T.);
#21870=EDGE_CURVE('',#17045,#15926,#8152,.F.);
#21871=EDGE_CURVE('',#16348,#17045,#11304,.T.);
#21872=EDGE_CURVE('',#16349,#16383,#11305,.T.);
#21873=EDGE_CURVE('',#16380,#16300,#11306,.T.);
#21874=EDGE_CURVE('',#17044,#16350,#8153,.T.);
#21875=EDGE_CURVE('',#16343,#17045,#11307,.T.);
#21876=EDGE_CURVE('',#16343,#17046,#11308,.T.);
#21877=EDGE_CURVE('',#16348,#17046,#11309,.T.);
#21878=EDGE_CURVE('',#17047,#16341,#11310,.T.);
#21879=EDGE_CURVE('',#17048,#17047,#11311,.T.);
#21880=EDGE_CURVE('',#16100,#17048,#10039,.T.);
#21881=EDGE_CURVE('',#17046,#16099,#8154,.F.);
#21882=EDGE_CURVE('',#17049,#16116,#8155,.T.);
#21883=EDGE_CURVE('',#16115,#17050,#207,.F.);
#21884=EDGE_CURVE('',#17050,#17049,#11312,.T.);
#21885=EDGE_CURVE('',#17051,#17052,#8156,.T.);
#21886=EDGE_CURVE('',#17052,#17053,#10040,.T.);
#21887=EDGE_CURVE('',#17053,#17049,#8157,.T.);
#21888=EDGE_CURVE('',#17049,#17051,#10041,.T.);
#21889=EDGE_CURVE('',#17053,#16116,#8158,.T.);
#21890=EDGE_CURVE('',#17054,#17055,#11313,.T.);
#21891=EDGE_CURVE('',#17055,#17051,#8159,.T.);
#21892=EDGE_CURVE('',#17051,#17056,#11314,.T.);
#21893=EDGE_CURVE('',#17056,#17057,#10042,.T.);
#21894=EDGE_CURVE('',#17057,#17054,#10043,.T.);
#21895=EDGE_CURVE('',#17057,#16953,#8160,.T.);
#21896=EDGE_CURVE('',#16953,#17058,#8161,.T.);
#21897=EDGE_CURVE('',#17058,#17054,#8162,.T.);
#21898=EDGE_CURVE('',#17055,#17052,#8163,.T.);
#21899=EDGE_CURVE('',#16952,#17058,#8164,.T.);
#21900=EDGE_CURVE('',#17053,#17059,#8165,.T.);
#21901=EDGE_CURVE('',#16117,#17059,#8166,.T.);
#21902=EDGE_CURVE('',#17060,#17052,#8167,.T.);
#21903=EDGE_CURVE('',#17059,#17060,#10044,.T.);
#21904=EDGE_CURVE('',#17055,#17061,#8168,.T.);
#21905=EDGE_CURVE('',#17061,#17060,#8169,.T.);
#21906=EDGE_CURVE('',#17061,#17058,#11315,.T.);
#21907=EDGE_CURVE('',#17061,#16956,#8170,.T.);
#21908=EDGE_CURVE('',#17062,#16112,#8171,.T.);
#21909=EDGE_CURVE('',#16111,#17063,#208,.F.);
#21910=EDGE_CURVE('',#17063,#17062,#11316,.T.);
#21911=EDGE_CURVE('',#17064,#15908,#8172,.T.);
#21912=EDGE_CURVE('',#15907,#17065,#209,.F.);
#21913=EDGE_CURVE('',#17065,#17064,#11317,.T.);
#21914=EDGE_CURVE('',#17066,#17067,#8173,.T.);
#21915=EDGE_CURVE('',#17067,#17068,#10045,.T.);
#21916=EDGE_CURVE('',#17068,#17064,#8174,.T.);
#21917=EDGE_CURVE('',#17064,#17066,#10046,.T.);
#21918=EDGE_CURVE('',#17068,#15908,#8175,.T.);
#21919=EDGE_CURVE('',#17069,#17070,#8176,.T.);
#21920=EDGE_CURVE('',#17070,#17071,#8177,.T.);
#21921=EDGE_CURVE('',#17071,#17072,#8178,.T.);
#21922=EDGE_CURVE('',#17072,#17069,#10047,.T.);
#21923=EDGE_CURVE('',#17072,#17073,#11318,.T.);
#21924=EDGE_CURVE('',#17073,#17066,#8179,.T.);
#21925=EDGE_CURVE('',#17066,#17074,#11319,.T.);
#21926=EDGE_CURVE('',#17074,#17069,#10048,.T.);
#21927=EDGE_CURVE('',#17073,#17067,#8180,.T.);
#21928=EDGE_CURVE('',#17075,#17070,#8181,.T.);
#21929=EDGE_CURVE('',#17070,#17076,#10049,.T.);
#21930=EDGE_CURVE('',#17076,#17062,#8182,.T.);
#21931=EDGE_CURVE('',#17062,#17075,#10050,.T.);
#21932=EDGE_CURVE('',#17075,#17071,#8183,.T.);
#21933=EDGE_CURVE('',#17076,#16112,#8184,.T.);
#21934=EDGE_CURVE('',#17077,#17071,#11320,.T.);
#21935=EDGE_CURVE('',#17073,#17077,#8185,.T.);
#21936=EDGE_CURVE('',#17075,#17078,#11321,.T.);
#21937=EDGE_CURVE('',#17077,#17078,#8186,.T.);
#21938=EDGE_CURVE('',#17079,#17063,#11322,.T.);
#21939=EDGE_CURVE('',#15911,#17079,#8187,.F.);
#21940=EDGE_CURVE('',#17078,#15910,#10051,.T.);
#21941=EDGE_CURVE('',#17076,#17080,#8188,.T.);
#21942=EDGE_CURVE('',#17080,#16113,#10052,.T.);
#21943=EDGE_CURVE('',#17074,#17080,#11323,.T.);
#21944=EDGE_CURVE('',#17068,#17081,#8189,.T.);
#21945=EDGE_CURVE('',#17081,#15909,#10053,.T.);
#21946=EDGE_CURVE('',#17081,#17082,#10054,.T.);
#21947=EDGE_CURVE('',#17082,#17078,#8190,.T.);
#21948=EDGE_CURVE('',#17077,#17082,#8191,.T.);
#21949=EDGE_CURVE('',#17082,#17067,#8192,.T.);
#21950=EDGE_CURVE('',#17083,#17065,#11324,.T.);
#21951=EDGE_CURVE('',#16114,#17083,#8193,.F.);
#21952=EDGE_CURVE('',#16955,#17059,#8194,.T.);
#21953=EDGE_CURVE('',#17060,#16956,#8195,.T.);
#21954=EDGE_CURVE('',#16117,#16955,#8196,.T.);
#21955=EDGE_CURVE('',#16954,#16118,#210,.F.);
#21956=EDGE_CURVE('',#17084,#17085,#8197,.T.);
#21957=EDGE_CURVE('',#17085,#17084,#8198,.T.);
#21958=EDGE_CURVE('',#17084,#15957,#8199,.T.);
#21959=EDGE_CURVE('',#17085,#17086,#11325,.T.);
#21960=EDGE_CURVE('',#17087,#17086,#8200,.T.);
#21961=EDGE_CURVE('',#17086,#17087,#8201,.T.);
#21962=EDGE_CURVE('',#16327,#17088,#8202,.T.);
#21963=EDGE_CURVE('',#17088,#15914,#10055,.T.);
#21964=EDGE_CURVE('',#17088,#17089,#10056,.T.);
#21965=EDGE_CURVE('',#17089,#16337,#8203,.T.);
#21966=EDGE_CURVE('',#16336,#17089,#8204,.T.);
#21967=EDGE_CURVE('',#17089,#16326,#8205,.T.);
#21968=EDGE_CURVE('',#16274,#17090,#8206,.T.);
#21969=EDGE_CURVE('',#17090,#15919,#10057,.T.);
#21970=EDGE_CURVE('',#17090,#17091,#10058,.T.);
#21971=EDGE_CURVE('',#17091,#16284,#8207,.T.);
#21972=EDGE_CURVE('',#16283,#17091,#8208,.T.);
#21973=EDGE_CURVE('',#17091,#16273,#8209,.T.);
#21974=EDGE_CURVE('',#16338,#16271,#11326,.T.);
#21975=EDGE_CURVE('',#17092,#16322,#11327,.T.);
#21976=EDGE_CURVE('',#17092,#16271,#11328,.T.);
#21977=EDGE_CURVE('',#17079,#16324,#11329,.T.);
#21978=EDGE_CURVE('',#17093,#17063,#11330,.T.);
#21979=EDGE_CURVE('',#17093,#16324,#11331,.T.);
#21980=EDGE_CURVE('',#16239,#17087,#8210,.T.);
#21981=EDGE_CURVE('',#15906,#17094,#8211,.F.);
#21982=EDGE_CURVE('',#17094,#17065,#11332,.T.);
#21983=EDGE_CURVE('',#17094,#17050,#11333,.T.);
#21984=EDGE_CURVE('',#17083,#17050,#11334,.T.);
#21985=EDGE_CURVE('',#16110,#17093,#8212,.F.);
#21986=EDGE_CURVE('',#16106,#17092,#8213,.F.);
#21987=EDGE_CURVE('',#16342,#17095,#11335,.T.);
#21988=EDGE_CURVE('',#17095,#17047,#10059,.T.);
#21989=EDGE_CURVE('',#16285,#16312,#11336,.T.);
#21990=EDGE_CURVE('',#16344,#16269,#11337,.T.);
#21991=EDGE_CURVE('',#17048,#16345,#8214,.T.);
#21992=EDGE_CURVE('',#17096,#16257,#11338,.T.);
#21993=EDGE_CURVE('',#15933,#17096,#8215,.F.);
#21994=EDGE_CURVE('',#16261,#17042,#11339,.T.);
#21995=EDGE_CURVE('',#16386,#17097,#11340,.T.);
#21996=EDGE_CURVE('',#17097,#17040,#10060,.T.);
#21997=EDGE_CURVE('',#17096,#16369,#11341,.T.);
#21998=EDGE_CURVE('',#16388,#16257,#11342,.T.);
#21999=EDGE_CURVE('',#17041,#16389,#8216,.T.);
#22000=EDGE_CURVE('',#17032,#17098,#11343,.T.);
#22001=EDGE_CURVE('',#17098,#17036,#10061,.T.);
#22002=EDGE_CURVE('',#16447,#16394,#11344,.T.);
#22003=EDGE_CURVE('',#17034,#16433,#11345,.T.);
#22004=EDGE_CURVE('',#17037,#17035,#8217,.T.);
#22005=EDGE_CURVE('',#16429,#17038,#11346,.T.);
#22006=EDGE_CURVE('',#16511,#15744,#11347,.T.);
#22007=EDGE_CURVE('',#15760,#16497,#11348,.T.);
#22008=EDGE_CURVE('',#15759,#15763,#8218,.T.);
#22009=EDGE_CURVE('',#16521,#17099,#11349,.T.);
#22010=EDGE_CURVE('',#17099,#17019,#10062,.T.);
#22011=EDGE_CURVE('',#16489,#16477,#11350,.T.);
#22012=EDGE_CURVE('',#16523,#16416,#11351,.T.);
#22013=EDGE_CURVE('',#17020,#16524,#8219,.T.);
#22014=EDGE_CURVE('',#16567,#17100,#11352,.T.);
#22015=EDGE_CURVE('',#17100,#17013,#10063,.T.);
#22016=EDGE_CURVE('',#16543,#16531,#11353,.T.);
#22017=EDGE_CURVE('',#16569,#16453,#11354,.T.);
#22018=EDGE_CURVE('',#17014,#16570,#8220,.T.);
#22019=EDGE_CURVE('',#16627,#17101,#11355,.T.);
#22020=EDGE_CURVE('',#17101,#17007,#10064,.T.);
#22021=EDGE_CURVE('',#16623,#16599,#11356,.T.);
#22022=EDGE_CURVE('',#16629,#16609,#11357,.T.);
#22023=EDGE_CURVE('',#17008,#16630,#8221,.T.);
#22024=EDGE_CURVE('',#16249,#17005,#11358,.T.);
#22025=EDGE_CURVE('',#16684,#15962,#11359,.T.);
#22026=EDGE_CURVE('',#15978,#16664,#11360,.T.);
#22027=EDGE_CURVE('',#15977,#15981,#8222,.T.);
#22028=EDGE_CURVE('',#16694,#17102,#11361,.T.);
#22029=EDGE_CURVE('',#17102,#16996,#10065,.T.);
#22030=EDGE_CURVE('',#16656,#16644,#11362,.T.);
#22031=EDGE_CURVE('',#16696,#16587,#11363,.T.);
#22032=EDGE_CURVE('',#16997,#16697,#8223,.T.);
#22033=EDGE_CURVE('',#17103,#16060,#11364,.T.);
#22034=EDGE_CURVE('',#15834,#17103,#8224,.F.);
#22035=EDGE_CURVE('',#16064,#16991,#11365,.T.);
#22036=EDGE_CURVE('',#16784,#17104,#11366,.T.);
#22037=EDGE_CURVE('',#17104,#16989,#10066,.T.);
#22038=EDGE_CURVE('',#17103,#16773,#11367,.T.);
#22039=EDGE_CURVE('',#16786,#16060,#11368,.T.);
#22040=EDGE_CURVE('',#16990,#16787,#8225,.T.);
#22041=EDGE_CURVE('',#16045,#16987,#11369,.T.);
#22042=EDGE_CURVE('',#16795,#17105,#11370,.T.);
#22043=EDGE_CURVE('',#17105,#16981,#10067,.T.);
#22044=EDGE_CURVE('',#16791,#16751,#11371,.T.);
#22045=EDGE_CURVE('',#16797,#16761,#11372,.T.);
#22046=EDGE_CURVE('',#16982,#16798,#8226,.T.);
#22047=EDGE_CURVE('',#16827,#15986,#11373,.T.);
#22048=EDGE_CURVE('',#16002,#16813,#11374,.T.);
#22049=EDGE_CURVE('',#16001,#16005,#8227,.T.);
#22050=EDGE_CURVE('',#16893,#17106,#11375,.T.);
#22051=EDGE_CURVE('',#17106,#16972,#10068,.T.);
#22052=EDGE_CURVE('',#16805,#16882,#11376,.T.);
#22053=EDGE_CURVE('',#16895,#16734,#11377,.T.);
#22054=EDGE_CURVE('',#16973,#16896,#8228,.T.);
#22055=EDGE_CURVE('',#17107,#16012,#11378,.T.);
#22056=EDGE_CURVE('',#15882,#17107,#8229,.F.);
#22057=EDGE_CURVE('',#16021,#16967,#11379,.T.);
#22058=EDGE_CURVE('',#16941,#17108,#11380,.T.);
#22059=EDGE_CURVE('',#17108,#16965,#10069,.T.);
#22060=EDGE_CURVE('',#17107,#16930,#11381,.T.);
#22061=EDGE_CURVE('',#16943,#16012,#11382,.T.);
#22062=EDGE_CURVE('',#16966,#16944,#8230,.T.);
#22063=EDGE_CURVE('',#16909,#17109,#11383,.T.);
#22064=EDGE_CURVE('',#17109,#16959,#10070,.T.);
#22065=EDGE_CURVE('',#16905,#16848,#11384,.T.);
#22066=EDGE_CURVE('',#16911,#16858,#11385,.T.);
#22067=EDGE_CURVE('',#16960,#16912,#8231,.T.);
#22068=EDGE_CURVE('',#16120,#16918,#10071,.T.);
#22069=EDGE_CURVE('',#17110,#16957,#11386,.T.);
#22070=EDGE_CURVE('',#16919,#17110,#11387,.T.);
#22071=EDGE_CURVE('',#17111,#16119,#8232,.F.);
#22072=EDGE_CURVE('',#17112,#17111,#11388,.T.);
#22073=EDGE_CURVE('',#15902,#17112,#8233,.F.);
#22074=EDGE_CURVE('',#17112,#16951,#11389,.T.);
#22075=EDGE_CURVE('',#16954,#17111,#11390,.T.);
#22076=EDGE_CURVE('',#17110,#17113,#10072,.T.);
#22077=EDGE_CURVE('',#17113,#16920,#11391,.T.);
#22078=EDGE_CURVE('',#16915,#17113,#8234,.T.);
#22079=EDGE_CURVE('',#16853,#17109,#8235,.T.);
#22080=EDGE_CURVE('',#16935,#17108,#8236,.T.);
#22081=EDGE_CURVE('',#16887,#17106,#8237,.T.);
#22082=EDGE_CURVE('',#16756,#17105,#8238,.T.);
#22083=EDGE_CURVE('',#16778,#17104,#8239,.T.);
#22084=EDGE_CURVE('',#16649,#17102,#8240,.T.);
#22085=EDGE_CURVE('',#16604,#17101,#8241,.T.);
#22086=EDGE_CURVE('',#16536,#17100,#8242,.T.);
#22087=EDGE_CURVE('',#16482,#17099,#8243,.T.);
#22088=EDGE_CURVE('',#16399,#17098,#8244,.T.);
#22089=EDGE_CURVE('',#16374,#17097,#8245,.T.);
#22090=EDGE_CURVE('',#16317,#17095,#8246,.T.);
#22091=EDGE_CURVE('',#17056,#16948,#11392,.T.);
#26333=ORIENTED_EDGE('',*,*,#19678,.T.);
#26334=ORIENTED_EDGE('',*,*,#19679,.T.);
#26335=ORIENTED_EDGE('',*,*,#19680,.T.);
#26336=ORIENTED_EDGE('',*,*,#19681,.T.);
#26337=ORIENTED_EDGE('',*,*,#19682,.T.);
#26338=ORIENTED_EDGE('',*,*,#19683,.T.);
#26339=ORIENTED_EDGE('',*,*,#19684,.T.);
#26340=ORIENTED_EDGE('',*,*,#19685,.T.);
#26341=ORIENTED_EDGE('',*,*,#19684,.F.);
#26342=ORIENTED_EDGE('',*,*,#19686,.T.);
#26343=ORIENTED_EDGE('',*,*,#19678,.F.);
#26344=ORIENTED_EDGE('',*,*,#19687,.T.);
#26345=ORIENTED_EDGE('',*,*,#19688,.T.);
#26346=ORIENTED_EDGE('',*,*,#19689,.T.);
#26347=ORIENTED_EDGE('',*,*,#19690,.T.);
#26348=ORIENTED_EDGE('',*,*,#19691,.T.);
#26349=ORIENTED_EDGE('',*,*,#19692,.T.);
#26350=ORIENTED_EDGE('',*,*,#19693,.T.);
#26351=ORIENTED_EDGE('',*,*,#19694,.T.);
#26352=ORIENTED_EDGE('',*,*,#19695,.T.);
#26353=ORIENTED_EDGE('',*,*,#19696,.T.);
#26354=ORIENTED_EDGE('',*,*,#19697,.T.);
#26355=ORIENTED_EDGE('',*,*,#19698,.T.);
#26356=ORIENTED_EDGE('',*,*,#19694,.F.);
#26357=ORIENTED_EDGE('',*,*,#19699,.T.);
#26358=ORIENTED_EDGE('',*,*,#19700,.T.);
#26359=ORIENTED_EDGE('',*,*,#19701,.T.);
#26360=ORIENTED_EDGE('',*,*,#19702,.T.);
#26361=ORIENTED_EDGE('',*,*,#19699,.F.);
#26362=ORIENTED_EDGE('',*,*,#19703,.T.);
#26363=ORIENTED_EDGE('',*,*,#19692,.F.);
#26364=ORIENTED_EDGE('',*,*,#19701,.F.);
#26365=ORIENTED_EDGE('',*,*,#19704,.T.);
#26366=ORIENTED_EDGE('',*,*,#19687,.F.);
#26367=ORIENTED_EDGE('',*,*,#19696,.F.);
#26368=ORIENTED_EDGE('',*,*,#19705,.T.);
#26369=ORIENTED_EDGE('',*,*,#19682,.F.);
#26370=ORIENTED_EDGE('',*,*,#19697,.F.);
#26371=ORIENTED_EDGE('',*,*,#19685,.F.);
#26372=ORIENTED_EDGE('',*,*,#19681,.F.);
#26373=ORIENTED_EDGE('',*,*,#19706,.F.);
#26374=ORIENTED_EDGE('',*,*,#19707,.F.);
#26375=ORIENTED_EDGE('',*,*,#19708,.F.);
#26376=ORIENTED_EDGE('',*,*,#19709,.F.);
#26377=ORIENTED_EDGE('',*,*,#19710,.F.);
#26378=ORIENTED_EDGE('',*,*,#19711,.F.);
#26379=ORIENTED_EDGE('',*,*,#19679,.F.);
#26380=ORIENTED_EDGE('',*,*,#19712,.F.);
#26381=ORIENTED_EDGE('',*,*,#19713,.F.);
#26382=ORIENTED_EDGE('',*,*,#19714,.F.);
#26383=ORIENTED_EDGE('',*,*,#19715,.T.);
#26384=ORIENTED_EDGE('',*,*,#19716,.F.);
#26385=ORIENTED_EDGE('',*,*,#19717,.T.);
#26386=ORIENTED_EDGE('',*,*,#19718,.F.);
#26387=ORIENTED_EDGE('',*,*,#19719,.T.);
#26388=ORIENTED_EDGE('',*,*,#19720,.F.);
#26389=ORIENTED_EDGE('',*,*,#19721,.T.);
#26390=ORIENTED_EDGE('',*,*,#19722,.F.);
#26391=ORIENTED_EDGE('',*,*,#19723,.F.);
#26392=ORIENTED_EDGE('',*,*,#19724,.F.);
#26393=ORIENTED_EDGE('',*,*,#19725,.F.);
#26394=ORIENTED_EDGE('',*,*,#19726,.F.);
#26395=ORIENTED_EDGE('',*,*,#19727,.T.);
#26396=ORIENTED_EDGE('',*,*,#19728,.F.);
#26397=ORIENTED_EDGE('',*,*,#19729,.T.);
#26398=ORIENTED_EDGE('',*,*,#19730,.F.);
#26399=ORIENTED_EDGE('',*,*,#19731,.T.);
#26400=ORIENTED_EDGE('',*,*,#19732,.F.);
#26401=ORIENTED_EDGE('',*,*,#19733,.T.);
#26402=ORIENTED_EDGE('',*,*,#19734,.F.);
#26403=ORIENTED_EDGE('',*,*,#19735,.F.);
#26404=ORIENTED_EDGE('',*,*,#19736,.F.);
#26405=ORIENTED_EDGE('',*,*,#19737,.F.);
#26406=ORIENTED_EDGE('',*,*,#19738,.F.);
#26407=ORIENTED_EDGE('',*,*,#19739,.T.);
#26408=ORIENTED_EDGE('',*,*,#19740,.F.);
#26409=ORIENTED_EDGE('',*,*,#19741,.T.);
#26410=ORIENTED_EDGE('',*,*,#19742,.F.);
#26411=ORIENTED_EDGE('',*,*,#19743,.T.);
#26412=ORIENTED_EDGE('',*,*,#19744,.F.);
#26413=ORIENTED_EDGE('',*,*,#19745,.T.);
#26414=ORIENTED_EDGE('',*,*,#19746,.F.);
#26415=ORIENTED_EDGE('',*,*,#19747,.F.);
#26416=ORIENTED_EDGE('',*,*,#19748,.F.);
#26417=ORIENTED_EDGE('',*,*,#19749,.F.);
#26418=ORIENTED_EDGE('',*,*,#19750,.F.);
#26419=ORIENTED_EDGE('',*,*,#19751,.T.);
#26420=ORIENTED_EDGE('',*,*,#19752,.F.);
#26421=ORIENTED_EDGE('',*,*,#19753,.T.);
#26422=ORIENTED_EDGE('',*,*,#19754,.F.);
#26423=ORIENTED_EDGE('',*,*,#19755,.T.);
#26424=ORIENTED_EDGE('',*,*,#19756,.F.);
#26425=ORIENTED_EDGE('',*,*,#19757,.T.);
#26426=ORIENTED_EDGE('',*,*,#19758,.F.);
#26427=ORIENTED_EDGE('',*,*,#19759,.F.);
#26428=ORIENTED_EDGE('',*,*,#19760,.F.);
#26429=ORIENTED_EDGE('',*,*,#19761,.F.);
#26430=ORIENTED_EDGE('',*,*,#19762,.F.);
#26431=ORIENTED_EDGE('',*,*,#19763,.T.);
#26432=ORIENTED_EDGE('',*,*,#19764,.F.);
#26433=ORIENTED_EDGE('',*,*,#19765,.T.);
#26434=ORIENTED_EDGE('',*,*,#19766,.F.);
#26435=ORIENTED_EDGE('',*,*,#19767,.T.);
#26436=ORIENTED_EDGE('',*,*,#19768,.F.);
#26437=ORIENTED_EDGE('',*,*,#19769,.T.);
#26438=ORIENTED_EDGE('',*,*,#19770,.F.);
#26439=ORIENTED_EDGE('',*,*,#19771,.F.);
#26440=ORIENTED_EDGE('',*,*,#19772,.F.);
#26441=ORIENTED_EDGE('',*,*,#19773,.F.);
#26442=ORIENTED_EDGE('',*,*,#19774,.F.);
#26443=ORIENTED_EDGE('',*,*,#19775,.T.);
#26444=ORIENTED_EDGE('',*,*,#19776,.F.);
#26445=ORIENTED_EDGE('',*,*,#19777,.T.);
#26446=ORIENTED_EDGE('',*,*,#19778,.F.);
#26447=ORIENTED_EDGE('',*,*,#19779,.T.);
#26448=ORIENTED_EDGE('',*,*,#19780,.F.);
#26449=ORIENTED_EDGE('',*,*,#19781,.T.);
#26450=ORIENTED_EDGE('',*,*,#19782,.F.);
#26451=ORIENTED_EDGE('',*,*,#19783,.F.);
#26452=ORIENTED_EDGE('',*,*,#19784,.F.);
#26453=ORIENTED_EDGE('',*,*,#19785,.F.);
#26454=ORIENTED_EDGE('',*,*,#19786,.F.);
#26455=ORIENTED_EDGE('',*,*,#19787,.F.);
#26456=ORIENTED_EDGE('',*,*,#19788,.F.);
#26457=ORIENTED_EDGE('',*,*,#19789,.T.);
#26458=ORIENTED_EDGE('',*,*,#19790,.F.);
#26459=ORIENTED_EDGE('',*,*,#19791,.T.);
#26460=ORIENTED_EDGE('',*,*,#19792,.F.);
#26461=ORIENTED_EDGE('',*,*,#19793,.T.);
#26462=ORIENTED_EDGE('',*,*,#19794,.F.);
#26463=ORIENTED_EDGE('',*,*,#19795,.F.);
#26464=ORIENTED_EDGE('',*,*,#19796,.F.);
#26465=ORIENTED_EDGE('',*,*,#19797,.F.);
#26466=ORIENTED_EDGE('',*,*,#19798,.F.);
#26467=ORIENTED_EDGE('',*,*,#19799,.T.);
#26468=ORIENTED_EDGE('',*,*,#19800,.F.);
#26469=ORIENTED_EDGE('',*,*,#19801,.T.);
#26470=ORIENTED_EDGE('',*,*,#19802,.F.);
#26471=ORIENTED_EDGE('',*,*,#19803,.T.);
#26472=ORIENTED_EDGE('',*,*,#19804,.F.);
#26473=ORIENTED_EDGE('',*,*,#19805,.T.);
#26474=ORIENTED_EDGE('',*,*,#19806,.F.);
#26475=ORIENTED_EDGE('',*,*,#19807,.F.);
#26476=ORIENTED_EDGE('',*,*,#19808,.F.);
#26477=ORIENTED_EDGE('',*,*,#19809,.F.);
#26478=ORIENTED_EDGE('',*,*,#19810,.F.);
#26479=ORIENTED_EDGE('',*,*,#19811,.T.);
#26480=ORIENTED_EDGE('',*,*,#19812,.F.);
#26481=ORIENTED_EDGE('',*,*,#19813,.T.);
#26482=ORIENTED_EDGE('',*,*,#19814,.F.);
#26483=ORIENTED_EDGE('',*,*,#19815,.T.);
#26484=ORIENTED_EDGE('',*,*,#19816,.F.);
#26485=ORIENTED_EDGE('',*,*,#19817,.T.);
#26486=ORIENTED_EDGE('',*,*,#19818,.F.);
#26487=ORIENTED_EDGE('',*,*,#19819,.F.);
#26488=ORIENTED_EDGE('',*,*,#19820,.F.);
#26489=ORIENTED_EDGE('',*,*,#19821,.F.);
#26490=ORIENTED_EDGE('',*,*,#19822,.F.);
#26491=ORIENTED_EDGE('',*,*,#19823,.T.);
#26492=ORIENTED_EDGE('',*,*,#19824,.F.);
#26493=ORIENTED_EDGE('',*,*,#19825,.T.);
#26494=ORIENTED_EDGE('',*,*,#19826,.F.);
#26495=ORIENTED_EDGE('',*,*,#19827,.F.);
#26496=ORIENTED_EDGE('',*,*,#19828,.F.);
#26497=ORIENTED_EDGE('',*,*,#19829,.T.);
#26498=ORIENTED_EDGE('',*,*,#19830,.F.);
#26499=ORIENTED_EDGE('',*,*,#19831,.F.);
#26500=ORIENTED_EDGE('',*,*,#19832,.F.);
#26501=ORIENTED_EDGE('',*,*,#19833,.F.);
#26502=ORIENTED_EDGE('',*,*,#19834,.F.);
#26503=ORIENTED_EDGE('',*,*,#19835,.T.);
#26504=ORIENTED_EDGE('',*,*,#19836,.F.);
#26505=ORIENTED_EDGE('',*,*,#19837,.T.);
#26506=ORIENTED_EDGE('',*,*,#19838,.F.);
#26507=ORIENTED_EDGE('',*,*,#19839,.T.);
#26508=ORIENTED_EDGE('',*,*,#19840,.F.);
#26509=ORIENTED_EDGE('',*,*,#19841,.T.);
#26510=ORIENTED_EDGE('',*,*,#19842,.F.);
#26511=ORIENTED_EDGE('',*,*,#19843,.F.);
#26512=ORIENTED_EDGE('',*,*,#19844,.F.);
#26513=ORIENTED_EDGE('',*,*,#19845,.F.);
#26514=ORIENTED_EDGE('',*,*,#19846,.F.);
#26515=ORIENTED_EDGE('',*,*,#19847,.T.);
#26516=ORIENTED_EDGE('',*,*,#19848,.F.);
#26517=ORIENTED_EDGE('',*,*,#19849,.T.);
#26518=ORIENTED_EDGE('',*,*,#19850,.F.);
#26519=ORIENTED_EDGE('',*,*,#19851,.F.);
#26520=ORIENTED_EDGE('',*,*,#19852,.F.);
#26521=ORIENTED_EDGE('',*,*,#19853,.T.);
#26522=ORIENTED_EDGE('',*,*,#19854,.F.);
#26523=ORIENTED_EDGE('',*,*,#19855,.F.);
#26524=ORIENTED_EDGE('',*,*,#19856,.F.);
#26525=ORIENTED_EDGE('',*,*,#19857,.F.);
#26526=ORIENTED_EDGE('',*,*,#19858,.T.);
#26527=ORIENTED_EDGE('',*,*,#19859,.F.);
#26528=ORIENTED_EDGE('',*,*,#19860,.F.);
#26529=ORIENTED_EDGE('',*,*,#19861,.F.);
#26530=ORIENTED_EDGE('',*,*,#19862,.F.);
#26531=ORIENTED_EDGE('',*,*,#19863,.T.);
#26532=ORIENTED_EDGE('',*,*,#19864,.F.);
#26533=ORIENTED_EDGE('',*,*,#19865,.F.);
#26534=ORIENTED_EDGE('',*,*,#19866,.F.);
#26535=ORIENTED_EDGE('',*,*,#19867,.F.);
#26536=ORIENTED_EDGE('',*,*,#19868,.T.);
#26537=ORIENTED_EDGE('',*,*,#19869,.F.);
#26538=ORIENTED_EDGE('',*,*,#19870,.F.);
#26539=ORIENTED_EDGE('',*,*,#19871,.F.);
#26540=ORIENTED_EDGE('',*,*,#19872,.F.);
#26541=ORIENTED_EDGE('',*,*,#19873,.F.);
#26542=ORIENTED_EDGE('',*,*,#19874,.T.);
#26543=ORIENTED_EDGE('',*,*,#19875,.F.);
#26544=ORIENTED_EDGE('',*,*,#19876,.T.);
#26545=ORIENTED_EDGE('',*,*,#19877,.F.);
#26546=ORIENTED_EDGE('',*,*,#19878,.T.);
#26547=ORIENTED_EDGE('',*,*,#19879,.F.);
#26548=ORIENTED_EDGE('',*,*,#19880,.T.);
#26549=ORIENTED_EDGE('',*,*,#19881,.F.);
#26550=ORIENTED_EDGE('',*,*,#19882,.F.);
#26551=ORIENTED_EDGE('',*,*,#19883,.F.);
#26552=ORIENTED_EDGE('',*,*,#19884,.F.);
#26553=ORIENTED_EDGE('',*,*,#19885,.F.);
#26554=ORIENTED_EDGE('',*,*,#19886,.T.);
#26555=ORIENTED_EDGE('',*,*,#19887,.F.);
#26556=ORIENTED_EDGE('',*,*,#19888,.T.);
#26557=ORIENTED_EDGE('',*,*,#19889,.F.);
#26558=ORIENTED_EDGE('',*,*,#19890,.T.);
#26559=ORIENTED_EDGE('',*,*,#19891,.F.);
#26560=ORIENTED_EDGE('',*,*,#19892,.T.);
#26561=ORIENTED_EDGE('',*,*,#19893,.F.);
#26562=ORIENTED_EDGE('',*,*,#19894,.F.);
#26563=ORIENTED_EDGE('',*,*,#19895,.F.);
#26564=ORIENTED_EDGE('',*,*,#19896,.F.);
#26565=ORIENTED_EDGE('',*,*,#19897,.F.);
#26566=ORIENTED_EDGE('',*,*,#19898,.T.);
#26567=ORIENTED_EDGE('',*,*,#19899,.F.);
#26568=ORIENTED_EDGE('',*,*,#19900,.T.);
#26569=ORIENTED_EDGE('',*,*,#19901,.F.);
#26570=ORIENTED_EDGE('',*,*,#19902,.T.);
#26571=ORIENTED_EDGE('',*,*,#19903,.F.);
#26572=ORIENTED_EDGE('',*,*,#19904,.T.);
#26573=ORIENTED_EDGE('',*,*,#19905,.F.);
#26574=ORIENTED_EDGE('',*,*,#19686,.F.);
#26575=ORIENTED_EDGE('',*,*,#19906,.T.);
#26576=ORIENTED_EDGE('',*,*,#19907,.F.);
#26577=ORIENTED_EDGE('',*,*,#19712,.T.);
#26578=ORIENTED_EDGE('',*,*,#19683,.F.);
#26579=ORIENTED_EDGE('',*,*,#19908,.F.);
#26580=ORIENTED_EDGE('',*,*,#19909,.F.);
#26581=ORIENTED_EDGE('',*,*,#19906,.F.);
#26582=ORIENTED_EDGE('',*,*,#19705,.F.);
#26583=ORIENTED_EDGE('',*,*,#19910,.T.);
#26584=ORIENTED_EDGE('',*,*,#19911,.T.);
#26585=ORIENTED_EDGE('',*,*,#19908,.T.);
#26586=ORIENTED_EDGE('',*,*,#19695,.F.);
#26587=ORIENTED_EDGE('',*,*,#19693,.F.);
#26588=ORIENTED_EDGE('',*,*,#19912,.F.);
#26589=ORIENTED_EDGE('',*,*,#19910,.F.);
#26590=ORIENTED_EDGE('',*,*,#19913,.T.);
#26591=ORIENTED_EDGE('',*,*,#19759,.T.);
#26592=ORIENTED_EDGE('',*,*,#19914,.T.);
#26593=ORIENTED_EDGE('',*,*,#19915,.T.);
#26594=ORIENTED_EDGE('',*,*,#19916,.T.);
#26595=ORIENTED_EDGE('',*,*,#19917,.T.);
#26596=ORIENTED_EDGE('',*,*,#19918,.T.);
#26597=ORIENTED_EDGE('',*,*,#19919,.T.);
#26598=ORIENTED_EDGE('',*,*,#19918,.F.);
#26599=ORIENTED_EDGE('',*,*,#19920,.T.);
#26600=ORIENTED_EDGE('',*,*,#19913,.F.);
#26601=ORIENTED_EDGE('',*,*,#19921,.T.);
#26602=ORIENTED_EDGE('',*,*,#19922,.T.);
#26603=ORIENTED_EDGE('',*,*,#19923,.T.);
#26604=ORIENTED_EDGE('',*,*,#19924,.T.);
#26605=ORIENTED_EDGE('',*,*,#19925,.T.);
#26606=ORIENTED_EDGE('',*,*,#19926,.T.);
#26607=ORIENTED_EDGE('',*,*,#19927,.T.);
#26608=ORIENTED_EDGE('',*,*,#19928,.T.);
#26609=ORIENTED_EDGE('',*,*,#19929,.T.);
#26610=ORIENTED_EDGE('',*,*,#19930,.T.);
#26611=ORIENTED_EDGE('',*,*,#19931,.T.);
#26612=ORIENTED_EDGE('',*,*,#19932,.T.);
#26613=ORIENTED_EDGE('',*,*,#19928,.F.);
#26614=ORIENTED_EDGE('',*,*,#19933,.T.);
#26615=ORIENTED_EDGE('',*,*,#19934,.T.);
#26616=ORIENTED_EDGE('',*,*,#19935,.T.);
#26617=ORIENTED_EDGE('',*,*,#19936,.T.);
#26618=ORIENTED_EDGE('',*,*,#19933,.F.);
#26619=ORIENTED_EDGE('',*,*,#19937,.T.);
#26620=ORIENTED_EDGE('',*,*,#19926,.F.);
#26621=ORIENTED_EDGE('',*,*,#19935,.F.);
#26622=ORIENTED_EDGE('',*,*,#19938,.T.);
#26623=ORIENTED_EDGE('',*,*,#19921,.F.);
#26624=ORIENTED_EDGE('',*,*,#19930,.F.);
#26625=ORIENTED_EDGE('',*,*,#19939,.T.);
#26626=ORIENTED_EDGE('',*,*,#19916,.F.);
#26627=ORIENTED_EDGE('',*,*,#19931,.F.);
#26628=ORIENTED_EDGE('',*,*,#19919,.F.);
#26629=ORIENTED_EDGE('',*,*,#19915,.F.);
#26630=ORIENTED_EDGE('',*,*,#19940,.F.);
#26631=ORIENTED_EDGE('',*,*,#19941,.F.);
#26632=ORIENTED_EDGE('',*,*,#19942,.F.);
#26633=ORIENTED_EDGE('',*,*,#19943,.F.);
#26634=ORIENTED_EDGE('',*,*,#19944,.F.);
#26635=ORIENTED_EDGE('',*,*,#19920,.F.);
#26636=ORIENTED_EDGE('',*,*,#19945,.T.);
#26637=ORIENTED_EDGE('',*,*,#19946,.F.);
#26638=ORIENTED_EDGE('',*,*,#19760,.T.);
#26639=ORIENTED_EDGE('',*,*,#19917,.F.);
#26640=ORIENTED_EDGE('',*,*,#19947,.F.);
#26641=ORIENTED_EDGE('',*,*,#19948,.F.);
#26642=ORIENTED_EDGE('',*,*,#19945,.F.);
#26643=ORIENTED_EDGE('',*,*,#19939,.F.);
#26644=ORIENTED_EDGE('',*,*,#19949,.T.);
#26645=ORIENTED_EDGE('',*,*,#19950,.T.);
#26646=ORIENTED_EDGE('',*,*,#19947,.T.);
#26647=ORIENTED_EDGE('',*,*,#19929,.F.);
#26648=ORIENTED_EDGE('',*,*,#19927,.F.);
#26649=ORIENTED_EDGE('',*,*,#19951,.F.);
#26650=ORIENTED_EDGE('',*,*,#19949,.F.);
#26651=ORIENTED_EDGE('',*,*,#19952,.T.);
#26652=ORIENTED_EDGE('',*,*,#19807,.T.);
#26653=ORIENTED_EDGE('',*,*,#19953,.T.);
#26654=ORIENTED_EDGE('',*,*,#19954,.T.);
#26655=ORIENTED_EDGE('',*,*,#19955,.T.);
#26656=ORIENTED_EDGE('',*,*,#19956,.T.);
#26657=ORIENTED_EDGE('',*,*,#19957,.T.);
#26658=ORIENTED_EDGE('',*,*,#19958,.T.);
#26659=ORIENTED_EDGE('',*,*,#19957,.F.);
#26660=ORIENTED_EDGE('',*,*,#19959,.T.);
#26661=ORIENTED_EDGE('',*,*,#19952,.F.);
#26662=ORIENTED_EDGE('',*,*,#19960,.T.);
#26663=ORIENTED_EDGE('',*,*,#19961,.T.);
#26664=ORIENTED_EDGE('',*,*,#19962,.T.);
#26665=ORIENTED_EDGE('',*,*,#19963,.T.);
#26666=ORIENTED_EDGE('',*,*,#19964,.T.);
#26667=ORIENTED_EDGE('',*,*,#19965,.T.);
#26668=ORIENTED_EDGE('',*,*,#19966,.T.);
#26669=ORIENTED_EDGE('',*,*,#19967,.T.);
#26670=ORIENTED_EDGE('',*,*,#19968,.T.);
#26671=ORIENTED_EDGE('',*,*,#19969,.T.);
#26672=ORIENTED_EDGE('',*,*,#19970,.T.);
#26673=ORIENTED_EDGE('',*,*,#19971,.T.);
#26674=ORIENTED_EDGE('',*,*,#19967,.F.);
#26675=ORIENTED_EDGE('',*,*,#19972,.T.);
#26676=ORIENTED_EDGE('',*,*,#19973,.T.);
#26677=ORIENTED_EDGE('',*,*,#19974,.T.);
#26678=ORIENTED_EDGE('',*,*,#19975,.T.);
#26679=ORIENTED_EDGE('',*,*,#19972,.F.);
#26680=ORIENTED_EDGE('',*,*,#19976,.T.);
#26681=ORIENTED_EDGE('',*,*,#19965,.F.);
#26682=ORIENTED_EDGE('',*,*,#19974,.F.);
#26683=ORIENTED_EDGE('',*,*,#19977,.T.);
#26684=ORIENTED_EDGE('',*,*,#19960,.F.);
#26685=ORIENTED_EDGE('',*,*,#19969,.F.);
#26686=ORIENTED_EDGE('',*,*,#19978,.T.);
#26687=ORIENTED_EDGE('',*,*,#19955,.F.);
#26688=ORIENTED_EDGE('',*,*,#19970,.F.);
#26689=ORIENTED_EDGE('',*,*,#19958,.F.);
#26690=ORIENTED_EDGE('',*,*,#19954,.F.);
#26691=ORIENTED_EDGE('',*,*,#19979,.F.);
#26692=ORIENTED_EDGE('',*,*,#19980,.F.);
#26693=ORIENTED_EDGE('',*,*,#19981,.F.);
#26694=ORIENTED_EDGE('',*,*,#19982,.F.);
#26695=ORIENTED_EDGE('',*,*,#19983,.F.);
#26696=ORIENTED_EDGE('',*,*,#19959,.F.);
#26697=ORIENTED_EDGE('',*,*,#19984,.T.);
#26698=ORIENTED_EDGE('',*,*,#19985,.F.);
#26699=ORIENTED_EDGE('',*,*,#19808,.T.);
#26700=ORIENTED_EDGE('',*,*,#19956,.F.);
#26701=ORIENTED_EDGE('',*,*,#19986,.F.);
#26702=ORIENTED_EDGE('',*,*,#19987,.F.);
#26703=ORIENTED_EDGE('',*,*,#19984,.F.);
#26704=ORIENTED_EDGE('',*,*,#19978,.F.);
#26705=ORIENTED_EDGE('',*,*,#19988,.T.);
#26706=ORIENTED_EDGE('',*,*,#19989,.T.);
#26707=ORIENTED_EDGE('',*,*,#19986,.T.);
#26708=ORIENTED_EDGE('',*,*,#19968,.F.);
#26709=ORIENTED_EDGE('',*,*,#19966,.F.);
#26710=ORIENTED_EDGE('',*,*,#19990,.F.);
#26711=ORIENTED_EDGE('',*,*,#19988,.F.);
#26712=ORIENTED_EDGE('',*,*,#19991,.T.);
#26713=ORIENTED_EDGE('',*,*,#19992,.T.);
#26714=ORIENTED_EDGE('',*,*,#19993,.T.);
#26715=ORIENTED_EDGE('',*,*,#19994,.T.);
#26716=ORIENTED_EDGE('',*,*,#19995,.T.);
#26717=ORIENTED_EDGE('',*,*,#19996,.T.);
#26718=ORIENTED_EDGE('',*,*,#19997,.T.);
#26719=ORIENTED_EDGE('',*,*,#19998,.T.);
#26720=ORIENTED_EDGE('',*,*,#19997,.F.);
#26721=ORIENTED_EDGE('',*,*,#19999,.T.);
#26722=ORIENTED_EDGE('',*,*,#19991,.F.);
#26723=ORIENTED_EDGE('',*,*,#20000,.T.);
#26724=ORIENTED_EDGE('',*,*,#20001,.T.);
#26725=ORIENTED_EDGE('',*,*,#20002,.T.);
#26726=ORIENTED_EDGE('',*,*,#20003,.T.);
#26727=ORIENTED_EDGE('',*,*,#20004,.T.);
#26728=ORIENTED_EDGE('',*,*,#20005,.T.);
#26729=ORIENTED_EDGE('',*,*,#20006,.T.);
#26730=ORIENTED_EDGE('',*,*,#20007,.T.);
#26731=ORIENTED_EDGE('',*,*,#20003,.F.);
#26732=ORIENTED_EDGE('',*,*,#20005,.F.);
#26733=ORIENTED_EDGE('',*,*,#20008,.T.);
#26734=ORIENTED_EDGE('',*,*,#19995,.F.);
#26735=ORIENTED_EDGE('',*,*,#20009,.T.);
#26736=ORIENTED_EDGE('',*,*,#19827,.T.);
#26737=ORIENTED_EDGE('',*,*,#20010,.T.);
#26738=ORIENTED_EDGE('',*,*,#20011,.T.);
#26739=ORIENTED_EDGE('',*,*,#20012,.T.);
#26740=ORIENTED_EDGE('',*,*,#20013,.T.);
#26741=ORIENTED_EDGE('',*,*,#20014,.T.);
#26742=ORIENTED_EDGE('',*,*,#20015,.T.);
#26743=ORIENTED_EDGE('',*,*,#20014,.F.);
#26744=ORIENTED_EDGE('',*,*,#20016,.T.);
#26745=ORIENTED_EDGE('',*,*,#20009,.F.);
#26746=ORIENTED_EDGE('',*,*,#20012,.F.);
#26747=ORIENTED_EDGE('',*,*,#20017,.T.);
#26748=ORIENTED_EDGE('',*,*,#20001,.F.);
#26749=ORIENTED_EDGE('',*,*,#19999,.F.);
#26750=ORIENTED_EDGE('',*,*,#20018,.T.);
#26751=ORIENTED_EDGE('',*,*,#20019,.F.);
#26752=ORIENTED_EDGE('',*,*,#20020,.T.);
#26753=ORIENTED_EDGE('',*,*,#19996,.F.);
#26754=ORIENTED_EDGE('',*,*,#20021,.F.);
#26755=ORIENTED_EDGE('',*,*,#20022,.F.);
#26756=ORIENTED_EDGE('',*,*,#20018,.F.);
#26757=ORIENTED_EDGE('',*,*,#20008,.F.);
#26758=ORIENTED_EDGE('',*,*,#20023,.T.);
#26759=ORIENTED_EDGE('',*,*,#20024,.T.);
#26760=ORIENTED_EDGE('',*,*,#20021,.T.);
#26761=ORIENTED_EDGE('',*,*,#20004,.F.);
#26762=ORIENTED_EDGE('',*,*,#20002,.F.);
#26763=ORIENTED_EDGE('',*,*,#20025,.F.);
#26764=ORIENTED_EDGE('',*,*,#20023,.F.);
#26765=ORIENTED_EDGE('',*,*,#20017,.F.);
#26766=ORIENTED_EDGE('',*,*,#20026,.T.);
#26767=ORIENTED_EDGE('',*,*,#20027,.F.);
#26768=ORIENTED_EDGE('',*,*,#20025,.T.);
#26769=ORIENTED_EDGE('',*,*,#20015,.F.);
#26770=ORIENTED_EDGE('',*,*,#20011,.F.);
#26771=ORIENTED_EDGE('',*,*,#20028,.F.);
#26772=ORIENTED_EDGE('',*,*,#20029,.F.);
#26773=ORIENTED_EDGE('',*,*,#20030,.F.);
#26774=ORIENTED_EDGE('',*,*,#20026,.F.);
#26775=ORIENTED_EDGE('',*,*,#20031,.T.);
#26776=ORIENTED_EDGE('',*,*,#20032,.T.);
#26777=ORIENTED_EDGE('',*,*,#20033,.T.);
#26778=ORIENTED_EDGE('',*,*,#20034,.T.);
#26779=ORIENTED_EDGE('',*,*,#20035,.T.);
#26780=ORIENTED_EDGE('',*,*,#20036,.T.);
#26781=ORIENTED_EDGE('',*,*,#20037,.T.);
#26782=ORIENTED_EDGE('',*,*,#20038,.T.);
#26783=ORIENTED_EDGE('',*,*,#20037,.F.);
#26784=ORIENTED_EDGE('',*,*,#20039,.T.);
#26785=ORIENTED_EDGE('',*,*,#20031,.F.);
#26786=ORIENTED_EDGE('',*,*,#20040,.T.);
#26787=ORIENTED_EDGE('',*,*,#20041,.T.);
#26788=ORIENTED_EDGE('',*,*,#20042,.T.);
#26789=ORIENTED_EDGE('',*,*,#20043,.T.);
#26790=ORIENTED_EDGE('',*,*,#20044,.T.);
#26791=ORIENTED_EDGE('',*,*,#20045,.T.);
#26792=ORIENTED_EDGE('',*,*,#20046,.T.);
#26793=ORIENTED_EDGE('',*,*,#20047,.T.);
#26794=ORIENTED_EDGE('',*,*,#20043,.F.);
#26795=ORIENTED_EDGE('',*,*,#20045,.F.);
#26796=ORIENTED_EDGE('',*,*,#20048,.T.);
#26797=ORIENTED_EDGE('',*,*,#20035,.F.);
#26798=ORIENTED_EDGE('',*,*,#20049,.T.);
#26799=ORIENTED_EDGE('',*,*,#19787,.T.);
#26800=ORIENTED_EDGE('',*,*,#20050,.T.);
#26801=ORIENTED_EDGE('',*,*,#20051,.T.);
#26802=ORIENTED_EDGE('',*,*,#20052,.T.);
#26803=ORIENTED_EDGE('',*,*,#20053,.T.);
#26804=ORIENTED_EDGE('',*,*,#20054,.T.);
#26805=ORIENTED_EDGE('',*,*,#20055,.T.);
#26806=ORIENTED_EDGE('',*,*,#20054,.F.);
#26807=ORIENTED_EDGE('',*,*,#20056,.T.);
#26808=ORIENTED_EDGE('',*,*,#20049,.F.);
#26809=ORIENTED_EDGE('',*,*,#20052,.F.);
#26810=ORIENTED_EDGE('',*,*,#20057,.T.);
#26811=ORIENTED_EDGE('',*,*,#20041,.F.);
#26812=ORIENTED_EDGE('',*,*,#20039,.F.);
#26813=ORIENTED_EDGE('',*,*,#20058,.T.);
#26814=ORIENTED_EDGE('',*,*,#20059,.F.);
#26815=ORIENTED_EDGE('',*,*,#20060,.T.);
#26816=ORIENTED_EDGE('',*,*,#20036,.F.);
#26817=ORIENTED_EDGE('',*,*,#20061,.F.);
#26818=ORIENTED_EDGE('',*,*,#20062,.F.);
#26819=ORIENTED_EDGE('',*,*,#20058,.F.);
#26820=ORIENTED_EDGE('',*,*,#20048,.F.);
#26821=ORIENTED_EDGE('',*,*,#20063,.T.);
#26822=ORIENTED_EDGE('',*,*,#20064,.T.);
#26823=ORIENTED_EDGE('',*,*,#20061,.T.);
#26824=ORIENTED_EDGE('',*,*,#20044,.F.);
#26825=ORIENTED_EDGE('',*,*,#20042,.F.);
#26826=ORIENTED_EDGE('',*,*,#20065,.F.);
#26827=ORIENTED_EDGE('',*,*,#20063,.F.);
#26828=ORIENTED_EDGE('',*,*,#20057,.F.);
#26829=ORIENTED_EDGE('',*,*,#20066,.T.);
#26830=ORIENTED_EDGE('',*,*,#20067,.F.);
#26831=ORIENTED_EDGE('',*,*,#20065,.T.);
#26832=ORIENTED_EDGE('',*,*,#20055,.F.);
#26833=ORIENTED_EDGE('',*,*,#20051,.F.);
#26834=ORIENTED_EDGE('',*,*,#20068,.F.);
#26835=ORIENTED_EDGE('',*,*,#20069,.F.);
#26836=ORIENTED_EDGE('',*,*,#20070,.F.);
#26837=ORIENTED_EDGE('',*,*,#20066,.F.);
#26838=ORIENTED_EDGE('',*,*,#20071,.T.);
#26839=ORIENTED_EDGE('',*,*,#20072,.T.);
#26840=ORIENTED_EDGE('',*,*,#20073,.T.);
#26841=ORIENTED_EDGE('',*,*,#20074,.T.);
#26842=ORIENTED_EDGE('',*,*,#20075,.T.);
#26843=ORIENTED_EDGE('',*,*,#20076,.T.);
#26844=ORIENTED_EDGE('',*,*,#20077,.T.);
#26845=ORIENTED_EDGE('',*,*,#20078,.T.);
#26846=ORIENTED_EDGE('',*,*,#20077,.F.);
#26847=ORIENTED_EDGE('',*,*,#20079,.T.);
#26848=ORIENTED_EDGE('',*,*,#20071,.F.);
#26849=ORIENTED_EDGE('',*,*,#20080,.T.);
#26850=ORIENTED_EDGE('',*,*,#20081,.T.);
#26851=ORIENTED_EDGE('',*,*,#20082,.T.);
#26852=ORIENTED_EDGE('',*,*,#20083,.T.);
#26853=ORIENTED_EDGE('',*,*,#20082,.F.);
#26854=ORIENTED_EDGE('',*,*,#20084,.T.);
#26855=ORIENTED_EDGE('',*,*,#20075,.F.);
#26856=ORIENTED_EDGE('',*,*,#19688,.F.);
#26857=ORIENTED_EDGE('',*,*,#20085,.F.);
#26858=ORIENTED_EDGE('',*,*,#19708,.T.);
#26859=ORIENTED_EDGE('',*,*,#20086,.F.);
#26860=ORIENTED_EDGE('',*,*,#20087,.F.);
#26861=ORIENTED_EDGE('',*,*,#20088,.F.);
#26862=ORIENTED_EDGE('',*,*,#20089,.F.);
#26863=ORIENTED_EDGE('',*,*,#20090,.F.);
#26864=ORIENTED_EDGE('',*,*,#20091,.F.);
#26865=ORIENTED_EDGE('',*,*,#20092,.F.);
#26866=ORIENTED_EDGE('',*,*,#20093,.F.);
#26867=ORIENTED_EDGE('',*,*,#20094,.F.);
#26868=ORIENTED_EDGE('',*,*,#20095,.T.);
#26869=ORIENTED_EDGE('',*,*,#20096,.F.);
#26870=ORIENTED_EDGE('',*,*,#20097,.T.);
#26871=ORIENTED_EDGE('',*,*,#20098,.F.);
#26872=ORIENTED_EDGE('',*,*,#20099,.F.);
#26873=ORIENTED_EDGE('',*,*,#20100,.F.);
#26874=ORIENTED_EDGE('',*,*,#20101,.F.);
#26875=ORIENTED_EDGE('',*,*,#20102,.F.);
#26876=ORIENTED_EDGE('',*,*,#20103,.F.);
#26877=ORIENTED_EDGE('',*,*,#20104,.F.);
#26878=ORIENTED_EDGE('',*,*,#20105,.F.);
#26879=ORIENTED_EDGE('',*,*,#20106,.F.);
#26880=ORIENTED_EDGE('',*,*,#20107,.T.);
#26881=ORIENTED_EDGE('',*,*,#20108,.F.);
#26882=ORIENTED_EDGE('',*,*,#20109,.T.);
#26883=ORIENTED_EDGE('',*,*,#20110,.F.);
#26884=ORIENTED_EDGE('',*,*,#20111,.F.);
#26885=ORIENTED_EDGE('',*,*,#20112,.F.);
#26886=ORIENTED_EDGE('',*,*,#20113,.F.);
#26887=ORIENTED_EDGE('',*,*,#20114,.F.);
#26888=ORIENTED_EDGE('',*,*,#20115,.F.);
#26889=ORIENTED_EDGE('',*,*,#20116,.F.);
#26890=ORIENTED_EDGE('',*,*,#20117,.F.);
#26891=ORIENTED_EDGE('',*,*,#20118,.F.);
#26892=ORIENTED_EDGE('',*,*,#20119,.T.);
#26893=ORIENTED_EDGE('',*,*,#20120,.F.);
#26894=ORIENTED_EDGE('',*,*,#20121,.T.);
#26895=ORIENTED_EDGE('',*,*,#20122,.F.);
#26896=ORIENTED_EDGE('',*,*,#20123,.F.);
#26897=ORIENTED_EDGE('',*,*,#20124,.F.);
#26898=ORIENTED_EDGE('',*,*,#20125,.T.);
#26899=ORIENTED_EDGE('',*,*,#20126,.F.);
#26900=ORIENTED_EDGE('',*,*,#20127,.F.);
#26901=ORIENTED_EDGE('',*,*,#20128,.F.);
#26902=ORIENTED_EDGE('',*,*,#20129,.T.);
#26903=ORIENTED_EDGE('',*,*,#20130,.F.);
#26904=ORIENTED_EDGE('',*,*,#20131,.F.);
#26905=ORIENTED_EDGE('',*,*,#20132,.F.);
#26906=ORIENTED_EDGE('',*,*,#20133,.T.);
#26907=ORIENTED_EDGE('',*,*,#20134,.F.);
#26908=ORIENTED_EDGE('',*,*,#20135,.F.);
#26909=ORIENTED_EDGE('',*,*,#20136,.F.);
#26910=ORIENTED_EDGE('',*,*,#20137,.F.);
#26911=ORIENTED_EDGE('',*,*,#20138,.F.);
#26912=ORIENTED_EDGE('',*,*,#20139,.T.);
#26913=ORIENTED_EDGE('',*,*,#20140,.F.);
#26914=ORIENTED_EDGE('',*,*,#20141,.T.);
#26915=ORIENTED_EDGE('',*,*,#20142,.F.);
#26916=ORIENTED_EDGE('',*,*,#20143,.T.);
#26917=ORIENTED_EDGE('',*,*,#20144,.F.);
#26918=ORIENTED_EDGE('',*,*,#20145,.T.);
#26919=ORIENTED_EDGE('',*,*,#20146,.F.);
#26920=ORIENTED_EDGE('',*,*,#20147,.F.);
#26921=ORIENTED_EDGE('',*,*,#20148,.F.);
#26922=ORIENTED_EDGE('',*,*,#20149,.F.);
#26923=ORIENTED_EDGE('',*,*,#20150,.F.);
#26924=ORIENTED_EDGE('',*,*,#20151,.F.);
#26925=ORIENTED_EDGE('',*,*,#20152,.F.);
#26926=ORIENTED_EDGE('',*,*,#20153,.F.);
#26927=ORIENTED_EDGE('',*,*,#20154,.F.);
#26928=ORIENTED_EDGE('',*,*,#20155,.T.);
#26929=ORIENTED_EDGE('',*,*,#20156,.F.);
#26930=ORIENTED_EDGE('',*,*,#20157,.T.);
#26931=ORIENTED_EDGE('',*,*,#20158,.F.);
#26932=ORIENTED_EDGE('',*,*,#19992,.F.);
#26933=ORIENTED_EDGE('',*,*,#20020,.F.);
#26934=ORIENTED_EDGE('',*,*,#20159,.F.);
#26935=ORIENTED_EDGE('',*,*,#20160,.F.);
#26936=ORIENTED_EDGE('',*,*,#20161,.F.);
#26937=ORIENTED_EDGE('',*,*,#20162,.F.);
#26938=ORIENTED_EDGE('',*,*,#20163,.F.);
#26939=ORIENTED_EDGE('',*,*,#20164,.F.);
#26940=ORIENTED_EDGE('',*,*,#20165,.T.);
#26941=ORIENTED_EDGE('',*,*,#20166,.F.);
#26942=ORIENTED_EDGE('',*,*,#20167,.T.);
#26943=ORIENTED_EDGE('',*,*,#20168,.F.);
#26944=ORIENTED_EDGE('',*,*,#20169,.F.);
#26945=ORIENTED_EDGE('',*,*,#20170,.F.);
#26946=ORIENTED_EDGE('',*,*,#20171,.F.);
#26947=ORIENTED_EDGE('',*,*,#20172,.F.);
#26948=ORIENTED_EDGE('',*,*,#20173,.F.);
#26949=ORIENTED_EDGE('',*,*,#20174,.F.);
#26950=ORIENTED_EDGE('',*,*,#20175,.F.);
#26951=ORIENTED_EDGE('',*,*,#20176,.F.);
#26952=ORIENTED_EDGE('',*,*,#19961,.F.);
#26953=ORIENTED_EDGE('',*,*,#20177,.F.);
#26954=ORIENTED_EDGE('',*,*,#19981,.T.);
#26955=ORIENTED_EDGE('',*,*,#20178,.F.);
#26956=ORIENTED_EDGE('',*,*,#20179,.F.);
#26957=ORIENTED_EDGE('',*,*,#20180,.F.);
#26958=ORIENTED_EDGE('',*,*,#20181,.F.);
#26959=ORIENTED_EDGE('',*,*,#20182,.F.);
#26960=ORIENTED_EDGE('',*,*,#20183,.F.);
#26961=ORIENTED_EDGE('',*,*,#20184,.F.);
#26962=ORIENTED_EDGE('',*,*,#20185,.F.);
#26963=ORIENTED_EDGE('',*,*,#20186,.F.);
#26964=ORIENTED_EDGE('',*,*,#20187,.T.);
#26965=ORIENTED_EDGE('',*,*,#20188,.F.);
#26966=ORIENTED_EDGE('',*,*,#20189,.T.);
#26967=ORIENTED_EDGE('',*,*,#20190,.F.);
#26968=ORIENTED_EDGE('',*,*,#20191,.F.);
#26969=ORIENTED_EDGE('',*,*,#20192,.F.);
#26970=ORIENTED_EDGE('',*,*,#20193,.F.);
#26971=ORIENTED_EDGE('',*,*,#20194,.F.);
#26972=ORIENTED_EDGE('',*,*,#20032,.F.);
#26973=ORIENTED_EDGE('',*,*,#20060,.F.);
#26974=ORIENTED_EDGE('',*,*,#20195,.F.);
#26975=ORIENTED_EDGE('',*,*,#20196,.F.);
#26976=ORIENTED_EDGE('',*,*,#20197,.T.);
#26977=ORIENTED_EDGE('',*,*,#20198,.F.);
#26978=ORIENTED_EDGE('',*,*,#20199,.T.);
#26979=ORIENTED_EDGE('',*,*,#20200,.F.);
#26980=ORIENTED_EDGE('',*,*,#20072,.F.);
#26981=ORIENTED_EDGE('',*,*,#20201,.F.);
#26982=ORIENTED_EDGE('',*,*,#20202,.F.);
#26983=ORIENTED_EDGE('',*,*,#20203,.F.);
#26984=ORIENTED_EDGE('',*,*,#20204,.F.);
#26985=ORIENTED_EDGE('',*,*,#20205,.F.);
#26986=ORIENTED_EDGE('',*,*,#20206,.F.);
#26987=ORIENTED_EDGE('',*,*,#20207,.F.);
#26988=ORIENTED_EDGE('',*,*,#20208,.T.);
#26989=ORIENTED_EDGE('',*,*,#20209,.F.);
#26990=ORIENTED_EDGE('',*,*,#20210,.T.);
#26991=ORIENTED_EDGE('',*,*,#20211,.F.);
#26992=ORIENTED_EDGE('',*,*,#20212,.F.);
#26993=ORIENTED_EDGE('',*,*,#20213,.F.);
#26994=ORIENTED_EDGE('',*,*,#20214,.F.);
#26995=ORIENTED_EDGE('',*,*,#20215,.F.);
#26996=ORIENTED_EDGE('',*,*,#20216,.F.);
#26997=ORIENTED_EDGE('',*,*,#20217,.F.);
#26998=ORIENTED_EDGE('',*,*,#20218,.F.);
#26999=ORIENTED_EDGE('',*,*,#20219,.F.);
#27000=ORIENTED_EDGE('',*,*,#19922,.F.);
#27001=ORIENTED_EDGE('',*,*,#20220,.F.);
#27002=ORIENTED_EDGE('',*,*,#19942,.T.);
#27003=ORIENTED_EDGE('',*,*,#20221,.F.);
#27004=ORIENTED_EDGE('',*,*,#20222,.F.);
#27005=ORIENTED_EDGE('',*,*,#20223,.F.);
#27006=ORIENTED_EDGE('',*,*,#20224,.F.);
#27007=ORIENTED_EDGE('',*,*,#20225,.F.);
#27008=ORIENTED_EDGE('',*,*,#20226,.F.);
#27009=ORIENTED_EDGE('',*,*,#20227,.F.);
#27010=ORIENTED_EDGE('',*,*,#20228,.F.);
#27011=ORIENTED_EDGE('',*,*,#20229,.F.);
#27012=ORIENTED_EDGE('',*,*,#20230,.T.);
#27013=ORIENTED_EDGE('',*,*,#20231,.F.);
#27014=ORIENTED_EDGE('',*,*,#20232,.T.);
#27015=ORIENTED_EDGE('',*,*,#20233,.F.);
#27016=ORIENTED_EDGE('',*,*,#20234,.F.);
#27017=ORIENTED_EDGE('',*,*,#20235,.F.);
#27018=ORIENTED_EDGE('',*,*,#20236,.F.);
#27019=ORIENTED_EDGE('',*,*,#20237,.F.);
#27020=ORIENTED_EDGE('',*,*,#20238,.F.);
#27021=ORIENTED_EDGE('',*,*,#20239,.F.);
#27022=ORIENTED_EDGE('',*,*,#20240,.F.);
#27023=ORIENTED_EDGE('',*,*,#20241,.F.);
#27024=ORIENTED_EDGE('',*,*,#20242,.T.);
#27025=ORIENTED_EDGE('',*,*,#20243,.F.);
#27026=ORIENTED_EDGE('',*,*,#20244,.T.);
#27027=ORIENTED_EDGE('',*,*,#20245,.F.);
#27028=ORIENTED_EDGE('',*,*,#20246,.F.);
#27029=ORIENTED_EDGE('',*,*,#20247,.F.);
#27030=ORIENTED_EDGE('',*,*,#20248,.F.);
#27031=ORIENTED_EDGE('',*,*,#20249,.F.);
#27032=ORIENTED_EDGE('',*,*,#20250,.F.);
#27033=ORIENTED_EDGE('',*,*,#20251,.F.);
#27034=ORIENTED_EDGE('',*,*,#20252,.F.);
#27035=ORIENTED_EDGE('',*,*,#20253,.F.);
#27036=ORIENTED_EDGE('',*,*,#20254,.T.);
#27037=ORIENTED_EDGE('',*,*,#20255,.F.);
#27038=ORIENTED_EDGE('',*,*,#20256,.T.);
#27039=ORIENTED_EDGE('',*,*,#20257,.F.);
#27040=ORIENTED_EDGE('',*,*,#20258,.F.);
#27041=ORIENTED_EDGE('',*,*,#20259,.F.);
#27042=ORIENTED_EDGE('',*,*,#20260,.F.);
#27043=ORIENTED_EDGE('',*,*,#20261,.F.);
#27044=ORIENTED_EDGE('',*,*,#20262,.F.);
#27045=ORIENTED_EDGE('',*,*,#20263,.F.);
#27046=ORIENTED_EDGE('',*,*,#20264,.F.);
#27047=ORIENTED_EDGE('',*,*,#20265,.F.);
#27048=ORIENTED_EDGE('',*,*,#20266,.F.);
#27049=ORIENTED_EDGE('',*,*,#20079,.F.);
#27050=ORIENTED_EDGE('',*,*,#20267,.T.);
#27051=ORIENTED_EDGE('',*,*,#20268,.F.);
#27052=ORIENTED_EDGE('',*,*,#20201,.T.);
#27053=ORIENTED_EDGE('',*,*,#20076,.F.);
#27054=ORIENTED_EDGE('',*,*,#20269,.F.);
#27055=ORIENTED_EDGE('',*,*,#20270,.F.);
#27056=ORIENTED_EDGE('',*,*,#20267,.F.);
#27057=ORIENTED_EDGE('',*,*,#20084,.F.);
#27058=ORIENTED_EDGE('',*,*,#20271,.T.);
#27059=ORIENTED_EDGE('',*,*,#20272,.T.);
#27060=ORIENTED_EDGE('',*,*,#20269,.T.);
#27061=ORIENTED_EDGE('',*,*,#20081,.F.);
#27062=ORIENTED_EDGE('',*,*,#20273,.F.);
#27063=ORIENTED_EDGE('',*,*,#20274,.F.);
#27064=ORIENTED_EDGE('',*,*,#20271,.F.);
#27065=ORIENTED_EDGE('',*,*,#20275,.T.);
#27066=ORIENTED_EDGE('',*,*,#20226,.T.);
#27067=ORIENTED_EDGE('',*,*,#20276,.T.);
#27068=ORIENTED_EDGE('',*,*,#20277,.T.);
#27069=ORIENTED_EDGE('',*,*,#20278,.T.);
#27070=ORIENTED_EDGE('',*,*,#20279,.T.);
#27071=ORIENTED_EDGE('',*,*,#20280,.T.);
#27072=ORIENTED_EDGE('',*,*,#20281,.T.);
#27073=ORIENTED_EDGE('',*,*,#20280,.F.);
#27074=ORIENTED_EDGE('',*,*,#20282,.T.);
#27075=ORIENTED_EDGE('',*,*,#20275,.F.);
#27076=ORIENTED_EDGE('',*,*,#20283,.T.);
#27077=ORIENTED_EDGE('',*,*,#20284,.T.);
#27078=ORIENTED_EDGE('',*,*,#20285,.T.);
#27079=ORIENTED_EDGE('',*,*,#20286,.T.);
#27080=ORIENTED_EDGE('',*,*,#20285,.F.);
#27081=ORIENTED_EDGE('',*,*,#20287,.T.);
#27082=ORIENTED_EDGE('',*,*,#20278,.F.);
#27083=ORIENTED_EDGE('',*,*,#20282,.F.);
#27084=ORIENTED_EDGE('',*,*,#20288,.T.);
#27085=ORIENTED_EDGE('',*,*,#20289,.F.);
#27086=ORIENTED_EDGE('',*,*,#20227,.T.);
#27087=ORIENTED_EDGE('',*,*,#20279,.F.);
#27088=ORIENTED_EDGE('',*,*,#20290,.F.);
#27089=ORIENTED_EDGE('',*,*,#20291,.F.);
#27090=ORIENTED_EDGE('',*,*,#20288,.F.);
#27091=ORIENTED_EDGE('',*,*,#20287,.F.);
#27092=ORIENTED_EDGE('',*,*,#20292,.T.);
#27093=ORIENTED_EDGE('',*,*,#20293,.T.);
#27094=ORIENTED_EDGE('',*,*,#20290,.T.);
#27095=ORIENTED_EDGE('',*,*,#20284,.F.);
#27096=ORIENTED_EDGE('',*,*,#20294,.F.);
#27097=ORIENTED_EDGE('',*,*,#20295,.F.);
#27098=ORIENTED_EDGE('',*,*,#20292,.F.);
#27099=ORIENTED_EDGE('',*,*,#20296,.T.);
#27100=ORIENTED_EDGE('',*,*,#20111,.T.);
#27101=ORIENTED_EDGE('',*,*,#20297,.T.);
#27102=ORIENTED_EDGE('',*,*,#20298,.T.);
#27103=ORIENTED_EDGE('',*,*,#20299,.T.);
#27104=ORIENTED_EDGE('',*,*,#20300,.T.);
#27105=ORIENTED_EDGE('',*,*,#20301,.T.);
#27106=ORIENTED_EDGE('',*,*,#20302,.T.);
#27107=ORIENTED_EDGE('',*,*,#20301,.F.);
#27108=ORIENTED_EDGE('',*,*,#20303,.T.);
#27109=ORIENTED_EDGE('',*,*,#20296,.F.);
#27110=ORIENTED_EDGE('',*,*,#20304,.T.);
#27111=ORIENTED_EDGE('',*,*,#20305,.T.);
#27112=ORIENTED_EDGE('',*,*,#20306,.T.);
#27113=ORIENTED_EDGE('',*,*,#20307,.T.);
#27114=ORIENTED_EDGE('',*,*,#20306,.F.);
#27115=ORIENTED_EDGE('',*,*,#20308,.T.);
#27116=ORIENTED_EDGE('',*,*,#20299,.F.);
#27117=ORIENTED_EDGE('',*,*,#20303,.F.);
#27118=ORIENTED_EDGE('',*,*,#20309,.T.);
#27119=ORIENTED_EDGE('',*,*,#20310,.F.);
#27120=ORIENTED_EDGE('',*,*,#20112,.T.);
#27121=ORIENTED_EDGE('',*,*,#20300,.F.);
#27122=ORIENTED_EDGE('',*,*,#20311,.F.);
#27123=ORIENTED_EDGE('',*,*,#20312,.F.);
#27124=ORIENTED_EDGE('',*,*,#20309,.F.);
#27125=ORIENTED_EDGE('',*,*,#20308,.F.);
#27126=ORIENTED_EDGE('',*,*,#20313,.T.);
#27127=ORIENTED_EDGE('',*,*,#20314,.T.);
#27128=ORIENTED_EDGE('',*,*,#20311,.T.);
#27129=ORIENTED_EDGE('',*,*,#20305,.F.);
#27130=ORIENTED_EDGE('',*,*,#20315,.F.);
#27131=ORIENTED_EDGE('',*,*,#20316,.F.);
#27132=ORIENTED_EDGE('',*,*,#20313,.F.);
#27133=ORIENTED_EDGE('',*,*,#20317,.T.);
#27134=ORIENTED_EDGE('',*,*,#20123,.T.);
#27135=ORIENTED_EDGE('',*,*,#20318,.T.);
#27136=ORIENTED_EDGE('',*,*,#20319,.T.);
#27137=ORIENTED_EDGE('',*,*,#20320,.T.);
#27138=ORIENTED_EDGE('',*,*,#19865,.T.);
#27139=ORIENTED_EDGE('',*,*,#20321,.T.);
#27140=ORIENTED_EDGE('',*,*,#20322,.T.);
#27141=ORIENTED_EDGE('',*,*,#20323,.T.);
#27142=ORIENTED_EDGE('',*,*,#20324,.T.);
#27143=ORIENTED_EDGE('',*,*,#20325,.T.);
#27144=ORIENTED_EDGE('',*,*,#20326,.T.);
#27145=ORIENTED_EDGE('',*,*,#20325,.F.);
#27146=ORIENTED_EDGE('',*,*,#20327,.T.);
#27147=ORIENTED_EDGE('',*,*,#20320,.F.);
#27148=ORIENTED_EDGE('',*,*,#20328,.T.);
#27149=ORIENTED_EDGE('',*,*,#20329,.T.);
#27150=ORIENTED_EDGE('',*,*,#20330,.T.);
#27151=ORIENTED_EDGE('',*,*,#20331,.T.);
#27152=ORIENTED_EDGE('',*,*,#20332,.T.);
#27153=ORIENTED_EDGE('',*,*,#20333,.T.);
#27154=ORIENTED_EDGE('',*,*,#20334,.T.);
#27155=ORIENTED_EDGE('',*,*,#20335,.T.);
#27156=ORIENTED_EDGE('',*,*,#20331,.F.);
#27157=ORIENTED_EDGE('',*,*,#20333,.F.);
#27158=ORIENTED_EDGE('',*,*,#20336,.T.);
#27159=ORIENTED_EDGE('',*,*,#20323,.F.);
#27160=ORIENTED_EDGE('',*,*,#20337,.T.);
#27161=ORIENTED_EDGE('',*,*,#20338,.T.);
#27162=ORIENTED_EDGE('',*,*,#20339,.T.);
#27163=ORIENTED_EDGE('',*,*,#20340,.T.);
#27164=ORIENTED_EDGE('',*,*,#20337,.F.);
#27165=ORIENTED_EDGE('',*,*,#20341,.T.);
#27166=ORIENTED_EDGE('',*,*,#20329,.F.);
#27167=ORIENTED_EDGE('',*,*,#20339,.F.);
#27168=ORIENTED_EDGE('',*,*,#20342,.T.);
#27169=ORIENTED_EDGE('',*,*,#20317,.F.);
#27170=ORIENTED_EDGE('',*,*,#20332,.F.);
#27171=ORIENTED_EDGE('',*,*,#20330,.F.);
#27172=ORIENTED_EDGE('',*,*,#20343,.F.);
#27173=ORIENTED_EDGE('',*,*,#20344,.F.);
#27174=ORIENTED_EDGE('',*,*,#20341,.F.);
#27175=ORIENTED_EDGE('',*,*,#20345,.T.);
#27176=ORIENTED_EDGE('',*,*,#20346,.F.);
#27177=ORIENTED_EDGE('',*,*,#20343,.T.);
#27178=ORIENTED_EDGE('',*,*,#20340,.F.);
#27179=ORIENTED_EDGE('',*,*,#20319,.F.);
#27180=ORIENTED_EDGE('',*,*,#20347,.F.);
#27181=ORIENTED_EDGE('',*,*,#20348,.F.);
#27182=ORIENTED_EDGE('',*,*,#19868,.F.);
#27183=ORIENTED_EDGE('',*,*,#20349,.F.);
#27184=ORIENTED_EDGE('',*,*,#20345,.F.);
#27185=ORIENTED_EDGE('',*,*,#20342,.F.);
#27186=ORIENTED_EDGE('',*,*,#20350,.T.);
#27187=ORIENTED_EDGE('',*,*,#20351,.T.);
#27188=ORIENTED_EDGE('',*,*,#20124,.T.);
#27189=ORIENTED_EDGE('',*,*,#20338,.F.);
#27190=ORIENTED_EDGE('',*,*,#20328,.F.);
#27191=ORIENTED_EDGE('',*,*,#20335,.F.);
#27192=ORIENTED_EDGE('',*,*,#20352,.T.);
#27193=ORIENTED_EDGE('',*,*,#20350,.F.);
#27194=ORIENTED_EDGE('',*,*,#20353,.T.);
#27195=ORIENTED_EDGE('',*,*,#20103,.T.);
#27196=ORIENTED_EDGE('',*,*,#20354,.T.);
#27197=ORIENTED_EDGE('',*,*,#20355,.T.);
#27198=ORIENTED_EDGE('',*,*,#20356,.T.);
#27199=ORIENTED_EDGE('',*,*,#20357,.T.);
#27200=ORIENTED_EDGE('',*,*,#20358,.T.);
#27201=ORIENTED_EDGE('',*,*,#20359,.T.);
#27202=ORIENTED_EDGE('',*,*,#20358,.F.);
#27203=ORIENTED_EDGE('',*,*,#20360,.T.);
#27204=ORIENTED_EDGE('',*,*,#20353,.F.);
#27205=ORIENTED_EDGE('',*,*,#20361,.T.);
#27206=ORIENTED_EDGE('',*,*,#20362,.T.);
#27207=ORIENTED_EDGE('',*,*,#20363,.T.);
#27208=ORIENTED_EDGE('',*,*,#20364,.T.);
#27209=ORIENTED_EDGE('',*,*,#20363,.F.);
#27210=ORIENTED_EDGE('',*,*,#20365,.T.);
#27211=ORIENTED_EDGE('',*,*,#20356,.F.);
#27212=ORIENTED_EDGE('',*,*,#20360,.F.);
#27213=ORIENTED_EDGE('',*,*,#20366,.T.);
#27214=ORIENTED_EDGE('',*,*,#20367,.F.);
#27215=ORIENTED_EDGE('',*,*,#20104,.T.);
#27216=ORIENTED_EDGE('',*,*,#20357,.F.);
#27217=ORIENTED_EDGE('',*,*,#20368,.F.);
#27218=ORIENTED_EDGE('',*,*,#20369,.F.);
#27219=ORIENTED_EDGE('',*,*,#20366,.F.);
#27220=ORIENTED_EDGE('',*,*,#20365,.F.);
#27221=ORIENTED_EDGE('',*,*,#20370,.T.);
#27222=ORIENTED_EDGE('',*,*,#20371,.T.);
#27223=ORIENTED_EDGE('',*,*,#20368,.T.);
#27224=ORIENTED_EDGE('',*,*,#20362,.F.);
#27225=ORIENTED_EDGE('',*,*,#20372,.F.);
#27226=ORIENTED_EDGE('',*,*,#20373,.F.);
#27227=ORIENTED_EDGE('',*,*,#20370,.F.);
#27228=ORIENTED_EDGE('',*,*,#20374,.T.);
#27229=ORIENTED_EDGE('',*,*,#20115,.T.);
#27230=ORIENTED_EDGE('',*,*,#20375,.T.);
#27231=ORIENTED_EDGE('',*,*,#20376,.T.);
#27232=ORIENTED_EDGE('',*,*,#20377,.T.);
#27233=ORIENTED_EDGE('',*,*,#20378,.T.);
#27234=ORIENTED_EDGE('',*,*,#20379,.T.);
#27235=ORIENTED_EDGE('',*,*,#20380,.T.);
#27236=ORIENTED_EDGE('',*,*,#20379,.F.);
#27237=ORIENTED_EDGE('',*,*,#20381,.T.);
#27238=ORIENTED_EDGE('',*,*,#20374,.F.);
#27239=ORIENTED_EDGE('',*,*,#20382,.T.);
#27240=ORIENTED_EDGE('',*,*,#20383,.T.);
#27241=ORIENTED_EDGE('',*,*,#20384,.T.);
#27242=ORIENTED_EDGE('',*,*,#20385,.T.);
#27243=ORIENTED_EDGE('',*,*,#20384,.F.);
#27244=ORIENTED_EDGE('',*,*,#20386,.T.);
#27245=ORIENTED_EDGE('',*,*,#20377,.F.);
#27246=ORIENTED_EDGE('',*,*,#20381,.F.);
#27247=ORIENTED_EDGE('',*,*,#20387,.T.);
#27248=ORIENTED_EDGE('',*,*,#20388,.F.);
#27249=ORIENTED_EDGE('',*,*,#20116,.T.);
#27250=ORIENTED_EDGE('',*,*,#20378,.F.);
#27251=ORIENTED_EDGE('',*,*,#20389,.F.);
#27252=ORIENTED_EDGE('',*,*,#20390,.F.);
#27253=ORIENTED_EDGE('',*,*,#20387,.F.);
#27254=ORIENTED_EDGE('',*,*,#20386,.F.);
#27255=ORIENTED_EDGE('',*,*,#20391,.T.);
#27256=ORIENTED_EDGE('',*,*,#20392,.T.);
#27257=ORIENTED_EDGE('',*,*,#20389,.T.);
#27258=ORIENTED_EDGE('',*,*,#20383,.F.);
#27259=ORIENTED_EDGE('',*,*,#20393,.F.);
#27260=ORIENTED_EDGE('',*,*,#20394,.F.);
#27261=ORIENTED_EDGE('',*,*,#20391,.F.);
#27262=ORIENTED_EDGE('',*,*,#20395,.T.);
#27263=ORIENTED_EDGE('',*,*,#19870,.T.);
#27264=ORIENTED_EDGE('',*,*,#20396,.T.);
#27265=ORIENTED_EDGE('',*,*,#20397,.T.);
#27266=ORIENTED_EDGE('',*,*,#20398,.T.);
#27267=ORIENTED_EDGE('',*,*,#20399,.T.);
#27268=ORIENTED_EDGE('',*,*,#20400,.T.);
#27269=ORIENTED_EDGE('',*,*,#20401,.T.);
#27270=ORIENTED_EDGE('',*,*,#20400,.F.);
#27271=ORIENTED_EDGE('',*,*,#20402,.T.);
#27272=ORIENTED_EDGE('',*,*,#20395,.F.);
#27273=ORIENTED_EDGE('',*,*,#20403,.T.);
#27274=ORIENTED_EDGE('',*,*,#20404,.T.);
#27275=ORIENTED_EDGE('',*,*,#20405,.T.);
#27276=ORIENTED_EDGE('',*,*,#20406,.T.);
#27277=ORIENTED_EDGE('',*,*,#20405,.F.);
#27278=ORIENTED_EDGE('',*,*,#20407,.T.);
#27279=ORIENTED_EDGE('',*,*,#20398,.F.);
#27280=ORIENTED_EDGE('',*,*,#20402,.F.);
#27281=ORIENTED_EDGE('',*,*,#20408,.T.);
#27282=ORIENTED_EDGE('',*,*,#20409,.F.);
#27283=ORIENTED_EDGE('',*,*,#19871,.T.);
#27284=ORIENTED_EDGE('',*,*,#20399,.F.);
#27285=ORIENTED_EDGE('',*,*,#20410,.F.);
#27286=ORIENTED_EDGE('',*,*,#20411,.F.);
#27287=ORIENTED_EDGE('',*,*,#20408,.F.);
#27288=ORIENTED_EDGE('',*,*,#20412,.T.);
#27289=ORIENTED_EDGE('',*,*,#20127,.T.);
#27290=ORIENTED_EDGE('',*,*,#20413,.T.);
#27291=ORIENTED_EDGE('',*,*,#20414,.T.);
#27292=ORIENTED_EDGE('',*,*,#20415,.T.);
#27293=ORIENTED_EDGE('',*,*,#19860,.T.);
#27294=ORIENTED_EDGE('',*,*,#20416,.T.);
#27295=ORIENTED_EDGE('',*,*,#20417,.T.);
#27296=ORIENTED_EDGE('',*,*,#20418,.T.);
#27297=ORIENTED_EDGE('',*,*,#20419,.T.);
#27298=ORIENTED_EDGE('',*,*,#20420,.T.);
#27299=ORIENTED_EDGE('',*,*,#20421,.T.);
#27300=ORIENTED_EDGE('',*,*,#20420,.F.);
#27301=ORIENTED_EDGE('',*,*,#20422,.T.);
#27302=ORIENTED_EDGE('',*,*,#20415,.F.);
#27303=ORIENTED_EDGE('',*,*,#20423,.T.);
#27304=ORIENTED_EDGE('',*,*,#20424,.T.);
#27305=ORIENTED_EDGE('',*,*,#20425,.T.);
#27306=ORIENTED_EDGE('',*,*,#20426,.T.);
#27307=ORIENTED_EDGE('',*,*,#20427,.T.);
#27308=ORIENTED_EDGE('',*,*,#20428,.T.);
#27309=ORIENTED_EDGE('',*,*,#20429,.T.);
#27310=ORIENTED_EDGE('',*,*,#20430,.T.);
#27311=ORIENTED_EDGE('',*,*,#20426,.F.);
#27312=ORIENTED_EDGE('',*,*,#20428,.F.);
#27313=ORIENTED_EDGE('',*,*,#20431,.T.);
#27314=ORIENTED_EDGE('',*,*,#20418,.F.);
#27315=ORIENTED_EDGE('',*,*,#20432,.T.);
#27316=ORIENTED_EDGE('',*,*,#20433,.T.);
#27317=ORIENTED_EDGE('',*,*,#20434,.T.);
#27318=ORIENTED_EDGE('',*,*,#20435,.T.);
#27319=ORIENTED_EDGE('',*,*,#20432,.F.);
#27320=ORIENTED_EDGE('',*,*,#20436,.T.);
#27321=ORIENTED_EDGE('',*,*,#20424,.F.);
#27322=ORIENTED_EDGE('',*,*,#20434,.F.);
#27323=ORIENTED_EDGE('',*,*,#20437,.T.);
#27324=ORIENTED_EDGE('',*,*,#20412,.F.);
#27325=ORIENTED_EDGE('',*,*,#20427,.F.);
#27326=ORIENTED_EDGE('',*,*,#20425,.F.);
#27327=ORIENTED_EDGE('',*,*,#20438,.F.);
#27328=ORIENTED_EDGE('',*,*,#20439,.F.);
#27329=ORIENTED_EDGE('',*,*,#20436,.F.);
#27330=ORIENTED_EDGE('',*,*,#20440,.T.);
#27331=ORIENTED_EDGE('',*,*,#20441,.F.);
#27332=ORIENTED_EDGE('',*,*,#20438,.T.);
#27333=ORIENTED_EDGE('',*,*,#20435,.F.);
#27334=ORIENTED_EDGE('',*,*,#20414,.F.);
#27335=ORIENTED_EDGE('',*,*,#20442,.F.);
#27336=ORIENTED_EDGE('',*,*,#20443,.F.);
#27337=ORIENTED_EDGE('',*,*,#19863,.F.);
#27338=ORIENTED_EDGE('',*,*,#20444,.F.);
#27339=ORIENTED_EDGE('',*,*,#20440,.F.);
#27340=ORIENTED_EDGE('',*,*,#20437,.F.);
#27341=ORIENTED_EDGE('',*,*,#20445,.T.);
#27342=ORIENTED_EDGE('',*,*,#20446,.T.);
#27343=ORIENTED_EDGE('',*,*,#20128,.T.);
#27344=ORIENTED_EDGE('',*,*,#20433,.F.);
#27345=ORIENTED_EDGE('',*,*,#20423,.F.);
#27346=ORIENTED_EDGE('',*,*,#20430,.F.);
#27347=ORIENTED_EDGE('',*,*,#20447,.T.);
#27348=ORIENTED_EDGE('',*,*,#20445,.F.);
#27349=ORIENTED_EDGE('',*,*,#20448,.T.);
#27350=ORIENTED_EDGE('',*,*,#20411,.T.);
#27351=ORIENTED_EDGE('',*,*,#20449,.T.);
#27352=ORIENTED_EDGE('',*,*,#20450,.T.);
#27353=ORIENTED_EDGE('',*,*,#20407,.F.);
#27354=ORIENTED_EDGE('',*,*,#20451,.T.);
#27355=ORIENTED_EDGE('',*,*,#20452,.T.);
#27356=ORIENTED_EDGE('',*,*,#20410,.T.);
#27357=ORIENTED_EDGE('',*,*,#20452,.F.);
#27358=ORIENTED_EDGE('',*,*,#20453,.T.);
#27359=ORIENTED_EDGE('',*,*,#20449,.F.);
#27360=ORIENTED_EDGE('',*,*,#20454,.T.);
#27361=ORIENTED_EDGE('',*,*,#20455,.T.);
#27362=ORIENTED_EDGE('',*,*,#20456,.T.);
#27363=ORIENTED_EDGE('',*,*,#19872,.T.);
#27364=ORIENTED_EDGE('',*,*,#20454,.F.);
#27365=ORIENTED_EDGE('',*,*,#20409,.T.);
#27366=ORIENTED_EDGE('',*,*,#20448,.F.);
#27367=ORIENTED_EDGE('',*,*,#20397,.F.);
#27368=ORIENTED_EDGE('',*,*,#20457,.F.);
#27369=ORIENTED_EDGE('',*,*,#20458,.F.);
#27370=ORIENTED_EDGE('',*,*,#20121,.F.);
#27371=ORIENTED_EDGE('',*,*,#20459,.F.);
#27372=ORIENTED_EDGE('',*,*,#20460,.F.);
#27373=ORIENTED_EDGE('',*,*,#20406,.F.);
#27374=ORIENTED_EDGE('',*,*,#20401,.F.);
#27375=ORIENTED_EDGE('',*,*,#20461,.T.);
#27376=ORIENTED_EDGE('',*,*,#20390,.T.);
#27377=ORIENTED_EDGE('',*,*,#20462,.T.);
#27378=ORIENTED_EDGE('',*,*,#20463,.T.);
#27379=ORIENTED_EDGE('',*,*,#20464,.T.);
#27380=ORIENTED_EDGE('',*,*,#20465,.T.);
#27381=ORIENTED_EDGE('',*,*,#20466,.T.);
#27382=ORIENTED_EDGE('',*,*,#20117,.T.);
#27383=ORIENTED_EDGE('',*,*,#20464,.F.);
#27384=ORIENTED_EDGE('',*,*,#20388,.T.);
#27385=ORIENTED_EDGE('',*,*,#20461,.F.);
#27386=ORIENTED_EDGE('',*,*,#20392,.F.);
#27387=ORIENTED_EDGE('',*,*,#20467,.T.);
#27388=ORIENTED_EDGE('',*,*,#20462,.F.);
#27389=ORIENTED_EDGE('',*,*,#20376,.F.);
#27390=ORIENTED_EDGE('',*,*,#20468,.F.);
#27391=ORIENTED_EDGE('',*,*,#20469,.F.);
#27392=ORIENTED_EDGE('',*,*,#19876,.F.);
#27393=ORIENTED_EDGE('',*,*,#20470,.F.);
#27394=ORIENTED_EDGE('',*,*,#20471,.F.);
#27395=ORIENTED_EDGE('',*,*,#20385,.F.);
#27396=ORIENTED_EDGE('',*,*,#20380,.F.);
#27397=ORIENTED_EDGE('',*,*,#20472,.T.);
#27398=ORIENTED_EDGE('',*,*,#20091,.T.);
#27399=ORIENTED_EDGE('',*,*,#20473,.T.);
#27400=ORIENTED_EDGE('',*,*,#20474,.T.);
#27401=ORIENTED_EDGE('',*,*,#20475,.T.);
#27402=ORIENTED_EDGE('',*,*,#20476,.T.);
#27403=ORIENTED_EDGE('',*,*,#20477,.T.);
#27404=ORIENTED_EDGE('',*,*,#20478,.T.);
#27405=ORIENTED_EDGE('',*,*,#20477,.F.);
#27406=ORIENTED_EDGE('',*,*,#20479,.T.);
#27407=ORIENTED_EDGE('',*,*,#20472,.F.);
#27408=ORIENTED_EDGE('',*,*,#20480,.T.);
#27409=ORIENTED_EDGE('',*,*,#20481,.T.);
#27410=ORIENTED_EDGE('',*,*,#20482,.T.);
#27411=ORIENTED_EDGE('',*,*,#20483,.T.);
#27412=ORIENTED_EDGE('',*,*,#20482,.F.);
#27413=ORIENTED_EDGE('',*,*,#20484,.T.);
#27414=ORIENTED_EDGE('',*,*,#20475,.F.);
#27415=ORIENTED_EDGE('',*,*,#20479,.F.);
#27416=ORIENTED_EDGE('',*,*,#20485,.T.);
#27417=ORIENTED_EDGE('',*,*,#20486,.F.);
#27418=ORIENTED_EDGE('',*,*,#20092,.T.);
#27419=ORIENTED_EDGE('',*,*,#20476,.F.);
#27420=ORIENTED_EDGE('',*,*,#20487,.F.);
#27421=ORIENTED_EDGE('',*,*,#20488,.F.);
#27422=ORIENTED_EDGE('',*,*,#20485,.F.);
#27423=ORIENTED_EDGE('',*,*,#20484,.F.);
#27424=ORIENTED_EDGE('',*,*,#20489,.T.);
#27425=ORIENTED_EDGE('',*,*,#20490,.T.);
#27426=ORIENTED_EDGE('',*,*,#20487,.T.);
#27427=ORIENTED_EDGE('',*,*,#20481,.F.);
#27428=ORIENTED_EDGE('',*,*,#20491,.F.);
#27429=ORIENTED_EDGE('',*,*,#20492,.F.);
#27430=ORIENTED_EDGE('',*,*,#20489,.F.);
#27431=ORIENTED_EDGE('',*,*,#20493,.T.);
#27432=ORIENTED_EDGE('',*,*,#20369,.T.);
#27433=ORIENTED_EDGE('',*,*,#20494,.T.);
#27434=ORIENTED_EDGE('',*,*,#20495,.T.);
#27435=ORIENTED_EDGE('',*,*,#20496,.T.);
#27436=ORIENTED_EDGE('',*,*,#20497,.T.);
#27437=ORIENTED_EDGE('',*,*,#20498,.T.);
#27438=ORIENTED_EDGE('',*,*,#20105,.T.);
#27439=ORIENTED_EDGE('',*,*,#20496,.F.);
#27440=ORIENTED_EDGE('',*,*,#20367,.T.);
#27441=ORIENTED_EDGE('',*,*,#20493,.F.);
#27442=ORIENTED_EDGE('',*,*,#20371,.F.);
#27443=ORIENTED_EDGE('',*,*,#20499,.T.);
#27444=ORIENTED_EDGE('',*,*,#20494,.F.);
#27445=ORIENTED_EDGE('',*,*,#20355,.F.);
#27446=ORIENTED_EDGE('',*,*,#20500,.F.);
#27447=ORIENTED_EDGE('',*,*,#20501,.F.);
#27448=ORIENTED_EDGE('',*,*,#19888,.F.);
#27449=ORIENTED_EDGE('',*,*,#20502,.F.);
#27450=ORIENTED_EDGE('',*,*,#20503,.F.);
#27451=ORIENTED_EDGE('',*,*,#20364,.F.);
#27452=ORIENTED_EDGE('',*,*,#20359,.F.);
#27453=ORIENTED_EDGE('',*,*,#20504,.T.);
#27454=ORIENTED_EDGE('',*,*,#19882,.T.);
#27455=ORIENTED_EDGE('',*,*,#20505,.T.);
#27456=ORIENTED_EDGE('',*,*,#20506,.T.);
#27457=ORIENTED_EDGE('',*,*,#20507,.T.);
#27458=ORIENTED_EDGE('',*,*,#20508,.T.);
#27459=ORIENTED_EDGE('',*,*,#20509,.T.);
#27460=ORIENTED_EDGE('',*,*,#20510,.T.);
#27461=ORIENTED_EDGE('',*,*,#20509,.F.);
#27462=ORIENTED_EDGE('',*,*,#20511,.T.);
#27463=ORIENTED_EDGE('',*,*,#20504,.F.);
#27464=ORIENTED_EDGE('',*,*,#20512,.T.);
#27465=ORIENTED_EDGE('',*,*,#20513,.T.);
#27466=ORIENTED_EDGE('',*,*,#20514,.T.);
#27467=ORIENTED_EDGE('',*,*,#20515,.T.);
#27468=ORIENTED_EDGE('',*,*,#20514,.F.);
#27469=ORIENTED_EDGE('',*,*,#20516,.T.);
#27470=ORIENTED_EDGE('',*,*,#20507,.F.);
#27471=ORIENTED_EDGE('',*,*,#20511,.F.);
#27472=ORIENTED_EDGE('',*,*,#20517,.T.);
#27473=ORIENTED_EDGE('',*,*,#20518,.F.);
#27474=ORIENTED_EDGE('',*,*,#19883,.T.);
#27475=ORIENTED_EDGE('',*,*,#20508,.F.);
#27476=ORIENTED_EDGE('',*,*,#20519,.F.);
#27477=ORIENTED_EDGE('',*,*,#20520,.F.);
#27478=ORIENTED_EDGE('',*,*,#20517,.F.);
#27479=ORIENTED_EDGE('',*,*,#20521,.T.);
#27480=ORIENTED_EDGE('',*,*,#20312,.T.);
#27481=ORIENTED_EDGE('',*,*,#20522,.T.);
#27482=ORIENTED_EDGE('',*,*,#20523,.T.);
#27483=ORIENTED_EDGE('',*,*,#20524,.T.);
#27484=ORIENTED_EDGE('',*,*,#20525,.T.);
#27485=ORIENTED_EDGE('',*,*,#20526,.T.);
#27486=ORIENTED_EDGE('',*,*,#20113,.T.);
#27487=ORIENTED_EDGE('',*,*,#20524,.F.);
#27488=ORIENTED_EDGE('',*,*,#20310,.T.);
#27489=ORIENTED_EDGE('',*,*,#20521,.F.);
#27490=ORIENTED_EDGE('',*,*,#20314,.F.);
#27491=ORIENTED_EDGE('',*,*,#20527,.T.);
#27492=ORIENTED_EDGE('',*,*,#20522,.F.);
#27493=ORIENTED_EDGE('',*,*,#20527,.F.);
#27494=ORIENTED_EDGE('',*,*,#20316,.T.);
#27495=ORIENTED_EDGE('',*,*,#20528,.T.);
#27496=ORIENTED_EDGE('',*,*,#20529,.T.);
#27497=ORIENTED_EDGE('',*,*,#20523,.F.);
#27498=ORIENTED_EDGE('',*,*,#20529,.F.);
#27499=ORIENTED_EDGE('',*,*,#20530,.F.);
#27500=ORIENTED_EDGE('',*,*,#20531,.F.);
#27501=ORIENTED_EDGE('',*,*,#19878,.F.);
#27502=ORIENTED_EDGE('',*,*,#20532,.F.);
#27503=ORIENTED_EDGE('',*,*,#20533,.F.);
#27504=ORIENTED_EDGE('',*,*,#20525,.F.);
#27505=ORIENTED_EDGE('',*,*,#20534,.T.);
#27506=ORIENTED_EDGE('',*,*,#20520,.T.);
#27507=ORIENTED_EDGE('',*,*,#20535,.T.);
#27508=ORIENTED_EDGE('',*,*,#20536,.T.);
#27509=ORIENTED_EDGE('',*,*,#20516,.F.);
#27510=ORIENTED_EDGE('',*,*,#20537,.T.);
#27511=ORIENTED_EDGE('',*,*,#20538,.T.);
#27512=ORIENTED_EDGE('',*,*,#20519,.T.);
#27513=ORIENTED_EDGE('',*,*,#20538,.F.);
#27514=ORIENTED_EDGE('',*,*,#20539,.T.);
#27515=ORIENTED_EDGE('',*,*,#20535,.F.);
#27516=ORIENTED_EDGE('',*,*,#20540,.T.);
#27517=ORIENTED_EDGE('',*,*,#20541,.T.);
#27518=ORIENTED_EDGE('',*,*,#20542,.T.);
#27519=ORIENTED_EDGE('',*,*,#19884,.T.);
#27520=ORIENTED_EDGE('',*,*,#20540,.F.);
#27521=ORIENTED_EDGE('',*,*,#20518,.T.);
#27522=ORIENTED_EDGE('',*,*,#20534,.F.);
#27523=ORIENTED_EDGE('',*,*,#20506,.F.);
#27524=ORIENTED_EDGE('',*,*,#20543,.F.);
#27525=ORIENTED_EDGE('',*,*,#20544,.F.);
#27526=ORIENTED_EDGE('',*,*,#20109,.F.);
#27527=ORIENTED_EDGE('',*,*,#20545,.F.);
#27528=ORIENTED_EDGE('',*,*,#20546,.F.);
#27529=ORIENTED_EDGE('',*,*,#20515,.F.);
#27530=ORIENTED_EDGE('',*,*,#20510,.F.);
#27531=ORIENTED_EDGE('',*,*,#20499,.F.);
#27532=ORIENTED_EDGE('',*,*,#20373,.T.);
#27533=ORIENTED_EDGE('',*,*,#20547,.T.);
#27534=ORIENTED_EDGE('',*,*,#20548,.T.);
#27535=ORIENTED_EDGE('',*,*,#20495,.F.);
#27536=ORIENTED_EDGE('',*,*,#20548,.F.);
#27537=ORIENTED_EDGE('',*,*,#20549,.F.);
#27538=ORIENTED_EDGE('',*,*,#20550,.F.);
#27539=ORIENTED_EDGE('',*,*,#19886,.F.);
#27540=ORIENTED_EDGE('',*,*,#20551,.F.);
#27541=ORIENTED_EDGE('',*,*,#20552,.F.);
#27542=ORIENTED_EDGE('',*,*,#20497,.F.);
#27543=ORIENTED_EDGE('',*,*,#20553,.T.);
#27544=ORIENTED_EDGE('',*,*,#19894,.T.);
#27545=ORIENTED_EDGE('',*,*,#20554,.T.);
#27546=ORIENTED_EDGE('',*,*,#20555,.T.);
#27547=ORIENTED_EDGE('',*,*,#20556,.T.);
#27548=ORIENTED_EDGE('',*,*,#20557,.T.);
#27549=ORIENTED_EDGE('',*,*,#20558,.T.);
#27550=ORIENTED_EDGE('',*,*,#20559,.T.);
#27551=ORIENTED_EDGE('',*,*,#20558,.F.);
#27552=ORIENTED_EDGE('',*,*,#20560,.T.);
#27553=ORIENTED_EDGE('',*,*,#20553,.F.);
#27554=ORIENTED_EDGE('',*,*,#20561,.T.);
#27555=ORIENTED_EDGE('',*,*,#20562,.T.);
#27556=ORIENTED_EDGE('',*,*,#20563,.T.);
#27557=ORIENTED_EDGE('',*,*,#20564,.T.);
#27558=ORIENTED_EDGE('',*,*,#20563,.F.);
#27559=ORIENTED_EDGE('',*,*,#20565,.T.);
#27560=ORIENTED_EDGE('',*,*,#20556,.F.);
#27561=ORIENTED_EDGE('',*,*,#20560,.F.);
#27562=ORIENTED_EDGE('',*,*,#20566,.T.);
#27563=ORIENTED_EDGE('',*,*,#20567,.F.);
#27564=ORIENTED_EDGE('',*,*,#19895,.T.);
#27565=ORIENTED_EDGE('',*,*,#20557,.F.);
#27566=ORIENTED_EDGE('',*,*,#20568,.F.);
#27567=ORIENTED_EDGE('',*,*,#20569,.F.);
#27568=ORIENTED_EDGE('',*,*,#20566,.F.);
#27569=ORIENTED_EDGE('',*,*,#20570,.T.);
#27570=ORIENTED_EDGE('',*,*,#20262,.T.);
#27571=ORIENTED_EDGE('',*,*,#20571,.T.);
#27572=ORIENTED_EDGE('',*,*,#20572,.T.);
#27573=ORIENTED_EDGE('',*,*,#20573,.T.);
#27574=ORIENTED_EDGE('',*,*,#20574,.T.);
#27575=ORIENTED_EDGE('',*,*,#20575,.T.);
#27576=ORIENTED_EDGE('',*,*,#20576,.T.);
#27577=ORIENTED_EDGE('',*,*,#20575,.F.);
#27578=ORIENTED_EDGE('',*,*,#20577,.T.);
#27579=ORIENTED_EDGE('',*,*,#20570,.F.);
#27580=ORIENTED_EDGE('',*,*,#20578,.T.);
#27581=ORIENTED_EDGE('',*,*,#20579,.T.);
#27582=ORIENTED_EDGE('',*,*,#20580,.T.);
#27583=ORIENTED_EDGE('',*,*,#20581,.T.);
#27584=ORIENTED_EDGE('',*,*,#20580,.F.);
#27585=ORIENTED_EDGE('',*,*,#20582,.T.);
#27586=ORIENTED_EDGE('',*,*,#20573,.F.);
#27587=ORIENTED_EDGE('',*,*,#20577,.F.);
#27588=ORIENTED_EDGE('',*,*,#20583,.T.);
#27589=ORIENTED_EDGE('',*,*,#20584,.F.);
#27590=ORIENTED_EDGE('',*,*,#20263,.T.);
#27591=ORIENTED_EDGE('',*,*,#20574,.F.);
#27592=ORIENTED_EDGE('',*,*,#20585,.F.);
#27593=ORIENTED_EDGE('',*,*,#20586,.F.);
#27594=ORIENTED_EDGE('',*,*,#20583,.F.);
#27595=ORIENTED_EDGE('',*,*,#20582,.F.);
#27596=ORIENTED_EDGE('',*,*,#20587,.T.);
#27597=ORIENTED_EDGE('',*,*,#20588,.T.);
#27598=ORIENTED_EDGE('',*,*,#20585,.T.);
#27599=ORIENTED_EDGE('',*,*,#20579,.F.);
#27600=ORIENTED_EDGE('',*,*,#20589,.F.);
#27601=ORIENTED_EDGE('',*,*,#20590,.F.);
#27602=ORIENTED_EDGE('',*,*,#20587,.F.);
#27603=ORIENTED_EDGE('',*,*,#20591,.T.);
#27604=ORIENTED_EDGE('',*,*,#20258,.T.);
#27605=ORIENTED_EDGE('',*,*,#20592,.T.);
#27606=ORIENTED_EDGE('',*,*,#20593,.T.);
#27607=ORIENTED_EDGE('',*,*,#20594,.T.);
#27608=ORIENTED_EDGE('',*,*,#20595,.T.);
#27609=ORIENTED_EDGE('',*,*,#20596,.T.);
#27610=ORIENTED_EDGE('',*,*,#20597,.T.);
#27611=ORIENTED_EDGE('',*,*,#20596,.F.);
#27612=ORIENTED_EDGE('',*,*,#20598,.T.);
#27613=ORIENTED_EDGE('',*,*,#20591,.F.);
#27614=ORIENTED_EDGE('',*,*,#20599,.T.);
#27615=ORIENTED_EDGE('',*,*,#20600,.T.);
#27616=ORIENTED_EDGE('',*,*,#20601,.T.);
#27617=ORIENTED_EDGE('',*,*,#20602,.T.);
#27618=ORIENTED_EDGE('',*,*,#20601,.F.);
#27619=ORIENTED_EDGE('',*,*,#20603,.T.);
#27620=ORIENTED_EDGE('',*,*,#20594,.F.);
#27621=ORIENTED_EDGE('',*,*,#20598,.F.);
#27622=ORIENTED_EDGE('',*,*,#20604,.T.);
#27623=ORIENTED_EDGE('',*,*,#20605,.F.);
#27624=ORIENTED_EDGE('',*,*,#20259,.T.);
#27625=ORIENTED_EDGE('',*,*,#20595,.F.);
#27626=ORIENTED_EDGE('',*,*,#20606,.F.);
#27627=ORIENTED_EDGE('',*,*,#20607,.F.);
#27628=ORIENTED_EDGE('',*,*,#20604,.F.);
#27629=ORIENTED_EDGE('',*,*,#20603,.F.);
#27630=ORIENTED_EDGE('',*,*,#20608,.T.);
#27631=ORIENTED_EDGE('',*,*,#20609,.T.);
#27632=ORIENTED_EDGE('',*,*,#20606,.T.);
#27633=ORIENTED_EDGE('',*,*,#20600,.F.);
#27634=ORIENTED_EDGE('',*,*,#20610,.F.);
#27635=ORIENTED_EDGE('',*,*,#20611,.F.);
#27636=ORIENTED_EDGE('',*,*,#20608,.F.);
#27637=ORIENTED_EDGE('',*,*,#20612,.T.);
#27638=ORIENTED_EDGE('',*,*,#20488,.T.);
#27639=ORIENTED_EDGE('',*,*,#20613,.T.);
#27640=ORIENTED_EDGE('',*,*,#20614,.T.);
#27641=ORIENTED_EDGE('',*,*,#20615,.T.);
#27642=ORIENTED_EDGE('',*,*,#20616,.T.);
#27643=ORIENTED_EDGE('',*,*,#20617,.T.);
#27644=ORIENTED_EDGE('',*,*,#20093,.T.);
#27645=ORIENTED_EDGE('',*,*,#20615,.F.);
#27646=ORIENTED_EDGE('',*,*,#20486,.T.);
#27647=ORIENTED_EDGE('',*,*,#20612,.F.);
#27648=ORIENTED_EDGE('',*,*,#20490,.F.);
#27649=ORIENTED_EDGE('',*,*,#20618,.T.);
#27650=ORIENTED_EDGE('',*,*,#20613,.F.);
#27651=ORIENTED_EDGE('',*,*,#20474,.F.);
#27652=ORIENTED_EDGE('',*,*,#20619,.F.);
#27653=ORIENTED_EDGE('',*,*,#20620,.F.);
#27654=ORIENTED_EDGE('',*,*,#19900,.F.);
#27655=ORIENTED_EDGE('',*,*,#20621,.F.);
#27656=ORIENTED_EDGE('',*,*,#20622,.F.);
#27657=ORIENTED_EDGE('',*,*,#20483,.F.);
#27658=ORIENTED_EDGE('',*,*,#20478,.F.);
#27659=ORIENTED_EDGE('',*,*,#20623,.T.);
#27660=ORIENTED_EDGE('',*,*,#20099,.T.);
#27661=ORIENTED_EDGE('',*,*,#20624,.T.);
#27662=ORIENTED_EDGE('',*,*,#20625,.T.);
#27663=ORIENTED_EDGE('',*,*,#20626,.T.);
#27664=ORIENTED_EDGE('',*,*,#20627,.T.);
#27665=ORIENTED_EDGE('',*,*,#20628,.T.);
#27666=ORIENTED_EDGE('',*,*,#20629,.T.);
#27667=ORIENTED_EDGE('',*,*,#20628,.F.);
#27668=ORIENTED_EDGE('',*,*,#20630,.T.);
#27669=ORIENTED_EDGE('',*,*,#20623,.F.);
#27670=ORIENTED_EDGE('',*,*,#20631,.T.);
#27671=ORIENTED_EDGE('',*,*,#20632,.T.);
#27672=ORIENTED_EDGE('',*,*,#20633,.T.);
#27673=ORIENTED_EDGE('',*,*,#20634,.T.);
#27674=ORIENTED_EDGE('',*,*,#20633,.F.);
#27675=ORIENTED_EDGE('',*,*,#20635,.T.);
#27676=ORIENTED_EDGE('',*,*,#20626,.F.);
#27677=ORIENTED_EDGE('',*,*,#20630,.F.);
#27678=ORIENTED_EDGE('',*,*,#20636,.T.);
#27679=ORIENTED_EDGE('',*,*,#20637,.F.);
#27680=ORIENTED_EDGE('',*,*,#20100,.T.);
#27681=ORIENTED_EDGE('',*,*,#20627,.F.);
#27682=ORIENTED_EDGE('',*,*,#20638,.F.);
#27683=ORIENTED_EDGE('',*,*,#20639,.F.);
#27684=ORIENTED_EDGE('',*,*,#20636,.F.);
#27685=ORIENTED_EDGE('',*,*,#20635,.F.);
#27686=ORIENTED_EDGE('',*,*,#20640,.T.);
#27687=ORIENTED_EDGE('',*,*,#20641,.T.);
#27688=ORIENTED_EDGE('',*,*,#20638,.T.);
#27689=ORIENTED_EDGE('',*,*,#20632,.F.);
#27690=ORIENTED_EDGE('',*,*,#20642,.F.);
#27691=ORIENTED_EDGE('',*,*,#20643,.F.);
#27692=ORIENTED_EDGE('',*,*,#20640,.F.);
#27693=ORIENTED_EDGE('',*,*,#20644,.T.);
#27694=ORIENTED_EDGE('',*,*,#20639,.T.);
#27695=ORIENTED_EDGE('',*,*,#20645,.T.);
#27696=ORIENTED_EDGE('',*,*,#20646,.T.);
#27697=ORIENTED_EDGE('',*,*,#20647,.T.);
#27698=ORIENTED_EDGE('',*,*,#20648,.T.);
#27699=ORIENTED_EDGE('',*,*,#20649,.T.);
#27700=ORIENTED_EDGE('',*,*,#20101,.T.);
#27701=ORIENTED_EDGE('',*,*,#20647,.F.);
#27702=ORIENTED_EDGE('',*,*,#20637,.T.);
#27703=ORIENTED_EDGE('',*,*,#20644,.F.);
#27704=ORIENTED_EDGE('',*,*,#20641,.F.);
#27705=ORIENTED_EDGE('',*,*,#20650,.T.);
#27706=ORIENTED_EDGE('',*,*,#20645,.F.);
#27707=ORIENTED_EDGE('',*,*,#20625,.F.);
#27708=ORIENTED_EDGE('',*,*,#20651,.F.);
#27709=ORIENTED_EDGE('',*,*,#20652,.F.);
#27710=ORIENTED_EDGE('',*,*,#19892,.F.);
#27711=ORIENTED_EDGE('',*,*,#20653,.F.);
#27712=ORIENTED_EDGE('',*,*,#20654,.F.);
#27713=ORIENTED_EDGE('',*,*,#20634,.F.);
#27714=ORIENTED_EDGE('',*,*,#20629,.F.);
#27715=ORIENTED_EDGE('',*,*,#20618,.F.);
#27716=ORIENTED_EDGE('',*,*,#20492,.T.);
#27717=ORIENTED_EDGE('',*,*,#20655,.T.);
#27718=ORIENTED_EDGE('',*,*,#20656,.T.);
#27719=ORIENTED_EDGE('',*,*,#20614,.F.);
#27720=ORIENTED_EDGE('',*,*,#20656,.F.);
#27721=ORIENTED_EDGE('',*,*,#20657,.F.);
#27722=ORIENTED_EDGE('',*,*,#20658,.F.);
#27723=ORIENTED_EDGE('',*,*,#19898,.F.);
#27724=ORIENTED_EDGE('',*,*,#20659,.F.);
#27725=ORIENTED_EDGE('',*,*,#20660,.F.);
#27726=ORIENTED_EDGE('',*,*,#20616,.F.);
#27727=ORIENTED_EDGE('',*,*,#20661,.T.);
#27728=ORIENTED_EDGE('',*,*,#20246,.T.);
#27729=ORIENTED_EDGE('',*,*,#20662,.T.);
#27730=ORIENTED_EDGE('',*,*,#20663,.T.);
#27731=ORIENTED_EDGE('',*,*,#20664,.T.);
#27732=ORIENTED_EDGE('',*,*,#20665,.T.);
#27733=ORIENTED_EDGE('',*,*,#20666,.T.);
#27734=ORIENTED_EDGE('',*,*,#20667,.T.);
#27735=ORIENTED_EDGE('',*,*,#20666,.F.);
#27736=ORIENTED_EDGE('',*,*,#20668,.T.);
#27737=ORIENTED_EDGE('',*,*,#20661,.F.);
#27738=ORIENTED_EDGE('',*,*,#20669,.T.);
#27739=ORIENTED_EDGE('',*,*,#20670,.T.);
#27740=ORIENTED_EDGE('',*,*,#20671,.T.);
#27741=ORIENTED_EDGE('',*,*,#20672,.T.);
#27742=ORIENTED_EDGE('',*,*,#20671,.F.);
#27743=ORIENTED_EDGE('',*,*,#20673,.T.);
#27744=ORIENTED_EDGE('',*,*,#20664,.F.);
#27745=ORIENTED_EDGE('',*,*,#20668,.F.);
#27746=ORIENTED_EDGE('',*,*,#20674,.T.);
#27747=ORIENTED_EDGE('',*,*,#20675,.F.);
#27748=ORIENTED_EDGE('',*,*,#20247,.T.);
#27749=ORIENTED_EDGE('',*,*,#20665,.F.);
#27750=ORIENTED_EDGE('',*,*,#20676,.F.);
#27751=ORIENTED_EDGE('',*,*,#20677,.F.);
#27752=ORIENTED_EDGE('',*,*,#20674,.F.);
#27753=ORIENTED_EDGE('',*,*,#20673,.F.);
#27754=ORIENTED_EDGE('',*,*,#20678,.T.);
#27755=ORIENTED_EDGE('',*,*,#20679,.T.);
#27756=ORIENTED_EDGE('',*,*,#20676,.T.);
#27757=ORIENTED_EDGE('',*,*,#20670,.F.);
#27758=ORIENTED_EDGE('',*,*,#20680,.F.);
#27759=ORIENTED_EDGE('',*,*,#20681,.F.);
#27760=ORIENTED_EDGE('',*,*,#20678,.F.);
#27761=ORIENTED_EDGE('',*,*,#20682,.T.);
#27762=ORIENTED_EDGE('',*,*,#20238,.T.);
#27763=ORIENTED_EDGE('',*,*,#20683,.T.);
#27764=ORIENTED_EDGE('',*,*,#20684,.T.);
#27765=ORIENTED_EDGE('',*,*,#20685,.T.);
#27766=ORIENTED_EDGE('',*,*,#20686,.T.);
#27767=ORIENTED_EDGE('',*,*,#20687,.T.);
#27768=ORIENTED_EDGE('',*,*,#20688,.T.);
#27769=ORIENTED_EDGE('',*,*,#20687,.F.);
#27770=ORIENTED_EDGE('',*,*,#20689,.T.);
#27771=ORIENTED_EDGE('',*,*,#20682,.F.);
#27772=ORIENTED_EDGE('',*,*,#20690,.T.);
#27773=ORIENTED_EDGE('',*,*,#20691,.T.);
#27774=ORIENTED_EDGE('',*,*,#20692,.T.);
#27775=ORIENTED_EDGE('',*,*,#20693,.T.);
#27776=ORIENTED_EDGE('',*,*,#20692,.F.);
#27777=ORIENTED_EDGE('',*,*,#20694,.T.);
#27778=ORIENTED_EDGE('',*,*,#20685,.F.);
#27779=ORIENTED_EDGE('',*,*,#20689,.F.);
#27780=ORIENTED_EDGE('',*,*,#20695,.T.);
#27781=ORIENTED_EDGE('',*,*,#20696,.F.);
#27782=ORIENTED_EDGE('',*,*,#20239,.T.);
#27783=ORIENTED_EDGE('',*,*,#20686,.F.);
#27784=ORIENTED_EDGE('',*,*,#20697,.F.);
#27785=ORIENTED_EDGE('',*,*,#20698,.F.);
#27786=ORIENTED_EDGE('',*,*,#20695,.F.);
#27787=ORIENTED_EDGE('',*,*,#20694,.F.);
#27788=ORIENTED_EDGE('',*,*,#20699,.T.);
#27789=ORIENTED_EDGE('',*,*,#20700,.T.);
#27790=ORIENTED_EDGE('',*,*,#20697,.T.);
#27791=ORIENTED_EDGE('',*,*,#20691,.F.);
#27792=ORIENTED_EDGE('',*,*,#20701,.F.);
#27793=ORIENTED_EDGE('',*,*,#20702,.F.);
#27794=ORIENTED_EDGE('',*,*,#20699,.F.);
#27795=ORIENTED_EDGE('',*,*,#20703,.T.);
#27796=ORIENTED_EDGE('',*,*,#19723,.T.);
#27797=ORIENTED_EDGE('',*,*,#20704,.T.);
#27798=ORIENTED_EDGE('',*,*,#20705,.T.);
#27799=ORIENTED_EDGE('',*,*,#20706,.T.);
#27800=ORIENTED_EDGE('',*,*,#20707,.T.);
#27801=ORIENTED_EDGE('',*,*,#20708,.T.);
#27802=ORIENTED_EDGE('',*,*,#20709,.T.);
#27803=ORIENTED_EDGE('',*,*,#20708,.F.);
#27804=ORIENTED_EDGE('',*,*,#20710,.T.);
#27805=ORIENTED_EDGE('',*,*,#20703,.F.);
#27806=ORIENTED_EDGE('',*,*,#20711,.T.);
#27807=ORIENTED_EDGE('',*,*,#20712,.T.);
#27808=ORIENTED_EDGE('',*,*,#20713,.T.);
#27809=ORIENTED_EDGE('',*,*,#20714,.T.);
#27810=ORIENTED_EDGE('',*,*,#20713,.F.);
#27811=ORIENTED_EDGE('',*,*,#20715,.T.);
#27812=ORIENTED_EDGE('',*,*,#20706,.F.);
#27813=ORIENTED_EDGE('',*,*,#20710,.F.);
#27814=ORIENTED_EDGE('',*,*,#20716,.T.);
#27815=ORIENTED_EDGE('',*,*,#20717,.F.);
#27816=ORIENTED_EDGE('',*,*,#19724,.T.);
#27817=ORIENTED_EDGE('',*,*,#20707,.F.);
#27818=ORIENTED_EDGE('',*,*,#20718,.F.);
#27819=ORIENTED_EDGE('',*,*,#20719,.F.);
#27820=ORIENTED_EDGE('',*,*,#20716,.F.);
#27821=ORIENTED_EDGE('',*,*,#20720,.T.);
#27822=ORIENTED_EDGE('',*,*,#20607,.T.);
#27823=ORIENTED_EDGE('',*,*,#20721,.T.);
#27824=ORIENTED_EDGE('',*,*,#20722,.T.);
#27825=ORIENTED_EDGE('',*,*,#20723,.T.);
#27826=ORIENTED_EDGE('',*,*,#20724,.T.);
#27827=ORIENTED_EDGE('',*,*,#20725,.T.);
#27828=ORIENTED_EDGE('',*,*,#20260,.T.);
#27829=ORIENTED_EDGE('',*,*,#20723,.F.);
#27830=ORIENTED_EDGE('',*,*,#20605,.T.);
#27831=ORIENTED_EDGE('',*,*,#20720,.F.);
#27832=ORIENTED_EDGE('',*,*,#20609,.F.);
#27833=ORIENTED_EDGE('',*,*,#20726,.T.);
#27834=ORIENTED_EDGE('',*,*,#20721,.F.);
#27835=ORIENTED_EDGE('',*,*,#20593,.F.);
#27836=ORIENTED_EDGE('',*,*,#20727,.F.);
#27837=ORIENTED_EDGE('',*,*,#20728,.F.);
#27838=ORIENTED_EDGE('',*,*,#19721,.F.);
#27839=ORIENTED_EDGE('',*,*,#20729,.F.);
#27840=ORIENTED_EDGE('',*,*,#20730,.F.);
#27841=ORIENTED_EDGE('',*,*,#20602,.F.);
#27842=ORIENTED_EDGE('',*,*,#20597,.F.);
#27843=ORIENTED_EDGE('',*,*,#20731,.T.);
#27844=ORIENTED_EDGE('',*,*,#20586,.T.);
#27845=ORIENTED_EDGE('',*,*,#20732,.T.);
#27846=ORIENTED_EDGE('',*,*,#20733,.T.);
#27847=ORIENTED_EDGE('',*,*,#20734,.T.);
#27848=ORIENTED_EDGE('',*,*,#20735,.T.);
#27849=ORIENTED_EDGE('',*,*,#20736,.T.);
#27850=ORIENTED_EDGE('',*,*,#20264,.T.);
#27851=ORIENTED_EDGE('',*,*,#20734,.F.);
#27852=ORIENTED_EDGE('',*,*,#20584,.T.);
#27853=ORIENTED_EDGE('',*,*,#20731,.F.);
#27854=ORIENTED_EDGE('',*,*,#20588,.F.);
#27855=ORIENTED_EDGE('',*,*,#20737,.T.);
#27856=ORIENTED_EDGE('',*,*,#20732,.F.);
#27857=ORIENTED_EDGE('',*,*,#20572,.F.);
#27858=ORIENTED_EDGE('',*,*,#20738,.F.);
#27859=ORIENTED_EDGE('',*,*,#20739,.F.);
#27860=ORIENTED_EDGE('',*,*,#19717,.F.);
#27861=ORIENTED_EDGE('',*,*,#20740,.F.);
#27862=ORIENTED_EDGE('',*,*,#20741,.F.);
#27863=ORIENTED_EDGE('',*,*,#20581,.F.);
#27864=ORIENTED_EDGE('',*,*,#20576,.F.);
#27865=ORIENTED_EDGE('',*,*,#20742,.T.);
#27866=ORIENTED_EDGE('',*,*,#20087,.T.);
#27867=ORIENTED_EDGE('',*,*,#20743,.T.);
#27868=ORIENTED_EDGE('',*,*,#20744,.T.);
#27869=ORIENTED_EDGE('',*,*,#20745,.T.);
#27870=ORIENTED_EDGE('',*,*,#20746,.T.);
#27871=ORIENTED_EDGE('',*,*,#20747,.T.);
#27872=ORIENTED_EDGE('',*,*,#20748,.T.);
#27873=ORIENTED_EDGE('',*,*,#20747,.F.);
#27874=ORIENTED_EDGE('',*,*,#20749,.T.);
#27875=ORIENTED_EDGE('',*,*,#20742,.F.);
#27876=ORIENTED_EDGE('',*,*,#20750,.T.);
#27877=ORIENTED_EDGE('',*,*,#20751,.T.);
#27878=ORIENTED_EDGE('',*,*,#20752,.T.);
#27879=ORIENTED_EDGE('',*,*,#20753,.T.);
#27880=ORIENTED_EDGE('',*,*,#20752,.F.);
#27881=ORIENTED_EDGE('',*,*,#20754,.T.);
#27882=ORIENTED_EDGE('',*,*,#20745,.F.);
#27883=ORIENTED_EDGE('',*,*,#20749,.F.);
#27884=ORIENTED_EDGE('',*,*,#20755,.T.);
#27885=ORIENTED_EDGE('',*,*,#20756,.F.);
#27886=ORIENTED_EDGE('',*,*,#20088,.T.);
#27887=ORIENTED_EDGE('',*,*,#20746,.F.);
#27888=ORIENTED_EDGE('',*,*,#20757,.F.);
#27889=ORIENTED_EDGE('',*,*,#20758,.F.);
#27890=ORIENTED_EDGE('',*,*,#20755,.F.);
#27891=ORIENTED_EDGE('',*,*,#20754,.F.);
#27892=ORIENTED_EDGE('',*,*,#20759,.T.);
#27893=ORIENTED_EDGE('',*,*,#20760,.T.);
#27894=ORIENTED_EDGE('',*,*,#20757,.T.);
#27895=ORIENTED_EDGE('',*,*,#20751,.F.);
#27896=ORIENTED_EDGE('',*,*,#20761,.F.);
#27897=ORIENTED_EDGE('',*,*,#20762,.F.);
#27898=ORIENTED_EDGE('',*,*,#20759,.F.);
#27899=ORIENTED_EDGE('',*,*,#20763,.T.);
#27900=ORIENTED_EDGE('',*,*,#20758,.T.);
#27901=ORIENTED_EDGE('',*,*,#20764,.T.);
#27902=ORIENTED_EDGE('',*,*,#20765,.T.);
#27903=ORIENTED_EDGE('',*,*,#20766,.T.);
#27904=ORIENTED_EDGE('',*,*,#20767,.T.);
#27905=ORIENTED_EDGE('',*,*,#20768,.T.);
#27906=ORIENTED_EDGE('',*,*,#20089,.T.);
#27907=ORIENTED_EDGE('',*,*,#20766,.F.);
#27908=ORIENTED_EDGE('',*,*,#20756,.T.);
#27909=ORIENTED_EDGE('',*,*,#20763,.F.);
#27910=ORIENTED_EDGE('',*,*,#20760,.F.);
#27911=ORIENTED_EDGE('',*,*,#20769,.T.);
#27912=ORIENTED_EDGE('',*,*,#20764,.F.);
#27913=ORIENTED_EDGE('',*,*,#20744,.F.);
#27914=ORIENTED_EDGE('',*,*,#20770,.F.);
#27915=ORIENTED_EDGE('',*,*,#20771,.F.);
#27916=ORIENTED_EDGE('',*,*,#19904,.F.);
#27917=ORIENTED_EDGE('',*,*,#20772,.F.);
#27918=ORIENTED_EDGE('',*,*,#20773,.F.);
#27919=ORIENTED_EDGE('',*,*,#20753,.F.);
#27920=ORIENTED_EDGE('',*,*,#20748,.F.);
#27921=ORIENTED_EDGE('',*,*,#20737,.F.);
#27922=ORIENTED_EDGE('',*,*,#20590,.T.);
#27923=ORIENTED_EDGE('',*,*,#20774,.T.);
#27924=ORIENTED_EDGE('',*,*,#20775,.T.);
#27925=ORIENTED_EDGE('',*,*,#20733,.F.);
#27926=ORIENTED_EDGE('',*,*,#20775,.F.);
#27927=ORIENTED_EDGE('',*,*,#20776,.F.);
#27928=ORIENTED_EDGE('',*,*,#20777,.F.);
#27929=ORIENTED_EDGE('',*,*,#19715,.F.);
#27930=ORIENTED_EDGE('',*,*,#20778,.F.);
#27931=ORIENTED_EDGE('',*,*,#20779,.F.);
#27932=ORIENTED_EDGE('',*,*,#20735,.F.);
#27933=ORIENTED_EDGE('',*,*,#20726,.F.);
#27934=ORIENTED_EDGE('',*,*,#20611,.T.);
#27935=ORIENTED_EDGE('',*,*,#20780,.T.);
#27936=ORIENTED_EDGE('',*,*,#20781,.T.);
#27937=ORIENTED_EDGE('',*,*,#20722,.F.);
#27938=ORIENTED_EDGE('',*,*,#20781,.F.);
#27939=ORIENTED_EDGE('',*,*,#20782,.F.);
#27940=ORIENTED_EDGE('',*,*,#20783,.F.);
#27941=ORIENTED_EDGE('',*,*,#19719,.F.);
#27942=ORIENTED_EDGE('',*,*,#20784,.F.);
#27943=ORIENTED_EDGE('',*,*,#20785,.F.);
#27944=ORIENTED_EDGE('',*,*,#20724,.F.);
#27945=ORIENTED_EDGE('',*,*,#20786,.T.);
#27946=ORIENTED_EDGE('',*,*,#20719,.T.);
#27947=ORIENTED_EDGE('',*,*,#20787,.T.);
#27948=ORIENTED_EDGE('',*,*,#20788,.T.);
#27949=ORIENTED_EDGE('',*,*,#20715,.F.);
#27950=ORIENTED_EDGE('',*,*,#20789,.T.);
#27951=ORIENTED_EDGE('',*,*,#20790,.T.);
#27952=ORIENTED_EDGE('',*,*,#20718,.T.);
#27953=ORIENTED_EDGE('',*,*,#20790,.F.);
#27954=ORIENTED_EDGE('',*,*,#20791,.T.);
#27955=ORIENTED_EDGE('',*,*,#20787,.F.);
#27956=ORIENTED_EDGE('',*,*,#20792,.T.);
#27957=ORIENTED_EDGE('',*,*,#20793,.T.);
#27958=ORIENTED_EDGE('',*,*,#20794,.T.);
#27959=ORIENTED_EDGE('',*,*,#19725,.T.);
#27960=ORIENTED_EDGE('',*,*,#20792,.F.);
#27961=ORIENTED_EDGE('',*,*,#20717,.T.);
#27962=ORIENTED_EDGE('',*,*,#20786,.F.);
#27963=ORIENTED_EDGE('',*,*,#20705,.F.);
#27964=ORIENTED_EDGE('',*,*,#20795,.F.);
#27965=ORIENTED_EDGE('',*,*,#20796,.F.);
#27966=ORIENTED_EDGE('',*,*,#20256,.F.);
#27967=ORIENTED_EDGE('',*,*,#20797,.F.);
#27968=ORIENTED_EDGE('',*,*,#20798,.F.);
#27969=ORIENTED_EDGE('',*,*,#20714,.F.);
#27970=ORIENTED_EDGE('',*,*,#20709,.F.);
#27971=ORIENTED_EDGE('',*,*,#20799,.T.);
#27972=ORIENTED_EDGE('',*,*,#20698,.T.);
#27973=ORIENTED_EDGE('',*,*,#20800,.T.);
#27974=ORIENTED_EDGE('',*,*,#20801,.T.);
#27975=ORIENTED_EDGE('',*,*,#20802,.T.);
#27976=ORIENTED_EDGE('',*,*,#20803,.T.);
#27977=ORIENTED_EDGE('',*,*,#20804,.T.);
#27978=ORIENTED_EDGE('',*,*,#20240,.T.);
#27979=ORIENTED_EDGE('',*,*,#20802,.F.);
#27980=ORIENTED_EDGE('',*,*,#20696,.T.);
#27981=ORIENTED_EDGE('',*,*,#20799,.F.);
#27982=ORIENTED_EDGE('',*,*,#20700,.F.);
#27983=ORIENTED_EDGE('',*,*,#20805,.T.);
#27984=ORIENTED_EDGE('',*,*,#20800,.F.);
#27985=ORIENTED_EDGE('',*,*,#20684,.F.);
#27986=ORIENTED_EDGE('',*,*,#20806,.F.);
#27987=ORIENTED_EDGE('',*,*,#20807,.F.);
#27988=ORIENTED_EDGE('',*,*,#19741,.F.);
#27989=ORIENTED_EDGE('',*,*,#20808,.F.);
#27990=ORIENTED_EDGE('',*,*,#20809,.F.);
#27991=ORIENTED_EDGE('',*,*,#20693,.F.);
#27992=ORIENTED_EDGE('',*,*,#20688,.F.);
#27993=ORIENTED_EDGE('',*,*,#20810,.T.);
#27994=ORIENTED_EDGE('',*,*,#19735,.T.);
#27995=ORIENTED_EDGE('',*,*,#20811,.T.);
#27996=ORIENTED_EDGE('',*,*,#20812,.T.);
#27997=ORIENTED_EDGE('',*,*,#20813,.T.);
#27998=ORIENTED_EDGE('',*,*,#20814,.T.);
#27999=ORIENTED_EDGE('',*,*,#20815,.T.);
#28000=ORIENTED_EDGE('',*,*,#20816,.T.);
#28001=ORIENTED_EDGE('',*,*,#20815,.F.);
#28002=ORIENTED_EDGE('',*,*,#20817,.T.);
#28003=ORIENTED_EDGE('',*,*,#20810,.F.);
#28004=ORIENTED_EDGE('',*,*,#20818,.T.);
#28005=ORIENTED_EDGE('',*,*,#20819,.T.);
#28006=ORIENTED_EDGE('',*,*,#20820,.T.);
#28007=ORIENTED_EDGE('',*,*,#20821,.T.);
#28008=ORIENTED_EDGE('',*,*,#20820,.F.);
#28009=ORIENTED_EDGE('',*,*,#20822,.T.);
#28010=ORIENTED_EDGE('',*,*,#20813,.F.);
#28011=ORIENTED_EDGE('',*,*,#20817,.F.);
#28012=ORIENTED_EDGE('',*,*,#20823,.T.);
#28013=ORIENTED_EDGE('',*,*,#20824,.F.);
#28014=ORIENTED_EDGE('',*,*,#19736,.T.);
#28015=ORIENTED_EDGE('',*,*,#20814,.F.);
#28016=ORIENTED_EDGE('',*,*,#20825,.F.);
#28017=ORIENTED_EDGE('',*,*,#20826,.F.);
#28018=ORIENTED_EDGE('',*,*,#20823,.F.);
#28019=ORIENTED_EDGE('',*,*,#20827,.T.);
#28020=ORIENTED_EDGE('',*,*,#20677,.T.);
#28021=ORIENTED_EDGE('',*,*,#20828,.T.);
#28022=ORIENTED_EDGE('',*,*,#20829,.T.);
#28023=ORIENTED_EDGE('',*,*,#20830,.T.);
#28024=ORIENTED_EDGE('',*,*,#20831,.T.);
#28025=ORIENTED_EDGE('',*,*,#20832,.T.);
#28026=ORIENTED_EDGE('',*,*,#20248,.T.);
#28027=ORIENTED_EDGE('',*,*,#20830,.F.);
#28028=ORIENTED_EDGE('',*,*,#20675,.T.);
#28029=ORIENTED_EDGE('',*,*,#20827,.F.);
#28030=ORIENTED_EDGE('',*,*,#20679,.F.);
#28031=ORIENTED_EDGE('',*,*,#20833,.T.);
#28032=ORIENTED_EDGE('',*,*,#20828,.F.);
#28033=ORIENTED_EDGE('',*,*,#20663,.F.);
#28034=ORIENTED_EDGE('',*,*,#20834,.F.);
#28035=ORIENTED_EDGE('',*,*,#20835,.F.);
#28036=ORIENTED_EDGE('',*,*,#19733,.F.);
#28037=ORIENTED_EDGE('',*,*,#20836,.F.);
#28038=ORIENTED_EDGE('',*,*,#20837,.F.);
#28039=ORIENTED_EDGE('',*,*,#20672,.F.);
#28040=ORIENTED_EDGE('',*,*,#20667,.F.);
#28041=ORIENTED_EDGE('',*,*,#20838,.T.);
#28042=ORIENTED_EDGE('',*,*,#20250,.T.);
#28043=ORIENTED_EDGE('',*,*,#20839,.T.);
#28044=ORIENTED_EDGE('',*,*,#20840,.T.);
#28045=ORIENTED_EDGE('',*,*,#20841,.T.);
#28046=ORIENTED_EDGE('',*,*,#20842,.T.);
#28047=ORIENTED_EDGE('',*,*,#20843,.T.);
#28048=ORIENTED_EDGE('',*,*,#20844,.T.);
#28049=ORIENTED_EDGE('',*,*,#20843,.F.);
#28050=ORIENTED_EDGE('',*,*,#20845,.T.);
#28051=ORIENTED_EDGE('',*,*,#20838,.F.);
#28052=ORIENTED_EDGE('',*,*,#20846,.T.);
#28053=ORIENTED_EDGE('',*,*,#20847,.T.);
#28054=ORIENTED_EDGE('',*,*,#20848,.T.);
#28055=ORIENTED_EDGE('',*,*,#20849,.T.);
#28056=ORIENTED_EDGE('',*,*,#20848,.F.);
#28057=ORIENTED_EDGE('',*,*,#20850,.T.);
#28058=ORIENTED_EDGE('',*,*,#20841,.F.);
#28059=ORIENTED_EDGE('',*,*,#20845,.F.);
#28060=ORIENTED_EDGE('',*,*,#20851,.T.);
#28061=ORIENTED_EDGE('',*,*,#20852,.F.);
#28062=ORIENTED_EDGE('',*,*,#20251,.T.);
#28063=ORIENTED_EDGE('',*,*,#20842,.F.);
#28064=ORIENTED_EDGE('',*,*,#20853,.F.);
#28065=ORIENTED_EDGE('',*,*,#20854,.F.);
#28066=ORIENTED_EDGE('',*,*,#20851,.F.);
#28067=ORIENTED_EDGE('',*,*,#20850,.F.);
#28068=ORIENTED_EDGE('',*,*,#20855,.T.);
#28069=ORIENTED_EDGE('',*,*,#20856,.T.);
#28070=ORIENTED_EDGE('',*,*,#20853,.T.);
#28071=ORIENTED_EDGE('',*,*,#20847,.F.);
#28072=ORIENTED_EDGE('',*,*,#20857,.F.);
#28073=ORIENTED_EDGE('',*,*,#20858,.F.);
#28074=ORIENTED_EDGE('',*,*,#20855,.F.);
#28075=ORIENTED_EDGE('',*,*,#20859,.T.);
#28076=ORIENTED_EDGE('',*,*,#20854,.T.);
#28077=ORIENTED_EDGE('',*,*,#20860,.T.);
#28078=ORIENTED_EDGE('',*,*,#20861,.T.);
#28079=ORIENTED_EDGE('',*,*,#20862,.T.);
#28080=ORIENTED_EDGE('',*,*,#20863,.T.);
#28081=ORIENTED_EDGE('',*,*,#20864,.T.);
#28082=ORIENTED_EDGE('',*,*,#20252,.T.);
#28083=ORIENTED_EDGE('',*,*,#20862,.F.);
#28084=ORIENTED_EDGE('',*,*,#20852,.T.);
#28085=ORIENTED_EDGE('',*,*,#20859,.F.);
#28086=ORIENTED_EDGE('',*,*,#20856,.F.);
#28087=ORIENTED_EDGE('',*,*,#20865,.T.);
#28088=ORIENTED_EDGE('',*,*,#20860,.F.);
#28089=ORIENTED_EDGE('',*,*,#20840,.F.);
#28090=ORIENTED_EDGE('',*,*,#20866,.F.);
#28091=ORIENTED_EDGE('',*,*,#20867,.F.);
#28092=ORIENTED_EDGE('',*,*,#19729,.F.);
#28093=ORIENTED_EDGE('',*,*,#20868,.F.);
#28094=ORIENTED_EDGE('',*,*,#20869,.F.);
#28095=ORIENTED_EDGE('',*,*,#20849,.F.);
#28096=ORIENTED_EDGE('',*,*,#20844,.F.);
#28097=ORIENTED_EDGE('',*,*,#20833,.F.);
#28098=ORIENTED_EDGE('',*,*,#20681,.T.);
#28099=ORIENTED_EDGE('',*,*,#20870,.T.);
#28100=ORIENTED_EDGE('',*,*,#20871,.T.);
#28101=ORIENTED_EDGE('',*,*,#20829,.F.);
#28102=ORIENTED_EDGE('',*,*,#20871,.F.);
#28103=ORIENTED_EDGE('',*,*,#20872,.F.);
#28104=ORIENTED_EDGE('',*,*,#20873,.F.);
#28105=ORIENTED_EDGE('',*,*,#19731,.F.);
#28106=ORIENTED_EDGE('',*,*,#20874,.F.);
#28107=ORIENTED_EDGE('',*,*,#20875,.F.);
#28108=ORIENTED_EDGE('',*,*,#20831,.F.);
#28109=ORIENTED_EDGE('',*,*,#20876,.T.);
#28110=ORIENTED_EDGE('',*,*,#20826,.T.);
#28111=ORIENTED_EDGE('',*,*,#20877,.T.);
#28112=ORIENTED_EDGE('',*,*,#20878,.T.);
#28113=ORIENTED_EDGE('',*,*,#20822,.F.);
#28114=ORIENTED_EDGE('',*,*,#20879,.T.);
#28115=ORIENTED_EDGE('',*,*,#20880,.T.);
#28116=ORIENTED_EDGE('',*,*,#20825,.T.);
#28117=ORIENTED_EDGE('',*,*,#20880,.F.);
#28118=ORIENTED_EDGE('',*,*,#20881,.T.);
#28119=ORIENTED_EDGE('',*,*,#20877,.F.);
#28120=ORIENTED_EDGE('',*,*,#20882,.T.);
#28121=ORIENTED_EDGE('',*,*,#20883,.T.);
#28122=ORIENTED_EDGE('',*,*,#20884,.T.);
#28123=ORIENTED_EDGE('',*,*,#19737,.T.);
#28124=ORIENTED_EDGE('',*,*,#20882,.F.);
#28125=ORIENTED_EDGE('',*,*,#20824,.T.);
#28126=ORIENTED_EDGE('',*,*,#20876,.F.);
#28127=ORIENTED_EDGE('',*,*,#20812,.F.);
#28128=ORIENTED_EDGE('',*,*,#20885,.F.);
#28129=ORIENTED_EDGE('',*,*,#20886,.F.);
#28130=ORIENTED_EDGE('',*,*,#20244,.F.);
#28131=ORIENTED_EDGE('',*,*,#20887,.F.);
#28132=ORIENTED_EDGE('',*,*,#20888,.F.);
#28133=ORIENTED_EDGE('',*,*,#20821,.F.);
#28134=ORIENTED_EDGE('',*,*,#20816,.F.);
#28135=ORIENTED_EDGE('',*,*,#20805,.F.);
#28136=ORIENTED_EDGE('',*,*,#20702,.T.);
#28137=ORIENTED_EDGE('',*,*,#20889,.T.);
#28138=ORIENTED_EDGE('',*,*,#20890,.T.);
#28139=ORIENTED_EDGE('',*,*,#20801,.F.);
#28140=ORIENTED_EDGE('',*,*,#20890,.F.);
#28141=ORIENTED_EDGE('',*,*,#20891,.F.);
#28142=ORIENTED_EDGE('',*,*,#20892,.F.);
#28143=ORIENTED_EDGE('',*,*,#19739,.F.);
#28144=ORIENTED_EDGE('',*,*,#20893,.F.);
#28145=ORIENTED_EDGE('',*,*,#20894,.F.);
#28146=ORIENTED_EDGE('',*,*,#20803,.F.);
#28147=ORIENTED_EDGE('',*,*,#20895,.T.);
#28148=ORIENTED_EDGE('',*,*,#20216,.T.);
#28149=ORIENTED_EDGE('',*,*,#20896,.T.);
#28150=ORIENTED_EDGE('',*,*,#20897,.T.);
#28151=ORIENTED_EDGE('',*,*,#20898,.T.);
#28152=ORIENTED_EDGE('',*,*,#20899,.T.);
#28153=ORIENTED_EDGE('',*,*,#20900,.T.);
#28154=ORIENTED_EDGE('',*,*,#20901,.T.);
#28155=ORIENTED_EDGE('',*,*,#20900,.F.);
#28156=ORIENTED_EDGE('',*,*,#20902,.T.);
#28157=ORIENTED_EDGE('',*,*,#20895,.F.);
#28158=ORIENTED_EDGE('',*,*,#20903,.T.);
#28159=ORIENTED_EDGE('',*,*,#20904,.T.);
#28160=ORIENTED_EDGE('',*,*,#20905,.T.);
#28161=ORIENTED_EDGE('',*,*,#20906,.T.);
#28162=ORIENTED_EDGE('',*,*,#20905,.F.);
#28163=ORIENTED_EDGE('',*,*,#20907,.T.);
#28164=ORIENTED_EDGE('',*,*,#20898,.F.);
#28165=ORIENTED_EDGE('',*,*,#20902,.F.);
#28166=ORIENTED_EDGE('',*,*,#20908,.T.);
#28167=ORIENTED_EDGE('',*,*,#20909,.F.);
#28168=ORIENTED_EDGE('',*,*,#20217,.T.);
#28169=ORIENTED_EDGE('',*,*,#20899,.F.);
#28170=ORIENTED_EDGE('',*,*,#20910,.F.);
#28171=ORIENTED_EDGE('',*,*,#20911,.F.);
#28172=ORIENTED_EDGE('',*,*,#20908,.F.);
#28173=ORIENTED_EDGE('',*,*,#20907,.F.);
#28174=ORIENTED_EDGE('',*,*,#20912,.T.);
#28175=ORIENTED_EDGE('',*,*,#20913,.T.);
#28176=ORIENTED_EDGE('',*,*,#20910,.T.);
#28177=ORIENTED_EDGE('',*,*,#20904,.F.);
#28178=ORIENTED_EDGE('',*,*,#20914,.F.);
#28179=ORIENTED_EDGE('',*,*,#20915,.F.);
#28180=ORIENTED_EDGE('',*,*,#20912,.F.);
#28181=ORIENTED_EDGE('',*,*,#20916,.T.);
#28182=ORIENTED_EDGE('',*,*,#20212,.T.);
#28183=ORIENTED_EDGE('',*,*,#20917,.T.);
#28184=ORIENTED_EDGE('',*,*,#20918,.T.);
#28185=ORIENTED_EDGE('',*,*,#20919,.T.);
#28186=ORIENTED_EDGE('',*,*,#20920,.T.);
#28187=ORIENTED_EDGE('',*,*,#20921,.T.);
#28188=ORIENTED_EDGE('',*,*,#20922,.T.);
#28189=ORIENTED_EDGE('',*,*,#20921,.F.);
#28190=ORIENTED_EDGE('',*,*,#20923,.T.);
#28191=ORIENTED_EDGE('',*,*,#20916,.F.);
#28192=ORIENTED_EDGE('',*,*,#20924,.T.);
#28193=ORIENTED_EDGE('',*,*,#20925,.T.);
#28194=ORIENTED_EDGE('',*,*,#20926,.T.);
#28195=ORIENTED_EDGE('',*,*,#20927,.T.);
#28196=ORIENTED_EDGE('',*,*,#20926,.F.);
#28197=ORIENTED_EDGE('',*,*,#20928,.T.);
#28198=ORIENTED_EDGE('',*,*,#20919,.F.);
#28199=ORIENTED_EDGE('',*,*,#20923,.F.);
#28200=ORIENTED_EDGE('',*,*,#20929,.T.);
#28201=ORIENTED_EDGE('',*,*,#20930,.F.);
#28202=ORIENTED_EDGE('',*,*,#20213,.T.);
#28203=ORIENTED_EDGE('',*,*,#20920,.F.);
#28204=ORIENTED_EDGE('',*,*,#20931,.F.);
#28205=ORIENTED_EDGE('',*,*,#20932,.F.);
#28206=ORIENTED_EDGE('',*,*,#20929,.F.);
#28207=ORIENTED_EDGE('',*,*,#20928,.F.);
#28208=ORIENTED_EDGE('',*,*,#20933,.T.);
#28209=ORIENTED_EDGE('',*,*,#20934,.T.);
#28210=ORIENTED_EDGE('',*,*,#20931,.T.);
#28211=ORIENTED_EDGE('',*,*,#20925,.F.);
#28212=ORIENTED_EDGE('',*,*,#20935,.F.);
#28213=ORIENTED_EDGE('',*,*,#20936,.F.);
#28214=ORIENTED_EDGE('',*,*,#20933,.F.);
#28215=ORIENTED_EDGE('',*,*,#20937,.T.);
#28216=ORIENTED_EDGE('',*,*,#19747,.T.);
#28217=ORIENTED_EDGE('',*,*,#20938,.T.);
#28218=ORIENTED_EDGE('',*,*,#20939,.T.);
#28219=ORIENTED_EDGE('',*,*,#20940,.T.);
#28220=ORIENTED_EDGE('',*,*,#20941,.T.);
#28221=ORIENTED_EDGE('',*,*,#20942,.T.);
#28222=ORIENTED_EDGE('',*,*,#20943,.T.);
#28223=ORIENTED_EDGE('',*,*,#20942,.F.);
#28224=ORIENTED_EDGE('',*,*,#20944,.T.);
#28225=ORIENTED_EDGE('',*,*,#20937,.F.);
#28226=ORIENTED_EDGE('',*,*,#20945,.T.);
#28227=ORIENTED_EDGE('',*,*,#20946,.T.);
#28228=ORIENTED_EDGE('',*,*,#20947,.T.);
#28229=ORIENTED_EDGE('',*,*,#20948,.T.);
#28230=ORIENTED_EDGE('',*,*,#20947,.F.);
#28231=ORIENTED_EDGE('',*,*,#20949,.T.);
#28232=ORIENTED_EDGE('',*,*,#20940,.F.);
#28233=ORIENTED_EDGE('',*,*,#20944,.F.);
#28234=ORIENTED_EDGE('',*,*,#20950,.T.);
#28235=ORIENTED_EDGE('',*,*,#20951,.F.);
#28236=ORIENTED_EDGE('',*,*,#19748,.T.);
#28237=ORIENTED_EDGE('',*,*,#20941,.F.);
#28238=ORIENTED_EDGE('',*,*,#20952,.F.);
#28239=ORIENTED_EDGE('',*,*,#20953,.F.);
#28240=ORIENTED_EDGE('',*,*,#20950,.F.);
#28241=ORIENTED_EDGE('',*,*,#20954,.T.);
#28242=ORIENTED_EDGE('',*,*,#20234,.T.);
#28243=ORIENTED_EDGE('',*,*,#20955,.T.);
#28244=ORIENTED_EDGE('',*,*,#20956,.T.);
#28245=ORIENTED_EDGE('',*,*,#20957,.T.);
#28246=ORIENTED_EDGE('',*,*,#20958,.T.);
#28247=ORIENTED_EDGE('',*,*,#20959,.T.);
#28248=ORIENTED_EDGE('',*,*,#20960,.T.);
#28249=ORIENTED_EDGE('',*,*,#20959,.F.);
#28250=ORIENTED_EDGE('',*,*,#20961,.T.);
#28251=ORIENTED_EDGE('',*,*,#20954,.F.);
#28252=ORIENTED_EDGE('',*,*,#20962,.T.);
#28253=ORIENTED_EDGE('',*,*,#20963,.T.);
#28254=ORIENTED_EDGE('',*,*,#20964,.T.);
#28255=ORIENTED_EDGE('',*,*,#20965,.T.);
#28256=ORIENTED_EDGE('',*,*,#20964,.F.);
#28257=ORIENTED_EDGE('',*,*,#20966,.T.);
#28258=ORIENTED_EDGE('',*,*,#20957,.F.);
#28259=ORIENTED_EDGE('',*,*,#20961,.F.);
#28260=ORIENTED_EDGE('',*,*,#20967,.T.);
#28261=ORIENTED_EDGE('',*,*,#20968,.F.);
#28262=ORIENTED_EDGE('',*,*,#20235,.T.);
#28263=ORIENTED_EDGE('',*,*,#20958,.F.);
#28264=ORIENTED_EDGE('',*,*,#20969,.F.);
#28265=ORIENTED_EDGE('',*,*,#20970,.F.);
#28266=ORIENTED_EDGE('',*,*,#20967,.F.);
#28267=ORIENTED_EDGE('',*,*,#20966,.F.);
#28268=ORIENTED_EDGE('',*,*,#20971,.T.);
#28269=ORIENTED_EDGE('',*,*,#20972,.T.);
#28270=ORIENTED_EDGE('',*,*,#20969,.T.);
#28271=ORIENTED_EDGE('',*,*,#20963,.F.);
#28272=ORIENTED_EDGE('',*,*,#20973,.F.);
#28273=ORIENTED_EDGE('',*,*,#20974,.F.);
#28274=ORIENTED_EDGE('',*,*,#20971,.F.);
#28275=ORIENTED_EDGE('',*,*,#20975,.T.);
#28276=ORIENTED_EDGE('',*,*,#20970,.T.);
#28277=ORIENTED_EDGE('',*,*,#20976,.T.);
#28278=ORIENTED_EDGE('',*,*,#20977,.T.);
#28279=ORIENTED_EDGE('',*,*,#20978,.T.);
#28280=ORIENTED_EDGE('',*,*,#20979,.T.);
#28281=ORIENTED_EDGE('',*,*,#20980,.T.);
#28282=ORIENTED_EDGE('',*,*,#20236,.T.);
#28283=ORIENTED_EDGE('',*,*,#20978,.F.);
#28284=ORIENTED_EDGE('',*,*,#20968,.T.);
#28285=ORIENTED_EDGE('',*,*,#20975,.F.);
#28286=ORIENTED_EDGE('',*,*,#20972,.F.);
#28287=ORIENTED_EDGE('',*,*,#20981,.T.);
#28288=ORIENTED_EDGE('',*,*,#20976,.F.);
#28289=ORIENTED_EDGE('',*,*,#20956,.F.);
#28290=ORIENTED_EDGE('',*,*,#20982,.F.);
#28291=ORIENTED_EDGE('',*,*,#20983,.F.);
#28292=ORIENTED_EDGE('',*,*,#19745,.F.);
#28293=ORIENTED_EDGE('',*,*,#20984,.F.);
#28294=ORIENTED_EDGE('',*,*,#20985,.F.);
#28295=ORIENTED_EDGE('',*,*,#20965,.F.);
#28296=ORIENTED_EDGE('',*,*,#20960,.F.);
#28297=ORIENTED_EDGE('',*,*,#20986,.T.);
#28298=ORIENTED_EDGE('',*,*,#20953,.T.);
#28299=ORIENTED_EDGE('',*,*,#20987,.T.);
#28300=ORIENTED_EDGE('',*,*,#20988,.T.);
#28301=ORIENTED_EDGE('',*,*,#20949,.F.);
#28302=ORIENTED_EDGE('',*,*,#20989,.T.);
#28303=ORIENTED_EDGE('',*,*,#20990,.T.);
#28304=ORIENTED_EDGE('',*,*,#20952,.T.);
#28305=ORIENTED_EDGE('',*,*,#20990,.F.);
#28306=ORIENTED_EDGE('',*,*,#20991,.T.);
#28307=ORIENTED_EDGE('',*,*,#20987,.F.);
#28308=ORIENTED_EDGE('',*,*,#20992,.T.);
#28309=ORIENTED_EDGE('',*,*,#20993,.T.);
#28310=ORIENTED_EDGE('',*,*,#20994,.T.);
#28311=ORIENTED_EDGE('',*,*,#19749,.T.);
#28312=ORIENTED_EDGE('',*,*,#20992,.F.);
#28313=ORIENTED_EDGE('',*,*,#20951,.T.);
#28314=ORIENTED_EDGE('',*,*,#20986,.F.);
#28315=ORIENTED_EDGE('',*,*,#20939,.F.);
#28316=ORIENTED_EDGE('',*,*,#20995,.F.);
#28317=ORIENTED_EDGE('',*,*,#20996,.F.);
#28318=ORIENTED_EDGE('',*,*,#20232,.F.);
#28319=ORIENTED_EDGE('',*,*,#20997,.F.);
#28320=ORIENTED_EDGE('',*,*,#20998,.F.);
#28321=ORIENTED_EDGE('',*,*,#20948,.F.);
#28322=ORIENTED_EDGE('',*,*,#20943,.F.);
#28323=ORIENTED_EDGE('',*,*,#20999,.T.);
#28324=ORIENTED_EDGE('',*,*,#20204,.T.);
#28325=ORIENTED_EDGE('',*,*,#21000,.T.);
#28326=ORIENTED_EDGE('',*,*,#21001,.T.);
#28327=ORIENTED_EDGE('',*,*,#21002,.T.);
#28328=ORIENTED_EDGE('',*,*,#21003,.T.);
#28329=ORIENTED_EDGE('',*,*,#21004,.T.);
#28330=ORIENTED_EDGE('',*,*,#21005,.T.);
#28331=ORIENTED_EDGE('',*,*,#21004,.F.);
#28332=ORIENTED_EDGE('',*,*,#21006,.T.);
#28333=ORIENTED_EDGE('',*,*,#20999,.F.);
#28334=ORIENTED_EDGE('',*,*,#21007,.T.);
#28335=ORIENTED_EDGE('',*,*,#21008,.T.);
#28336=ORIENTED_EDGE('',*,*,#21009,.T.);
#28337=ORIENTED_EDGE('',*,*,#21010,.T.);
#28338=ORIENTED_EDGE('',*,*,#21009,.F.);
#28339=ORIENTED_EDGE('',*,*,#21011,.T.);
#28340=ORIENTED_EDGE('',*,*,#21002,.F.);
#28341=ORIENTED_EDGE('',*,*,#21006,.F.);
#28342=ORIENTED_EDGE('',*,*,#21012,.T.);
#28343=ORIENTED_EDGE('',*,*,#21013,.F.);
#28344=ORIENTED_EDGE('',*,*,#20205,.T.);
#28345=ORIENTED_EDGE('',*,*,#21003,.F.);
#28346=ORIENTED_EDGE('',*,*,#21014,.F.);
#28347=ORIENTED_EDGE('',*,*,#21015,.F.);
#28348=ORIENTED_EDGE('',*,*,#21012,.F.);
#28349=ORIENTED_EDGE('',*,*,#21011,.F.);
#28350=ORIENTED_EDGE('',*,*,#21016,.T.);
#28351=ORIENTED_EDGE('',*,*,#21017,.T.);
#28352=ORIENTED_EDGE('',*,*,#21014,.T.);
#28353=ORIENTED_EDGE('',*,*,#21008,.F.);
#28354=ORIENTED_EDGE('',*,*,#21018,.F.);
#28355=ORIENTED_EDGE('',*,*,#21019,.F.);
#28356=ORIENTED_EDGE('',*,*,#21016,.F.);
#28357=ORIENTED_EDGE('',*,*,#21020,.T.);
#28358=ORIENTED_EDGE('',*,*,#19771,.T.);
#28359=ORIENTED_EDGE('',*,*,#21021,.T.);
#28360=ORIENTED_EDGE('',*,*,#21022,.T.);
#28361=ORIENTED_EDGE('',*,*,#21023,.T.);
#28362=ORIENTED_EDGE('',*,*,#21024,.T.);
#28363=ORIENTED_EDGE('',*,*,#21025,.T.);
#28364=ORIENTED_EDGE('',*,*,#21026,.T.);
#28365=ORIENTED_EDGE('',*,*,#21025,.F.);
#28366=ORIENTED_EDGE('',*,*,#21027,.T.);
#28367=ORIENTED_EDGE('',*,*,#21020,.F.);
#28368=ORIENTED_EDGE('',*,*,#21028,.T.);
#28369=ORIENTED_EDGE('',*,*,#21029,.T.);
#28370=ORIENTED_EDGE('',*,*,#21030,.T.);
#28371=ORIENTED_EDGE('',*,*,#21031,.T.);
#28372=ORIENTED_EDGE('',*,*,#21030,.F.);
#28373=ORIENTED_EDGE('',*,*,#21032,.T.);
#28374=ORIENTED_EDGE('',*,*,#21023,.F.);
#28375=ORIENTED_EDGE('',*,*,#21027,.F.);
#28376=ORIENTED_EDGE('',*,*,#21033,.T.);
#28377=ORIENTED_EDGE('',*,*,#21034,.F.);
#28378=ORIENTED_EDGE('',*,*,#19772,.T.);
#28379=ORIENTED_EDGE('',*,*,#21024,.F.);
#28380=ORIENTED_EDGE('',*,*,#21035,.F.);
#28381=ORIENTED_EDGE('',*,*,#21036,.F.);
#28382=ORIENTED_EDGE('',*,*,#21033,.F.);
#28383=ORIENTED_EDGE('',*,*,#21037,.T.);
#28384=ORIENTED_EDGE('',*,*,#20932,.T.);
#28385=ORIENTED_EDGE('',*,*,#21038,.T.);
#28386=ORIENTED_EDGE('',*,*,#21039,.T.);
#28387=ORIENTED_EDGE('',*,*,#21040,.T.);
#28388=ORIENTED_EDGE('',*,*,#21041,.T.);
#28389=ORIENTED_EDGE('',*,*,#21042,.T.);
#28390=ORIENTED_EDGE('',*,*,#20214,.T.);
#28391=ORIENTED_EDGE('',*,*,#21040,.F.);
#28392=ORIENTED_EDGE('',*,*,#20930,.T.);
#28393=ORIENTED_EDGE('',*,*,#21037,.F.);
#28394=ORIENTED_EDGE('',*,*,#20934,.F.);
#28395=ORIENTED_EDGE('',*,*,#21043,.T.);
#28396=ORIENTED_EDGE('',*,*,#21038,.F.);
#28397=ORIENTED_EDGE('',*,*,#20918,.F.);
#28398=ORIENTED_EDGE('',*,*,#21044,.F.);
#28399=ORIENTED_EDGE('',*,*,#21045,.F.);
#28400=ORIENTED_EDGE('',*,*,#19769,.F.);
#28401=ORIENTED_EDGE('',*,*,#21046,.F.);
#28402=ORIENTED_EDGE('',*,*,#21047,.F.);
#28403=ORIENTED_EDGE('',*,*,#20927,.F.);
#28404=ORIENTED_EDGE('',*,*,#20922,.F.);
#28405=ORIENTED_EDGE('',*,*,#21048,.T.);
#28406=ORIENTED_EDGE('',*,*,#20911,.T.);
#28407=ORIENTED_EDGE('',*,*,#21049,.T.);
#28408=ORIENTED_EDGE('',*,*,#21050,.T.);
#28409=ORIENTED_EDGE('',*,*,#21051,.T.);
#28410=ORIENTED_EDGE('',*,*,#21052,.T.);
#28411=ORIENTED_EDGE('',*,*,#21053,.T.);
#28412=ORIENTED_EDGE('',*,*,#20218,.T.);
#28413=ORIENTED_EDGE('',*,*,#21051,.F.);
#28414=ORIENTED_EDGE('',*,*,#20909,.T.);
#28415=ORIENTED_EDGE('',*,*,#21048,.F.);
#28416=ORIENTED_EDGE('',*,*,#20913,.F.);
#28417=ORIENTED_EDGE('',*,*,#21054,.T.);
#28418=ORIENTED_EDGE('',*,*,#21049,.F.);
#28419=ORIENTED_EDGE('',*,*,#20897,.F.);
#28420=ORIENTED_EDGE('',*,*,#21055,.F.);
#28421=ORIENTED_EDGE('',*,*,#21056,.F.);
#28422=ORIENTED_EDGE('',*,*,#19765,.F.);
#28423=ORIENTED_EDGE('',*,*,#21057,.F.);
#28424=ORIENTED_EDGE('',*,*,#21058,.F.);
#28425=ORIENTED_EDGE('',*,*,#20906,.F.);
#28426=ORIENTED_EDGE('',*,*,#20901,.F.);
#28427=ORIENTED_EDGE('',*,*,#21059,.T.);
#28428=ORIENTED_EDGE('',*,*,#20222,.T.);
#28429=ORIENTED_EDGE('',*,*,#21060,.T.);
#28430=ORIENTED_EDGE('',*,*,#21061,.T.);
#28431=ORIENTED_EDGE('',*,*,#21062,.T.);
#28432=ORIENTED_EDGE('',*,*,#21063,.T.);
#28433=ORIENTED_EDGE('',*,*,#21064,.T.);
#28434=ORIENTED_EDGE('',*,*,#21065,.T.);
#28435=ORIENTED_EDGE('',*,*,#21064,.F.);
#28436=ORIENTED_EDGE('',*,*,#21066,.T.);
#28437=ORIENTED_EDGE('',*,*,#21059,.F.);
#28438=ORIENTED_EDGE('',*,*,#21067,.T.);
#28439=ORIENTED_EDGE('',*,*,#21068,.T.);
#28440=ORIENTED_EDGE('',*,*,#21069,.T.);
#28441=ORIENTED_EDGE('',*,*,#21070,.T.);
#28442=ORIENTED_EDGE('',*,*,#21069,.F.);
#28443=ORIENTED_EDGE('',*,*,#21071,.T.);
#28444=ORIENTED_EDGE('',*,*,#21062,.F.);
#28445=ORIENTED_EDGE('',*,*,#21066,.F.);
#28446=ORIENTED_EDGE('',*,*,#21072,.T.);
#28447=ORIENTED_EDGE('',*,*,#21073,.F.);
#28448=ORIENTED_EDGE('',*,*,#20223,.T.);
#28449=ORIENTED_EDGE('',*,*,#21063,.F.);
#28450=ORIENTED_EDGE('',*,*,#21074,.F.);
#28451=ORIENTED_EDGE('',*,*,#21075,.F.);
#28452=ORIENTED_EDGE('',*,*,#21072,.F.);
#28453=ORIENTED_EDGE('',*,*,#21071,.F.);
#28454=ORIENTED_EDGE('',*,*,#21076,.T.);
#28455=ORIENTED_EDGE('',*,*,#21077,.T.);
#28456=ORIENTED_EDGE('',*,*,#21074,.T.);
#28457=ORIENTED_EDGE('',*,*,#21068,.F.);
#28458=ORIENTED_EDGE('',*,*,#21078,.F.);
#28459=ORIENTED_EDGE('',*,*,#21079,.F.);
#28460=ORIENTED_EDGE('',*,*,#21076,.F.);
#28461=ORIENTED_EDGE('',*,*,#21080,.T.);
#28462=ORIENTED_EDGE('',*,*,#20291,.T.);
#28463=ORIENTED_EDGE('',*,*,#21081,.T.);
#28464=ORIENTED_EDGE('',*,*,#21082,.T.);
#28465=ORIENTED_EDGE('',*,*,#21083,.T.);
#28466=ORIENTED_EDGE('',*,*,#21084,.T.);
#28467=ORIENTED_EDGE('',*,*,#21085,.T.);
#28468=ORIENTED_EDGE('',*,*,#20228,.T.);
#28469=ORIENTED_EDGE('',*,*,#21083,.F.);
#28470=ORIENTED_EDGE('',*,*,#20289,.T.);
#28471=ORIENTED_EDGE('',*,*,#21080,.F.);
#28472=ORIENTED_EDGE('',*,*,#20293,.F.);
#28473=ORIENTED_EDGE('',*,*,#21086,.T.);
#28474=ORIENTED_EDGE('',*,*,#21081,.F.);
#28475=ORIENTED_EDGE('',*,*,#21086,.F.);
#28476=ORIENTED_EDGE('',*,*,#20295,.T.);
#28477=ORIENTED_EDGE('',*,*,#21087,.T.);
#28478=ORIENTED_EDGE('',*,*,#21088,.T.);
#28479=ORIENTED_EDGE('',*,*,#21082,.F.);
#28480=ORIENTED_EDGE('',*,*,#21088,.F.);
#28481=ORIENTED_EDGE('',*,*,#21089,.F.);
#28482=ORIENTED_EDGE('',*,*,#21090,.F.);
#28483=ORIENTED_EDGE('',*,*,#19751,.F.);
#28484=ORIENTED_EDGE('',*,*,#21091,.F.);
#28485=ORIENTED_EDGE('',*,*,#21092,.F.);
#28486=ORIENTED_EDGE('',*,*,#21084,.F.);
#28487=ORIENTED_EDGE('',*,*,#21093,.T.);
#28488=ORIENTED_EDGE('',*,*,#21075,.T.);
#28489=ORIENTED_EDGE('',*,*,#21094,.T.);
#28490=ORIENTED_EDGE('',*,*,#21095,.T.);
#28491=ORIENTED_EDGE('',*,*,#21096,.T.);
#28492=ORIENTED_EDGE('',*,*,#21097,.T.);
#28493=ORIENTED_EDGE('',*,*,#21098,.T.);
#28494=ORIENTED_EDGE('',*,*,#20224,.T.);
#28495=ORIENTED_EDGE('',*,*,#21096,.F.);
#28496=ORIENTED_EDGE('',*,*,#21073,.T.);
#28497=ORIENTED_EDGE('',*,*,#21093,.F.);
#28498=ORIENTED_EDGE('',*,*,#21077,.F.);
#28499=ORIENTED_EDGE('',*,*,#21099,.T.);
#28500=ORIENTED_EDGE('',*,*,#21094,.F.);
#28501=ORIENTED_EDGE('',*,*,#21061,.F.);
#28502=ORIENTED_EDGE('',*,*,#21100,.F.);
#28503=ORIENTED_EDGE('',*,*,#21101,.F.);
#28504=ORIENTED_EDGE('',*,*,#19757,.F.);
#28505=ORIENTED_EDGE('',*,*,#21102,.F.);
#28506=ORIENTED_EDGE('',*,*,#21103,.F.);
#28507=ORIENTED_EDGE('',*,*,#21070,.F.);
#28508=ORIENTED_EDGE('',*,*,#21065,.F.);
#28509=ORIENTED_EDGE('',*,*,#21054,.F.);
#28510=ORIENTED_EDGE('',*,*,#20915,.T.);
#28511=ORIENTED_EDGE('',*,*,#21104,.T.);
#28512=ORIENTED_EDGE('',*,*,#21105,.T.);
#28513=ORIENTED_EDGE('',*,*,#21050,.F.);
#28514=ORIENTED_EDGE('',*,*,#21105,.F.);
#28515=ORIENTED_EDGE('',*,*,#21106,.F.);
#28516=ORIENTED_EDGE('',*,*,#21107,.F.);
#28517=ORIENTED_EDGE('',*,*,#19763,.F.);
#28518=ORIENTED_EDGE('',*,*,#21108,.F.);
#28519=ORIENTED_EDGE('',*,*,#21109,.F.);
#28520=ORIENTED_EDGE('',*,*,#21052,.F.);
#28521=ORIENTED_EDGE('',*,*,#21043,.F.);
#28522=ORIENTED_EDGE('',*,*,#20936,.T.);
#28523=ORIENTED_EDGE('',*,*,#21110,.T.);
#28524=ORIENTED_EDGE('',*,*,#21111,.T.);
#28525=ORIENTED_EDGE('',*,*,#21039,.F.);
#28526=ORIENTED_EDGE('',*,*,#21111,.F.);
#28527=ORIENTED_EDGE('',*,*,#21112,.F.);
#28528=ORIENTED_EDGE('',*,*,#21113,.F.);
#28529=ORIENTED_EDGE('',*,*,#19767,.F.);
#28530=ORIENTED_EDGE('',*,*,#21114,.F.);
#28531=ORIENTED_EDGE('',*,*,#21115,.F.);
#28532=ORIENTED_EDGE('',*,*,#21041,.F.);
#28533=ORIENTED_EDGE('',*,*,#21116,.T.);
#28534=ORIENTED_EDGE('',*,*,#21036,.T.);
#28535=ORIENTED_EDGE('',*,*,#21117,.T.);
#28536=ORIENTED_EDGE('',*,*,#21118,.T.);
#28537=ORIENTED_EDGE('',*,*,#21032,.F.);
#28538=ORIENTED_EDGE('',*,*,#21119,.T.);
#28539=ORIENTED_EDGE('',*,*,#21120,.T.);
#28540=ORIENTED_EDGE('',*,*,#21035,.T.);
#28541=ORIENTED_EDGE('',*,*,#21120,.F.);
#28542=ORIENTED_EDGE('',*,*,#21121,.T.);
#28543=ORIENTED_EDGE('',*,*,#21117,.F.);
#28544=ORIENTED_EDGE('',*,*,#21122,.T.);
#28545=ORIENTED_EDGE('',*,*,#21123,.T.);
#28546=ORIENTED_EDGE('',*,*,#21124,.T.);
#28547=ORIENTED_EDGE('',*,*,#19773,.T.);
#28548=ORIENTED_EDGE('',*,*,#21122,.F.);
#28549=ORIENTED_EDGE('',*,*,#21034,.T.);
#28550=ORIENTED_EDGE('',*,*,#21116,.F.);
#28551=ORIENTED_EDGE('',*,*,#21022,.F.);
#28552=ORIENTED_EDGE('',*,*,#21125,.F.);
#28553=ORIENTED_EDGE('',*,*,#21126,.F.);
#28554=ORIENTED_EDGE('',*,*,#20210,.F.);
#28555=ORIENTED_EDGE('',*,*,#21127,.F.);
#28556=ORIENTED_EDGE('',*,*,#21128,.F.);
#28557=ORIENTED_EDGE('',*,*,#21031,.F.);
#28558=ORIENTED_EDGE('',*,*,#21026,.F.);
#28559=ORIENTED_EDGE('',*,*,#21129,.T.);
#28560=ORIENTED_EDGE('',*,*,#21015,.T.);
#28561=ORIENTED_EDGE('',*,*,#21130,.T.);
#28562=ORIENTED_EDGE('',*,*,#21131,.T.);
#28563=ORIENTED_EDGE('',*,*,#21132,.T.);
#28564=ORIENTED_EDGE('',*,*,#21133,.T.);
#28565=ORIENTED_EDGE('',*,*,#21134,.T.);
#28566=ORIENTED_EDGE('',*,*,#20206,.T.);
#28567=ORIENTED_EDGE('',*,*,#21132,.F.);
#28568=ORIENTED_EDGE('',*,*,#21013,.T.);
#28569=ORIENTED_EDGE('',*,*,#21129,.F.);
#28570=ORIENTED_EDGE('',*,*,#21017,.F.);
#28571=ORIENTED_EDGE('',*,*,#21135,.T.);
#28572=ORIENTED_EDGE('',*,*,#21130,.F.);
#28573=ORIENTED_EDGE('',*,*,#21001,.F.);
#28574=ORIENTED_EDGE('',*,*,#21136,.F.);
#28575=ORIENTED_EDGE('',*,*,#21137,.F.);
#28576=ORIENTED_EDGE('',*,*,#19777,.F.);
#28577=ORIENTED_EDGE('',*,*,#21138,.F.);
#28578=ORIENTED_EDGE('',*,*,#21139,.F.);
#28579=ORIENTED_EDGE('',*,*,#21010,.F.);
#28580=ORIENTED_EDGE('',*,*,#21005,.F.);
#28581=ORIENTED_EDGE('',*,*,#21140,.T.);
#28582=ORIENTED_EDGE('',*,*,#20183,.T.);
#28583=ORIENTED_EDGE('',*,*,#21141,.T.);
#28584=ORIENTED_EDGE('',*,*,#21142,.T.);
#28585=ORIENTED_EDGE('',*,*,#21143,.T.);
#28586=ORIENTED_EDGE('',*,*,#21144,.T.);
#28587=ORIENTED_EDGE('',*,*,#21145,.T.);
#28588=ORIENTED_EDGE('',*,*,#21146,.T.);
#28589=ORIENTED_EDGE('',*,*,#21145,.F.);
#28590=ORIENTED_EDGE('',*,*,#21147,.T.);
#28591=ORIENTED_EDGE('',*,*,#21140,.F.);
#28592=ORIENTED_EDGE('',*,*,#21148,.T.);
#28593=ORIENTED_EDGE('',*,*,#21149,.T.);
#28594=ORIENTED_EDGE('',*,*,#21150,.T.);
#28595=ORIENTED_EDGE('',*,*,#21151,.T.);
#28596=ORIENTED_EDGE('',*,*,#21150,.F.);
#28597=ORIENTED_EDGE('',*,*,#21152,.T.);
#28598=ORIENTED_EDGE('',*,*,#21143,.F.);
#28599=ORIENTED_EDGE('',*,*,#21147,.F.);
#28600=ORIENTED_EDGE('',*,*,#21153,.T.);
#28601=ORIENTED_EDGE('',*,*,#21154,.F.);
#28602=ORIENTED_EDGE('',*,*,#20184,.T.);
#28603=ORIENTED_EDGE('',*,*,#21144,.F.);
#28604=ORIENTED_EDGE('',*,*,#21155,.F.);
#28605=ORIENTED_EDGE('',*,*,#21156,.F.);
#28606=ORIENTED_EDGE('',*,*,#21153,.F.);
#28607=ORIENTED_EDGE('',*,*,#21152,.F.);
#28608=ORIENTED_EDGE('',*,*,#21157,.T.);
#28609=ORIENTED_EDGE('',*,*,#21158,.T.);
#28610=ORIENTED_EDGE('',*,*,#21155,.T.);
#28611=ORIENTED_EDGE('',*,*,#21149,.F.);
#28612=ORIENTED_EDGE('',*,*,#21159,.F.);
#28613=ORIENTED_EDGE('',*,*,#21160,.F.);
#28614=ORIENTED_EDGE('',*,*,#21157,.F.);
#28615=ORIENTED_EDGE('',*,*,#21161,.T.);
#28616=ORIENTED_EDGE('',*,*,#20270,.T.);
#28617=ORIENTED_EDGE('',*,*,#21162,.T.);
#28618=ORIENTED_EDGE('',*,*,#21163,.T.);
#28619=ORIENTED_EDGE('',*,*,#21164,.T.);
#28620=ORIENTED_EDGE('',*,*,#21165,.T.);
#28621=ORIENTED_EDGE('',*,*,#21166,.T.);
#28622=ORIENTED_EDGE('',*,*,#20202,.T.);
#28623=ORIENTED_EDGE('',*,*,#21164,.F.);
#28624=ORIENTED_EDGE('',*,*,#20268,.T.);
#28625=ORIENTED_EDGE('',*,*,#21161,.F.);
#28626=ORIENTED_EDGE('',*,*,#20272,.F.);
#28627=ORIENTED_EDGE('',*,*,#21167,.T.);
#28628=ORIENTED_EDGE('',*,*,#21162,.F.);
#28629=ORIENTED_EDGE('',*,*,#21167,.F.);
#28630=ORIENTED_EDGE('',*,*,#20274,.T.);
#28631=ORIENTED_EDGE('',*,*,#21168,.T.);
#28632=ORIENTED_EDGE('',*,*,#21169,.T.);
#28633=ORIENTED_EDGE('',*,*,#21163,.F.);
#28634=ORIENTED_EDGE('',*,*,#21169,.F.);
#28635=ORIENTED_EDGE('',*,*,#21170,.F.);
#28636=ORIENTED_EDGE('',*,*,#21171,.F.);
#28637=ORIENTED_EDGE('',*,*,#19779,.F.);
#28638=ORIENTED_EDGE('',*,*,#21172,.F.);
#28639=ORIENTED_EDGE('',*,*,#21173,.F.);
#28640=ORIENTED_EDGE('',*,*,#21165,.F.);
#28641=ORIENTED_EDGE('',*,*,#21174,.T.);
#28642=ORIENTED_EDGE('',*,*,#20173,.T.);
#28643=ORIENTED_EDGE('',*,*,#21175,.T.);
#28644=ORIENTED_EDGE('',*,*,#21176,.T.);
#28645=ORIENTED_EDGE('',*,*,#21177,.T.);
#28646=ORIENTED_EDGE('',*,*,#21178,.T.);
#28647=ORIENTED_EDGE('',*,*,#21179,.T.);
#28648=ORIENTED_EDGE('',*,*,#21180,.T.);
#28649=ORIENTED_EDGE('',*,*,#21179,.F.);
#28650=ORIENTED_EDGE('',*,*,#21181,.T.);
#28651=ORIENTED_EDGE('',*,*,#21174,.F.);
#28652=ORIENTED_EDGE('',*,*,#21182,.T.);
#28653=ORIENTED_EDGE('',*,*,#21183,.T.);
#28654=ORIENTED_EDGE('',*,*,#21184,.T.);
#28655=ORIENTED_EDGE('',*,*,#21185,.T.);
#28656=ORIENTED_EDGE('',*,*,#21184,.F.);
#28657=ORIENTED_EDGE('',*,*,#21186,.T.);
#28658=ORIENTED_EDGE('',*,*,#21177,.F.);
#28659=ORIENTED_EDGE('',*,*,#21181,.F.);
#28660=ORIENTED_EDGE('',*,*,#21187,.T.);
#28661=ORIENTED_EDGE('',*,*,#21188,.F.);
#28662=ORIENTED_EDGE('',*,*,#20174,.T.);
#28663=ORIENTED_EDGE('',*,*,#21178,.F.);
#28664=ORIENTED_EDGE('',*,*,#21189,.F.);
#28665=ORIENTED_EDGE('',*,*,#21190,.F.);
#28666=ORIENTED_EDGE('',*,*,#21187,.F.);
#28667=ORIENTED_EDGE('',*,*,#21186,.F.);
#28668=ORIENTED_EDGE('',*,*,#21191,.T.);
#28669=ORIENTED_EDGE('',*,*,#21192,.T.);
#28670=ORIENTED_EDGE('',*,*,#21189,.T.);
#28671=ORIENTED_EDGE('',*,*,#21183,.F.);
#28672=ORIENTED_EDGE('',*,*,#21193,.F.);
#28673=ORIENTED_EDGE('',*,*,#21194,.F.);
#28674=ORIENTED_EDGE('',*,*,#21191,.F.);
#28675=ORIENTED_EDGE('',*,*,#21195,.T.);
#28676=ORIENTED_EDGE('',*,*,#20169,.T.);
#28677=ORIENTED_EDGE('',*,*,#21196,.T.);
#28678=ORIENTED_EDGE('',*,*,#21197,.T.);
#28679=ORIENTED_EDGE('',*,*,#21198,.T.);
#28680=ORIENTED_EDGE('',*,*,#21199,.T.);
#28681=ORIENTED_EDGE('',*,*,#21200,.T.);
#28682=ORIENTED_EDGE('',*,*,#21201,.T.);
#28683=ORIENTED_EDGE('',*,*,#21200,.F.);
#28684=ORIENTED_EDGE('',*,*,#21202,.T.);
#28685=ORIENTED_EDGE('',*,*,#21195,.F.);
#28686=ORIENTED_EDGE('',*,*,#21203,.T.);
#28687=ORIENTED_EDGE('',*,*,#21204,.T.);
#28688=ORIENTED_EDGE('',*,*,#21205,.T.);
#28689=ORIENTED_EDGE('',*,*,#21206,.T.);
#28690=ORIENTED_EDGE('',*,*,#21205,.F.);
#28691=ORIENTED_EDGE('',*,*,#21207,.T.);
#28692=ORIENTED_EDGE('',*,*,#21198,.F.);
#28693=ORIENTED_EDGE('',*,*,#21202,.F.);
#28694=ORIENTED_EDGE('',*,*,#21208,.T.);
#28695=ORIENTED_EDGE('',*,*,#21209,.F.);
#28696=ORIENTED_EDGE('',*,*,#20170,.T.);
#28697=ORIENTED_EDGE('',*,*,#21199,.F.);
#28698=ORIENTED_EDGE('',*,*,#21210,.F.);
#28699=ORIENTED_EDGE('',*,*,#21211,.F.);
#28700=ORIENTED_EDGE('',*,*,#21208,.F.);
#28701=ORIENTED_EDGE('',*,*,#21207,.F.);
#28702=ORIENTED_EDGE('',*,*,#21212,.T.);
#28703=ORIENTED_EDGE('',*,*,#21213,.T.);
#28704=ORIENTED_EDGE('',*,*,#21210,.T.);
#28705=ORIENTED_EDGE('',*,*,#21204,.F.);
#28706=ORIENTED_EDGE('',*,*,#21214,.F.);
#28707=ORIENTED_EDGE('',*,*,#21215,.F.);
#28708=ORIENTED_EDGE('',*,*,#21212,.F.);
#28709=ORIENTED_EDGE('',*,*,#21216,.T.);
#28710=ORIENTED_EDGE('',*,*,#21156,.T.);
#28711=ORIENTED_EDGE('',*,*,#21217,.T.);
#28712=ORIENTED_EDGE('',*,*,#21218,.T.);
#28713=ORIENTED_EDGE('',*,*,#21219,.T.);
#28714=ORIENTED_EDGE('',*,*,#21220,.T.);
#28715=ORIENTED_EDGE('',*,*,#21221,.T.);
#28716=ORIENTED_EDGE('',*,*,#20185,.T.);
#28717=ORIENTED_EDGE('',*,*,#21219,.F.);
#28718=ORIENTED_EDGE('',*,*,#21154,.T.);
#28719=ORIENTED_EDGE('',*,*,#21216,.F.);
#28720=ORIENTED_EDGE('',*,*,#21158,.F.);
#28721=ORIENTED_EDGE('',*,*,#21222,.T.);
#28722=ORIENTED_EDGE('',*,*,#21217,.F.);
#28723=ORIENTED_EDGE('',*,*,#21142,.F.);
#28724=ORIENTED_EDGE('',*,*,#21223,.F.);
#28725=ORIENTED_EDGE('',*,*,#21224,.F.);
#28726=ORIENTED_EDGE('',*,*,#19801,.F.);
#28727=ORIENTED_EDGE('',*,*,#21225,.F.);
#28728=ORIENTED_EDGE('',*,*,#21226,.F.);
#28729=ORIENTED_EDGE('',*,*,#21151,.F.);
#28730=ORIENTED_EDGE('',*,*,#21146,.F.);
#28731=ORIENTED_EDGE('',*,*,#21227,.T.);
#28732=ORIENTED_EDGE('',*,*,#19795,.T.);
#28733=ORIENTED_EDGE('',*,*,#21228,.T.);
#28734=ORIENTED_EDGE('',*,*,#21229,.T.);
#28735=ORIENTED_EDGE('',*,*,#21230,.T.);
#28736=ORIENTED_EDGE('',*,*,#21231,.T.);
#28737=ORIENTED_EDGE('',*,*,#21232,.T.);
#28738=ORIENTED_EDGE('',*,*,#21233,.T.);
#28739=ORIENTED_EDGE('',*,*,#21232,.F.);
#28740=ORIENTED_EDGE('',*,*,#21234,.T.);
#28741=ORIENTED_EDGE('',*,*,#21227,.F.);
#28742=ORIENTED_EDGE('',*,*,#21235,.T.);
#28743=ORIENTED_EDGE('',*,*,#21236,.T.);
#28744=ORIENTED_EDGE('',*,*,#21237,.T.);
#28745=ORIENTED_EDGE('',*,*,#21238,.T.);
#28746=ORIENTED_EDGE('',*,*,#21237,.F.);
#28747=ORIENTED_EDGE('',*,*,#21239,.T.);
#28748=ORIENTED_EDGE('',*,*,#21230,.F.);
#28749=ORIENTED_EDGE('',*,*,#21234,.F.);
#28750=ORIENTED_EDGE('',*,*,#21240,.T.);
#28751=ORIENTED_EDGE('',*,*,#21241,.F.);
#28752=ORIENTED_EDGE('',*,*,#19796,.T.);
#28753=ORIENTED_EDGE('',*,*,#21231,.F.);
#28754=ORIENTED_EDGE('',*,*,#21242,.F.);
#28755=ORIENTED_EDGE('',*,*,#21243,.F.);
#28756=ORIENTED_EDGE('',*,*,#21240,.F.);
#28757=ORIENTED_EDGE('',*,*,#21244,.T.);
#28758=ORIENTED_EDGE('',*,*,#20191,.T.);
#28759=ORIENTED_EDGE('',*,*,#21245,.T.);
#28760=ORIENTED_EDGE('',*,*,#21246,.T.);
#28761=ORIENTED_EDGE('',*,*,#21247,.T.);
#28762=ORIENTED_EDGE('',*,*,#21248,.T.);
#28763=ORIENTED_EDGE('',*,*,#21249,.T.);
#28764=ORIENTED_EDGE('',*,*,#21250,.T.);
#28765=ORIENTED_EDGE('',*,*,#21249,.F.);
#28766=ORIENTED_EDGE('',*,*,#21251,.T.);
#28767=ORIENTED_EDGE('',*,*,#21244,.F.);
#28768=ORIENTED_EDGE('',*,*,#21252,.T.);
#28769=ORIENTED_EDGE('',*,*,#21253,.T.);
#28770=ORIENTED_EDGE('',*,*,#21254,.T.);
#28771=ORIENTED_EDGE('',*,*,#21255,.T.);
#28772=ORIENTED_EDGE('',*,*,#21254,.F.);
#28773=ORIENTED_EDGE('',*,*,#21256,.T.);
#28774=ORIENTED_EDGE('',*,*,#21247,.F.);
#28775=ORIENTED_EDGE('',*,*,#21251,.F.);
#28776=ORIENTED_EDGE('',*,*,#21257,.T.);
#28777=ORIENTED_EDGE('',*,*,#21258,.F.);
#28778=ORIENTED_EDGE('',*,*,#20192,.T.);
#28779=ORIENTED_EDGE('',*,*,#21248,.F.);
#28780=ORIENTED_EDGE('',*,*,#21259,.F.);
#28781=ORIENTED_EDGE('',*,*,#21260,.F.);
#28782=ORIENTED_EDGE('',*,*,#21257,.F.);
#28783=ORIENTED_EDGE('',*,*,#21256,.F.);
#28784=ORIENTED_EDGE('',*,*,#21261,.T.);
#28785=ORIENTED_EDGE('',*,*,#21262,.T.);
#28786=ORIENTED_EDGE('',*,*,#21259,.T.);
#28787=ORIENTED_EDGE('',*,*,#21253,.F.);
#28788=ORIENTED_EDGE('',*,*,#21263,.F.);
#28789=ORIENTED_EDGE('',*,*,#21264,.F.);
#28790=ORIENTED_EDGE('',*,*,#21261,.F.);
#28791=ORIENTED_EDGE('',*,*,#21265,.T.);
#28792=ORIENTED_EDGE('',*,*,#20062,.T.);
#28793=ORIENTED_EDGE('',*,*,#21266,.T.);
#28794=ORIENTED_EDGE('',*,*,#20070,.T.);
#28795=ORIENTED_EDGE('',*,*,#21267,.T.);
#28796=ORIENTED_EDGE('',*,*,#20069,.T.);
#28797=ORIENTED_EDGE('',*,*,#21268,.T.);
#28798=ORIENTED_EDGE('',*,*,#20195,.T.);
#28799=ORIENTED_EDGE('',*,*,#21267,.F.);
#28800=ORIENTED_EDGE('',*,*,#20059,.T.);
#28801=ORIENTED_EDGE('',*,*,#21265,.F.);
#28802=ORIENTED_EDGE('',*,*,#20064,.F.);
#28803=ORIENTED_EDGE('',*,*,#20067,.T.);
#28804=ORIENTED_EDGE('',*,*,#21266,.F.);
#28805=ORIENTED_EDGE('',*,*,#21269,.T.);
#28806=ORIENTED_EDGE('',*,*,#19783,.T.);
#28807=ORIENTED_EDGE('',*,*,#21270,.T.);
#28808=ORIENTED_EDGE('',*,*,#21271,.T.);
#28809=ORIENTED_EDGE('',*,*,#21272,.T.);
#28810=ORIENTED_EDGE('',*,*,#21273,.T.);
#28811=ORIENTED_EDGE('',*,*,#21274,.T.);
#28812=ORIENTED_EDGE('',*,*,#21275,.T.);
#28813=ORIENTED_EDGE('',*,*,#21274,.F.);
#28814=ORIENTED_EDGE('',*,*,#21276,.T.);
#28815=ORIENTED_EDGE('',*,*,#21269,.F.);
#28816=ORIENTED_EDGE('',*,*,#21277,.T.);
#28817=ORIENTED_EDGE('',*,*,#21278,.T.);
#28818=ORIENTED_EDGE('',*,*,#21279,.T.);
#28819=ORIENTED_EDGE('',*,*,#21280,.T.);
#28820=ORIENTED_EDGE('',*,*,#21279,.F.);
#28821=ORIENTED_EDGE('',*,*,#21281,.T.);
#28822=ORIENTED_EDGE('',*,*,#21272,.F.);
#28823=ORIENTED_EDGE('',*,*,#21276,.F.);
#28824=ORIENTED_EDGE('',*,*,#21282,.T.);
#28825=ORIENTED_EDGE('',*,*,#21283,.F.);
#28826=ORIENTED_EDGE('',*,*,#19784,.T.);
#28827=ORIENTED_EDGE('',*,*,#21273,.F.);
#28828=ORIENTED_EDGE('',*,*,#21284,.F.);
#28829=ORIENTED_EDGE('',*,*,#21285,.F.);
#28830=ORIENTED_EDGE('',*,*,#21282,.F.);
#28831=ORIENTED_EDGE('',*,*,#21286,.T.);
#28832=ORIENTED_EDGE('',*,*,#21285,.T.);
#28833=ORIENTED_EDGE('',*,*,#21287,.T.);
#28834=ORIENTED_EDGE('',*,*,#21288,.T.);
#28835=ORIENTED_EDGE('',*,*,#21281,.F.);
#28836=ORIENTED_EDGE('',*,*,#21289,.T.);
#28837=ORIENTED_EDGE('',*,*,#21290,.T.);
#28838=ORIENTED_EDGE('',*,*,#21284,.T.);
#28839=ORIENTED_EDGE('',*,*,#21290,.F.);
#28840=ORIENTED_EDGE('',*,*,#21291,.T.);
#28841=ORIENTED_EDGE('',*,*,#21287,.F.);
#28842=ORIENTED_EDGE('',*,*,#21292,.T.);
#28843=ORIENTED_EDGE('',*,*,#21293,.T.);
#28844=ORIENTED_EDGE('',*,*,#21294,.T.);
#28845=ORIENTED_EDGE('',*,*,#19785,.T.);
#28846=ORIENTED_EDGE('',*,*,#21292,.F.);
#28847=ORIENTED_EDGE('',*,*,#21283,.T.);
#28848=ORIENTED_EDGE('',*,*,#21286,.F.);
#28849=ORIENTED_EDGE('',*,*,#21271,.F.);
#28850=ORIENTED_EDGE('',*,*,#21295,.F.);
#28851=ORIENTED_EDGE('',*,*,#21296,.F.);
#28852=ORIENTED_EDGE('',*,*,#20199,.F.);
#28853=ORIENTED_EDGE('',*,*,#21297,.F.);
#28854=ORIENTED_EDGE('',*,*,#21298,.F.);
#28855=ORIENTED_EDGE('',*,*,#21280,.F.);
#28856=ORIENTED_EDGE('',*,*,#21275,.F.);
#28857=ORIENTED_EDGE('',*,*,#21299,.T.);
#28858=ORIENTED_EDGE('',*,*,#21260,.T.);
#28859=ORIENTED_EDGE('',*,*,#21300,.T.);
#28860=ORIENTED_EDGE('',*,*,#21301,.T.);
#28861=ORIENTED_EDGE('',*,*,#21302,.T.);
#28862=ORIENTED_EDGE('',*,*,#21303,.T.);
#28863=ORIENTED_EDGE('',*,*,#21304,.T.);
#28864=ORIENTED_EDGE('',*,*,#20193,.T.);
#28865=ORIENTED_EDGE('',*,*,#21302,.F.);
#28866=ORIENTED_EDGE('',*,*,#21258,.T.);
#28867=ORIENTED_EDGE('',*,*,#21299,.F.);
#28868=ORIENTED_EDGE('',*,*,#21262,.F.);
#28869=ORIENTED_EDGE('',*,*,#21305,.T.);
#28870=ORIENTED_EDGE('',*,*,#21300,.F.);
#28871=ORIENTED_EDGE('',*,*,#21246,.F.);
#28872=ORIENTED_EDGE('',*,*,#21306,.F.);
#28873=ORIENTED_EDGE('',*,*,#21307,.F.);
#28874=ORIENTED_EDGE('',*,*,#19793,.F.);
#28875=ORIENTED_EDGE('',*,*,#21308,.F.);
#28876=ORIENTED_EDGE('',*,*,#21309,.F.);
#28877=ORIENTED_EDGE('',*,*,#21255,.F.);
#28878=ORIENTED_EDGE('',*,*,#21250,.F.);
#28879=ORIENTED_EDGE('',*,*,#21310,.T.);
#28880=ORIENTED_EDGE('',*,*,#21243,.T.);
#28881=ORIENTED_EDGE('',*,*,#21311,.T.);
#28882=ORIENTED_EDGE('',*,*,#21312,.T.);
#28883=ORIENTED_EDGE('',*,*,#21239,.F.);
#28884=ORIENTED_EDGE('',*,*,#21313,.T.);
#28885=ORIENTED_EDGE('',*,*,#21314,.T.);
#28886=ORIENTED_EDGE('',*,*,#21242,.T.);
#28887=ORIENTED_EDGE('',*,*,#21314,.F.);
#28888=ORIENTED_EDGE('',*,*,#21315,.T.);
#28889=ORIENTED_EDGE('',*,*,#21311,.F.);
#28890=ORIENTED_EDGE('',*,*,#21316,.T.);
#28891=ORIENTED_EDGE('',*,*,#21317,.T.);
#28892=ORIENTED_EDGE('',*,*,#21318,.T.);
#28893=ORIENTED_EDGE('',*,*,#19797,.T.);
#28894=ORIENTED_EDGE('',*,*,#21316,.F.);
#28895=ORIENTED_EDGE('',*,*,#21241,.T.);
#28896=ORIENTED_EDGE('',*,*,#21310,.F.);
#28897=ORIENTED_EDGE('',*,*,#21229,.F.);
#28898=ORIENTED_EDGE('',*,*,#21319,.F.);
#28899=ORIENTED_EDGE('',*,*,#21320,.F.);
#28900=ORIENTED_EDGE('',*,*,#20189,.F.);
#28901=ORIENTED_EDGE('',*,*,#21321,.F.);
#28902=ORIENTED_EDGE('',*,*,#21322,.F.);
#28903=ORIENTED_EDGE('',*,*,#21238,.F.);
#28904=ORIENTED_EDGE('',*,*,#21233,.F.);
#28905=ORIENTED_EDGE('',*,*,#21222,.F.);
#28906=ORIENTED_EDGE('',*,*,#21160,.T.);
#28907=ORIENTED_EDGE('',*,*,#21323,.T.);
#28908=ORIENTED_EDGE('',*,*,#21324,.T.);
#28909=ORIENTED_EDGE('',*,*,#21218,.F.);
#28910=ORIENTED_EDGE('',*,*,#21324,.F.);
#28911=ORIENTED_EDGE('',*,*,#21325,.F.);
#28912=ORIENTED_EDGE('',*,*,#21326,.F.);
#28913=ORIENTED_EDGE('',*,*,#19799,.F.);
#28914=ORIENTED_EDGE('',*,*,#21327,.F.);
#28915=ORIENTED_EDGE('',*,*,#21328,.F.);
#28916=ORIENTED_EDGE('',*,*,#21220,.F.);
#28917=ORIENTED_EDGE('',*,*,#21329,.T.);
#28918=ORIENTED_EDGE('',*,*,#21211,.T.);
#28919=ORIENTED_EDGE('',*,*,#21330,.T.);
#28920=ORIENTED_EDGE('',*,*,#21331,.T.);
#28921=ORIENTED_EDGE('',*,*,#21332,.T.);
#28922=ORIENTED_EDGE('',*,*,#21333,.T.);
#28923=ORIENTED_EDGE('',*,*,#21334,.T.);
#28924=ORIENTED_EDGE('',*,*,#20171,.T.);
#28925=ORIENTED_EDGE('',*,*,#21332,.F.);
#28926=ORIENTED_EDGE('',*,*,#21209,.T.);
#28927=ORIENTED_EDGE('',*,*,#21329,.F.);
#28928=ORIENTED_EDGE('',*,*,#21213,.F.);
#28929=ORIENTED_EDGE('',*,*,#21335,.T.);
#28930=ORIENTED_EDGE('',*,*,#21330,.F.);
#28931=ORIENTED_EDGE('',*,*,#21197,.F.);
#28932=ORIENTED_EDGE('',*,*,#21336,.F.);
#28933=ORIENTED_EDGE('',*,*,#21337,.F.);
#28934=ORIENTED_EDGE('',*,*,#19817,.F.);
#28935=ORIENTED_EDGE('',*,*,#21338,.F.);
#28936=ORIENTED_EDGE('',*,*,#21339,.F.);
#28937=ORIENTED_EDGE('',*,*,#21206,.F.);
#28938=ORIENTED_EDGE('',*,*,#21201,.F.);
#28939=ORIENTED_EDGE('',*,*,#21340,.T.);
#28940=ORIENTED_EDGE('',*,*,#21190,.T.);
#28941=ORIENTED_EDGE('',*,*,#21341,.T.);
#28942=ORIENTED_EDGE('',*,*,#21342,.T.);
#28943=ORIENTED_EDGE('',*,*,#21343,.T.);
#28944=ORIENTED_EDGE('',*,*,#21344,.T.);
#28945=ORIENTED_EDGE('',*,*,#21345,.T.);
#28946=ORIENTED_EDGE('',*,*,#20175,.T.);
#28947=ORIENTED_EDGE('',*,*,#21343,.F.);
#28948=ORIENTED_EDGE('',*,*,#21188,.T.);
#28949=ORIENTED_EDGE('',*,*,#21340,.F.);
#28950=ORIENTED_EDGE('',*,*,#21192,.F.);
#28951=ORIENTED_EDGE('',*,*,#21346,.T.);
#28952=ORIENTED_EDGE('',*,*,#21341,.F.);
#28953=ORIENTED_EDGE('',*,*,#21176,.F.);
#28954=ORIENTED_EDGE('',*,*,#21347,.F.);
#28955=ORIENTED_EDGE('',*,*,#21348,.F.);
#28956=ORIENTED_EDGE('',*,*,#19813,.F.);
#28957=ORIENTED_EDGE('',*,*,#21349,.F.);
#28958=ORIENTED_EDGE('',*,*,#21350,.F.);
#28959=ORIENTED_EDGE('',*,*,#21185,.F.);
#28960=ORIENTED_EDGE('',*,*,#21180,.F.);
#28961=ORIENTED_EDGE('',*,*,#21351,.T.);
#28962=ORIENTED_EDGE('',*,*,#20179,.T.);
#28963=ORIENTED_EDGE('',*,*,#21352,.T.);
#28964=ORIENTED_EDGE('',*,*,#21353,.T.);
#28965=ORIENTED_EDGE('',*,*,#21354,.T.);
#28966=ORIENTED_EDGE('',*,*,#21355,.T.);
#28967=ORIENTED_EDGE('',*,*,#21356,.T.);
#28968=ORIENTED_EDGE('',*,*,#21357,.T.);
#28969=ORIENTED_EDGE('',*,*,#21356,.F.);
#28970=ORIENTED_EDGE('',*,*,#21358,.T.);
#28971=ORIENTED_EDGE('',*,*,#21351,.F.);
#28972=ORIENTED_EDGE('',*,*,#21359,.T.);
#28973=ORIENTED_EDGE('',*,*,#21360,.T.);
#28974=ORIENTED_EDGE('',*,*,#21361,.T.);
#28975=ORIENTED_EDGE('',*,*,#21362,.T.);
#28976=ORIENTED_EDGE('',*,*,#21361,.F.);
#28977=ORIENTED_EDGE('',*,*,#21363,.T.);
#28978=ORIENTED_EDGE('',*,*,#21354,.F.);
#28979=ORIENTED_EDGE('',*,*,#21358,.F.);
#28980=ORIENTED_EDGE('',*,*,#21364,.T.);
#28981=ORIENTED_EDGE('',*,*,#21365,.F.);
#28982=ORIENTED_EDGE('',*,*,#20180,.T.);
#28983=ORIENTED_EDGE('',*,*,#21355,.F.);
#28984=ORIENTED_EDGE('',*,*,#21366,.F.);
#28985=ORIENTED_EDGE('',*,*,#21367,.F.);
#28986=ORIENTED_EDGE('',*,*,#21364,.F.);
#28987=ORIENTED_EDGE('',*,*,#21363,.F.);
#28988=ORIENTED_EDGE('',*,*,#21368,.T.);
#28989=ORIENTED_EDGE('',*,*,#21369,.T.);
#28990=ORIENTED_EDGE('',*,*,#21366,.T.);
#28991=ORIENTED_EDGE('',*,*,#21360,.F.);
#28992=ORIENTED_EDGE('',*,*,#21370,.F.);
#28993=ORIENTED_EDGE('',*,*,#21371,.F.);
#28994=ORIENTED_EDGE('',*,*,#21368,.F.);
#28995=ORIENTED_EDGE('',*,*,#21372,.T.);
#28996=ORIENTED_EDGE('',*,*,#21367,.T.);
#28997=ORIENTED_EDGE('',*,*,#21373,.T.);
#28998=ORIENTED_EDGE('',*,*,#21374,.T.);
#28999=ORIENTED_EDGE('',*,*,#21375,.T.);
#29000=ORIENTED_EDGE('',*,*,#21376,.T.);
#29001=ORIENTED_EDGE('',*,*,#21377,.T.);
#29002=ORIENTED_EDGE('',*,*,#20181,.T.);
#29003=ORIENTED_EDGE('',*,*,#21375,.F.);
#29004=ORIENTED_EDGE('',*,*,#21365,.T.);
#29005=ORIENTED_EDGE('',*,*,#21372,.F.);
#29006=ORIENTED_EDGE('',*,*,#21369,.F.);
#29007=ORIENTED_EDGE('',*,*,#21378,.T.);
#29008=ORIENTED_EDGE('',*,*,#21373,.F.);
#29009=ORIENTED_EDGE('',*,*,#21353,.F.);
#29010=ORIENTED_EDGE('',*,*,#21379,.F.);
#29011=ORIENTED_EDGE('',*,*,#21380,.F.);
#29012=ORIENTED_EDGE('',*,*,#19805,.F.);
#29013=ORIENTED_EDGE('',*,*,#21381,.F.);
#29014=ORIENTED_EDGE('',*,*,#21382,.F.);
#29015=ORIENTED_EDGE('',*,*,#21362,.F.);
#29016=ORIENTED_EDGE('',*,*,#21357,.F.);
#29017=ORIENTED_EDGE('',*,*,#21346,.F.);
#29018=ORIENTED_EDGE('',*,*,#21194,.T.);
#29019=ORIENTED_EDGE('',*,*,#21383,.T.);
#29020=ORIENTED_EDGE('',*,*,#21384,.T.);
#29021=ORIENTED_EDGE('',*,*,#21342,.F.);
#29022=ORIENTED_EDGE('',*,*,#21384,.F.);
#29023=ORIENTED_EDGE('',*,*,#21385,.F.);
#29024=ORIENTED_EDGE('',*,*,#21386,.F.);
#29025=ORIENTED_EDGE('',*,*,#19811,.F.);
#29026=ORIENTED_EDGE('',*,*,#21387,.F.);
#29027=ORIENTED_EDGE('',*,*,#21388,.F.);
#29028=ORIENTED_EDGE('',*,*,#21344,.F.);
#29029=ORIENTED_EDGE('',*,*,#21335,.F.);
#29030=ORIENTED_EDGE('',*,*,#21215,.T.);
#29031=ORIENTED_EDGE('',*,*,#21389,.T.);
#29032=ORIENTED_EDGE('',*,*,#21390,.T.);
#29033=ORIENTED_EDGE('',*,*,#21331,.F.);
#29034=ORIENTED_EDGE('',*,*,#21390,.F.);
#29035=ORIENTED_EDGE('',*,*,#21391,.F.);
#29036=ORIENTED_EDGE('',*,*,#21392,.F.);
#29037=ORIENTED_EDGE('',*,*,#19815,.F.);
#29038=ORIENTED_EDGE('',*,*,#21393,.F.);
#29039=ORIENTED_EDGE('',*,*,#21394,.F.);
#29040=ORIENTED_EDGE('',*,*,#21333,.F.);
#29041=ORIENTED_EDGE('',*,*,#21395,.T.);
#29042=ORIENTED_EDGE('',*,*,#20151,.T.);
#29043=ORIENTED_EDGE('',*,*,#21396,.T.);
#29044=ORIENTED_EDGE('',*,*,#21397,.T.);
#29045=ORIENTED_EDGE('',*,*,#21398,.T.);
#29046=ORIENTED_EDGE('',*,*,#21399,.T.);
#29047=ORIENTED_EDGE('',*,*,#21400,.T.);
#29048=ORIENTED_EDGE('',*,*,#21401,.T.);
#29049=ORIENTED_EDGE('',*,*,#21400,.F.);
#29050=ORIENTED_EDGE('',*,*,#21402,.T.);
#29051=ORIENTED_EDGE('',*,*,#21395,.F.);
#29052=ORIENTED_EDGE('',*,*,#21403,.T.);
#29053=ORIENTED_EDGE('',*,*,#21404,.T.);
#29054=ORIENTED_EDGE('',*,*,#21405,.T.);
#29055=ORIENTED_EDGE('',*,*,#21406,.T.);
#29056=ORIENTED_EDGE('',*,*,#21405,.F.);
#29057=ORIENTED_EDGE('',*,*,#21407,.T.);
#29058=ORIENTED_EDGE('',*,*,#21398,.F.);
#29059=ORIENTED_EDGE('',*,*,#21402,.F.);
#29060=ORIENTED_EDGE('',*,*,#21408,.T.);
#29061=ORIENTED_EDGE('',*,*,#21409,.F.);
#29062=ORIENTED_EDGE('',*,*,#20152,.T.);
#29063=ORIENTED_EDGE('',*,*,#21399,.F.);
#29064=ORIENTED_EDGE('',*,*,#21410,.F.);
#29065=ORIENTED_EDGE('',*,*,#21411,.F.);
#29066=ORIENTED_EDGE('',*,*,#21408,.F.);
#29067=ORIENTED_EDGE('',*,*,#21407,.F.);
#29068=ORIENTED_EDGE('',*,*,#21412,.T.);
#29069=ORIENTED_EDGE('',*,*,#21413,.T.);
#29070=ORIENTED_EDGE('',*,*,#21410,.T.);
#29071=ORIENTED_EDGE('',*,*,#21404,.F.);
#29072=ORIENTED_EDGE('',*,*,#21414,.F.);
#29073=ORIENTED_EDGE('',*,*,#21415,.F.);
#29074=ORIENTED_EDGE('',*,*,#21412,.F.);
#29075=ORIENTED_EDGE('',*,*,#21416,.T.);
#29076=ORIENTED_EDGE('',*,*,#19843,.T.);
#29077=ORIENTED_EDGE('',*,*,#21417,.T.);
#29078=ORIENTED_EDGE('',*,*,#21418,.T.);
#29079=ORIENTED_EDGE('',*,*,#21419,.T.);
#29080=ORIENTED_EDGE('',*,*,#21420,.T.);
#29081=ORIENTED_EDGE('',*,*,#21421,.T.);
#29082=ORIENTED_EDGE('',*,*,#21422,.T.);
#29083=ORIENTED_EDGE('',*,*,#21421,.F.);
#29084=ORIENTED_EDGE('',*,*,#21423,.T.);
#29085=ORIENTED_EDGE('',*,*,#21416,.F.);
#29086=ORIENTED_EDGE('',*,*,#21424,.T.);
#29087=ORIENTED_EDGE('',*,*,#21425,.T.);
#29088=ORIENTED_EDGE('',*,*,#21426,.T.);
#29089=ORIENTED_EDGE('',*,*,#21427,.T.);
#29090=ORIENTED_EDGE('',*,*,#21426,.F.);
#29091=ORIENTED_EDGE('',*,*,#21428,.T.);
#29092=ORIENTED_EDGE('',*,*,#21419,.F.);
#29093=ORIENTED_EDGE('',*,*,#21423,.F.);
#29094=ORIENTED_EDGE('',*,*,#21429,.T.);
#29095=ORIENTED_EDGE('',*,*,#21430,.F.);
#29096=ORIENTED_EDGE('',*,*,#19844,.T.);
#29097=ORIENTED_EDGE('',*,*,#21420,.F.);
#29098=ORIENTED_EDGE('',*,*,#21431,.F.);
#29099=ORIENTED_EDGE('',*,*,#21432,.F.);
#29100=ORIENTED_EDGE('',*,*,#21429,.F.);
#29101=ORIENTED_EDGE('',*,*,#21433,.T.);
#29102=ORIENTED_EDGE('',*,*,#20147,.T.);
#29103=ORIENTED_EDGE('',*,*,#21434,.T.);
#29104=ORIENTED_EDGE('',*,*,#21435,.T.);
#29105=ORIENTED_EDGE('',*,*,#21436,.T.);
#29106=ORIENTED_EDGE('',*,*,#21437,.T.);
#29107=ORIENTED_EDGE('',*,*,#21438,.T.);
#29108=ORIENTED_EDGE('',*,*,#21439,.T.);
#29109=ORIENTED_EDGE('',*,*,#21438,.F.);
#29110=ORIENTED_EDGE('',*,*,#21440,.T.);
#29111=ORIENTED_EDGE('',*,*,#21433,.F.);
#29112=ORIENTED_EDGE('',*,*,#21441,.T.);
#29113=ORIENTED_EDGE('',*,*,#21442,.T.);
#29114=ORIENTED_EDGE('',*,*,#21443,.T.);
#29115=ORIENTED_EDGE('',*,*,#21444,.T.);
#29116=ORIENTED_EDGE('',*,*,#21443,.F.);
#29117=ORIENTED_EDGE('',*,*,#21445,.T.);
#29118=ORIENTED_EDGE('',*,*,#21436,.F.);
#29119=ORIENTED_EDGE('',*,*,#21440,.F.);
#29120=ORIENTED_EDGE('',*,*,#21446,.T.);
#29121=ORIENTED_EDGE('',*,*,#21447,.F.);
#29122=ORIENTED_EDGE('',*,*,#20148,.T.);
#29123=ORIENTED_EDGE('',*,*,#21437,.F.);
#29124=ORIENTED_EDGE('',*,*,#21448,.F.);
#29125=ORIENTED_EDGE('',*,*,#21449,.F.);
#29126=ORIENTED_EDGE('',*,*,#21446,.F.);
#29127=ORIENTED_EDGE('',*,*,#21445,.F.);
#29128=ORIENTED_EDGE('',*,*,#21450,.T.);
#29129=ORIENTED_EDGE('',*,*,#21451,.T.);
#29130=ORIENTED_EDGE('',*,*,#21448,.T.);
#29131=ORIENTED_EDGE('',*,*,#21442,.F.);
#29132=ORIENTED_EDGE('',*,*,#21452,.F.);
#29133=ORIENTED_EDGE('',*,*,#21453,.F.);
#29134=ORIENTED_EDGE('',*,*,#21450,.F.);
#29135=ORIENTED_EDGE('',*,*,#21454,.T.);
#29136=ORIENTED_EDGE('',*,*,#20161,.T.);
#29137=ORIENTED_EDGE('',*,*,#21455,.T.);
#29138=ORIENTED_EDGE('',*,*,#21456,.T.);
#29139=ORIENTED_EDGE('',*,*,#21457,.T.);
#29140=ORIENTED_EDGE('',*,*,#21458,.T.);
#29141=ORIENTED_EDGE('',*,*,#21459,.T.);
#29142=ORIENTED_EDGE('',*,*,#21460,.T.);
#29143=ORIENTED_EDGE('',*,*,#21459,.F.);
#29144=ORIENTED_EDGE('',*,*,#21461,.T.);
#29145=ORIENTED_EDGE('',*,*,#21454,.F.);
#29146=ORIENTED_EDGE('',*,*,#21462,.T.);
#29147=ORIENTED_EDGE('',*,*,#21463,.T.);
#29148=ORIENTED_EDGE('',*,*,#21464,.T.);
#29149=ORIENTED_EDGE('',*,*,#21465,.T.);
#29150=ORIENTED_EDGE('',*,*,#21464,.F.);
#29151=ORIENTED_EDGE('',*,*,#21466,.T.);
#29152=ORIENTED_EDGE('',*,*,#21457,.F.);
#29153=ORIENTED_EDGE('',*,*,#21461,.F.);
#29154=ORIENTED_EDGE('',*,*,#21467,.T.);
#29155=ORIENTED_EDGE('',*,*,#21468,.F.);
#29156=ORIENTED_EDGE('',*,*,#20162,.T.);
#29157=ORIENTED_EDGE('',*,*,#21458,.F.);
#29158=ORIENTED_EDGE('',*,*,#21469,.F.);
#29159=ORIENTED_EDGE('',*,*,#21470,.F.);
#29160=ORIENTED_EDGE('',*,*,#21467,.F.);
#29161=ORIENTED_EDGE('',*,*,#21466,.F.);
#29162=ORIENTED_EDGE('',*,*,#21471,.T.);
#29163=ORIENTED_EDGE('',*,*,#21472,.T.);
#29164=ORIENTED_EDGE('',*,*,#21469,.T.);
#29165=ORIENTED_EDGE('',*,*,#21463,.F.);
#29166=ORIENTED_EDGE('',*,*,#21473,.F.);
#29167=ORIENTED_EDGE('',*,*,#21474,.F.);
#29168=ORIENTED_EDGE('',*,*,#21471,.F.);
#29169=ORIENTED_EDGE('',*,*,#21475,.T.);
#29170=ORIENTED_EDGE('',*,*,#19819,.T.);
#29171=ORIENTED_EDGE('',*,*,#21476,.T.);
#29172=ORIENTED_EDGE('',*,*,#21477,.T.);
#29173=ORIENTED_EDGE('',*,*,#21478,.T.);
#29174=ORIENTED_EDGE('',*,*,#21479,.T.);
#29175=ORIENTED_EDGE('',*,*,#21480,.T.);
#29176=ORIENTED_EDGE('',*,*,#21481,.T.);
#29177=ORIENTED_EDGE('',*,*,#21480,.F.);
#29178=ORIENTED_EDGE('',*,*,#21482,.T.);
#29179=ORIENTED_EDGE('',*,*,#21475,.F.);
#29180=ORIENTED_EDGE('',*,*,#21483,.T.);
#29181=ORIENTED_EDGE('',*,*,#21484,.T.);
#29182=ORIENTED_EDGE('',*,*,#21485,.T.);
#29183=ORIENTED_EDGE('',*,*,#21486,.T.);
#29184=ORIENTED_EDGE('',*,*,#21485,.F.);
#29185=ORIENTED_EDGE('',*,*,#21487,.T.);
#29186=ORIENTED_EDGE('',*,*,#21478,.F.);
#29187=ORIENTED_EDGE('',*,*,#21482,.F.);
#29188=ORIENTED_EDGE('',*,*,#21488,.T.);
#29189=ORIENTED_EDGE('',*,*,#21489,.F.);
#29190=ORIENTED_EDGE('',*,*,#19820,.T.);
#29191=ORIENTED_EDGE('',*,*,#21479,.F.);
#29192=ORIENTED_EDGE('',*,*,#21490,.F.);
#29193=ORIENTED_EDGE('',*,*,#21491,.F.);
#29194=ORIENTED_EDGE('',*,*,#21488,.F.);
#29195=ORIENTED_EDGE('',*,*,#21492,.T.);
#29196=ORIENTED_EDGE('',*,*,#21491,.T.);
#29197=ORIENTED_EDGE('',*,*,#21493,.T.);
#29198=ORIENTED_EDGE('',*,*,#21494,.T.);
#29199=ORIENTED_EDGE('',*,*,#21487,.F.);
#29200=ORIENTED_EDGE('',*,*,#21495,.T.);
#29201=ORIENTED_EDGE('',*,*,#21496,.T.);
#29202=ORIENTED_EDGE('',*,*,#21490,.T.);
#29203=ORIENTED_EDGE('',*,*,#21496,.F.);
#29204=ORIENTED_EDGE('',*,*,#21497,.T.);
#29205=ORIENTED_EDGE('',*,*,#21493,.F.);
#29206=ORIENTED_EDGE('',*,*,#21498,.T.);
#29207=ORIENTED_EDGE('',*,*,#21499,.T.);
#29208=ORIENTED_EDGE('',*,*,#21500,.T.);
#29209=ORIENTED_EDGE('',*,*,#19821,.T.);
#29210=ORIENTED_EDGE('',*,*,#21498,.F.);
#29211=ORIENTED_EDGE('',*,*,#21489,.T.);
#29212=ORIENTED_EDGE('',*,*,#21492,.F.);
#29213=ORIENTED_EDGE('',*,*,#21477,.F.);
#29214=ORIENTED_EDGE('',*,*,#21501,.F.);
#29215=ORIENTED_EDGE('',*,*,#21502,.F.);
#29216=ORIENTED_EDGE('',*,*,#20167,.F.);
#29217=ORIENTED_EDGE('',*,*,#21503,.F.);
#29218=ORIENTED_EDGE('',*,*,#21504,.F.);
#29219=ORIENTED_EDGE('',*,*,#21486,.F.);
#29220=ORIENTED_EDGE('',*,*,#21481,.F.);
#29221=ORIENTED_EDGE('',*,*,#21505,.T.);
#29222=ORIENTED_EDGE('',*,*,#21470,.T.);
#29223=ORIENTED_EDGE('',*,*,#21506,.T.);
#29224=ORIENTED_EDGE('',*,*,#21507,.T.);
#29225=ORIENTED_EDGE('',*,*,#21508,.T.);
#29226=ORIENTED_EDGE('',*,*,#21509,.T.);
#29227=ORIENTED_EDGE('',*,*,#21510,.T.);
#29228=ORIENTED_EDGE('',*,*,#20163,.T.);
#29229=ORIENTED_EDGE('',*,*,#21508,.F.);
#29230=ORIENTED_EDGE('',*,*,#21468,.T.);
#29231=ORIENTED_EDGE('',*,*,#21505,.F.);
#29232=ORIENTED_EDGE('',*,*,#21472,.F.);
#29233=ORIENTED_EDGE('',*,*,#21511,.T.);
#29234=ORIENTED_EDGE('',*,*,#21506,.F.);
#29235=ORIENTED_EDGE('',*,*,#21456,.F.);
#29236=ORIENTED_EDGE('',*,*,#21512,.F.);
#29237=ORIENTED_EDGE('',*,*,#21513,.F.);
#29238=ORIENTED_EDGE('',*,*,#19825,.F.);
#29239=ORIENTED_EDGE('',*,*,#21514,.F.);
#29240=ORIENTED_EDGE('',*,*,#21515,.F.);
#29241=ORIENTED_EDGE('',*,*,#21465,.F.);
#29242=ORIENTED_EDGE('',*,*,#21460,.F.);
#29243=ORIENTED_EDGE('',*,*,#21516,.T.);
#29244=ORIENTED_EDGE('',*,*,#21449,.T.);
#29245=ORIENTED_EDGE('',*,*,#21517,.T.);
#29246=ORIENTED_EDGE('',*,*,#21518,.T.);
#29247=ORIENTED_EDGE('',*,*,#21519,.T.);
#29248=ORIENTED_EDGE('',*,*,#21520,.T.);
#29249=ORIENTED_EDGE('',*,*,#21521,.T.);
#29250=ORIENTED_EDGE('',*,*,#20149,.T.);
#29251=ORIENTED_EDGE('',*,*,#21519,.F.);
#29252=ORIENTED_EDGE('',*,*,#21447,.T.);
#29253=ORIENTED_EDGE('',*,*,#21516,.F.);
#29254=ORIENTED_EDGE('',*,*,#21451,.F.);
#29255=ORIENTED_EDGE('',*,*,#21522,.T.);
#29256=ORIENTED_EDGE('',*,*,#21517,.F.);
#29257=ORIENTED_EDGE('',*,*,#21435,.F.);
#29258=ORIENTED_EDGE('',*,*,#21523,.F.);
#29259=ORIENTED_EDGE('',*,*,#21524,.F.);
#29260=ORIENTED_EDGE('',*,*,#19841,.F.);
#29261=ORIENTED_EDGE('',*,*,#21525,.F.);
#29262=ORIENTED_EDGE('',*,*,#21526,.F.);
#29263=ORIENTED_EDGE('',*,*,#21444,.F.);
#29264=ORIENTED_EDGE('',*,*,#21439,.F.);
#29265=ORIENTED_EDGE('',*,*,#21527,.T.);
#29266=ORIENTED_EDGE('',*,*,#21432,.T.);
#29267=ORIENTED_EDGE('',*,*,#21528,.T.);
#29268=ORIENTED_EDGE('',*,*,#21529,.T.);
#29269=ORIENTED_EDGE('',*,*,#21428,.F.);
#29270=ORIENTED_EDGE('',*,*,#21530,.T.);
#29271=ORIENTED_EDGE('',*,*,#21531,.T.);
#29272=ORIENTED_EDGE('',*,*,#21431,.T.);
#29273=ORIENTED_EDGE('',*,*,#21531,.F.);
#29274=ORIENTED_EDGE('',*,*,#21532,.T.);
#29275=ORIENTED_EDGE('',*,*,#21528,.F.);
#29276=ORIENTED_EDGE('',*,*,#21533,.T.);
#29277=ORIENTED_EDGE('',*,*,#21534,.T.);
#29278=ORIENTED_EDGE('',*,*,#21535,.T.);
#29279=ORIENTED_EDGE('',*,*,#19845,.T.);
#29280=ORIENTED_EDGE('',*,*,#21533,.F.);
#29281=ORIENTED_EDGE('',*,*,#21430,.T.);
#29282=ORIENTED_EDGE('',*,*,#21527,.F.);
#29283=ORIENTED_EDGE('',*,*,#21418,.F.);
#29284=ORIENTED_EDGE('',*,*,#21536,.F.);
#29285=ORIENTED_EDGE('',*,*,#21537,.F.);
#29286=ORIENTED_EDGE('',*,*,#20145,.F.);
#29287=ORIENTED_EDGE('',*,*,#21538,.F.);
#29288=ORIENTED_EDGE('',*,*,#21539,.F.);
#29289=ORIENTED_EDGE('',*,*,#21427,.F.);
#29290=ORIENTED_EDGE('',*,*,#21422,.F.);
#29291=ORIENTED_EDGE('',*,*,#21540,.T.);
#29292=ORIENTED_EDGE('',*,*,#21541,.T.);
#29293=ORIENTED_EDGE('',*,*,#21542,.T.);
#29294=ORIENTED_EDGE('',*,*,#21543,.T.);
#29295=ORIENTED_EDGE('',*,*,#21540,.F.);
#29296=ORIENTED_EDGE('',*,*,#21544,.T.);
#29297=ORIENTED_EDGE('',*,*,#21545,.F.);
#29298=ORIENTED_EDGE('',*,*,#21546,.T.);
#29299=ORIENTED_EDGE('',*,*,#21547,.F.);
#29300=ORIENTED_EDGE('',*,*,#21548,.F.);
#29301=ORIENTED_EDGE('',*,*,#21543,.F.);
#29302=ORIENTED_EDGE('',*,*,#21549,.F.);
#29303=ORIENTED_EDGE('',*,*,#21550,.F.);
#29304=ORIENTED_EDGE('',*,*,#19847,.F.);
#29305=ORIENTED_EDGE('',*,*,#21551,.F.);
#29306=ORIENTED_EDGE('',*,*,#21552,.F.);
#29307=ORIENTED_EDGE('',*,*,#21553,.F.);
#29308=ORIENTED_EDGE('',*,*,#20141,.F.);
#29309=ORIENTED_EDGE('',*,*,#21554,.F.);
#29310=ORIENTED_EDGE('',*,*,#21544,.F.);
#29311=ORIENTED_EDGE('',*,*,#21555,.T.);
#29312=ORIENTED_EDGE('',*,*,#21411,.T.);
#29313=ORIENTED_EDGE('',*,*,#21556,.T.);
#29314=ORIENTED_EDGE('',*,*,#21557,.T.);
#29315=ORIENTED_EDGE('',*,*,#21558,.T.);
#29316=ORIENTED_EDGE('',*,*,#21559,.T.);
#29317=ORIENTED_EDGE('',*,*,#21560,.T.);
#29318=ORIENTED_EDGE('',*,*,#20153,.T.);
#29319=ORIENTED_EDGE('',*,*,#21558,.F.);
#29320=ORIENTED_EDGE('',*,*,#21409,.T.);
#29321=ORIENTED_EDGE('',*,*,#21555,.F.);
#29322=ORIENTED_EDGE('',*,*,#21413,.F.);
#29323=ORIENTED_EDGE('',*,*,#21561,.T.);
#29324=ORIENTED_EDGE('',*,*,#21556,.F.);
#29325=ORIENTED_EDGE('',*,*,#21397,.F.);
#29326=ORIENTED_EDGE('',*,*,#21562,.F.);
#29327=ORIENTED_EDGE('',*,*,#21563,.F.);
#29328=ORIENTED_EDGE('',*,*,#19837,.F.);
#29329=ORIENTED_EDGE('',*,*,#21564,.F.);
#29330=ORIENTED_EDGE('',*,*,#21565,.F.);
#29331=ORIENTED_EDGE('',*,*,#21406,.F.);
#29332=ORIENTED_EDGE('',*,*,#21401,.F.);
#29333=ORIENTED_EDGE('',*,*,#21566,.T.);
#29334=ORIENTED_EDGE('',*,*,#19831,.T.);
#29335=ORIENTED_EDGE('',*,*,#21567,.T.);
#29336=ORIENTED_EDGE('',*,*,#21568,.T.);
#29337=ORIENTED_EDGE('',*,*,#21569,.T.);
#29338=ORIENTED_EDGE('',*,*,#21570,.T.);
#29339=ORIENTED_EDGE('',*,*,#21571,.T.);
#29340=ORIENTED_EDGE('',*,*,#21572,.T.);
#29341=ORIENTED_EDGE('',*,*,#21571,.F.);
#29342=ORIENTED_EDGE('',*,*,#21573,.T.);
#29343=ORIENTED_EDGE('',*,*,#21566,.F.);
#29344=ORIENTED_EDGE('',*,*,#21574,.T.);
#29345=ORIENTED_EDGE('',*,*,#21575,.T.);
#29346=ORIENTED_EDGE('',*,*,#21576,.T.);
#29347=ORIENTED_EDGE('',*,*,#21577,.T.);
#29348=ORIENTED_EDGE('',*,*,#21576,.F.);
#29349=ORIENTED_EDGE('',*,*,#21578,.T.);
#29350=ORIENTED_EDGE('',*,*,#21569,.F.);
#29351=ORIENTED_EDGE('',*,*,#21573,.F.);
#29352=ORIENTED_EDGE('',*,*,#21579,.T.);
#29353=ORIENTED_EDGE('',*,*,#21580,.F.);
#29354=ORIENTED_EDGE('',*,*,#19832,.T.);
#29355=ORIENTED_EDGE('',*,*,#21570,.F.);
#29356=ORIENTED_EDGE('',*,*,#21581,.F.);
#29357=ORIENTED_EDGE('',*,*,#21582,.F.);
#29358=ORIENTED_EDGE('',*,*,#21579,.F.);
#29359=ORIENTED_EDGE('',*,*,#21583,.T.);
#29360=ORIENTED_EDGE('',*,*,#20022,.T.);
#29361=ORIENTED_EDGE('',*,*,#21584,.T.);
#29362=ORIENTED_EDGE('',*,*,#20030,.T.);
#29363=ORIENTED_EDGE('',*,*,#21585,.T.);
#29364=ORIENTED_EDGE('',*,*,#20029,.T.);
#29365=ORIENTED_EDGE('',*,*,#21586,.T.);
#29366=ORIENTED_EDGE('',*,*,#20159,.T.);
#29367=ORIENTED_EDGE('',*,*,#21585,.F.);
#29368=ORIENTED_EDGE('',*,*,#20019,.T.);
#29369=ORIENTED_EDGE('',*,*,#21583,.F.);
#29370=ORIENTED_EDGE('',*,*,#20024,.F.);
#29371=ORIENTED_EDGE('',*,*,#20027,.T.);
#29372=ORIENTED_EDGE('',*,*,#21584,.F.);
#29373=ORIENTED_EDGE('',*,*,#21587,.T.);
#29374=ORIENTED_EDGE('',*,*,#21582,.T.);
#29375=ORIENTED_EDGE('',*,*,#21588,.T.);
#29376=ORIENTED_EDGE('',*,*,#21589,.T.);
#29377=ORIENTED_EDGE('',*,*,#21578,.F.);
#29378=ORIENTED_EDGE('',*,*,#21590,.T.);
#29379=ORIENTED_EDGE('',*,*,#21591,.T.);
#29380=ORIENTED_EDGE('',*,*,#21581,.T.);
#29381=ORIENTED_EDGE('',*,*,#21591,.F.);
#29382=ORIENTED_EDGE('',*,*,#21592,.T.);
#29383=ORIENTED_EDGE('',*,*,#21588,.F.);
#29384=ORIENTED_EDGE('',*,*,#21593,.T.);
#29385=ORIENTED_EDGE('',*,*,#21594,.T.);
#29386=ORIENTED_EDGE('',*,*,#21595,.T.);
#29387=ORIENTED_EDGE('',*,*,#19833,.T.);
#29388=ORIENTED_EDGE('',*,*,#21593,.F.);
#29389=ORIENTED_EDGE('',*,*,#21580,.T.);
#29390=ORIENTED_EDGE('',*,*,#21587,.F.);
#29391=ORIENTED_EDGE('',*,*,#21568,.F.);
#29392=ORIENTED_EDGE('',*,*,#21596,.F.);
#29393=ORIENTED_EDGE('',*,*,#21597,.F.);
#29394=ORIENTED_EDGE('',*,*,#20157,.F.);
#29395=ORIENTED_EDGE('',*,*,#21598,.F.);
#29396=ORIENTED_EDGE('',*,*,#21599,.F.);
#29397=ORIENTED_EDGE('',*,*,#21577,.F.);
#29398=ORIENTED_EDGE('',*,*,#21572,.F.);
#29399=ORIENTED_EDGE('',*,*,#21561,.F.);
#29400=ORIENTED_EDGE('',*,*,#21415,.T.);
#29401=ORIENTED_EDGE('',*,*,#21600,.T.);
#29402=ORIENTED_EDGE('',*,*,#21601,.T.);
#29403=ORIENTED_EDGE('',*,*,#21557,.F.);
#29404=ORIENTED_EDGE('',*,*,#21601,.F.);
#29405=ORIENTED_EDGE('',*,*,#21602,.F.);
#29406=ORIENTED_EDGE('',*,*,#21603,.F.);
#29407=ORIENTED_EDGE('',*,*,#19835,.F.);
#29408=ORIENTED_EDGE('',*,*,#21604,.F.);
#29409=ORIENTED_EDGE('',*,*,#21605,.F.);
#29410=ORIENTED_EDGE('',*,*,#21559,.F.);
#29411=ORIENTED_EDGE('',*,*,#21606,.T.);
#29412=ORIENTED_EDGE('',*,*,#19852,.T.);
#29413=ORIENTED_EDGE('',*,*,#21607,.T.);
#29414=ORIENTED_EDGE('',*,*,#21608,.T.);
#29415=ORIENTED_EDGE('',*,*,#21609,.T.);
#29416=ORIENTED_EDGE('',*,*,#19851,.T.);
#29417=ORIENTED_EDGE('',*,*,#21610,.T.);
#29418=ORIENTED_EDGE('',*,*,#21611,.T.);
#29419=ORIENTED_EDGE('',*,*,#21609,.F.);
#29420=ORIENTED_EDGE('',*,*,#21612,.T.);
#29421=ORIENTED_EDGE('',*,*,#21607,.F.);
#29422=ORIENTED_EDGE('',*,*,#21612,.F.);
#29423=ORIENTED_EDGE('',*,*,#21613,.T.);
#29424=ORIENTED_EDGE('',*,*,#21614,.T.);
#29425=ORIENTED_EDGE('',*,*,#21615,.T.);
#29426=ORIENTED_EDGE('',*,*,#21611,.F.);
#29427=ORIENTED_EDGE('',*,*,#21616,.F.);
#29428=ORIENTED_EDGE('',*,*,#21617,.F.);
#29429=ORIENTED_EDGE('',*,*,#21618,.F.);
#29430=ORIENTED_EDGE('',*,*,#21619,.F.);
#29431=ORIENTED_EDGE('',*,*,#21613,.F.);
#29432=ORIENTED_EDGE('',*,*,#21620,.T.);
#29433=ORIENTED_EDGE('',*,*,#19848,.T.);
#29434=ORIENTED_EDGE('',*,*,#21550,.T.);
#29435=ORIENTED_EDGE('',*,*,#21621,.T.);
#29436=ORIENTED_EDGE('',*,*,#21622,.T.);
#29437=ORIENTED_EDGE('',*,*,#21551,.T.);
#29438=ORIENTED_EDGE('',*,*,#19846,.T.);
#29439=ORIENTED_EDGE('',*,*,#21535,.F.);
#29440=ORIENTED_EDGE('',*,*,#21622,.F.);
#29441=ORIENTED_EDGE('',*,*,#21623,.T.);
#29442=ORIENTED_EDGE('',*,*,#21624,.F.);
#29443=ORIENTED_EDGE('',*,*,#21552,.T.);
#29444=ORIENTED_EDGE('',*,*,#21529,.F.);
#29445=ORIENTED_EDGE('',*,*,#21625,.F.);
#29446=ORIENTED_EDGE('',*,*,#21626,.F.);
#29447=ORIENTED_EDGE('',*,*,#21627,.F.);
#29448=ORIENTED_EDGE('',*,*,#20143,.F.);
#29449=ORIENTED_EDGE('',*,*,#21628,.F.);
#29450=ORIENTED_EDGE('',*,*,#21623,.F.);
#29451=ORIENTED_EDGE('',*,*,#21534,.F.);
#29452=ORIENTED_EDGE('',*,*,#21522,.F.);
#29453=ORIENTED_EDGE('',*,*,#21453,.T.);
#29454=ORIENTED_EDGE('',*,*,#21629,.T.);
#29455=ORIENTED_EDGE('',*,*,#21630,.T.);
#29456=ORIENTED_EDGE('',*,*,#21518,.F.);
#29457=ORIENTED_EDGE('',*,*,#21630,.F.);
#29458=ORIENTED_EDGE('',*,*,#21631,.F.);
#29459=ORIENTED_EDGE('',*,*,#21632,.F.);
#29460=ORIENTED_EDGE('',*,*,#19839,.F.);
#29461=ORIENTED_EDGE('',*,*,#21633,.F.);
#29462=ORIENTED_EDGE('',*,*,#21634,.F.);
#29463=ORIENTED_EDGE('',*,*,#21520,.F.);
#29464=ORIENTED_EDGE('',*,*,#21525,.T.);
#29465=ORIENTED_EDGE('',*,*,#19840,.T.);
#29466=ORIENTED_EDGE('',*,*,#21632,.T.);
#29467=ORIENTED_EDGE('',*,*,#21635,.T.);
#29468=ORIENTED_EDGE('',*,*,#21563,.T.);
#29469=ORIENTED_EDGE('',*,*,#21636,.T.);
#29470=ORIENTED_EDGE('',*,*,#21633,.T.);
#29471=ORIENTED_EDGE('',*,*,#19838,.T.);
#29472=ORIENTED_EDGE('',*,*,#21636,.F.);
#29473=ORIENTED_EDGE('',*,*,#21562,.T.);
#29474=ORIENTED_EDGE('',*,*,#21637,.F.);
#29475=ORIENTED_EDGE('',*,*,#21634,.T.);
#29476=ORIENTED_EDGE('',*,*,#21564,.T.);
#29477=ORIENTED_EDGE('',*,*,#19836,.T.);
#29478=ORIENTED_EDGE('',*,*,#21603,.T.);
#29479=ORIENTED_EDGE('',*,*,#21638,.T.);
#29480=ORIENTED_EDGE('',*,*,#21639,.T.);
#29481=ORIENTED_EDGE('',*,*,#21604,.T.);
#29482=ORIENTED_EDGE('',*,*,#19834,.T.);
#29483=ORIENTED_EDGE('',*,*,#21595,.F.);
#29484=ORIENTED_EDGE('',*,*,#21639,.F.);
#29485=ORIENTED_EDGE('',*,*,#21640,.T.);
#29486=ORIENTED_EDGE('',*,*,#21641,.F.);
#29487=ORIENTED_EDGE('',*,*,#21605,.T.);
#29488=ORIENTED_EDGE('',*,*,#21589,.F.);
#29489=ORIENTED_EDGE('',*,*,#21642,.F.);
#29490=ORIENTED_EDGE('',*,*,#21643,.F.);
#29491=ORIENTED_EDGE('',*,*,#21644,.F.);
#29492=ORIENTED_EDGE('',*,*,#20155,.F.);
#29493=ORIENTED_EDGE('',*,*,#21645,.F.);
#29494=ORIENTED_EDGE('',*,*,#21640,.F.);
#29495=ORIENTED_EDGE('',*,*,#21594,.F.);
#29496=ORIENTED_EDGE('',*,*,#20016,.F.);
#29497=ORIENTED_EDGE('',*,*,#21646,.T.);
#29498=ORIENTED_EDGE('',*,*,#21647,.T.);
#29499=ORIENTED_EDGE('',*,*,#19828,.T.);
#29500=ORIENTED_EDGE('',*,*,#21513,.T.);
#29501=ORIENTED_EDGE('',*,*,#21648,.T.);
#29502=ORIENTED_EDGE('',*,*,#20010,.F.);
#29503=ORIENTED_EDGE('',*,*,#19826,.T.);
#29504=ORIENTED_EDGE('',*,*,#21648,.F.);
#29505=ORIENTED_EDGE('',*,*,#21512,.T.);
#29506=ORIENTED_EDGE('',*,*,#21649,.F.);
#29507=ORIENTED_EDGE('',*,*,#20028,.T.);
#29508=ORIENTED_EDGE('',*,*,#21511,.F.);
#29509=ORIENTED_EDGE('',*,*,#21474,.T.);
#29510=ORIENTED_EDGE('',*,*,#21650,.T.);
#29511=ORIENTED_EDGE('',*,*,#21651,.T.);
#29512=ORIENTED_EDGE('',*,*,#21507,.F.);
#29513=ORIENTED_EDGE('',*,*,#21651,.F.);
#29514=ORIENTED_EDGE('',*,*,#21652,.F.);
#29515=ORIENTED_EDGE('',*,*,#21653,.F.);
#29516=ORIENTED_EDGE('',*,*,#19823,.F.);
#29517=ORIENTED_EDGE('',*,*,#21654,.F.);
#29518=ORIENTED_EDGE('',*,*,#21655,.F.);
#29519=ORIENTED_EDGE('',*,*,#21509,.F.);
#29520=ORIENTED_EDGE('',*,*,#21514,.T.);
#29521=ORIENTED_EDGE('',*,*,#19824,.T.);
#29522=ORIENTED_EDGE('',*,*,#21653,.T.);
#29523=ORIENTED_EDGE('',*,*,#21656,.T.);
#29524=ORIENTED_EDGE('',*,*,#21657,.T.);
#29525=ORIENTED_EDGE('',*,*,#21654,.T.);
#29526=ORIENTED_EDGE('',*,*,#19822,.T.);
#29527=ORIENTED_EDGE('',*,*,#21500,.F.);
#29528=ORIENTED_EDGE('',*,*,#21657,.F.);
#29529=ORIENTED_EDGE('',*,*,#21658,.T.);
#29530=ORIENTED_EDGE('',*,*,#21659,.F.);
#29531=ORIENTED_EDGE('',*,*,#21655,.T.);
#29532=ORIENTED_EDGE('',*,*,#21494,.F.);
#29533=ORIENTED_EDGE('',*,*,#21660,.F.);
#29534=ORIENTED_EDGE('',*,*,#21661,.F.);
#29535=ORIENTED_EDGE('',*,*,#21662,.F.);
#29536=ORIENTED_EDGE('',*,*,#20165,.F.);
#29537=ORIENTED_EDGE('',*,*,#21663,.F.);
#29538=ORIENTED_EDGE('',*,*,#21658,.F.);
#29539=ORIENTED_EDGE('',*,*,#21499,.F.);
#29540=ORIENTED_EDGE('',*,*,#21338,.T.);
#29541=ORIENTED_EDGE('',*,*,#19816,.T.);
#29542=ORIENTED_EDGE('',*,*,#21392,.T.);
#29543=ORIENTED_EDGE('',*,*,#21664,.T.);
#29544=ORIENTED_EDGE('',*,*,#21348,.T.);
#29545=ORIENTED_EDGE('',*,*,#21665,.T.);
#29546=ORIENTED_EDGE('',*,*,#21393,.T.);
#29547=ORIENTED_EDGE('',*,*,#19814,.T.);
#29548=ORIENTED_EDGE('',*,*,#21665,.F.);
#29549=ORIENTED_EDGE('',*,*,#21347,.T.);
#29550=ORIENTED_EDGE('',*,*,#21666,.F.);
#29551=ORIENTED_EDGE('',*,*,#21394,.T.);
#29552=ORIENTED_EDGE('',*,*,#21349,.T.);
#29553=ORIENTED_EDGE('',*,*,#19812,.T.);
#29554=ORIENTED_EDGE('',*,*,#21386,.T.);
#29555=ORIENTED_EDGE('',*,*,#21667,.T.);
#29556=ORIENTED_EDGE('',*,*,#21378,.F.);
#29557=ORIENTED_EDGE('',*,*,#21371,.T.);
#29558=ORIENTED_EDGE('',*,*,#21668,.T.);
#29559=ORIENTED_EDGE('',*,*,#21669,.T.);
#29560=ORIENTED_EDGE('',*,*,#21374,.F.);
#29561=ORIENTED_EDGE('',*,*,#21669,.F.);
#29562=ORIENTED_EDGE('',*,*,#21670,.F.);
#29563=ORIENTED_EDGE('',*,*,#21671,.F.);
#29564=ORIENTED_EDGE('',*,*,#19803,.F.);
#29565=ORIENTED_EDGE('',*,*,#21672,.F.);
#29566=ORIENTED_EDGE('',*,*,#21673,.F.);
#29567=ORIENTED_EDGE('',*,*,#21376,.F.);
#29568=ORIENTED_EDGE('',*,*,#21674,.T.);
#29569=ORIENTED_EDGE('',*,*,#19987,.T.);
#29570=ORIENTED_EDGE('',*,*,#21675,.T.);
#29571=ORIENTED_EDGE('',*,*,#21676,.T.);
#29572=ORIENTED_EDGE('',*,*,#19989,.F.);
#29573=ORIENTED_EDGE('',*,*,#21677,.T.);
#29574=ORIENTED_EDGE('',*,*,#21675,.F.);
#29575=ORIENTED_EDGE('',*,*,#21678,.T.);
#29576=ORIENTED_EDGE('',*,*,#21679,.T.);
#29577=ORIENTED_EDGE('',*,*,#21680,.T.);
#29578=ORIENTED_EDGE('',*,*,#19809,.T.);
#29579=ORIENTED_EDGE('',*,*,#21678,.F.);
#29580=ORIENTED_EDGE('',*,*,#19985,.T.);
#29581=ORIENTED_EDGE('',*,*,#21674,.F.);
#29582=ORIENTED_EDGE('',*,*,#21681,.T.);
#29583=ORIENTED_EDGE('',*,*,#21387,.T.);
#29584=ORIENTED_EDGE('',*,*,#19810,.T.);
#29585=ORIENTED_EDGE('',*,*,#21680,.F.);
#29586=ORIENTED_EDGE('',*,*,#21681,.F.);
#29587=ORIENTED_EDGE('',*,*,#21682,.T.);
#29588=ORIENTED_EDGE('',*,*,#21683,.F.);
#29589=ORIENTED_EDGE('',*,*,#21388,.T.);
#29590=ORIENTED_EDGE('',*,*,#19963,.F.);
#29591=ORIENTED_EDGE('',*,*,#21682,.F.);
#29592=ORIENTED_EDGE('',*,*,#21679,.F.);
#29593=ORIENTED_EDGE('',*,*,#21676,.F.);
#29594=ORIENTED_EDGE('',*,*,#21684,.F.);
#29595=ORIENTED_EDGE('',*,*,#19975,.F.);
#29596=ORIENTED_EDGE('',*,*,#21381,.T.);
#29597=ORIENTED_EDGE('',*,*,#19804,.T.);
#29598=ORIENTED_EDGE('',*,*,#21671,.T.);
#29599=ORIENTED_EDGE('',*,*,#21685,.T.);
#29600=ORIENTED_EDGE('',*,*,#21224,.T.);
#29601=ORIENTED_EDGE('',*,*,#21686,.T.);
#29602=ORIENTED_EDGE('',*,*,#21672,.T.);
#29603=ORIENTED_EDGE('',*,*,#19802,.T.);
#29604=ORIENTED_EDGE('',*,*,#21686,.F.);
#29605=ORIENTED_EDGE('',*,*,#21223,.T.);
#29606=ORIENTED_EDGE('',*,*,#21687,.F.);
#29607=ORIENTED_EDGE('',*,*,#21673,.T.);
#29608=ORIENTED_EDGE('',*,*,#21225,.T.);
#29609=ORIENTED_EDGE('',*,*,#19800,.T.);
#29610=ORIENTED_EDGE('',*,*,#21326,.T.);
#29611=ORIENTED_EDGE('',*,*,#21688,.T.);
#29612=ORIENTED_EDGE('',*,*,#21689,.T.);
#29613=ORIENTED_EDGE('',*,*,#21327,.T.);
#29614=ORIENTED_EDGE('',*,*,#19798,.T.);
#29615=ORIENTED_EDGE('',*,*,#21318,.F.);
#29616=ORIENTED_EDGE('',*,*,#21689,.F.);
#29617=ORIENTED_EDGE('',*,*,#21690,.T.);
#29618=ORIENTED_EDGE('',*,*,#21691,.F.);
#29619=ORIENTED_EDGE('',*,*,#21328,.T.);
#29620=ORIENTED_EDGE('',*,*,#21312,.F.);
#29621=ORIENTED_EDGE('',*,*,#21692,.F.);
#29622=ORIENTED_EDGE('',*,*,#21693,.F.);
#29623=ORIENTED_EDGE('',*,*,#21694,.F.);
#29624=ORIENTED_EDGE('',*,*,#20187,.F.);
#29625=ORIENTED_EDGE('',*,*,#21695,.F.);
#29626=ORIENTED_EDGE('',*,*,#21690,.F.);
#29627=ORIENTED_EDGE('',*,*,#21317,.F.);
#29628=ORIENTED_EDGE('',*,*,#21305,.F.);
#29629=ORIENTED_EDGE('',*,*,#21264,.T.);
#29630=ORIENTED_EDGE('',*,*,#21696,.T.);
#29631=ORIENTED_EDGE('',*,*,#21697,.T.);
#29632=ORIENTED_EDGE('',*,*,#21301,.F.);
#29633=ORIENTED_EDGE('',*,*,#21697,.F.);
#29634=ORIENTED_EDGE('',*,*,#21698,.F.);
#29635=ORIENTED_EDGE('',*,*,#21699,.F.);
#29636=ORIENTED_EDGE('',*,*,#19791,.F.);
#29637=ORIENTED_EDGE('',*,*,#21700,.F.);
#29638=ORIENTED_EDGE('',*,*,#21701,.F.);
#29639=ORIENTED_EDGE('',*,*,#21303,.F.);
#29640=ORIENTED_EDGE('',*,*,#21308,.T.);
#29641=ORIENTED_EDGE('',*,*,#19792,.T.);
#29642=ORIENTED_EDGE('',*,*,#21699,.T.);
#29643=ORIENTED_EDGE('',*,*,#21702,.T.);
#29644=ORIENTED_EDGE('',*,*,#21703,.T.);
#29645=ORIENTED_EDGE('',*,*,#21704,.T.);
#29646=ORIENTED_EDGE('',*,*,#21700,.T.);
#29647=ORIENTED_EDGE('',*,*,#19790,.T.);
#29648=ORIENTED_EDGE('',*,*,#21704,.F.);
#29649=ORIENTED_EDGE('',*,*,#21705,.T.);
#29650=ORIENTED_EDGE('',*,*,#21706,.F.);
#29651=ORIENTED_EDGE('',*,*,#21701,.T.);
#29652=ORIENTED_EDGE('',*,*,#20056,.F.);
#29653=ORIENTED_EDGE('',*,*,#21707,.T.);
#29654=ORIENTED_EDGE('',*,*,#21708,.T.);
#29655=ORIENTED_EDGE('',*,*,#19788,.T.);
#29656=ORIENTED_EDGE('',*,*,#21709,.T.);
#29657=ORIENTED_EDGE('',*,*,#20050,.F.);
#29658=ORIENTED_EDGE('',*,*,#19786,.T.);
#29659=ORIENTED_EDGE('',*,*,#21294,.F.);
#29660=ORIENTED_EDGE('',*,*,#21709,.F.);
#29661=ORIENTED_EDGE('',*,*,#21710,.T.);
#29662=ORIENTED_EDGE('',*,*,#21711,.F.);
#29663=ORIENTED_EDGE('',*,*,#20068,.T.);
#29664=ORIENTED_EDGE('',*,*,#21288,.F.);
#29665=ORIENTED_EDGE('',*,*,#21712,.F.);
#29666=ORIENTED_EDGE('',*,*,#21713,.F.);
#29667=ORIENTED_EDGE('',*,*,#21714,.F.);
#29668=ORIENTED_EDGE('',*,*,#20197,.F.);
#29669=ORIENTED_EDGE('',*,*,#21715,.F.);
#29670=ORIENTED_EDGE('',*,*,#21710,.F.);
#29671=ORIENTED_EDGE('',*,*,#21293,.F.);
#29672=ORIENTED_EDGE('',*,*,#21716,.T.);
#29673=ORIENTED_EDGE('',*,*,#19780,.T.);
#29674=ORIENTED_EDGE('',*,*,#21171,.T.);
#29675=ORIENTED_EDGE('',*,*,#21717,.T.);
#29676=ORIENTED_EDGE('',*,*,#21137,.T.);
#29677=ORIENTED_EDGE('',*,*,#21718,.T.);
#29678=ORIENTED_EDGE('',*,*,#21172,.T.);
#29679=ORIENTED_EDGE('',*,*,#19778,.T.);
#29680=ORIENTED_EDGE('',*,*,#21718,.F.);
#29681=ORIENTED_EDGE('',*,*,#21136,.T.);
#29682=ORIENTED_EDGE('',*,*,#21719,.F.);
#29683=ORIENTED_EDGE('',*,*,#21173,.T.);
#29684=ORIENTED_EDGE('',*,*,#21135,.F.);
#29685=ORIENTED_EDGE('',*,*,#21019,.T.);
#29686=ORIENTED_EDGE('',*,*,#21720,.T.);
#29687=ORIENTED_EDGE('',*,*,#21721,.T.);
#29688=ORIENTED_EDGE('',*,*,#21131,.F.);
#29689=ORIENTED_EDGE('',*,*,#21721,.F.);
#29690=ORIENTED_EDGE('',*,*,#21722,.F.);
#29691=ORIENTED_EDGE('',*,*,#21723,.F.);
#29692=ORIENTED_EDGE('',*,*,#19775,.F.);
#29693=ORIENTED_EDGE('',*,*,#21724,.F.);
#29694=ORIENTED_EDGE('',*,*,#21725,.F.);
#29695=ORIENTED_EDGE('',*,*,#21133,.F.);
#29696=ORIENTED_EDGE('',*,*,#21138,.T.);
#29697=ORIENTED_EDGE('',*,*,#19776,.T.);
#29698=ORIENTED_EDGE('',*,*,#21723,.T.);
#29699=ORIENTED_EDGE('',*,*,#21726,.T.);
#29700=ORIENTED_EDGE('',*,*,#21727,.T.);
#29701=ORIENTED_EDGE('',*,*,#21724,.T.);
#29702=ORIENTED_EDGE('',*,*,#19774,.T.);
#29703=ORIENTED_EDGE('',*,*,#21124,.F.);
#29704=ORIENTED_EDGE('',*,*,#21727,.F.);
#29705=ORIENTED_EDGE('',*,*,#21728,.T.);
#29706=ORIENTED_EDGE('',*,*,#21729,.F.);
#29707=ORIENTED_EDGE('',*,*,#21725,.T.);
#29708=ORIENTED_EDGE('',*,*,#21118,.F.);
#29709=ORIENTED_EDGE('',*,*,#21730,.F.);
#29710=ORIENTED_EDGE('',*,*,#21731,.F.);
#29711=ORIENTED_EDGE('',*,*,#21732,.F.);
#29712=ORIENTED_EDGE('',*,*,#20208,.F.);
#29713=ORIENTED_EDGE('',*,*,#21733,.F.);
#29714=ORIENTED_EDGE('',*,*,#21728,.F.);
#29715=ORIENTED_EDGE('',*,*,#21123,.F.);
#29716=ORIENTED_EDGE('',*,*,#21046,.T.);
#29717=ORIENTED_EDGE('',*,*,#19768,.T.);
#29718=ORIENTED_EDGE('',*,*,#21113,.T.);
#29719=ORIENTED_EDGE('',*,*,#21734,.T.);
#29720=ORIENTED_EDGE('',*,*,#21056,.T.);
#29721=ORIENTED_EDGE('',*,*,#21735,.T.);
#29722=ORIENTED_EDGE('',*,*,#21114,.T.);
#29723=ORIENTED_EDGE('',*,*,#19766,.T.);
#29724=ORIENTED_EDGE('',*,*,#21735,.F.);
#29725=ORIENTED_EDGE('',*,*,#21055,.T.);
#29726=ORIENTED_EDGE('',*,*,#21736,.F.);
#29727=ORIENTED_EDGE('',*,*,#21115,.T.);
#29728=ORIENTED_EDGE('',*,*,#21057,.T.);
#29729=ORIENTED_EDGE('',*,*,#19764,.T.);
#29730=ORIENTED_EDGE('',*,*,#21107,.T.);
#29731=ORIENTED_EDGE('',*,*,#21737,.T.);
#29732=ORIENTED_EDGE('',*,*,#21099,.F.);
#29733=ORIENTED_EDGE('',*,*,#21079,.T.);
#29734=ORIENTED_EDGE('',*,*,#21738,.T.);
#29735=ORIENTED_EDGE('',*,*,#21739,.T.);
#29736=ORIENTED_EDGE('',*,*,#21095,.F.);
#29737=ORIENTED_EDGE('',*,*,#21739,.F.);
#29738=ORIENTED_EDGE('',*,*,#21740,.F.);
#29739=ORIENTED_EDGE('',*,*,#21741,.F.);
#29740=ORIENTED_EDGE('',*,*,#19755,.F.);
#29741=ORIENTED_EDGE('',*,*,#21742,.F.);
#29742=ORIENTED_EDGE('',*,*,#21743,.F.);
#29743=ORIENTED_EDGE('',*,*,#21097,.F.);
#29744=ORIENTED_EDGE('',*,*,#21744,.T.);
#29745=ORIENTED_EDGE('',*,*,#19948,.T.);
#29746=ORIENTED_EDGE('',*,*,#21745,.T.);
#29747=ORIENTED_EDGE('',*,*,#21746,.T.);
#29748=ORIENTED_EDGE('',*,*,#19950,.F.);
#29749=ORIENTED_EDGE('',*,*,#21747,.T.);
#29750=ORIENTED_EDGE('',*,*,#21745,.F.);
#29751=ORIENTED_EDGE('',*,*,#21748,.T.);
#29752=ORIENTED_EDGE('',*,*,#21749,.T.);
#29753=ORIENTED_EDGE('',*,*,#21750,.T.);
#29754=ORIENTED_EDGE('',*,*,#19761,.T.);
#29755=ORIENTED_EDGE('',*,*,#21748,.F.);
#29756=ORIENTED_EDGE('',*,*,#19946,.T.);
#29757=ORIENTED_EDGE('',*,*,#21744,.F.);
#29758=ORIENTED_EDGE('',*,*,#21751,.T.);
#29759=ORIENTED_EDGE('',*,*,#21108,.T.);
#29760=ORIENTED_EDGE('',*,*,#19762,.T.);
#29761=ORIENTED_EDGE('',*,*,#21750,.F.);
#29762=ORIENTED_EDGE('',*,*,#21751,.F.);
#29763=ORIENTED_EDGE('',*,*,#21752,.T.);
#29764=ORIENTED_EDGE('',*,*,#21753,.F.);
#29765=ORIENTED_EDGE('',*,*,#21109,.T.);
#29766=ORIENTED_EDGE('',*,*,#19924,.F.);
#29767=ORIENTED_EDGE('',*,*,#21752,.F.);
#29768=ORIENTED_EDGE('',*,*,#21749,.F.);
#29769=ORIENTED_EDGE('',*,*,#21746,.F.);
#29770=ORIENTED_EDGE('',*,*,#21754,.F.);
#29771=ORIENTED_EDGE('',*,*,#19936,.F.);
#29772=ORIENTED_EDGE('',*,*,#21102,.T.);
#29773=ORIENTED_EDGE('',*,*,#19756,.T.);
#29774=ORIENTED_EDGE('',*,*,#21741,.T.);
#29775=ORIENTED_EDGE('',*,*,#21755,.T.);
#29776=ORIENTED_EDGE('',*,*,#21756,.T.);
#29777=ORIENTED_EDGE('',*,*,#21757,.T.);
#29778=ORIENTED_EDGE('',*,*,#21742,.T.);
#29779=ORIENTED_EDGE('',*,*,#19754,.T.);
#29780=ORIENTED_EDGE('',*,*,#21757,.F.);
#29781=ORIENTED_EDGE('',*,*,#21758,.T.);
#29782=ORIENTED_EDGE('',*,*,#21759,.F.);
#29783=ORIENTED_EDGE('',*,*,#21743,.T.);
#29784=ORIENTED_EDGE('',*,*,#21760,.T.);
#29785=ORIENTED_EDGE('',*,*,#19752,.T.);
#29786=ORIENTED_EDGE('',*,*,#21090,.T.);
#29787=ORIENTED_EDGE('',*,*,#21761,.T.);
#29788=ORIENTED_EDGE('',*,*,#21762,.T.);
#29789=ORIENTED_EDGE('',*,*,#21091,.T.);
#29790=ORIENTED_EDGE('',*,*,#19750,.T.);
#29791=ORIENTED_EDGE('',*,*,#20994,.F.);
#29792=ORIENTED_EDGE('',*,*,#21762,.F.);
#29793=ORIENTED_EDGE('',*,*,#21763,.T.);
#29794=ORIENTED_EDGE('',*,*,#21764,.F.);
#29795=ORIENTED_EDGE('',*,*,#21092,.T.);
#29796=ORIENTED_EDGE('',*,*,#20988,.F.);
#29797=ORIENTED_EDGE('',*,*,#21765,.F.);
#29798=ORIENTED_EDGE('',*,*,#21766,.F.);
#29799=ORIENTED_EDGE('',*,*,#21767,.F.);
#29800=ORIENTED_EDGE('',*,*,#20230,.F.);
#29801=ORIENTED_EDGE('',*,*,#21768,.F.);
#29802=ORIENTED_EDGE('',*,*,#21763,.F.);
#29803=ORIENTED_EDGE('',*,*,#20993,.F.);
#29804=ORIENTED_EDGE('',*,*,#20981,.F.);
#29805=ORIENTED_EDGE('',*,*,#20974,.T.);
#29806=ORIENTED_EDGE('',*,*,#21769,.T.);
#29807=ORIENTED_EDGE('',*,*,#21770,.T.);
#29808=ORIENTED_EDGE('',*,*,#20977,.F.);
#29809=ORIENTED_EDGE('',*,*,#21770,.F.);
#29810=ORIENTED_EDGE('',*,*,#21771,.F.);
#29811=ORIENTED_EDGE('',*,*,#21772,.F.);
#29812=ORIENTED_EDGE('',*,*,#19743,.F.);
#29813=ORIENTED_EDGE('',*,*,#21773,.F.);
#29814=ORIENTED_EDGE('',*,*,#21774,.F.);
#29815=ORIENTED_EDGE('',*,*,#20979,.F.);
#29816=ORIENTED_EDGE('',*,*,#20984,.T.);
#29817=ORIENTED_EDGE('',*,*,#19744,.T.);
#29818=ORIENTED_EDGE('',*,*,#21772,.T.);
#29819=ORIENTED_EDGE('',*,*,#21775,.T.);
#29820=ORIENTED_EDGE('',*,*,#20807,.T.);
#29821=ORIENTED_EDGE('',*,*,#21776,.T.);
#29822=ORIENTED_EDGE('',*,*,#21773,.T.);
#29823=ORIENTED_EDGE('',*,*,#19742,.T.);
#29824=ORIENTED_EDGE('',*,*,#21776,.F.);
#29825=ORIENTED_EDGE('',*,*,#20806,.T.);
#29826=ORIENTED_EDGE('',*,*,#21777,.F.);
#29827=ORIENTED_EDGE('',*,*,#21774,.T.);
#29828=ORIENTED_EDGE('',*,*,#20808,.T.);
#29829=ORIENTED_EDGE('',*,*,#19740,.T.);
#29830=ORIENTED_EDGE('',*,*,#20892,.T.);
#29831=ORIENTED_EDGE('',*,*,#21778,.T.);
#29832=ORIENTED_EDGE('',*,*,#21779,.T.);
#29833=ORIENTED_EDGE('',*,*,#20893,.T.);
#29834=ORIENTED_EDGE('',*,*,#19738,.T.);
#29835=ORIENTED_EDGE('',*,*,#20884,.F.);
#29836=ORIENTED_EDGE('',*,*,#21779,.F.);
#29837=ORIENTED_EDGE('',*,*,#21780,.T.);
#29838=ORIENTED_EDGE('',*,*,#21781,.F.);
#29839=ORIENTED_EDGE('',*,*,#20894,.T.);
#29840=ORIENTED_EDGE('',*,*,#20878,.F.);
#29841=ORIENTED_EDGE('',*,*,#21782,.F.);
#29842=ORIENTED_EDGE('',*,*,#21783,.F.);
#29843=ORIENTED_EDGE('',*,*,#21784,.F.);
#29844=ORIENTED_EDGE('',*,*,#20242,.F.);
#29845=ORIENTED_EDGE('',*,*,#21785,.F.);
#29846=ORIENTED_EDGE('',*,*,#21780,.F.);
#29847=ORIENTED_EDGE('',*,*,#20883,.F.);
#29848=ORIENTED_EDGE('',*,*,#20836,.T.);
#29849=ORIENTED_EDGE('',*,*,#19732,.T.);
#29850=ORIENTED_EDGE('',*,*,#20873,.T.);
#29851=ORIENTED_EDGE('',*,*,#21786,.T.);
#29852=ORIENTED_EDGE('',*,*,#20867,.T.);
#29853=ORIENTED_EDGE('',*,*,#21787,.T.);
#29854=ORIENTED_EDGE('',*,*,#20874,.T.);
#29855=ORIENTED_EDGE('',*,*,#19730,.T.);
#29856=ORIENTED_EDGE('',*,*,#21787,.F.);
#29857=ORIENTED_EDGE('',*,*,#20866,.T.);
#29858=ORIENTED_EDGE('',*,*,#21788,.F.);
#29859=ORIENTED_EDGE('',*,*,#20875,.T.);
#29860=ORIENTED_EDGE('',*,*,#20865,.F.);
#29861=ORIENTED_EDGE('',*,*,#20858,.T.);
#29862=ORIENTED_EDGE('',*,*,#21789,.T.);
#29863=ORIENTED_EDGE('',*,*,#21790,.T.);
#29864=ORIENTED_EDGE('',*,*,#20861,.F.);
#29865=ORIENTED_EDGE('',*,*,#21790,.F.);
#29866=ORIENTED_EDGE('',*,*,#21791,.F.);
#29867=ORIENTED_EDGE('',*,*,#21792,.F.);
#29868=ORIENTED_EDGE('',*,*,#19727,.F.);
#29869=ORIENTED_EDGE('',*,*,#21793,.F.);
#29870=ORIENTED_EDGE('',*,*,#21794,.F.);
#29871=ORIENTED_EDGE('',*,*,#20863,.F.);
#29872=ORIENTED_EDGE('',*,*,#20868,.T.);
#29873=ORIENTED_EDGE('',*,*,#19728,.T.);
#29874=ORIENTED_EDGE('',*,*,#21792,.T.);
#29875=ORIENTED_EDGE('',*,*,#21795,.T.);
#29876=ORIENTED_EDGE('',*,*,#21796,.T.);
#29877=ORIENTED_EDGE('',*,*,#21793,.T.);
#29878=ORIENTED_EDGE('',*,*,#19726,.T.);
#29879=ORIENTED_EDGE('',*,*,#20794,.F.);
#29880=ORIENTED_EDGE('',*,*,#21796,.F.);
#29881=ORIENTED_EDGE('',*,*,#21797,.T.);
#29882=ORIENTED_EDGE('',*,*,#21798,.F.);
#29883=ORIENTED_EDGE('',*,*,#21794,.T.);
#29884=ORIENTED_EDGE('',*,*,#20788,.F.);
#29885=ORIENTED_EDGE('',*,*,#21799,.F.);
#29886=ORIENTED_EDGE('',*,*,#21800,.F.);
#29887=ORIENTED_EDGE('',*,*,#21801,.F.);
#29888=ORIENTED_EDGE('',*,*,#20254,.F.);
#29889=ORIENTED_EDGE('',*,*,#21802,.F.);
#29890=ORIENTED_EDGE('',*,*,#21797,.F.);
#29891=ORIENTED_EDGE('',*,*,#20793,.F.);
#29892=ORIENTED_EDGE('',*,*,#20729,.T.);
#29893=ORIENTED_EDGE('',*,*,#19720,.T.);
#29894=ORIENTED_EDGE('',*,*,#20783,.T.);
#29895=ORIENTED_EDGE('',*,*,#21803,.T.);
#29896=ORIENTED_EDGE('',*,*,#20739,.T.);
#29897=ORIENTED_EDGE('',*,*,#21804,.T.);
#29898=ORIENTED_EDGE('',*,*,#20784,.T.);
#29899=ORIENTED_EDGE('',*,*,#19718,.T.);
#29900=ORIENTED_EDGE('',*,*,#21804,.F.);
#29901=ORIENTED_EDGE('',*,*,#20738,.T.);
#29902=ORIENTED_EDGE('',*,*,#21805,.F.);
#29903=ORIENTED_EDGE('',*,*,#20785,.T.);
#29904=ORIENTED_EDGE('',*,*,#20740,.T.);
#29905=ORIENTED_EDGE('',*,*,#19716,.T.);
#29906=ORIENTED_EDGE('',*,*,#20777,.T.);
#29907=ORIENTED_EDGE('',*,*,#21806,.T.);
#29908=ORIENTED_EDGE('',*,*,#20769,.F.);
#29909=ORIENTED_EDGE('',*,*,#20762,.T.);
#29910=ORIENTED_EDGE('',*,*,#21807,.T.);
#29911=ORIENTED_EDGE('',*,*,#21808,.T.);
#29912=ORIENTED_EDGE('',*,*,#20765,.F.);
#29913=ORIENTED_EDGE('',*,*,#21808,.F.);
#29914=ORIENTED_EDGE('',*,*,#21809,.F.);
#29915=ORIENTED_EDGE('',*,*,#21810,.F.);
#29916=ORIENTED_EDGE('',*,*,#19902,.F.);
#29917=ORIENTED_EDGE('',*,*,#21811,.F.);
#29918=ORIENTED_EDGE('',*,*,#21812,.F.);
#29919=ORIENTED_EDGE('',*,*,#20767,.F.);
#29920=ORIENTED_EDGE('',*,*,#21813,.T.);
#29921=ORIENTED_EDGE('',*,*,#19909,.T.);
#29922=ORIENTED_EDGE('',*,*,#21814,.T.);
#29923=ORIENTED_EDGE('',*,*,#21815,.T.);
#29924=ORIENTED_EDGE('',*,*,#19911,.F.);
#29925=ORIENTED_EDGE('',*,*,#21816,.T.);
#29926=ORIENTED_EDGE('',*,*,#21814,.F.);
#29927=ORIENTED_EDGE('',*,*,#21817,.T.);
#29928=ORIENTED_EDGE('',*,*,#21818,.T.);
#29929=ORIENTED_EDGE('',*,*,#21819,.T.);
#29930=ORIENTED_EDGE('',*,*,#19713,.T.);
#29931=ORIENTED_EDGE('',*,*,#21817,.F.);
#29932=ORIENTED_EDGE('',*,*,#19907,.T.);
#29933=ORIENTED_EDGE('',*,*,#21813,.F.);
#29934=ORIENTED_EDGE('',*,*,#21820,.T.);
#29935=ORIENTED_EDGE('',*,*,#20778,.T.);
#29936=ORIENTED_EDGE('',*,*,#19714,.T.);
#29937=ORIENTED_EDGE('',*,*,#21819,.F.);
#29938=ORIENTED_EDGE('',*,*,#21820,.F.);
#29939=ORIENTED_EDGE('',*,*,#21821,.T.);
#29940=ORIENTED_EDGE('',*,*,#21822,.F.);
#29941=ORIENTED_EDGE('',*,*,#20779,.T.);
#29942=ORIENTED_EDGE('',*,*,#19690,.F.);
#29943=ORIENTED_EDGE('',*,*,#21821,.F.);
#29944=ORIENTED_EDGE('',*,*,#21818,.F.);
#29945=ORIENTED_EDGE('',*,*,#21815,.F.);
#29946=ORIENTED_EDGE('',*,*,#21823,.F.);
#29947=ORIENTED_EDGE('',*,*,#19702,.F.);
#29948=ORIENTED_EDGE('',*,*,#20772,.T.);
#29949=ORIENTED_EDGE('',*,*,#19903,.T.);
#29950=ORIENTED_EDGE('',*,*,#21810,.T.);
#29951=ORIENTED_EDGE('',*,*,#21824,.T.);
#29952=ORIENTED_EDGE('',*,*,#20620,.T.);
#29953=ORIENTED_EDGE('',*,*,#21825,.T.);
#29954=ORIENTED_EDGE('',*,*,#21811,.T.);
#29955=ORIENTED_EDGE('',*,*,#19901,.T.);
#29956=ORIENTED_EDGE('',*,*,#21825,.F.);
#29957=ORIENTED_EDGE('',*,*,#20619,.T.);
#29958=ORIENTED_EDGE('',*,*,#21826,.F.);
#29959=ORIENTED_EDGE('',*,*,#21812,.T.);
#29960=ORIENTED_EDGE('',*,*,#20621,.T.);
#29961=ORIENTED_EDGE('',*,*,#19899,.T.);
#29962=ORIENTED_EDGE('',*,*,#20658,.T.);
#29963=ORIENTED_EDGE('',*,*,#21827,.T.);
#29964=ORIENTED_EDGE('',*,*,#20650,.F.);
#29965=ORIENTED_EDGE('',*,*,#20643,.T.);
#29966=ORIENTED_EDGE('',*,*,#21828,.T.);
#29967=ORIENTED_EDGE('',*,*,#21829,.T.);
#29968=ORIENTED_EDGE('',*,*,#20646,.F.);
#29969=ORIENTED_EDGE('',*,*,#21829,.F.);
#29970=ORIENTED_EDGE('',*,*,#21830,.F.);
#29971=ORIENTED_EDGE('',*,*,#21831,.F.);
#29972=ORIENTED_EDGE('',*,*,#19890,.F.);
#29973=ORIENTED_EDGE('',*,*,#21832,.F.);
#29974=ORIENTED_EDGE('',*,*,#21833,.F.);
#29975=ORIENTED_EDGE('',*,*,#20648,.F.);
#29976=ORIENTED_EDGE('',*,*,#21834,.T.);
#29977=ORIENTED_EDGE('',*,*,#20569,.T.);
#29978=ORIENTED_EDGE('',*,*,#21835,.T.);
#29979=ORIENTED_EDGE('',*,*,#21836,.T.);
#29980=ORIENTED_EDGE('',*,*,#20565,.F.);
#29981=ORIENTED_EDGE('',*,*,#21837,.T.);
#29982=ORIENTED_EDGE('',*,*,#21838,.T.);
#29983=ORIENTED_EDGE('',*,*,#20568,.T.);
#29984=ORIENTED_EDGE('',*,*,#21838,.F.);
#29985=ORIENTED_EDGE('',*,*,#21839,.T.);
#29986=ORIENTED_EDGE('',*,*,#21835,.F.);
#29987=ORIENTED_EDGE('',*,*,#19896,.T.);
#29988=ORIENTED_EDGE('',*,*,#21840,.T.);
#29989=ORIENTED_EDGE('',*,*,#21841,.T.);
#29990=ORIENTED_EDGE('',*,*,#21842,.T.);
#29991=ORIENTED_EDGE('',*,*,#21843,.T.);
#29992=ORIENTED_EDGE('',*,*,#20659,.T.);
#29993=ORIENTED_EDGE('',*,*,#19897,.T.);
#29994=ORIENTED_EDGE('',*,*,#21842,.F.);
#29995=ORIENTED_EDGE('',*,*,#21840,.F.);
#29996=ORIENTED_EDGE('',*,*,#20567,.T.);
#29997=ORIENTED_EDGE('',*,*,#21834,.F.);
#29998=ORIENTED_EDGE('',*,*,#20555,.F.);
#29999=ORIENTED_EDGE('',*,*,#21844,.F.);
#30000=ORIENTED_EDGE('',*,*,#21845,.F.);
#30001=ORIENTED_EDGE('',*,*,#20097,.F.);
#30002=ORIENTED_EDGE('',*,*,#21846,.F.);
#30003=ORIENTED_EDGE('',*,*,#21847,.F.);
#30004=ORIENTED_EDGE('',*,*,#20564,.F.);
#30005=ORIENTED_EDGE('',*,*,#20559,.F.);
#30006=ORIENTED_EDGE('',*,*,#21836,.F.);
#30007=ORIENTED_EDGE('',*,*,#21848,.F.);
#30008=ORIENTED_EDGE('',*,*,#21849,.F.);
#30009=ORIENTED_EDGE('',*,*,#21850,.F.);
#30010=ORIENTED_EDGE('',*,*,#20095,.F.);
#30011=ORIENTED_EDGE('',*,*,#21851,.F.);
#30012=ORIENTED_EDGE('',*,*,#21852,.F.);
#30013=ORIENTED_EDGE('',*,*,#21841,.F.);
#30014=ORIENTED_EDGE('',*,*,#20653,.T.);
#30015=ORIENTED_EDGE('',*,*,#19891,.T.);
#30016=ORIENTED_EDGE('',*,*,#21831,.T.);
#30017=ORIENTED_EDGE('',*,*,#21853,.T.);
#30018=ORIENTED_EDGE('',*,*,#20501,.T.);
#30019=ORIENTED_EDGE('',*,*,#21854,.T.);
#30020=ORIENTED_EDGE('',*,*,#21832,.T.);
#30021=ORIENTED_EDGE('',*,*,#19889,.T.);
#30022=ORIENTED_EDGE('',*,*,#21854,.F.);
#30023=ORIENTED_EDGE('',*,*,#20500,.T.);
#30024=ORIENTED_EDGE('',*,*,#21855,.F.);
#30025=ORIENTED_EDGE('',*,*,#21833,.T.);
#30026=ORIENTED_EDGE('',*,*,#20502,.T.);
#30027=ORIENTED_EDGE('',*,*,#19887,.T.);
#30028=ORIENTED_EDGE('',*,*,#20550,.T.);
#30029=ORIENTED_EDGE('',*,*,#21856,.T.);
#30030=ORIENTED_EDGE('',*,*,#21857,.T.);
#30031=ORIENTED_EDGE('',*,*,#20551,.T.);
#30032=ORIENTED_EDGE('',*,*,#19885,.T.);
#30033=ORIENTED_EDGE('',*,*,#20542,.F.);
#30034=ORIENTED_EDGE('',*,*,#21857,.F.);
#30035=ORIENTED_EDGE('',*,*,#21858,.T.);
#30036=ORIENTED_EDGE('',*,*,#21859,.F.);
#30037=ORIENTED_EDGE('',*,*,#20552,.T.);
#30038=ORIENTED_EDGE('',*,*,#20536,.F.);
#30039=ORIENTED_EDGE('',*,*,#21860,.F.);
#30040=ORIENTED_EDGE('',*,*,#21861,.F.);
#30041=ORIENTED_EDGE('',*,*,#21862,.F.);
#30042=ORIENTED_EDGE('',*,*,#20107,.F.);
#30043=ORIENTED_EDGE('',*,*,#21863,.F.);
#30044=ORIENTED_EDGE('',*,*,#21858,.F.);
#30045=ORIENTED_EDGE('',*,*,#20541,.F.);
#30046=ORIENTED_EDGE('',*,*,#21864,.T.);
#30047=ORIENTED_EDGE('',*,*,#19879,.T.);
#30048=ORIENTED_EDGE('',*,*,#20531,.T.);
#30049=ORIENTED_EDGE('',*,*,#21865,.T.);
#30050=ORIENTED_EDGE('',*,*,#20467,.F.);
#30051=ORIENTED_EDGE('',*,*,#20394,.T.);
#30052=ORIENTED_EDGE('',*,*,#21866,.T.);
#30053=ORIENTED_EDGE('',*,*,#21867,.T.);
#30054=ORIENTED_EDGE('',*,*,#20463,.F.);
#30055=ORIENTED_EDGE('',*,*,#21867,.F.);
#30056=ORIENTED_EDGE('',*,*,#21868,.F.);
#30057=ORIENTED_EDGE('',*,*,#21869,.F.);
#30058=ORIENTED_EDGE('',*,*,#19874,.F.);
#30059=ORIENTED_EDGE('',*,*,#21870,.F.);
#30060=ORIENTED_EDGE('',*,*,#21871,.F.);
#30061=ORIENTED_EDGE('',*,*,#20465,.F.);
#30062=ORIENTED_EDGE('',*,*,#20469,.T.);
#30063=ORIENTED_EDGE('',*,*,#21872,.T.);
#30064=ORIENTED_EDGE('',*,*,#20532,.T.);
#30065=ORIENTED_EDGE('',*,*,#19877,.T.);
#30066=ORIENTED_EDGE('',*,*,#21872,.F.);
#30067=ORIENTED_EDGE('',*,*,#20468,.T.);
#30068=ORIENTED_EDGE('',*,*,#21873,.F.);
#30069=ORIENTED_EDGE('',*,*,#20533,.T.);
#30070=ORIENTED_EDGE('',*,*,#20470,.T.);
#30071=ORIENTED_EDGE('',*,*,#19875,.T.);
#30072=ORIENTED_EDGE('',*,*,#21869,.T.);
#30073=ORIENTED_EDGE('',*,*,#21874,.T.);
#30074=ORIENTED_EDGE('',*,*,#21875,.T.);
#30075=ORIENTED_EDGE('',*,*,#21870,.T.);
#30076=ORIENTED_EDGE('',*,*,#19873,.T.);
#30077=ORIENTED_EDGE('',*,*,#20456,.F.);
#30078=ORIENTED_EDGE('',*,*,#21875,.F.);
#30079=ORIENTED_EDGE('',*,*,#21876,.T.);
#30080=ORIENTED_EDGE('',*,*,#21877,.F.);
#30081=ORIENTED_EDGE('',*,*,#21871,.T.);
#30082=ORIENTED_EDGE('',*,*,#20450,.F.);
#30083=ORIENTED_EDGE('',*,*,#21878,.F.);
#30084=ORIENTED_EDGE('',*,*,#21879,.F.);
#30085=ORIENTED_EDGE('',*,*,#21880,.F.);
#30086=ORIENTED_EDGE('',*,*,#20119,.F.);
#30087=ORIENTED_EDGE('',*,*,#21881,.F.);
#30088=ORIENTED_EDGE('',*,*,#21876,.F.);
#30089=ORIENTED_EDGE('',*,*,#20455,.F.);
#30090=ORIENTED_EDGE('',*,*,#21882,.T.);
#30091=ORIENTED_EDGE('',*,*,#20135,.T.);
#30092=ORIENTED_EDGE('',*,*,#21883,.T.);
#30093=ORIENTED_EDGE('',*,*,#21884,.T.);
#30094=ORIENTED_EDGE('',*,*,#21885,.T.);
#30095=ORIENTED_EDGE('',*,*,#21886,.T.);
#30096=ORIENTED_EDGE('',*,*,#21887,.T.);
#30097=ORIENTED_EDGE('',*,*,#21888,.T.);
#30098=ORIENTED_EDGE('',*,*,#21887,.F.);
#30099=ORIENTED_EDGE('',*,*,#21889,.T.);
#30100=ORIENTED_EDGE('',*,*,#21882,.F.);
#30101=ORIENTED_EDGE('',*,*,#21890,.T.);
#30102=ORIENTED_EDGE('',*,*,#21891,.T.);
#30103=ORIENTED_EDGE('',*,*,#21892,.T.);
#30104=ORIENTED_EDGE('',*,*,#21893,.T.);
#30105=ORIENTED_EDGE('',*,*,#21894,.T.);
#30106=ORIENTED_EDGE('',*,*,#21895,.T.);
#30107=ORIENTED_EDGE('',*,*,#21896,.T.);
#30108=ORIENTED_EDGE('',*,*,#21897,.T.);
#30109=ORIENTED_EDGE('',*,*,#21894,.F.);
#30110=ORIENTED_EDGE('',*,*,#21891,.F.);
#30111=ORIENTED_EDGE('',*,*,#21898,.T.);
#30112=ORIENTED_EDGE('',*,*,#21885,.F.);
#30113=ORIENTED_EDGE('',*,*,#21614,.F.);
#30114=ORIENTED_EDGE('',*,*,#21899,.T.);
#30115=ORIENTED_EDGE('',*,*,#21896,.F.);
#30116=ORIENTED_EDGE('',*,*,#21889,.F.);
#30117=ORIENTED_EDGE('',*,*,#21900,.T.);
#30118=ORIENTED_EDGE('',*,*,#21901,.F.);
#30119=ORIENTED_EDGE('',*,*,#20136,.T.);
#30120=ORIENTED_EDGE('',*,*,#21886,.F.);
#30121=ORIENTED_EDGE('',*,*,#21902,.F.);
#30122=ORIENTED_EDGE('',*,*,#21903,.F.);
#30123=ORIENTED_EDGE('',*,*,#21900,.F.);
#30124=ORIENTED_EDGE('',*,*,#21898,.F.);
#30125=ORIENTED_EDGE('',*,*,#21904,.T.);
#30126=ORIENTED_EDGE('',*,*,#21905,.T.);
#30127=ORIENTED_EDGE('',*,*,#21902,.T.);
#30128=ORIENTED_EDGE('',*,*,#21890,.F.);
#30129=ORIENTED_EDGE('',*,*,#21897,.F.);
#30130=ORIENTED_EDGE('',*,*,#21906,.F.);
#30131=ORIENTED_EDGE('',*,*,#21904,.F.);
#30132=ORIENTED_EDGE('',*,*,#21899,.F.);
#30133=ORIENTED_EDGE('',*,*,#21619,.T.);
#30134=ORIENTED_EDGE('',*,*,#21907,.F.);
#30135=ORIENTED_EDGE('',*,*,#21906,.T.);
#30136=ORIENTED_EDGE('',*,*,#21908,.T.);
#30137=ORIENTED_EDGE('',*,*,#20131,.T.);
#30138=ORIENTED_EDGE('',*,*,#21909,.T.);
#30139=ORIENTED_EDGE('',*,*,#21910,.T.);
#30140=ORIENTED_EDGE('',*,*,#21911,.T.);
#30141=ORIENTED_EDGE('',*,*,#19855,.T.);
#30142=ORIENTED_EDGE('',*,*,#21912,.T.);
#30143=ORIENTED_EDGE('',*,*,#21913,.T.);
#30144=ORIENTED_EDGE('',*,*,#21914,.T.);
#30145=ORIENTED_EDGE('',*,*,#21915,.T.);
#30146=ORIENTED_EDGE('',*,*,#21916,.T.);
#30147=ORIENTED_EDGE('',*,*,#21917,.T.);
#30148=ORIENTED_EDGE('',*,*,#21916,.F.);
#30149=ORIENTED_EDGE('',*,*,#21918,.T.);
#30150=ORIENTED_EDGE('',*,*,#21911,.F.);
#30151=ORIENTED_EDGE('',*,*,#21919,.T.);
#30152=ORIENTED_EDGE('',*,*,#21920,.T.);
#30153=ORIENTED_EDGE('',*,*,#21921,.T.);
#30154=ORIENTED_EDGE('',*,*,#21922,.T.);
#30155=ORIENTED_EDGE('',*,*,#21923,.T.);
#30156=ORIENTED_EDGE('',*,*,#21924,.T.);
#30157=ORIENTED_EDGE('',*,*,#21925,.T.);
#30158=ORIENTED_EDGE('',*,*,#21926,.T.);
#30159=ORIENTED_EDGE('',*,*,#21922,.F.);
#30160=ORIENTED_EDGE('',*,*,#21924,.F.);
#30161=ORIENTED_EDGE('',*,*,#21927,.T.);
#30162=ORIENTED_EDGE('',*,*,#21914,.F.);
#30163=ORIENTED_EDGE('',*,*,#21928,.T.);
#30164=ORIENTED_EDGE('',*,*,#21929,.T.);
#30165=ORIENTED_EDGE('',*,*,#21930,.T.);
#30166=ORIENTED_EDGE('',*,*,#21931,.T.);
#30167=ORIENTED_EDGE('',*,*,#21928,.F.);
#30168=ORIENTED_EDGE('',*,*,#21932,.T.);
#30169=ORIENTED_EDGE('',*,*,#21920,.F.);
#30170=ORIENTED_EDGE('',*,*,#21930,.F.);
#30171=ORIENTED_EDGE('',*,*,#21933,.T.);
#30172=ORIENTED_EDGE('',*,*,#21908,.F.);
#30173=ORIENTED_EDGE('',*,*,#21923,.F.);
#30174=ORIENTED_EDGE('',*,*,#21921,.F.);
#30175=ORIENTED_EDGE('',*,*,#21934,.F.);
#30176=ORIENTED_EDGE('',*,*,#21935,.F.);
#30177=ORIENTED_EDGE('',*,*,#21932,.F.);
#30178=ORIENTED_EDGE('',*,*,#21936,.T.);
#30179=ORIENTED_EDGE('',*,*,#21937,.F.);
#30180=ORIENTED_EDGE('',*,*,#21934,.T.);
#30181=ORIENTED_EDGE('',*,*,#21931,.F.);
#30182=ORIENTED_EDGE('',*,*,#21910,.F.);
#30183=ORIENTED_EDGE('',*,*,#21938,.F.);
#30184=ORIENTED_EDGE('',*,*,#21939,.F.);
#30185=ORIENTED_EDGE('',*,*,#19858,.F.);
#30186=ORIENTED_EDGE('',*,*,#21940,.F.);
#30187=ORIENTED_EDGE('',*,*,#21936,.F.);
#30188=ORIENTED_EDGE('',*,*,#21933,.F.);
#30189=ORIENTED_EDGE('',*,*,#21941,.T.);
#30190=ORIENTED_EDGE('',*,*,#21942,.T.);
#30191=ORIENTED_EDGE('',*,*,#20132,.T.);
#30192=ORIENTED_EDGE('',*,*,#21929,.F.);
#30193=ORIENTED_EDGE('',*,*,#21919,.F.);
#30194=ORIENTED_EDGE('',*,*,#21926,.F.);
#30195=ORIENTED_EDGE('',*,*,#21943,.T.);
#30196=ORIENTED_EDGE('',*,*,#21941,.F.);
#30197=ORIENTED_EDGE('',*,*,#21918,.F.);
#30198=ORIENTED_EDGE('',*,*,#21944,.T.);
#30199=ORIENTED_EDGE('',*,*,#21945,.T.);
#30200=ORIENTED_EDGE('',*,*,#19856,.T.);
#30201=ORIENTED_EDGE('',*,*,#21946,.T.);
#30202=ORIENTED_EDGE('',*,*,#21947,.T.);
#30203=ORIENTED_EDGE('',*,*,#21940,.T.);
#30204=ORIENTED_EDGE('',*,*,#19857,.T.);
#30205=ORIENTED_EDGE('',*,*,#21945,.F.);
#30206=ORIENTED_EDGE('',*,*,#21927,.F.);
#30207=ORIENTED_EDGE('',*,*,#21935,.T.);
#30208=ORIENTED_EDGE('',*,*,#21948,.T.);
#30209=ORIENTED_EDGE('',*,*,#21949,.T.);
#30210=ORIENTED_EDGE('',*,*,#21948,.F.);
#30211=ORIENTED_EDGE('',*,*,#21937,.T.);
#30212=ORIENTED_EDGE('',*,*,#21947,.F.);
#30213=ORIENTED_EDGE('',*,*,#21915,.F.);
#30214=ORIENTED_EDGE('',*,*,#21949,.F.);
#30215=ORIENTED_EDGE('',*,*,#21946,.F.);
#30216=ORIENTED_EDGE('',*,*,#21944,.F.);
#30217=ORIENTED_EDGE('',*,*,#21913,.F.);
#30218=ORIENTED_EDGE('',*,*,#21950,.F.);
#30219=ORIENTED_EDGE('',*,*,#21951,.F.);
#30220=ORIENTED_EDGE('',*,*,#20133,.F.);
#30221=ORIENTED_EDGE('',*,*,#21942,.F.);
#30222=ORIENTED_EDGE('',*,*,#21943,.F.);
#30223=ORIENTED_EDGE('',*,*,#21925,.F.);
#30224=ORIENTED_EDGE('',*,*,#21917,.F.);
#30225=ORIENTED_EDGE('',*,*,#21952,.T.);
#30226=ORIENTED_EDGE('',*,*,#21903,.T.);
#30227=ORIENTED_EDGE('',*,*,#21953,.T.);
#30228=ORIENTED_EDGE('',*,*,#21618,.T.);
#30229=ORIENTED_EDGE('',*,*,#21954,.T.);
#30230=ORIENTED_EDGE('',*,*,#21617,.T.);
#30231=ORIENTED_EDGE('',*,*,#21955,.T.);
#30232=ORIENTED_EDGE('',*,*,#20137,.T.);
#30233=ORIENTED_EDGE('',*,*,#21954,.F.);
#30234=ORIENTED_EDGE('',*,*,#21901,.T.);
#30235=ORIENTED_EDGE('',*,*,#21952,.F.);
#30236=ORIENTED_EDGE('',*,*,#21905,.F.);
#30237=ORIENTED_EDGE('',*,*,#21907,.T.);
#30238=ORIENTED_EDGE('',*,*,#21953,.F.);
#30239=ORIENTED_EDGE('',*,*,#21956,.T.);
#30240=ORIENTED_EDGE('',*,*,#21957,.T.);
#30241=ORIENTED_EDGE('',*,*,#21958,.T.);
#30242=ORIENTED_EDGE('',*,*,#19905,.T.);
#30243=ORIENTED_EDGE('',*,*,#21958,.F.);
#30244=ORIENTED_EDGE('',*,*,#21956,.F.);
#30245=ORIENTED_EDGE('',*,*,#21957,.F.);
#30246=ORIENTED_EDGE('',*,*,#21959,.T.);
#30247=ORIENTED_EDGE('',*,*,#21960,.F.);
#30248=ORIENTED_EDGE('',*,*,#21961,.F.);
#30249=ORIENTED_EDGE('',*,*,#21959,.F.);
#30250=ORIENTED_EDGE('',*,*,#20422,.F.);
#30251=ORIENTED_EDGE('',*,*,#21962,.T.);
#30252=ORIENTED_EDGE('',*,*,#21963,.T.);
#30253=ORIENTED_EDGE('',*,*,#19861,.T.);
#30254=ORIENTED_EDGE('',*,*,#21964,.T.);
#30255=ORIENTED_EDGE('',*,*,#21965,.T.);
#30256=ORIENTED_EDGE('',*,*,#20444,.T.);
#30257=ORIENTED_EDGE('',*,*,#19862,.T.);
#30258=ORIENTED_EDGE('',*,*,#21963,.F.);
#30259=ORIENTED_EDGE('',*,*,#20431,.F.);
#30260=ORIENTED_EDGE('',*,*,#20439,.T.);
#30261=ORIENTED_EDGE('',*,*,#21966,.T.);
#30262=ORIENTED_EDGE('',*,*,#21967,.T.);
#30263=ORIENTED_EDGE('',*,*,#21966,.F.);
#30264=ORIENTED_EDGE('',*,*,#20441,.T.);
#30265=ORIENTED_EDGE('',*,*,#21965,.F.);
#30266=ORIENTED_EDGE('',*,*,#20327,.F.);
#30267=ORIENTED_EDGE('',*,*,#21968,.T.);
#30268=ORIENTED_EDGE('',*,*,#21969,.T.);
#30269=ORIENTED_EDGE('',*,*,#19866,.T.);
#30270=ORIENTED_EDGE('',*,*,#21970,.T.);
#30271=ORIENTED_EDGE('',*,*,#21971,.T.);
#30272=ORIENTED_EDGE('',*,*,#20349,.T.);
#30273=ORIENTED_EDGE('',*,*,#19867,.T.);
#30274=ORIENTED_EDGE('',*,*,#21969,.F.);
#30275=ORIENTED_EDGE('',*,*,#20336,.F.);
#30276=ORIENTED_EDGE('',*,*,#20344,.T.);
#30277=ORIENTED_EDGE('',*,*,#21972,.T.);
#30278=ORIENTED_EDGE('',*,*,#21973,.T.);
#30279=ORIENTED_EDGE('',*,*,#21972,.F.);
#30280=ORIENTED_EDGE('',*,*,#20346,.T.);
#30281=ORIENTED_EDGE('',*,*,#21971,.F.);
#30282=ORIENTED_EDGE('',*,*,#20324,.F.);
#30283=ORIENTED_EDGE('',*,*,#21973,.F.);
#30284=ORIENTED_EDGE('',*,*,#21970,.F.);
#30285=ORIENTED_EDGE('',*,*,#21968,.F.);
#30286=ORIENTED_EDGE('',*,*,#20443,.T.);
#30287=ORIENTED_EDGE('',*,*,#21974,.T.);
#30288=ORIENTED_EDGE('',*,*,#20321,.F.);
#30289=ORIENTED_EDGE('',*,*,#19864,.T.);
#30290=ORIENTED_EDGE('',*,*,#21974,.F.);
#30291=ORIENTED_EDGE('',*,*,#20442,.T.);
#30292=ORIENTED_EDGE('',*,*,#21975,.F.);
#30293=ORIENTED_EDGE('',*,*,#21976,.T.);
#30294=ORIENTED_EDGE('',*,*,#20419,.F.);
#30295=ORIENTED_EDGE('',*,*,#21967,.F.);
#30296=ORIENTED_EDGE('',*,*,#21964,.F.);
#30297=ORIENTED_EDGE('',*,*,#21962,.F.);
#30298=ORIENTED_EDGE('',*,*,#21939,.T.);
#30299=ORIENTED_EDGE('',*,*,#21977,.T.);
#30300=ORIENTED_EDGE('',*,*,#20416,.F.);
#30301=ORIENTED_EDGE('',*,*,#19859,.T.);
#30302=ORIENTED_EDGE('',*,*,#21977,.F.);
#30303=ORIENTED_EDGE('',*,*,#21938,.T.);
#30304=ORIENTED_EDGE('',*,*,#21978,.F.);
#30305=ORIENTED_EDGE('',*,*,#21979,.T.);
#30306=ORIENTED_EDGE('',*,*,#20266,.T.);
#30307=ORIENTED_EDGE('',*,*,#21980,.T.);
#30308=ORIENTED_EDGE('',*,*,#21960,.T.);
#30309=ORIENTED_EDGE('',*,*,#21961,.T.);
#30310=ORIENTED_EDGE('',*,*,#21980,.F.);
#30311=ORIENTED_EDGE('',*,*,#21981,.T.);
#30312=ORIENTED_EDGE('',*,*,#21982,.T.);
#30313=ORIENTED_EDGE('',*,*,#21912,.F.);
#30314=ORIENTED_EDGE('',*,*,#19854,.T.);
#30315=ORIENTED_EDGE('',*,*,#21982,.F.);
#30316=ORIENTED_EDGE('',*,*,#21983,.T.);
#30317=ORIENTED_EDGE('',*,*,#21984,.F.);
#30318=ORIENTED_EDGE('',*,*,#21950,.T.);
#30319=ORIENTED_EDGE('',*,*,#21951,.T.);
#30320=ORIENTED_EDGE('',*,*,#21984,.T.);
#30321=ORIENTED_EDGE('',*,*,#21883,.F.);
#30322=ORIENTED_EDGE('',*,*,#20134,.T.);
#30323=ORIENTED_EDGE('',*,*,#21985,.T.);
#30324=ORIENTED_EDGE('',*,*,#21978,.T.);
#30325=ORIENTED_EDGE('',*,*,#21909,.F.);
#30326=ORIENTED_EDGE('',*,*,#20130,.T.);
#30327=ORIENTED_EDGE('',*,*,#21986,.T.);
#30328=ORIENTED_EDGE('',*,*,#21975,.T.);
#30329=ORIENTED_EDGE('',*,*,#20413,.F.);
#30330=ORIENTED_EDGE('',*,*,#20126,.T.);
#30331=ORIENTED_EDGE('',*,*,#20453,.F.);
#30332=ORIENTED_EDGE('',*,*,#21987,.T.);
#30333=ORIENTED_EDGE('',*,*,#21988,.T.);
#30334=ORIENTED_EDGE('',*,*,#21878,.T.);
#30335=ORIENTED_EDGE('',*,*,#20348,.T.);
#30336=ORIENTED_EDGE('',*,*,#21989,.T.);
#30337=ORIENTED_EDGE('',*,*,#20396,.F.);
#30338=ORIENTED_EDGE('',*,*,#19869,.T.);
#30339=ORIENTED_EDGE('',*,*,#21989,.F.);
#30340=ORIENTED_EDGE('',*,*,#20347,.T.);
#30341=ORIENTED_EDGE('',*,*,#21990,.F.);
#30342=ORIENTED_EDGE('',*,*,#20457,.T.);
#30343=ORIENTED_EDGE('',*,*,#20458,.T.);
#30344=ORIENTED_EDGE('',*,*,#21990,.T.);
#30345=ORIENTED_EDGE('',*,*,#20318,.F.);
#30346=ORIENTED_EDGE('',*,*,#20122,.T.);
#30347=ORIENTED_EDGE('',*,*,#21880,.T.);
#30348=ORIENTED_EDGE('',*,*,#21991,.T.);
#30349=ORIENTED_EDGE('',*,*,#20459,.T.);
#30350=ORIENTED_EDGE('',*,*,#20120,.T.);
#30351=ORIENTED_EDGE('',*,*,#21877,.T.);
#30352=ORIENTED_EDGE('',*,*,#21881,.T.);
#30353=ORIENTED_EDGE('',*,*,#20118,.T.);
#30354=ORIENTED_EDGE('',*,*,#20466,.F.);
#30355=ORIENTED_EDGE('',*,*,#21873,.T.);
#30356=ORIENTED_EDGE('',*,*,#20375,.F.);
#30357=ORIENTED_EDGE('',*,*,#20114,.T.);
#30358=ORIENTED_EDGE('',*,*,#20526,.F.);
#30359=ORIENTED_EDGE('',*,*,#20298,.F.);
#30360=ORIENTED_EDGE('',*,*,#21992,.F.);
#30361=ORIENTED_EDGE('',*,*,#21993,.F.);
#30362=ORIENTED_EDGE('',*,*,#19880,.F.);
#30363=ORIENTED_EDGE('',*,*,#21864,.F.);
#30364=ORIENTED_EDGE('',*,*,#21994,.F.);
#30365=ORIENTED_EDGE('',*,*,#20307,.F.);
#30366=ORIENTED_EDGE('',*,*,#20302,.F.);
#30367=ORIENTED_EDGE('',*,*,#20539,.F.);
#30368=ORIENTED_EDGE('',*,*,#21995,.T.);
#30369=ORIENTED_EDGE('',*,*,#21996,.T.);
#30370=ORIENTED_EDGE('',*,*,#21860,.T.);
#30371=ORIENTED_EDGE('',*,*,#21993,.T.);
#30372=ORIENTED_EDGE('',*,*,#21997,.T.);
#30373=ORIENTED_EDGE('',*,*,#20505,.F.);
#30374=ORIENTED_EDGE('',*,*,#19881,.T.);
#30375=ORIENTED_EDGE('',*,*,#21997,.F.);
#30376=ORIENTED_EDGE('',*,*,#21992,.T.);
#30377=ORIENTED_EDGE('',*,*,#21998,.F.);
#30378=ORIENTED_EDGE('',*,*,#20543,.T.);
#30379=ORIENTED_EDGE('',*,*,#20544,.T.);
#30380=ORIENTED_EDGE('',*,*,#21998,.T.);
#30381=ORIENTED_EDGE('',*,*,#20297,.F.);
#30382=ORIENTED_EDGE('',*,*,#20110,.T.);
#30383=ORIENTED_EDGE('',*,*,#21862,.T.);
#30384=ORIENTED_EDGE('',*,*,#21999,.T.);
#30385=ORIENTED_EDGE('',*,*,#20545,.T.);
#30386=ORIENTED_EDGE('',*,*,#20108,.T.);
#30387=ORIENTED_EDGE('',*,*,#21859,.T.);
#30388=ORIENTED_EDGE('',*,*,#21863,.T.);
#30389=ORIENTED_EDGE('',*,*,#20106,.T.);
#30390=ORIENTED_EDGE('',*,*,#20498,.F.);
#30391=ORIENTED_EDGE('',*,*,#21855,.T.);
#30392=ORIENTED_EDGE('',*,*,#20354,.F.);
#30393=ORIENTED_EDGE('',*,*,#20102,.T.);
#30394=ORIENTED_EDGE('',*,*,#20649,.F.);
#30395=ORIENTED_EDGE('',*,*,#21839,.F.);
#30396=ORIENTED_EDGE('',*,*,#22000,.T.);
#30397=ORIENTED_EDGE('',*,*,#22001,.T.);
#30398=ORIENTED_EDGE('',*,*,#21848,.T.);
#30399=ORIENTED_EDGE('',*,*,#20652,.T.);
#30400=ORIENTED_EDGE('',*,*,#22002,.T.);
#30401=ORIENTED_EDGE('',*,*,#20554,.F.);
#30402=ORIENTED_EDGE('',*,*,#19893,.T.);
#30403=ORIENTED_EDGE('',*,*,#22002,.F.);
#30404=ORIENTED_EDGE('',*,*,#20651,.T.);
#30405=ORIENTED_EDGE('',*,*,#22003,.F.);
#30406=ORIENTED_EDGE('',*,*,#21844,.T.);
#30407=ORIENTED_EDGE('',*,*,#21845,.T.);
#30408=ORIENTED_EDGE('',*,*,#22003,.T.);
#30409=ORIENTED_EDGE('',*,*,#20624,.F.);
#30410=ORIENTED_EDGE('',*,*,#20098,.T.);
#30411=ORIENTED_EDGE('',*,*,#21850,.T.);
#30412=ORIENTED_EDGE('',*,*,#22004,.T.);
#30413=ORIENTED_EDGE('',*,*,#21846,.T.);
#30414=ORIENTED_EDGE('',*,*,#20096,.T.);
#30415=ORIENTED_EDGE('',*,*,#22005,.T.);
#30416=ORIENTED_EDGE('',*,*,#21851,.T.);
#30417=ORIENTED_EDGE('',*,*,#20094,.T.);
#30418=ORIENTED_EDGE('',*,*,#20617,.F.);
#30419=ORIENTED_EDGE('',*,*,#21843,.F.);
#30420=ORIENTED_EDGE('',*,*,#21852,.T.);
#30421=ORIENTED_EDGE('',*,*,#22005,.F.);
#30422=ORIENTED_EDGE('',*,*,#20660,.T.);
#30423=ORIENTED_EDGE('',*,*,#21826,.T.);
#30424=ORIENTED_EDGE('',*,*,#20473,.F.);
#30425=ORIENTED_EDGE('',*,*,#20090,.T.);
#30426=ORIENTED_EDGE('',*,*,#20768,.F.);
#30427=ORIENTED_EDGE('',*,*,#19703,.F.);
#30428=ORIENTED_EDGE('',*,*,#21823,.T.);
#30429=ORIENTED_EDGE('',*,*,#21816,.F.);
#30430=ORIENTED_EDGE('',*,*,#19912,.T.);
#30431=ORIENTED_EDGE('',*,*,#20771,.T.);
#30432=ORIENTED_EDGE('',*,*,#22006,.T.);
#30433=ORIENTED_EDGE('',*,*,#19680,.F.);
#30434=ORIENTED_EDGE('',*,*,#19711,.T.);
#30435=ORIENTED_EDGE('',*,*,#22006,.F.);
#30436=ORIENTED_EDGE('',*,*,#20770,.T.);
#30437=ORIENTED_EDGE('',*,*,#22007,.F.);
#30438=ORIENTED_EDGE('',*,*,#19706,.T.);
#30439=ORIENTED_EDGE('',*,*,#19707,.T.);
#30440=ORIENTED_EDGE('',*,*,#22007,.T.);
#30441=ORIENTED_EDGE('',*,*,#20743,.F.);
#30442=ORIENTED_EDGE('',*,*,#20086,.T.);
#30443=ORIENTED_EDGE('',*,*,#19704,.F.);
#30444=ORIENTED_EDGE('',*,*,#22008,.T.);
#30445=ORIENTED_EDGE('',*,*,#19709,.T.);
#30446=ORIENTED_EDGE('',*,*,#20085,.T.);
#30447=ORIENTED_EDGE('',*,*,#21822,.T.);
#30448=ORIENTED_EDGE('',*,*,#19689,.F.);
#30449=ORIENTED_EDGE('',*,*,#20265,.T.);
#30450=ORIENTED_EDGE('',*,*,#20736,.F.);
#30451=ORIENTED_EDGE('',*,*,#21805,.T.);
#30452=ORIENTED_EDGE('',*,*,#20571,.F.);
#30453=ORIENTED_EDGE('',*,*,#20261,.T.);
#30454=ORIENTED_EDGE('',*,*,#20725,.F.);
#30455=ORIENTED_EDGE('',*,*,#20791,.F.);
#30456=ORIENTED_EDGE('',*,*,#22009,.T.);
#30457=ORIENTED_EDGE('',*,*,#22010,.T.);
#30458=ORIENTED_EDGE('',*,*,#21799,.T.);
#30459=ORIENTED_EDGE('',*,*,#20728,.T.);
#30460=ORIENTED_EDGE('',*,*,#22011,.T.);
#30461=ORIENTED_EDGE('',*,*,#20704,.F.);
#30462=ORIENTED_EDGE('',*,*,#19722,.T.);
#30463=ORIENTED_EDGE('',*,*,#22011,.F.);
#30464=ORIENTED_EDGE('',*,*,#20727,.T.);
#30465=ORIENTED_EDGE('',*,*,#22012,.F.);
#30466=ORIENTED_EDGE('',*,*,#20795,.T.);
#30467=ORIENTED_EDGE('',*,*,#20796,.T.);
#30468=ORIENTED_EDGE('',*,*,#22012,.T.);
#30469=ORIENTED_EDGE('',*,*,#20592,.F.);
#30470=ORIENTED_EDGE('',*,*,#20257,.T.);
#30471=ORIENTED_EDGE('',*,*,#21801,.T.);
#30472=ORIENTED_EDGE('',*,*,#22013,.T.);
#30473=ORIENTED_EDGE('',*,*,#20797,.T.);
#30474=ORIENTED_EDGE('',*,*,#20255,.T.);
#30475=ORIENTED_EDGE('',*,*,#21798,.T.);
#30476=ORIENTED_EDGE('',*,*,#21802,.T.);
#30477=ORIENTED_EDGE('',*,*,#20253,.T.);
#30478=ORIENTED_EDGE('',*,*,#20864,.F.);
#30479=ORIENTED_EDGE('',*,*,#21788,.T.);
#30480=ORIENTED_EDGE('',*,*,#20839,.F.);
#30481=ORIENTED_EDGE('',*,*,#20249,.T.);
#30482=ORIENTED_EDGE('',*,*,#20832,.F.);
#30483=ORIENTED_EDGE('',*,*,#20881,.F.);
#30484=ORIENTED_EDGE('',*,*,#22014,.T.);
#30485=ORIENTED_EDGE('',*,*,#22015,.T.);
#30486=ORIENTED_EDGE('',*,*,#21782,.T.);
#30487=ORIENTED_EDGE('',*,*,#20835,.T.);
#30488=ORIENTED_EDGE('',*,*,#22016,.T.);
#30489=ORIENTED_EDGE('',*,*,#20811,.F.);
#30490=ORIENTED_EDGE('',*,*,#19734,.T.);
#30491=ORIENTED_EDGE('',*,*,#22016,.F.);
#30492=ORIENTED_EDGE('',*,*,#20834,.T.);
#30493=ORIENTED_EDGE('',*,*,#22017,.F.);
#30494=ORIENTED_EDGE('',*,*,#20885,.T.);
#30495=ORIENTED_EDGE('',*,*,#20886,.T.);
#30496=ORIENTED_EDGE('',*,*,#22017,.T.);
#30497=ORIENTED_EDGE('',*,*,#20662,.F.);
#30498=ORIENTED_EDGE('',*,*,#20245,.T.);
#30499=ORIENTED_EDGE('',*,*,#21784,.T.);
#30500=ORIENTED_EDGE('',*,*,#22018,.T.);
#30501=ORIENTED_EDGE('',*,*,#20887,.T.);
#30502=ORIENTED_EDGE('',*,*,#20243,.T.);
#30503=ORIENTED_EDGE('',*,*,#21781,.T.);
#30504=ORIENTED_EDGE('',*,*,#21785,.T.);
#30505=ORIENTED_EDGE('',*,*,#20241,.T.);
#30506=ORIENTED_EDGE('',*,*,#20804,.F.);
#30507=ORIENTED_EDGE('',*,*,#21777,.T.);
#30508=ORIENTED_EDGE('',*,*,#20683,.F.);
#30509=ORIENTED_EDGE('',*,*,#20237,.T.);
#30510=ORIENTED_EDGE('',*,*,#20980,.F.);
#30511=ORIENTED_EDGE('',*,*,#20991,.F.);
#30512=ORIENTED_EDGE('',*,*,#22019,.T.);
#30513=ORIENTED_EDGE('',*,*,#22020,.T.);
#30514=ORIENTED_EDGE('',*,*,#21765,.T.);
#30515=ORIENTED_EDGE('',*,*,#20983,.T.);
#30516=ORIENTED_EDGE('',*,*,#22021,.T.);
#30517=ORIENTED_EDGE('',*,*,#20938,.F.);
#30518=ORIENTED_EDGE('',*,*,#19746,.T.);
#30519=ORIENTED_EDGE('',*,*,#22021,.F.);
#30520=ORIENTED_EDGE('',*,*,#20982,.T.);
#30521=ORIENTED_EDGE('',*,*,#22022,.F.);
#30522=ORIENTED_EDGE('',*,*,#20995,.T.);
#30523=ORIENTED_EDGE('',*,*,#20996,.T.);
#30524=ORIENTED_EDGE('',*,*,#22022,.T.);
#30525=ORIENTED_EDGE('',*,*,#20955,.F.);
#30526=ORIENTED_EDGE('',*,*,#20233,.T.);
#30527=ORIENTED_EDGE('',*,*,#21767,.T.);
#30528=ORIENTED_EDGE('',*,*,#22023,.T.);
#30529=ORIENTED_EDGE('',*,*,#20997,.T.);
#30530=ORIENTED_EDGE('',*,*,#20231,.T.);
#30531=ORIENTED_EDGE('',*,*,#21764,.T.);
#30532=ORIENTED_EDGE('',*,*,#21768,.T.);
#30533=ORIENTED_EDGE('',*,*,#20229,.T.);
#30534=ORIENTED_EDGE('',*,*,#21085,.F.);
#30535=ORIENTED_EDGE('',*,*,#20277,.F.);
#30536=ORIENTED_EDGE('',*,*,#21758,.F.);
#30537=ORIENTED_EDGE('',*,*,#21756,.F.);
#30538=ORIENTED_EDGE('',*,*,#19753,.F.);
#30539=ORIENTED_EDGE('',*,*,#21760,.F.);
#30540=ORIENTED_EDGE('',*,*,#22024,.F.);
#30541=ORIENTED_EDGE('',*,*,#20286,.F.);
#30542=ORIENTED_EDGE('',*,*,#20281,.F.);
#30543=ORIENTED_EDGE('',*,*,#21759,.T.);
#30544=ORIENTED_EDGE('',*,*,#20276,.F.);
#30545=ORIENTED_EDGE('',*,*,#20225,.T.);
#30546=ORIENTED_EDGE('',*,*,#21098,.F.);
#30547=ORIENTED_EDGE('',*,*,#19937,.F.);
#30548=ORIENTED_EDGE('',*,*,#21754,.T.);
#30549=ORIENTED_EDGE('',*,*,#21747,.F.);
#30550=ORIENTED_EDGE('',*,*,#19951,.T.);
#30551=ORIENTED_EDGE('',*,*,#21101,.T.);
#30552=ORIENTED_EDGE('',*,*,#22025,.T.);
#30553=ORIENTED_EDGE('',*,*,#19914,.F.);
#30554=ORIENTED_EDGE('',*,*,#19758,.T.);
#30555=ORIENTED_EDGE('',*,*,#22025,.F.);
#30556=ORIENTED_EDGE('',*,*,#21100,.T.);
#30557=ORIENTED_EDGE('',*,*,#22026,.F.);
#30558=ORIENTED_EDGE('',*,*,#19940,.T.);
#30559=ORIENTED_EDGE('',*,*,#19941,.T.);
#30560=ORIENTED_EDGE('',*,*,#22026,.T.);
#30561=ORIENTED_EDGE('',*,*,#21060,.F.);
#30562=ORIENTED_EDGE('',*,*,#20221,.T.);
#30563=ORIENTED_EDGE('',*,*,#19938,.F.);
#30564=ORIENTED_EDGE('',*,*,#22027,.T.);
#30565=ORIENTED_EDGE('',*,*,#19943,.T.);
#30566=ORIENTED_EDGE('',*,*,#20220,.T.);
#30567=ORIENTED_EDGE('',*,*,#21753,.T.);
#30568=ORIENTED_EDGE('',*,*,#19923,.F.);
#30569=ORIENTED_EDGE('',*,*,#20219,.T.);
#30570=ORIENTED_EDGE('',*,*,#21053,.F.);
#30571=ORIENTED_EDGE('',*,*,#21736,.T.);
#30572=ORIENTED_EDGE('',*,*,#20896,.F.);
#30573=ORIENTED_EDGE('',*,*,#20215,.T.);
#30574=ORIENTED_EDGE('',*,*,#21042,.F.);
#30575=ORIENTED_EDGE('',*,*,#21121,.F.);
#30576=ORIENTED_EDGE('',*,*,#22028,.T.);
#30577=ORIENTED_EDGE('',*,*,#22029,.T.);
#30578=ORIENTED_EDGE('',*,*,#21730,.T.);
#30579=ORIENTED_EDGE('',*,*,#21045,.T.);
#30580=ORIENTED_EDGE('',*,*,#22030,.T.);
#30581=ORIENTED_EDGE('',*,*,#21021,.F.);
#30582=ORIENTED_EDGE('',*,*,#19770,.T.);
#30583=ORIENTED_EDGE('',*,*,#22030,.F.);
#30584=ORIENTED_EDGE('',*,*,#21044,.T.);
#30585=ORIENTED_EDGE('',*,*,#22031,.F.);
#30586=ORIENTED_EDGE('',*,*,#21125,.T.);
#30587=ORIENTED_EDGE('',*,*,#21126,.T.);
#30588=ORIENTED_EDGE('',*,*,#22031,.T.);
#30589=ORIENTED_EDGE('',*,*,#20917,.F.);
#30590=ORIENTED_EDGE('',*,*,#20211,.T.);
#30591=ORIENTED_EDGE('',*,*,#21732,.T.);
#30592=ORIENTED_EDGE('',*,*,#22032,.T.);
#30593=ORIENTED_EDGE('',*,*,#21127,.T.);
#30594=ORIENTED_EDGE('',*,*,#20209,.T.);
#30595=ORIENTED_EDGE('',*,*,#21729,.T.);
#30596=ORIENTED_EDGE('',*,*,#21733,.T.);
#30597=ORIENTED_EDGE('',*,*,#20207,.T.);
#30598=ORIENTED_EDGE('',*,*,#21134,.F.);
#30599=ORIENTED_EDGE('',*,*,#21719,.T.);
#30600=ORIENTED_EDGE('',*,*,#21000,.F.);
#30601=ORIENTED_EDGE('',*,*,#20203,.T.);
#30602=ORIENTED_EDGE('',*,*,#21166,.F.);
#30603=ORIENTED_EDGE('',*,*,#20074,.F.);
#30604=ORIENTED_EDGE('',*,*,#22033,.F.);
#30605=ORIENTED_EDGE('',*,*,#22034,.F.);
#30606=ORIENTED_EDGE('',*,*,#19781,.F.);
#30607=ORIENTED_EDGE('',*,*,#21716,.F.);
#30608=ORIENTED_EDGE('',*,*,#22035,.F.);
#30609=ORIENTED_EDGE('',*,*,#20083,.F.);
#30610=ORIENTED_EDGE('',*,*,#20078,.F.);
#30611=ORIENTED_EDGE('',*,*,#21291,.F.);
#30612=ORIENTED_EDGE('',*,*,#22036,.T.);
#30613=ORIENTED_EDGE('',*,*,#22037,.T.);
#30614=ORIENTED_EDGE('',*,*,#21712,.T.);
#30615=ORIENTED_EDGE('',*,*,#22034,.T.);
#30616=ORIENTED_EDGE('',*,*,#22038,.T.);
#30617=ORIENTED_EDGE('',*,*,#21270,.F.);
#30618=ORIENTED_EDGE('',*,*,#19782,.T.);
#30619=ORIENTED_EDGE('',*,*,#22038,.F.);
#30620=ORIENTED_EDGE('',*,*,#22033,.T.);
#30621=ORIENTED_EDGE('',*,*,#22039,.F.);
#30622=ORIENTED_EDGE('',*,*,#21295,.T.);
#30623=ORIENTED_EDGE('',*,*,#21296,.T.);
#30624=ORIENTED_EDGE('',*,*,#22039,.T.);
#30625=ORIENTED_EDGE('',*,*,#20073,.F.);
#30626=ORIENTED_EDGE('',*,*,#20200,.T.);
#30627=ORIENTED_EDGE('',*,*,#21714,.T.);
#30628=ORIENTED_EDGE('',*,*,#22040,.T.);
#30629=ORIENTED_EDGE('',*,*,#21297,.T.);
#30630=ORIENTED_EDGE('',*,*,#20198,.T.);
#30631=ORIENTED_EDGE('',*,*,#21711,.T.);
#30632=ORIENTED_EDGE('',*,*,#21715,.T.);
#30633=ORIENTED_EDGE('',*,*,#20196,.T.);
#30634=ORIENTED_EDGE('',*,*,#21268,.F.);
#30635=ORIENTED_EDGE('',*,*,#20034,.F.);
#30636=ORIENTED_EDGE('',*,*,#21705,.F.);
#30637=ORIENTED_EDGE('',*,*,#21703,.F.);
#30638=ORIENTED_EDGE('',*,*,#19789,.F.);
#30639=ORIENTED_EDGE('',*,*,#21708,.F.);
#30640=ORIENTED_EDGE('',*,*,#22041,.F.);
#30641=ORIENTED_EDGE('',*,*,#20046,.F.);
#30642=ORIENTED_EDGE('',*,*,#20038,.F.);
#30643=ORIENTED_EDGE('',*,*,#21706,.T.);
#30644=ORIENTED_EDGE('',*,*,#20033,.F.);
#30645=ORIENTED_EDGE('',*,*,#20194,.T.);
#30646=ORIENTED_EDGE('',*,*,#21304,.F.);
#30647=ORIENTED_EDGE('',*,*,#21315,.F.);
#30648=ORIENTED_EDGE('',*,*,#22042,.T.);
#30649=ORIENTED_EDGE('',*,*,#22043,.T.);
#30650=ORIENTED_EDGE('',*,*,#21692,.T.);
#30651=ORIENTED_EDGE('',*,*,#21307,.T.);
#30652=ORIENTED_EDGE('',*,*,#22044,.T.);
#30653=ORIENTED_EDGE('',*,*,#21228,.F.);
#30654=ORIENTED_EDGE('',*,*,#19794,.T.);
#30655=ORIENTED_EDGE('',*,*,#22044,.F.);
#30656=ORIENTED_EDGE('',*,*,#21306,.T.);
#30657=ORIENTED_EDGE('',*,*,#22045,.F.);
#30658=ORIENTED_EDGE('',*,*,#21319,.T.);
#30659=ORIENTED_EDGE('',*,*,#21320,.T.);
#30660=ORIENTED_EDGE('',*,*,#22045,.T.);
#30661=ORIENTED_EDGE('',*,*,#21245,.F.);
#30662=ORIENTED_EDGE('',*,*,#20190,.T.);
#30663=ORIENTED_EDGE('',*,*,#21694,.T.);
#30664=ORIENTED_EDGE('',*,*,#22046,.T.);
#30665=ORIENTED_EDGE('',*,*,#21321,.T.);
#30666=ORIENTED_EDGE('',*,*,#20188,.T.);
#30667=ORIENTED_EDGE('',*,*,#21691,.T.);
#30668=ORIENTED_EDGE('',*,*,#21695,.T.);
#30669=ORIENTED_EDGE('',*,*,#20186,.T.);
#30670=ORIENTED_EDGE('',*,*,#21221,.F.);
#30671=ORIENTED_EDGE('',*,*,#21687,.T.);
#30672=ORIENTED_EDGE('',*,*,#21141,.F.);
#30673=ORIENTED_EDGE('',*,*,#20182,.T.);
#30674=ORIENTED_EDGE('',*,*,#21377,.F.);
#30675=ORIENTED_EDGE('',*,*,#19976,.F.);
#30676=ORIENTED_EDGE('',*,*,#21684,.T.);
#30677=ORIENTED_EDGE('',*,*,#21677,.F.);
#30678=ORIENTED_EDGE('',*,*,#19990,.T.);
#30679=ORIENTED_EDGE('',*,*,#21380,.T.);
#30680=ORIENTED_EDGE('',*,*,#22047,.T.);
#30681=ORIENTED_EDGE('',*,*,#19953,.F.);
#30682=ORIENTED_EDGE('',*,*,#19806,.T.);
#30683=ORIENTED_EDGE('',*,*,#22047,.F.);
#30684=ORIENTED_EDGE('',*,*,#21379,.T.);
#30685=ORIENTED_EDGE('',*,*,#22048,.F.);
#30686=ORIENTED_EDGE('',*,*,#19979,.T.);
#30687=ORIENTED_EDGE('',*,*,#19980,.T.);
#30688=ORIENTED_EDGE('',*,*,#22048,.T.);
#30689=ORIENTED_EDGE('',*,*,#21352,.F.);
#30690=ORIENTED_EDGE('',*,*,#20178,.T.);
#30691=ORIENTED_EDGE('',*,*,#19977,.F.);
#30692=ORIENTED_EDGE('',*,*,#22049,.T.);
#30693=ORIENTED_EDGE('',*,*,#19982,.T.);
#30694=ORIENTED_EDGE('',*,*,#20177,.T.);
#30695=ORIENTED_EDGE('',*,*,#21683,.T.);
#30696=ORIENTED_EDGE('',*,*,#19962,.F.);
#30697=ORIENTED_EDGE('',*,*,#20176,.T.);
#30698=ORIENTED_EDGE('',*,*,#21345,.F.);
#30699=ORIENTED_EDGE('',*,*,#21666,.T.);
#30700=ORIENTED_EDGE('',*,*,#21175,.F.);
#30701=ORIENTED_EDGE('',*,*,#20172,.T.);
#30702=ORIENTED_EDGE('',*,*,#21334,.F.);
#30703=ORIENTED_EDGE('',*,*,#21497,.F.);
#30704=ORIENTED_EDGE('',*,*,#22050,.T.);
#30705=ORIENTED_EDGE('',*,*,#22051,.T.);
#30706=ORIENTED_EDGE('',*,*,#21660,.T.);
#30707=ORIENTED_EDGE('',*,*,#21337,.T.);
#30708=ORIENTED_EDGE('',*,*,#22052,.T.);
#30709=ORIENTED_EDGE('',*,*,#21476,.F.);
#30710=ORIENTED_EDGE('',*,*,#19818,.T.);
#30711=ORIENTED_EDGE('',*,*,#22052,.F.);
#30712=ORIENTED_EDGE('',*,*,#21336,.T.);
#30713=ORIENTED_EDGE('',*,*,#22053,.F.);
#30714=ORIENTED_EDGE('',*,*,#21501,.T.);
#30715=ORIENTED_EDGE('',*,*,#21502,.T.);
#30716=ORIENTED_EDGE('',*,*,#22053,.T.);
#30717=ORIENTED_EDGE('',*,*,#21196,.F.);
#30718=ORIENTED_EDGE('',*,*,#20168,.T.);
#30719=ORIENTED_EDGE('',*,*,#21662,.T.);
#30720=ORIENTED_EDGE('',*,*,#22054,.T.);
#30721=ORIENTED_EDGE('',*,*,#21503,.T.);
#30722=ORIENTED_EDGE('',*,*,#20166,.T.);
#30723=ORIENTED_EDGE('',*,*,#21659,.T.);
#30724=ORIENTED_EDGE('',*,*,#21663,.T.);
#30725=ORIENTED_EDGE('',*,*,#20164,.T.);
#30726=ORIENTED_EDGE('',*,*,#21510,.F.);
#30727=ORIENTED_EDGE('',*,*,#21649,.T.);
#30728=ORIENTED_EDGE('',*,*,#21455,.F.);
#30729=ORIENTED_EDGE('',*,*,#20160,.T.);
#30730=ORIENTED_EDGE('',*,*,#21586,.F.);
#30731=ORIENTED_EDGE('',*,*,#19994,.F.);
#30732=ORIENTED_EDGE('',*,*,#22055,.F.);
#30733=ORIENTED_EDGE('',*,*,#22056,.F.);
#30734=ORIENTED_EDGE('',*,*,#19829,.F.);
#30735=ORIENTED_EDGE('',*,*,#21647,.F.);
#30736=ORIENTED_EDGE('',*,*,#22057,.F.);
#30737=ORIENTED_EDGE('',*,*,#20006,.F.);
#30738=ORIENTED_EDGE('',*,*,#19998,.F.);
#30739=ORIENTED_EDGE('',*,*,#21592,.F.);
#30740=ORIENTED_EDGE('',*,*,#22058,.T.);
#30741=ORIENTED_EDGE('',*,*,#22059,.T.);
#30742=ORIENTED_EDGE('',*,*,#21642,.T.);
#30743=ORIENTED_EDGE('',*,*,#22056,.T.);
#30744=ORIENTED_EDGE('',*,*,#22060,.T.);
#30745=ORIENTED_EDGE('',*,*,#21567,.F.);
#30746=ORIENTED_EDGE('',*,*,#19830,.T.);
#30747=ORIENTED_EDGE('',*,*,#22060,.F.);
#30748=ORIENTED_EDGE('',*,*,#22055,.T.);
#30749=ORIENTED_EDGE('',*,*,#22061,.F.);
#30750=ORIENTED_EDGE('',*,*,#21596,.T.);
#30751=ORIENTED_EDGE('',*,*,#21597,.T.);
#30752=ORIENTED_EDGE('',*,*,#22061,.T.);
#30753=ORIENTED_EDGE('',*,*,#19993,.F.);
#30754=ORIENTED_EDGE('',*,*,#20158,.T.);
#30755=ORIENTED_EDGE('',*,*,#21644,.T.);
#30756=ORIENTED_EDGE('',*,*,#22062,.T.);
#30757=ORIENTED_EDGE('',*,*,#21598,.T.);
#30758=ORIENTED_EDGE('',*,*,#20156,.T.);
#30759=ORIENTED_EDGE('',*,*,#21641,.T.);
#30760=ORIENTED_EDGE('',*,*,#21645,.T.);
#30761=ORIENTED_EDGE('',*,*,#20154,.T.);
#30762=ORIENTED_EDGE('',*,*,#21560,.F.);
#30763=ORIENTED_EDGE('',*,*,#21637,.T.);
#30764=ORIENTED_EDGE('',*,*,#21396,.F.);
#30765=ORIENTED_EDGE('',*,*,#20150,.T.);
#30766=ORIENTED_EDGE('',*,*,#21521,.F.);
#30767=ORIENTED_EDGE('',*,*,#21532,.F.);
#30768=ORIENTED_EDGE('',*,*,#22063,.T.);
#30769=ORIENTED_EDGE('',*,*,#22064,.T.);
#30770=ORIENTED_EDGE('',*,*,#21625,.T.);
#30771=ORIENTED_EDGE('',*,*,#21524,.T.);
#30772=ORIENTED_EDGE('',*,*,#22065,.T.);
#30773=ORIENTED_EDGE('',*,*,#21417,.F.);
#30774=ORIENTED_EDGE('',*,*,#19842,.T.);
#30775=ORIENTED_EDGE('',*,*,#22065,.F.);
#30776=ORIENTED_EDGE('',*,*,#21523,.T.);
#30777=ORIENTED_EDGE('',*,*,#22066,.F.);
#30778=ORIENTED_EDGE('',*,*,#21536,.T.);
#30779=ORIENTED_EDGE('',*,*,#21537,.T.);
#30780=ORIENTED_EDGE('',*,*,#22066,.T.);
#30781=ORIENTED_EDGE('',*,*,#21434,.F.);
#30782=ORIENTED_EDGE('',*,*,#20146,.T.);
#30783=ORIENTED_EDGE('',*,*,#21627,.T.);
#30784=ORIENTED_EDGE('',*,*,#22067,.T.);
#30785=ORIENTED_EDGE('',*,*,#21538,.T.);
#30786=ORIENTED_EDGE('',*,*,#20144,.T.);
#30787=ORIENTED_EDGE('',*,*,#21553,.T.);
#30788=ORIENTED_EDGE('',*,*,#21624,.T.);
#30789=ORIENTED_EDGE('',*,*,#21628,.T.);
#30790=ORIENTED_EDGE('',*,*,#20142,.T.);
#30791=ORIENTED_EDGE('',*,*,#22068,.T.);
#30792=ORIENTED_EDGE('',*,*,#21545,.T.);
#30793=ORIENTED_EDGE('',*,*,#21554,.T.);
#30794=ORIENTED_EDGE('',*,*,#20140,.T.);
#30795=ORIENTED_EDGE('',*,*,#21620,.F.);
#30796=ORIENTED_EDGE('',*,*,#22069,.F.);
#30797=ORIENTED_EDGE('',*,*,#22070,.F.);
#30798=ORIENTED_EDGE('',*,*,#21546,.F.);
#30799=ORIENTED_EDGE('',*,*,#22068,.F.);
#30800=ORIENTED_EDGE('',*,*,#20139,.F.);
#30801=ORIENTED_EDGE('',*,*,#22071,.F.);
#30802=ORIENTED_EDGE('',*,*,#22072,.F.);
#30803=ORIENTED_EDGE('',*,*,#22073,.F.);
#30804=ORIENTED_EDGE('',*,*,#19849,.F.);
#30805=ORIENTED_EDGE('',*,*,#22073,.T.);
#30806=ORIENTED_EDGE('',*,*,#22074,.T.);
#30807=ORIENTED_EDGE('',*,*,#21610,.F.);
#30808=ORIENTED_EDGE('',*,*,#19850,.T.);
#30809=ORIENTED_EDGE('',*,*,#22074,.F.);
#30810=ORIENTED_EDGE('',*,*,#22072,.T.);
#30811=ORIENTED_EDGE('',*,*,#22075,.F.);
#30812=ORIENTED_EDGE('',*,*,#21616,.T.);
#30813=ORIENTED_EDGE('',*,*,#22075,.T.);
#30814=ORIENTED_EDGE('',*,*,#22071,.T.);
#30815=ORIENTED_EDGE('',*,*,#20138,.T.);
#30816=ORIENTED_EDGE('',*,*,#21955,.F.);
#30817=ORIENTED_EDGE('',*,*,#22076,.T.);
#30818=ORIENTED_EDGE('',*,*,#22077,.T.);
#30819=ORIENTED_EDGE('',*,*,#21547,.T.);
#30820=ORIENTED_EDGE('',*,*,#22070,.T.);
#30821=ORIENTED_EDGE('',*,*,#21542,.F.);
#30822=ORIENTED_EDGE('',*,*,#22078,.T.);
#30823=ORIENTED_EDGE('',*,*,#22076,.F.);
#30824=ORIENTED_EDGE('',*,*,#22069,.T.);
#30825=ORIENTED_EDGE('',*,*,#21621,.F.);
#30826=ORIENTED_EDGE('',*,*,#21549,.T.);
#30827=ORIENTED_EDGE('',*,*,#21541,.F.);
#30828=ORIENTED_EDGE('',*,*,#21548,.T.);
#30829=ORIENTED_EDGE('',*,*,#22077,.F.);
#30830=ORIENTED_EDGE('',*,*,#22078,.F.);
#30831=ORIENTED_EDGE('',*,*,#21424,.F.);
#30832=ORIENTED_EDGE('',*,*,#21539,.T.);
#30833=ORIENTED_EDGE('',*,*,#22067,.F.);
#30834=ORIENTED_EDGE('',*,*,#21626,.T.);
#30835=ORIENTED_EDGE('',*,*,#22064,.F.);
#30836=ORIENTED_EDGE('',*,*,#22079,.F.);
#30837=ORIENTED_EDGE('',*,*,#21425,.F.);
#30838=ORIENTED_EDGE('',*,*,#22079,.T.);
#30839=ORIENTED_EDGE('',*,*,#22063,.F.);
#30840=ORIENTED_EDGE('',*,*,#21530,.F.);
#30841=ORIENTED_EDGE('',*,*,#21441,.F.);
#30842=ORIENTED_EDGE('',*,*,#21526,.T.);
#30843=ORIENTED_EDGE('',*,*,#21635,.F.);
#30844=ORIENTED_EDGE('',*,*,#21631,.T.);
#30845=ORIENTED_EDGE('',*,*,#21629,.F.);
#30846=ORIENTED_EDGE('',*,*,#21452,.T.);
#30847=ORIENTED_EDGE('',*,*,#21403,.F.);
#30848=ORIENTED_EDGE('',*,*,#21565,.T.);
#30849=ORIENTED_EDGE('',*,*,#21638,.F.);
#30850=ORIENTED_EDGE('',*,*,#21602,.T.);
#30851=ORIENTED_EDGE('',*,*,#21600,.F.);
#30852=ORIENTED_EDGE('',*,*,#21414,.T.);
#30853=ORIENTED_EDGE('',*,*,#21574,.F.);
#30854=ORIENTED_EDGE('',*,*,#21599,.T.);
#30855=ORIENTED_EDGE('',*,*,#22062,.F.);
#30856=ORIENTED_EDGE('',*,*,#21643,.T.);
#30857=ORIENTED_EDGE('',*,*,#22059,.F.);
#30858=ORIENTED_EDGE('',*,*,#22080,.F.);
#30859=ORIENTED_EDGE('',*,*,#21575,.F.);
#30860=ORIENTED_EDGE('',*,*,#22080,.T.);
#30861=ORIENTED_EDGE('',*,*,#22058,.F.);
#30862=ORIENTED_EDGE('',*,*,#21590,.F.);
#30863=ORIENTED_EDGE('',*,*,#20007,.F.);
#30864=ORIENTED_EDGE('',*,*,#22057,.T.);
#30865=ORIENTED_EDGE('',*,*,#21646,.F.);
#30866=ORIENTED_EDGE('',*,*,#20013,.F.);
#30867=ORIENTED_EDGE('',*,*,#20000,.F.);
#30868=ORIENTED_EDGE('',*,*,#21462,.F.);
#30869=ORIENTED_EDGE('',*,*,#21515,.T.);
#30870=ORIENTED_EDGE('',*,*,#21656,.F.);
#30871=ORIENTED_EDGE('',*,*,#21652,.T.);
#30872=ORIENTED_EDGE('',*,*,#21650,.F.);
#30873=ORIENTED_EDGE('',*,*,#21473,.T.);
#30874=ORIENTED_EDGE('',*,*,#21483,.F.);
#30875=ORIENTED_EDGE('',*,*,#21504,.T.);
#30876=ORIENTED_EDGE('',*,*,#22054,.F.);
#30877=ORIENTED_EDGE('',*,*,#21661,.T.);
#30878=ORIENTED_EDGE('',*,*,#22051,.F.);
#30879=ORIENTED_EDGE('',*,*,#22081,.F.);
#30880=ORIENTED_EDGE('',*,*,#21484,.F.);
#30881=ORIENTED_EDGE('',*,*,#22081,.T.);
#30882=ORIENTED_EDGE('',*,*,#22050,.F.);
#30883=ORIENTED_EDGE('',*,*,#21495,.F.);
#30884=ORIENTED_EDGE('',*,*,#21203,.F.);
#30885=ORIENTED_EDGE('',*,*,#21339,.T.);
#30886=ORIENTED_EDGE('',*,*,#21664,.F.);
#30887=ORIENTED_EDGE('',*,*,#21391,.T.);
#30888=ORIENTED_EDGE('',*,*,#21389,.F.);
#30889=ORIENTED_EDGE('',*,*,#21214,.T.);
#30890=ORIENTED_EDGE('',*,*,#21182,.F.);
#30891=ORIENTED_EDGE('',*,*,#21350,.T.);
#30892=ORIENTED_EDGE('',*,*,#21667,.F.);
#30893=ORIENTED_EDGE('',*,*,#21385,.T.);
#30894=ORIENTED_EDGE('',*,*,#21383,.F.);
#30895=ORIENTED_EDGE('',*,*,#21193,.T.);
#30896=ORIENTED_EDGE('',*,*,#19971,.F.);
#30897=ORIENTED_EDGE('',*,*,#19983,.T.);
#30898=ORIENTED_EDGE('',*,*,#22049,.F.);
#30899=ORIENTED_EDGE('',*,*,#19973,.F.);
#30900=ORIENTED_EDGE('',*,*,#19964,.F.);
#30901=ORIENTED_EDGE('',*,*,#21359,.F.);
#30902=ORIENTED_EDGE('',*,*,#21382,.T.);
#30903=ORIENTED_EDGE('',*,*,#21685,.F.);
#30904=ORIENTED_EDGE('',*,*,#21670,.T.);
#30905=ORIENTED_EDGE('',*,*,#21668,.F.);
#30906=ORIENTED_EDGE('',*,*,#21370,.T.);
#30907=ORIENTED_EDGE('',*,*,#21148,.F.);
#30908=ORIENTED_EDGE('',*,*,#21226,.T.);
#30909=ORIENTED_EDGE('',*,*,#21688,.F.);
#30910=ORIENTED_EDGE('',*,*,#21325,.T.);
#30911=ORIENTED_EDGE('',*,*,#21323,.F.);
#30912=ORIENTED_EDGE('',*,*,#21159,.T.);
#30913=ORIENTED_EDGE('',*,*,#21235,.F.);
#30914=ORIENTED_EDGE('',*,*,#21322,.T.);
#30915=ORIENTED_EDGE('',*,*,#22046,.F.);
#30916=ORIENTED_EDGE('',*,*,#21693,.T.);
#30917=ORIENTED_EDGE('',*,*,#22043,.F.);
#30918=ORIENTED_EDGE('',*,*,#22082,.F.);
#30919=ORIENTED_EDGE('',*,*,#21236,.F.);
#30920=ORIENTED_EDGE('',*,*,#22082,.T.);
#30921=ORIENTED_EDGE('',*,*,#22042,.F.);
#30922=ORIENTED_EDGE('',*,*,#21313,.F.);
#30923=ORIENTED_EDGE('',*,*,#21252,.F.);
#30924=ORIENTED_EDGE('',*,*,#21309,.T.);
#30925=ORIENTED_EDGE('',*,*,#21702,.F.);
#30926=ORIENTED_EDGE('',*,*,#21698,.T.);
#30927=ORIENTED_EDGE('',*,*,#21696,.F.);
#30928=ORIENTED_EDGE('',*,*,#21263,.T.);
#30929=ORIENTED_EDGE('',*,*,#20047,.F.);
#30930=ORIENTED_EDGE('',*,*,#22041,.T.);
#30931=ORIENTED_EDGE('',*,*,#21707,.F.);
#30932=ORIENTED_EDGE('',*,*,#20053,.F.);
#30933=ORIENTED_EDGE('',*,*,#20040,.F.);
#30934=ORIENTED_EDGE('',*,*,#21277,.F.);
#30935=ORIENTED_EDGE('',*,*,#21298,.T.);
#30936=ORIENTED_EDGE('',*,*,#22040,.F.);
#30937=ORIENTED_EDGE('',*,*,#21713,.T.);
#30938=ORIENTED_EDGE('',*,*,#22037,.F.);
#30939=ORIENTED_EDGE('',*,*,#22083,.F.);
#30940=ORIENTED_EDGE('',*,*,#21278,.F.);
#30941=ORIENTED_EDGE('',*,*,#22083,.T.);
#30942=ORIENTED_EDGE('',*,*,#22036,.F.);
#30943=ORIENTED_EDGE('',*,*,#21289,.F.);
#30944=ORIENTED_EDGE('',*,*,#20080,.F.);
#30945=ORIENTED_EDGE('',*,*,#22035,.T.);
#30946=ORIENTED_EDGE('',*,*,#21717,.F.);
#30947=ORIENTED_EDGE('',*,*,#21170,.T.);
#30948=ORIENTED_EDGE('',*,*,#21168,.F.);
#30949=ORIENTED_EDGE('',*,*,#20273,.T.);
#30950=ORIENTED_EDGE('',*,*,#21007,.F.);
#30951=ORIENTED_EDGE('',*,*,#21139,.T.);
#30952=ORIENTED_EDGE('',*,*,#21726,.F.);
#30953=ORIENTED_EDGE('',*,*,#21722,.T.);
#30954=ORIENTED_EDGE('',*,*,#21720,.F.);
#30955=ORIENTED_EDGE('',*,*,#21018,.T.);
#30956=ORIENTED_EDGE('',*,*,#21028,.F.);
#30957=ORIENTED_EDGE('',*,*,#21128,.T.);
#30958=ORIENTED_EDGE('',*,*,#22032,.F.);
#30959=ORIENTED_EDGE('',*,*,#21731,.T.);
#30960=ORIENTED_EDGE('',*,*,#22029,.F.);
#30961=ORIENTED_EDGE('',*,*,#22084,.F.);
#30962=ORIENTED_EDGE('',*,*,#21029,.F.);
#30963=ORIENTED_EDGE('',*,*,#22084,.T.);
#30964=ORIENTED_EDGE('',*,*,#22028,.F.);
#30965=ORIENTED_EDGE('',*,*,#21119,.F.);
#30966=ORIENTED_EDGE('',*,*,#20924,.F.);
#30967=ORIENTED_EDGE('',*,*,#21047,.T.);
#30968=ORIENTED_EDGE('',*,*,#21734,.F.);
#30969=ORIENTED_EDGE('',*,*,#21112,.T.);
#30970=ORIENTED_EDGE('',*,*,#21110,.F.);
#30971=ORIENTED_EDGE('',*,*,#20935,.T.);
#30972=ORIENTED_EDGE('',*,*,#20903,.F.);
#30973=ORIENTED_EDGE('',*,*,#21058,.T.);
#30974=ORIENTED_EDGE('',*,*,#21737,.F.);
#30975=ORIENTED_EDGE('',*,*,#21106,.T.);
#30976=ORIENTED_EDGE('',*,*,#21104,.F.);
#30977=ORIENTED_EDGE('',*,*,#20914,.T.);
#30978=ORIENTED_EDGE('',*,*,#19932,.F.);
#30979=ORIENTED_EDGE('',*,*,#19944,.T.);
#30980=ORIENTED_EDGE('',*,*,#22027,.F.);
#30981=ORIENTED_EDGE('',*,*,#19934,.F.);
#30982=ORIENTED_EDGE('',*,*,#19925,.F.);
#30983=ORIENTED_EDGE('',*,*,#21067,.F.);
#30984=ORIENTED_EDGE('',*,*,#21103,.T.);
#30985=ORIENTED_EDGE('',*,*,#21755,.F.);
#30986=ORIENTED_EDGE('',*,*,#21740,.T.);
#30987=ORIENTED_EDGE('',*,*,#21738,.F.);
#30988=ORIENTED_EDGE('',*,*,#21078,.T.);
#30989=ORIENTED_EDGE('',*,*,#20283,.F.);
#30990=ORIENTED_EDGE('',*,*,#22024,.T.);
#30991=ORIENTED_EDGE('',*,*,#21761,.F.);
#30992=ORIENTED_EDGE('',*,*,#21089,.T.);
#30993=ORIENTED_EDGE('',*,*,#21087,.F.);
#30994=ORIENTED_EDGE('',*,*,#20294,.T.);
#30995=ORIENTED_EDGE('',*,*,#20945,.F.);
#30996=ORIENTED_EDGE('',*,*,#20998,.T.);
#30997=ORIENTED_EDGE('',*,*,#22023,.F.);
#30998=ORIENTED_EDGE('',*,*,#21766,.T.);
#30999=ORIENTED_EDGE('',*,*,#22020,.F.);
#31000=ORIENTED_EDGE('',*,*,#22085,.F.);
#31001=ORIENTED_EDGE('',*,*,#20946,.F.);
#31002=ORIENTED_EDGE('',*,*,#22085,.T.);
#31003=ORIENTED_EDGE('',*,*,#22019,.F.);
#31004=ORIENTED_EDGE('',*,*,#20989,.F.);
#31005=ORIENTED_EDGE('',*,*,#20962,.F.);
#31006=ORIENTED_EDGE('',*,*,#20985,.T.);
#31007=ORIENTED_EDGE('',*,*,#21775,.F.);
#31008=ORIENTED_EDGE('',*,*,#21771,.T.);
#31009=ORIENTED_EDGE('',*,*,#21769,.F.);
#31010=ORIENTED_EDGE('',*,*,#20973,.T.);
#31011=ORIENTED_EDGE('',*,*,#20690,.F.);
#31012=ORIENTED_EDGE('',*,*,#20809,.T.);
#31013=ORIENTED_EDGE('',*,*,#21778,.F.);
#31014=ORIENTED_EDGE('',*,*,#20891,.T.);
#31015=ORIENTED_EDGE('',*,*,#20889,.F.);
#31016=ORIENTED_EDGE('',*,*,#20701,.T.);
#31017=ORIENTED_EDGE('',*,*,#20818,.F.);
#31018=ORIENTED_EDGE('',*,*,#20888,.T.);
#31019=ORIENTED_EDGE('',*,*,#22018,.F.);
#31020=ORIENTED_EDGE('',*,*,#21783,.T.);
#31021=ORIENTED_EDGE('',*,*,#22015,.F.);
#31022=ORIENTED_EDGE('',*,*,#22086,.F.);
#31023=ORIENTED_EDGE('',*,*,#20819,.F.);
#31024=ORIENTED_EDGE('',*,*,#22086,.T.);
#31025=ORIENTED_EDGE('',*,*,#22014,.F.);
#31026=ORIENTED_EDGE('',*,*,#20879,.F.);
#31027=ORIENTED_EDGE('',*,*,#20669,.F.);
#31028=ORIENTED_EDGE('',*,*,#20837,.T.);
#31029=ORIENTED_EDGE('',*,*,#21786,.F.);
#31030=ORIENTED_EDGE('',*,*,#20872,.T.);
#31031=ORIENTED_EDGE('',*,*,#20870,.F.);
#31032=ORIENTED_EDGE('',*,*,#20680,.T.);
#31033=ORIENTED_EDGE('',*,*,#20846,.F.);
#31034=ORIENTED_EDGE('',*,*,#20869,.T.);
#31035=ORIENTED_EDGE('',*,*,#21795,.F.);
#31036=ORIENTED_EDGE('',*,*,#21791,.T.);
#31037=ORIENTED_EDGE('',*,*,#21789,.F.);
#31038=ORIENTED_EDGE('',*,*,#20857,.T.);
#31039=ORIENTED_EDGE('',*,*,#20711,.F.);
#31040=ORIENTED_EDGE('',*,*,#20798,.T.);
#31041=ORIENTED_EDGE('',*,*,#22013,.F.);
#31042=ORIENTED_EDGE('',*,*,#21800,.T.);
#31043=ORIENTED_EDGE('',*,*,#22010,.F.);
#31044=ORIENTED_EDGE('',*,*,#22087,.F.);
#31045=ORIENTED_EDGE('',*,*,#20712,.F.);
#31046=ORIENTED_EDGE('',*,*,#22087,.T.);
#31047=ORIENTED_EDGE('',*,*,#22009,.F.);
#31048=ORIENTED_EDGE('',*,*,#20789,.F.);
#31049=ORIENTED_EDGE('',*,*,#20599,.F.);
#31050=ORIENTED_EDGE('',*,*,#20730,.T.);
#31051=ORIENTED_EDGE('',*,*,#21803,.F.);
#31052=ORIENTED_EDGE('',*,*,#20782,.T.);
#31053=ORIENTED_EDGE('',*,*,#20780,.F.);
#31054=ORIENTED_EDGE('',*,*,#20610,.T.);
#31055=ORIENTED_EDGE('',*,*,#20578,.F.);
#31056=ORIENTED_EDGE('',*,*,#20741,.T.);
#31057=ORIENTED_EDGE('',*,*,#21806,.F.);
#31058=ORIENTED_EDGE('',*,*,#20776,.T.);
#31059=ORIENTED_EDGE('',*,*,#20774,.F.);
#31060=ORIENTED_EDGE('',*,*,#20589,.T.);
#31061=ORIENTED_EDGE('',*,*,#19698,.F.);
#31062=ORIENTED_EDGE('',*,*,#19710,.T.);
#31063=ORIENTED_EDGE('',*,*,#22008,.F.);
#31064=ORIENTED_EDGE('',*,*,#19700,.F.);
#31065=ORIENTED_EDGE('',*,*,#19691,.F.);
#31066=ORIENTED_EDGE('',*,*,#20750,.F.);
#31067=ORIENTED_EDGE('',*,*,#20773,.T.);
#31068=ORIENTED_EDGE('',*,*,#21824,.F.);
#31069=ORIENTED_EDGE('',*,*,#21809,.T.);
#31070=ORIENTED_EDGE('',*,*,#21807,.F.);
#31071=ORIENTED_EDGE('',*,*,#20761,.T.);
#31072=ORIENTED_EDGE('',*,*,#20480,.F.);
#31073=ORIENTED_EDGE('',*,*,#20622,.T.);
#31074=ORIENTED_EDGE('',*,*,#21827,.F.);
#31075=ORIENTED_EDGE('',*,*,#20657,.T.);
#31076=ORIENTED_EDGE('',*,*,#20655,.F.);
#31077=ORIENTED_EDGE('',*,*,#20491,.T.);
#31078=ORIENTED_EDGE('',*,*,#20561,.F.);
#31079=ORIENTED_EDGE('',*,*,#21847,.T.);
#31080=ORIENTED_EDGE('',*,*,#22004,.F.);
#31081=ORIENTED_EDGE('',*,*,#21849,.T.);
#31082=ORIENTED_EDGE('',*,*,#22001,.F.);
#31083=ORIENTED_EDGE('',*,*,#22088,.F.);
#31084=ORIENTED_EDGE('',*,*,#20562,.F.);
#31085=ORIENTED_EDGE('',*,*,#22088,.T.);
#31086=ORIENTED_EDGE('',*,*,#22000,.F.);
#31087=ORIENTED_EDGE('',*,*,#21837,.F.);
#31088=ORIENTED_EDGE('',*,*,#20631,.F.);
#31089=ORIENTED_EDGE('',*,*,#20654,.T.);
#31090=ORIENTED_EDGE('',*,*,#21853,.F.);
#31091=ORIENTED_EDGE('',*,*,#21830,.T.);
#31092=ORIENTED_EDGE('',*,*,#21828,.F.);
#31093=ORIENTED_EDGE('',*,*,#20642,.T.);
#31094=ORIENTED_EDGE('',*,*,#20361,.F.);
#31095=ORIENTED_EDGE('',*,*,#20503,.T.);
#31096=ORIENTED_EDGE('',*,*,#21856,.F.);
#31097=ORIENTED_EDGE('',*,*,#20549,.T.);
#31098=ORIENTED_EDGE('',*,*,#20547,.F.);
#31099=ORIENTED_EDGE('',*,*,#20372,.T.);
#31100=ORIENTED_EDGE('',*,*,#20512,.F.);
#31101=ORIENTED_EDGE('',*,*,#20546,.T.);
#31102=ORIENTED_EDGE('',*,*,#21999,.F.);
#31103=ORIENTED_EDGE('',*,*,#21861,.T.);
#31104=ORIENTED_EDGE('',*,*,#21996,.F.);
#31105=ORIENTED_EDGE('',*,*,#22089,.F.);
#31106=ORIENTED_EDGE('',*,*,#20513,.F.);
#31107=ORIENTED_EDGE('',*,*,#22089,.T.);
#31108=ORIENTED_EDGE('',*,*,#21995,.F.);
#31109=ORIENTED_EDGE('',*,*,#20537,.F.);
#31110=ORIENTED_EDGE('',*,*,#20304,.F.);
#31111=ORIENTED_EDGE('',*,*,#21994,.T.);
#31112=ORIENTED_EDGE('',*,*,#21865,.F.);
#31113=ORIENTED_EDGE('',*,*,#20530,.T.);
#31114=ORIENTED_EDGE('',*,*,#20528,.F.);
#31115=ORIENTED_EDGE('',*,*,#20315,.T.);
#31116=ORIENTED_EDGE('',*,*,#20382,.F.);
#31117=ORIENTED_EDGE('',*,*,#20471,.T.);
#31118=ORIENTED_EDGE('',*,*,#21874,.F.);
#31119=ORIENTED_EDGE('',*,*,#21868,.T.);
#31120=ORIENTED_EDGE('',*,*,#21866,.F.);
#31121=ORIENTED_EDGE('',*,*,#20393,.T.);
#31122=ORIENTED_EDGE('',*,*,#20403,.F.);
#31123=ORIENTED_EDGE('',*,*,#20460,.T.);
#31124=ORIENTED_EDGE('',*,*,#21991,.F.);
#31125=ORIENTED_EDGE('',*,*,#21879,.T.);
#31126=ORIENTED_EDGE('',*,*,#21988,.F.);
#31127=ORIENTED_EDGE('',*,*,#22090,.F.);
#31128=ORIENTED_EDGE('',*,*,#20404,.F.);
#31129=ORIENTED_EDGE('',*,*,#22090,.T.);
#31130=ORIENTED_EDGE('',*,*,#21987,.F.);
#31131=ORIENTED_EDGE('',*,*,#20451,.F.);
#31132=ORIENTED_EDGE('',*,*,#20322,.F.);
#31133=ORIENTED_EDGE('',*,*,#21976,.F.);
#31134=ORIENTED_EDGE('',*,*,#21986,.F.);
#31135=ORIENTED_EDGE('',*,*,#20125,.F.);
#31136=ORIENTED_EDGE('',*,*,#20351,.F.);
#31137=ORIENTED_EDGE('',*,*,#20352,.F.);
#31138=ORIENTED_EDGE('',*,*,#20334,.F.);
#31139=ORIENTED_EDGE('',*,*,#20326,.F.);
#31140=ORIENTED_EDGE('',*,*,#20417,.F.);
#31141=ORIENTED_EDGE('',*,*,#21979,.F.);
#31142=ORIENTED_EDGE('',*,*,#21985,.F.);
#31143=ORIENTED_EDGE('',*,*,#20129,.F.);
#31144=ORIENTED_EDGE('',*,*,#20446,.F.);
#31145=ORIENTED_EDGE('',*,*,#20447,.F.);
#31146=ORIENTED_EDGE('',*,*,#20429,.F.);
#31147=ORIENTED_EDGE('',*,*,#20421,.F.);
#31148=ORIENTED_EDGE('',*,*,#21608,.F.);
#31149=ORIENTED_EDGE('',*,*,#21615,.F.);
#31150=ORIENTED_EDGE('',*,*,#21895,.F.);
#31151=ORIENTED_EDGE('',*,*,#21893,.F.);
#31152=ORIENTED_EDGE('',*,*,#22091,.T.);
#31153=ORIENTED_EDGE('',*,*,#21606,.F.);
#31154=ORIENTED_EDGE('',*,*,#22091,.F.);
#31155=ORIENTED_EDGE('',*,*,#21892,.F.);
#31156=ORIENTED_EDGE('',*,*,#21888,.F.);
#31157=ORIENTED_EDGE('',*,*,#21884,.F.);
#31158=ORIENTED_EDGE('',*,*,#21983,.F.);
#31159=ORIENTED_EDGE('',*,*,#21981,.F.);
#31160=ORIENTED_EDGE('',*,*,#19853,.F.);
#37325=CYLINDRICAL_SURFACE('',#40905,0.3);
#37326=CYLINDRICAL_SURFACE('',#40912,0.3);
#37327=CYLINDRICAL_SURFACE('',#40919,0.3);
#37328=CYLINDRICAL_SURFACE('',#40989,38.5);
#37329=CYLINDRICAL_SURFACE('',#40990,0.3);
#37330=CYLINDRICAL_SURFACE('',#40997,0.3);
#37331=CYLINDRICAL_SURFACE('',#41004,0.3);
#37332=CYLINDRICAL_SURFACE('',#41024,38.5);
#37333=CYLINDRICAL_SURFACE('',#41025,0.3);
#37334=CYLINDRICAL_SURFACE('',#41032,0.3);
#37335=CYLINDRICAL_SURFACE('',#41039,0.3);
#37336=CYLINDRICAL_SURFACE('',#41059,38.5);
#37337=CYLINDRICAL_SURFACE('',#41060,0.3);
#37338=CYLINDRICAL_SURFACE('',#41071,0.3);
#37339=CYLINDRICAL_SURFACE('',#41075,0.3);
#37340=CYLINDRICAL_SURFACE('',#41093,38.5);
#37341=CYLINDRICAL_SURFACE('',#41094,0.3);
#37342=CYLINDRICAL_SURFACE('',#41097,0.3);
#37343=CYLINDRICAL_SURFACE('',#41108,0.3);
#37344=CYLINDRICAL_SURFACE('',#41112,0.3);
#37345=CYLINDRICAL_SURFACE('',#41130,38.5);
#37346=CYLINDRICAL_SURFACE('',#41131,0.3);
#37347=CYLINDRICAL_SURFACE('',#41134,0.3);
#37348=CYLINDRICAL_SURFACE('',#41141,0.3);
#37349=CYLINDRICAL_SURFACE('',#41201,38.5);
#37350=CYLINDRICAL_SURFACE('',#41203,0.3);
#37351=CYLINDRICAL_SURFACE('',#41210,0.3);
#37352=CYLINDRICAL_SURFACE('',#41222,38.5);
#37353=CYLINDRICAL_SURFACE('',#41224,0.3);
#37354=CYLINDRICAL_SURFACE('',#41231,0.3);
#37355=CYLINDRICAL_SURFACE('',#41243,38.5);
#37356=CYLINDRICAL_SURFACE('',#41245,0.3);
#37357=CYLINDRICAL_SURFACE('',#41248,0.3);
#37358=CYLINDRICAL_SURFACE('',#41259,0.3);
#37359=CYLINDRICAL_SURFACE('',#41269,38.5);
#37360=CYLINDRICAL_SURFACE('',#41271,0.3);
#37361=CYLINDRICAL_SURFACE('',#41278,0.3);
#37362=CYLINDRICAL_SURFACE('',#41285,0.3);
#37363=CYLINDRICAL_SURFACE('',#41297,38.5);
#37364=CYLINDRICAL_SURFACE('',#41299,0.3);
#37365=CYLINDRICAL_SURFACE('',#41306,0.3);
#37366=CYLINDRICAL_SURFACE('',#41318,38.5);
#37367=CYLINDRICAL_SURFACE('',#41320,0.3);
#37368=CYLINDRICAL_SURFACE('',#41327,0.3);
#37369=CYLINDRICAL_SURFACE('',#41336,0.3);
#37370=CYLINDRICAL_SURFACE('',#41339,0.3);
#37371=CYLINDRICAL_SURFACE('',#41350,0.3);
#37372=CYLINDRICAL_SURFACE('',#41360,38.5);
#37373=CYLINDRICAL_SURFACE('',#41362,0.3);
#37374=CYLINDRICAL_SURFACE('',#41376,0.3);
#37375=CYLINDRICAL_SURFACE('',#41384,0.3);
#37376=CYLINDRICAL_SURFACE('',#41392,0.3);
#37377=CYLINDRICAL_SURFACE('',#41399,0.3);
#37378=CYLINDRICAL_SURFACE('',#41411,38.5);
#37379=CYLINDRICAL_SURFACE('',#41415,0.3);
#37380=CYLINDRICAL_SURFACE('',#41423,0.3);
#37381=CYLINDRICAL_SURFACE('',#41430,0.3);
#37382=CYLINDRICAL_SURFACE('',#41441,0.3);
#37383=CYLINDRICAL_SURFACE('',#41447,0.3);
#37384=CYLINDRICAL_SURFACE('',#41457,0.3);
#37385=CYLINDRICAL_SURFACE('',#41463,0.3);
#37386=CYLINDRICAL_SURFACE('',#41466,0.3);
#37387=CYLINDRICAL_SURFACE('',#41473,0.3);
#37388=CYLINDRICAL_SURFACE('',#41482,0.3);
#37389=CYLINDRICAL_SURFACE('',#41489,0.3);
#37390=CYLINDRICAL_SURFACE('',#41501,38.5);
#37391=CYLINDRICAL_SURFACE('',#41503,0.3);
#37392=CYLINDRICAL_SURFACE('',#41510,0.3);
#37393=CYLINDRICAL_SURFACE('',#41522,38.5);
#37394=CYLINDRICAL_SURFACE('',#41526,0.3);
#37395=CYLINDRICAL_SURFACE('',#41534,0.3);
#37396=CYLINDRICAL_SURFACE('',#41541,0.3);
#37397=CYLINDRICAL_SURFACE('',#41553,38.5);
#37398=CYLINDRICAL_SURFACE('',#41557,0.3);
#37399=CYLINDRICAL_SURFACE('',#41565,0.3);
#37400=CYLINDRICAL_SURFACE('',#41568,0.3);
#37401=CYLINDRICAL_SURFACE('',#41575,0.3);
#37402=CYLINDRICAL_SURFACE('',#41587,38.5);
#37403=CYLINDRICAL_SURFACE('',#41589,0.3);
#37404=CYLINDRICAL_SURFACE('',#41596,0.3);
#37405=CYLINDRICAL_SURFACE('',#41608,38.5);
#37406=CYLINDRICAL_SURFACE('',#41610,0.3);
#37407=CYLINDRICAL_SURFACE('',#41617,0.3);
#37408=CYLINDRICAL_SURFACE('',#41628,0.3);
#37409=CYLINDRICAL_SURFACE('',#41638,0.3);
#37410=CYLINDRICAL_SURFACE('',#41646,0.3);
#37411=CYLINDRICAL_SURFACE('',#41653,0.3);
#37412=CYLINDRICAL_SURFACE('',#41665,38.5);
#37413=CYLINDRICAL_SURFACE('',#41669,0.3);
#37414=CYLINDRICAL_SURFACE('',#41677,0.3);
#37415=CYLINDRICAL_SURFACE('',#41680,0.3);
#37416=CYLINDRICAL_SURFACE('',#41690,0.3);
#37417=CYLINDRICAL_SURFACE('',#41698,0.3);
#37418=CYLINDRICAL_SURFACE('',#41706,0.3);
#37419=CYLINDRICAL_SURFACE('',#41713,0.3);
#37420=CYLINDRICAL_SURFACE('',#41724,0.3);
#37421=CYLINDRICAL_SURFACE('',#41732,0.3);
#37422=CYLINDRICAL_SURFACE('',#41739,0.3);
#37423=CYLINDRICAL_SURFACE('',#41751,38.5);
#37424=CYLINDRICAL_SURFACE('',#41755,0.3);
#37425=CYLINDRICAL_SURFACE('',#41763,0.3);
#37426=CYLINDRICAL_SURFACE('',#41773,0.3);
#37427=CYLINDRICAL_SURFACE('',#41779,0.3);
#37428=CYLINDRICAL_SURFACE('',#41782,0.3);
#37429=CYLINDRICAL_SURFACE('',#41789,0.3);
#37430=CYLINDRICAL_SURFACE('',#41801,38.5);
#37431=CYLINDRICAL_SURFACE('',#41803,0.3);
#37432=CYLINDRICAL_SURFACE('',#41810,0.3);
#37433=CYLINDRICAL_SURFACE('',#41822,38.5);
#37434=CYLINDRICAL_SURFACE('',#41824,0.3);
#37435=CYLINDRICAL_SURFACE('',#41831,0.3);
#37436=CYLINDRICAL_SURFACE('',#41840,0.3);
#37437=CYLINDRICAL_SURFACE('',#41847,0.3);
#37438=CYLINDRICAL_SURFACE('',#41859,38.5);
#37439=CYLINDRICAL_SURFACE('',#41863,0.3);
#37440=CYLINDRICAL_SURFACE('',#41878,0.3);
#37441=CYLINDRICAL_SURFACE('',#41884,0.3);
#37442=CYLINDRICAL_SURFACE('',#41891,0.3);
#37443=CYLINDRICAL_SURFACE('',#41903,38.5);
#37444=CYLINDRICAL_SURFACE('',#41905,0.3);
#37445=CYLINDRICAL_SURFACE('',#41912,0.3);
#37446=CYLINDRICAL_SURFACE('',#41923,0.3);
#37447=CYLINDRICAL_SURFACE('',#41933,0.3);
#37448=CYLINDRICAL_SURFACE('',#41941,0.3);
#37449=CYLINDRICAL_SURFACE('',#41948,0.3);
#37450=CYLINDRICAL_SURFACE('',#41960,38.5);
#37451=CYLINDRICAL_SURFACE('',#41964,0.3);
#37452=CYLINDRICAL_SURFACE('',#41970,0.3);
#37453=CYLINDRICAL_SURFACE('',#41975,0.3);
#37454=CYLINDRICAL_SURFACE('',#41983,0.3);
#37455=CYLINDRICAL_SURFACE('',#41986,0.3);
#37456=CYLINDRICAL_SURFACE('',#41996,0.3);
#37457=CYLINDRICAL_SURFACE('',#42004,0.3);
#37458=CYLINDRICAL_SURFACE('',#42012,0.3);
#37459=CYLINDRICAL_SURFACE('',#42019,0.3);
#37460=CYLINDRICAL_SURFACE('',#42031,38.5);
#37461=CYLINDRICAL_SURFACE('',#42035,0.3);
#37462=CYLINDRICAL_SURFACE('',#42041,0.3);
#37463=CYLINDRICAL_SURFACE('',#42044,0.3);
#37464=CYLINDRICAL_SURFACE('',#42051,0.3);
#37465=CYLINDRICAL_SURFACE('',#42063,38.5);
#37466=CYLINDRICAL_SURFACE('',#42065,0.3);
#37467=CYLINDRICAL_SURFACE('',#42072,0.3);
#37468=CYLINDRICAL_SURFACE('',#42084,38.5);
#37469=CYLINDRICAL_SURFACE('',#42088,0.3);
#37470=CYLINDRICAL_SURFACE('',#42096,0.3);
#37471=CYLINDRICAL_SURFACE('',#42103,0.3);
#37472=CYLINDRICAL_SURFACE('',#42112,0.3);
#37473=CYLINDRICAL_SURFACE('',#42119,0.3);
#37474=CYLINDRICAL_SURFACE('',#42131,38.5);
#37475=CYLINDRICAL_SURFACE('',#42135,0.3);
#37476=CYLINDRICAL_SURFACE('',#42140,0.3);
#37477=CYLINDRICAL_SURFACE('',#42147,0.3);
#37478=CYLINDRICAL_SURFACE('',#42163,0.3);
#37479=CYLINDRICAL_SURFACE('',#42171,0.3);
#37480=CYLINDRICAL_SURFACE('',#42186,0.3);
#37481=CYLINDRICAL_SURFACE('',#42192,0.3);
#37482=CYLINDRICAL_SURFACE('',#42197,0.3);
#37483=CYLINDRICAL_SURFACE('',#42207,0.3);
#37484=CYLINDRICAL_SURFACE('',#42215,0.3);
#37485=CYLINDRICAL_SURFACE('',#42222,0.3);
#37486=CYLINDRICAL_SURFACE('',#42234,38.5);
#37487=CYLINDRICAL_SURFACE('',#42238,0.3);
#37488=CYLINDRICAL_SURFACE('',#42246,0.3);
#37489=CYLINDRICAL_SURFACE('',#42249,0.3);
#37490=CYLINDRICAL_SURFACE('',#42252,0.3);
#37491=CYLINDRICAL_SURFACE('',#42259,0.3);
#37492=CYLINDRICAL_SURFACE('',#42271,38.5);
#37493=CYLINDRICAL_SURFACE('',#42273,0.3);
#37494=CYLINDRICAL_SURFACE('',#42280,0.3);
#37495=CYLINDRICAL_SURFACE('',#42289,0.3);
#37496=CYLINDRICAL_SURFACE('',#42296,0.3);
#37497=CYLINDRICAL_SURFACE('',#42308,38.5);
#37498=CYLINDRICAL_SURFACE('',#42310,0.3);
#37499=CYLINDRICAL_SURFACE('',#42317,0.3);
#37500=CYLINDRICAL_SURFACE('',#42329,38.5);
#37501=CYLINDRICAL_SURFACE('',#42331,0.3);
#37502=CYLINDRICAL_SURFACE('',#42338,0.3);
#37503=CYLINDRICAL_SURFACE('',#42354,0.3);
#37504=CYLINDRICAL_SURFACE('',#42362,0.3);
#37505=CYLINDRICAL_SURFACE('',#42372,0.3);
#37506=CYLINDRICAL_SURFACE('',#42387,0.3);
#37507=CYLINDRICAL_SURFACE('',#42393,0.3);
#37508=CYLINDRICAL_SURFACE('',#42402,0.3);
#37509=CYLINDRICAL_SURFACE('',#42410,0.3);
#37510=CYLINDRICAL_SURFACE('',#42417,0.3);
#37511=CYLINDRICAL_SURFACE('',#42428,0.3);
#37512=CYLINDRICAL_SURFACE('',#42440,0.3);
#37513=CYLINDRICAL_SURFACE('',#42446,0.3);
#37514=CYLINDRICAL_SURFACE('',#42452,0.3);
#37515=CYLINDRICAL_SURFACE('',#42461,0.3);
#37516=CYLINDRICAL_SURFACE('',#42465,0.3);
#37517=CYLINDRICAL_SURFACE('',#42470,0.3);
#37518=CYLINDRICAL_SURFACE('',#42474,0.3);
#37519=CYLINDRICAL_SURFACE('',#42480,0.3);
#37520=CYLINDRICAL_SURFACE('',#42482,0.3);
#37521=CYLINDRICAL_SURFACE('',#42487,0.3);
#37522=CYLINDRICAL_SURFACE('',#42493,0.3);
#37523=CYLINDRICAL_SURFACE('',#42497,0.3);
#37524=CYLINDRICAL_SURFACE('',#42504,0.3);
#37525=CYLINDRICAL_SURFACE('',#42508,0.3);
#37526=CYLINDRICAL_SURFACE('',#42513,0.3);
#37527=CYLINDRICAL_SURFACE('',#42517,0.3);
#37528=CYLINDRICAL_SURFACE('',#42521,0.3);
#37529=CYLINDRICAL_SURFACE('',#42526,0.3);
#37530=CYLINDRICAL_SURFACE('',#42531,0.3);
#37531=CYLINDRICAL_SURFACE('',#42537,0.3);
#37532=CYLINDRICAL_SURFACE('',#42539,0.3);
#37533=CYLINDRICAL_SURFACE('',#42544,0.3);
#37534=CYLINDRICAL_SURFACE('',#42550,0.3);
#37535=CYLINDRICAL_SURFACE('',#42554,0.3);
#37536=CYLINDRICAL_SURFACE('',#42561,0.3);
#37537=CYLINDRICAL_SURFACE('',#42565,0.3);
#37538=CYLINDRICAL_SURFACE('',#42570,0.3);
#37539=CYLINDRICAL_SURFACE('',#42575,0.3);
#37540=CYLINDRICAL_SURFACE('',#42579,0.3);
#37541=CYLINDRICAL_SURFACE('',#42584,0.3);
#37542=CYLINDRICAL_SURFACE('',#42588,0.3);
#37543=CYLINDRICAL_SURFACE('',#42594,0.3);
#37544=CYLINDRICAL_SURFACE('',#42596,0.3);
#37545=CYLINDRICAL_SURFACE('',#42601,0.3);
#37546=CYLINDRICAL_SURFACE('',#42607,0.3);
#37547=CYLINDRICAL_SURFACE('',#42611,0.3);
#37548=CYLINDRICAL_SURFACE('',#42618,0.3);
#37549=CYLINDRICAL_SURFACE('',#42622,0.3);
#37550=CYLINDRICAL_SURFACE('',#42627,0.3);
#37551=CYLINDRICAL_SURFACE('',#42631,0.3);
#37552=CYLINDRICAL_SURFACE('',#42641,0.3);
#37553=CYLINDRICAL_SURFACE('',#42644,0.3);
#37554=CYLINDRICAL_SURFACE('',#42652,0.3);
#37555=CYLINDRICAL_SURFACE('',#42656,0.3);
#37556=CYLINDRICAL_SURFACE('',#42662,0.3);
#37557=CYLINDRICAL_SURFACE('',#42665,0.3);
#37558=CYLINDRICAL_SURFACE('',#42669,0.3);
#37559=CYLINDRICAL_SURFACE('',#42673,0.3);
#37560=CYLINDRICAL_SURFACE('',#42680,0.3);
#37561=CYLINDRICAL_SURFACE('',#42698,38.5);
#37562=CYLINDRICAL_SURFACE('',#42699,0.3);
#37563=CYLINDRICAL_SURFACE('',#42701,0.3);
#37564=CYLINDRICAL_SURFACE('',#42704,0.3);
#37565=CYLINDRICAL_SURFACE('',#42715,0.3);
#37566=CYLINDRICAL_SURFACE('',#42725,38.5);
#37567=CYLINDRICAL_SURFACE('',#42727,0.3);
#37568=CYLINDRICAL_SURFACE('',#42746,0.3);
#37569=CYLINDRICAL_SURFACE('',#42755,33.);
#37570=CYLINDRICAL_SURFACE('',#42773,0.3);
#37571=CYLINDRICAL_SURFACE('',#42776,0.3);
#37572=CYLINDRICAL_SURFACE('',#42780,0.3);
#37573=CYLINDRICAL_SURFACE('',#42783,0.3);
#37574=CYLINDRICAL_SURFACE('',#42784,0.3);
#37575=CYLINDRICAL_SURFACE('',#42786,0.3);
#37576=CYLINDRICAL_SURFACE('',#42788,0.3);
#37577=CYLINDRICAL_SURFACE('',#42789,0.3);
#37578=CYLINDRICAL_SURFACE('',#42791,0.3);
#37579=CYLINDRICAL_SURFACE('',#42794,0.3);
#37580=CYLINDRICAL_SURFACE('',#42795,0.3);
#37581=CYLINDRICAL_SURFACE('',#42798,0.3);
#37582=CYLINDRICAL_SURFACE('',#42799,0.3);
#37583=CYLINDRICAL_SURFACE('',#42801,0.3);
#37584=CYLINDRICAL_SURFACE('',#42804,0.3);
#37585=CYLINDRICAL_SURFACE('',#42805,0.3);
#37586=CYLINDRICAL_SURFACE('',#42806,0.3);
#37587=CYLINDRICAL_SURFACE('',#42807,0.3);
#37588=CYLINDRICAL_SURFACE('',#42809,0.3);
#37589=CYLINDRICAL_SURFACE('',#42812,0.3);
#37590=CYLINDRICAL_SURFACE('',#42814,0.3);
#37591=CYLINDRICAL_SURFACE('',#42815,0.3);
#37592=CYLINDRICAL_SURFACE('',#42816,0.3);
#37593=CYLINDRICAL_SURFACE('',#42818,0.3);
#37594=CYLINDRICAL_SURFACE('',#42821,0.3);
#37595=CYLINDRICAL_SURFACE('',#42822,0.3);
#37596=CYLINDRICAL_SURFACE('',#42823,0.3);
#37597=CYLINDRICAL_SURFACE('',#42824,0.3);
#37598=CYLINDRICAL_SURFACE('',#42826,0.3);
#37599=CYLINDRICAL_SURFACE('',#42829,0.3);
#37600=CYLINDRICAL_SURFACE('',#42830,0.3);
#37601=CYLINDRICAL_SURFACE('',#42831,0.3);
#37602=CYLINDRICAL_SURFACE('',#42832,0.3);
#37603=CYLINDRICAL_SURFACE('',#42834,0.3);
#37604=CYLINDRICAL_SURFACE('',#42837,0.3);
#37605=CYLINDRICAL_SURFACE('',#42838,0.3);
#37606=CYLINDRICAL_SURFACE('',#42839,0.3);
#37607=CYLINDRICAL_SURFACE('',#42840,0.3);
#37608=CYLINDRICAL_SURFACE('',#42842,0.3);
#37609=CYLINDRICAL_SURFACE('',#42845,0.3);
#37610=CYLINDRICAL_SURFACE('',#42847,0.3);
#37611=CYLINDRICAL_SURFACE('',#42848,0.3);
#37612=CYLINDRICAL_SURFACE('',#42849,0.3);
#37613=CYLINDRICAL_SURFACE('',#42851,0.3);
#37614=CYLINDRICAL_SURFACE('',#42854,0.3);
#37615=CYLINDRICAL_SURFACE('',#42855,0.3);
#37616=CYLINDRICAL_SURFACE('',#42856,0.3);
#37617=CYLINDRICAL_SURFACE('',#42857,0.3);
#37618=CYLINDRICAL_SURFACE('',#42859,0.3);
#37619=CYLINDRICAL_SURFACE('',#42862,0.3);
#37620=CYLINDRICAL_SURFACE('',#42863,0.3);
#37621=CYLINDRICAL_SURFACE('',#42866,0.3);
#37622=CYLINDRICAL_SURFACE('',#42867,0.3);
#37623=CYLINDRICAL_SURFACE('',#42869,0.3);
#37624=CYLINDRICAL_SURFACE('',#42872,0.3);
#37625=CYLINDRICAL_SURFACE('',#42874,0.3);
#37626=CYLINDRICAL_SURFACE('',#42875,0.3);
#37627=CYLINDRICAL_SURFACE('',#42876,0.3);
#37628=CYLINDRICAL_SURFACE('',#42878,0.3);
#37629=CYLINDRICAL_SURFACE('',#42881,0.3);
#37630=CYLINDRICAL_SURFACE('',#42882,0.3);
#37631=CYLINDRICAL_SURFACE('',#42883,0.3);
#37632=CYLINDRICAL_SURFACE('',#42884,0.3);
#37633=CYLINDRICAL_SURFACE('',#42886,0.3);
#37634=CYLINDRICAL_SURFACE('',#42889,0.3);
#37635=CYLINDRICAL_SURFACE('',#42890,0.3);
#37636=CYLINDRICAL_SURFACE('',#42891,0.3);
#37637=CYLINDRICAL_SURFACE('',#42892,0.3);
#37638=CYLINDRICAL_SURFACE('',#42894,0.3);
#37639=CYLINDRICAL_SURFACE('',#42897,0.3);
#37640=CYLINDRICAL_SURFACE('',#42898,0.3);
#37641=CYLINDRICAL_SURFACE('',#42901,0.3);
#37642=CYLINDRICAL_SURFACE('',#42902,0.3);
#37643=CYLINDRICAL_SURFACE('',#42904,0.3);
#37644=CYLINDRICAL_SURFACE('',#42907,0.3);
#37645=CYLINDRICAL_SURFACE('',#42908,0.3);
#37646=CYLINDRICAL_SURFACE('',#42909,0.3);
#37647=CYLINDRICAL_SURFACE('',#42910,0.3);
#37648=CYLINDRICAL_SURFACE('',#42912,0.3);
#37649=CYLINDRICAL_SURFACE('',#42915,0.3);
#37650=CYLINDRICAL_SURFACE('',#42920,0.3);
#37651=CYLINDRICAL_SURFACE('',#42922,0.3);
#37652=CYLINDRICAL_SURFACE('',#42923,0.3);
#37653=CYLINDRICAL_SURFACE('',#42926,38.5);
#37654=CYLINDRICAL_SURFACE('',#42929,38.5);
#37655=CYLINDRICAL_SURFACE('',#42934,38.5);
#37656=CYLINDRICAL_SURFACE('',#42939,38.5);
#37657=CYLINDRICAL_SURFACE('',#42947,38.5);
#37658=CYLINDRICAL_SURFACE('',#42952,38.5);
#37659=CYLINDRICAL_SURFACE('',#42957,38.5);
#37660=CYLINDRICAL_SURFACE('',#42965,38.5);
#37661=CYLINDRICAL_SURFACE('',#42970,38.5);
#37662=CYLINDRICAL_SURFACE('',#42975,38.5);
#37663=CYLINDRICAL_SURFACE('',#42983,38.5);
#37664=CYLINDRICAL_SURFACE('',#42988,38.5);
#37665=CYLINDRICAL_SURFACE('',#42993,38.5);
#38166=ADVANCED_FACE('',(#2363),#37325,.T.);
#38167=ADVANCED_FACE('',(#2364),#1980,.F.);
#38168=ADVANCED_FACE('',(#2365),#302,.T.);
#38169=ADVANCED_FACE('',(#2366),#37326,.T.);
#38170=ADVANCED_FACE('',(#2367),#801,.T.);
#38171=ADVANCED_FACE('',(#2368),#37327,.T.);
#38172=ADVANCED_FACE('',(#2369),#1981,.F.);
#38173=ADVANCED_FACE('',(#2370),#303,.T.);
#38174=ADVANCED_FACE('',(#2371),#304,.T.);
#38175=ADVANCED_FACE('',(#2372),#305,.T.);
#38176=ADVANCED_FACE('',(#2373),#1156,.F.);
#38177=ADVANCED_FACE('',(#2374,#1047),#1157,.T.);
#38178=ADVANCED_FACE('',(#2375),#802,.T.);
#38179=ADVANCED_FACE('',(#2376),#577,.T.);
#38180=ADVANCED_FACE('',(#2377),#803,.T.);
#38181=ADVANCED_FACE('',(#2378),#37328,.T.);
#38182=ADVANCED_FACE('',(#2379),#37329,.T.);
#38183=ADVANCED_FACE('',(#2380),#1982,.F.);
#38184=ADVANCED_FACE('',(#2381),#306,.T.);
#38185=ADVANCED_FACE('',(#2382),#37330,.T.);
#38186=ADVANCED_FACE('',(#2383),#804,.T.);
#38187=ADVANCED_FACE('',(#2384),#37331,.T.);
#38188=ADVANCED_FACE('',(#2385),#1983,.F.);
#38189=ADVANCED_FACE('',(#2386),#307,.T.);
#38190=ADVANCED_FACE('',(#2387),#308,.T.);
#38191=ADVANCED_FACE('',(#2388),#309,.T.);
#38192=ADVANCED_FACE('',(#2389),#1158,.F.);
#38193=ADVANCED_FACE('',(#2390),#805,.T.);
#38194=ADVANCED_FACE('',(#2391),#578,.T.);
#38195=ADVANCED_FACE('',(#2392),#806,.T.);
#38196=ADVANCED_FACE('',(#2393),#37332,.T.);
#38197=ADVANCED_FACE('',(#2394),#37333,.T.);
#38198=ADVANCED_FACE('',(#2395),#1984,.F.);
#38199=ADVANCED_FACE('',(#2396),#310,.T.);
#38200=ADVANCED_FACE('',(#2397),#37334,.T.);
#38201=ADVANCED_FACE('',(#2398),#807,.T.);
#38202=ADVANCED_FACE('',(#2399),#37335,.T.);
#38203=ADVANCED_FACE('',(#2400),#1985,.F.);
#38204=ADVANCED_FACE('',(#2401),#311,.T.);
#38205=ADVANCED_FACE('',(#2402),#312,.T.);
#38206=ADVANCED_FACE('',(#2403),#313,.T.);
#38207=ADVANCED_FACE('',(#2404),#1159,.F.);
#38208=ADVANCED_FACE('',(#2405),#808,.T.);
#38209=ADVANCED_FACE('',(#2406),#579,.T.);
#38210=ADVANCED_FACE('',(#2407),#809,.T.);
#38211=ADVANCED_FACE('',(#2408),#37336,.T.);
#38212=ADVANCED_FACE('',(#2409),#37337,.T.);
#38213=ADVANCED_FACE('',(#2410),#1986,.F.);
#38214=ADVANCED_FACE('',(#2411),#314,.T.);
#38215=ADVANCED_FACE('',(#2412),#810,.T.);
#38216=ADVANCED_FACE('',(#2413),#37338,.T.);
#38217=ADVANCED_FACE('',(#2414),#315,.T.);
#38218=ADVANCED_FACE('',(#2415),#37339,.T.);
#38219=ADVANCED_FACE('',(#2416),#1987,.F.);
#38220=ADVANCED_FACE('',(#2417),#316,.T.);
#38221=ADVANCED_FACE('',(#2418),#317,.T.);
#38222=ADVANCED_FACE('',(#2419),#811,.T.);
#38223=ADVANCED_FACE('',(#2420),#580,.T.);
#38224=ADVANCED_FACE('',(#2421),#812,.T.);
#38225=ADVANCED_FACE('',(#2422),#37340,.T.);
#38226=ADVANCED_FACE('',(#2423),#37341,.T.);
#38227=ADVANCED_FACE('',(#2424),#1160,.F.);
#38228=ADVANCED_FACE('',(#2425),#37342,.T.);
#38229=ADVANCED_FACE('',(#2426),#1988,.F.);
#38230=ADVANCED_FACE('',(#2427),#318,.T.);
#38231=ADVANCED_FACE('',(#2428),#813,.T.);
#38232=ADVANCED_FACE('',(#2429),#37343,.T.);
#38233=ADVANCED_FACE('',(#2430),#319,.T.);
#38234=ADVANCED_FACE('',(#2431),#37344,.T.);
#38235=ADVANCED_FACE('',(#2432),#1989,.F.);
#38236=ADVANCED_FACE('',(#2433),#320,.T.);
#38237=ADVANCED_FACE('',(#2434),#321,.T.);
#38238=ADVANCED_FACE('',(#2435),#814,.T.);
#38239=ADVANCED_FACE('',(#2436),#581,.T.);
#38240=ADVANCED_FACE('',(#2437),#815,.T.);
#38241=ADVANCED_FACE('',(#2438),#37345,.T.);
#38242=ADVANCED_FACE('',(#2439),#37346,.T.);
#38243=ADVANCED_FACE('',(#2440),#1161,.F.);
#38244=ADVANCED_FACE('',(#2441),#37347,.T.);
#38245=ADVANCED_FACE('',(#2442),#1990,.F.);
#38246=ADVANCED_FACE('',(#2443),#322,.T.);
#38247=ADVANCED_FACE('',(#2444),#37348,.T.);
#38248=ADVANCED_FACE('',(#2445),#323,.T.);
#38249=ADVANCED_FACE('',(#2446,#1048),#1162,.T.);
#38250=ADVANCED_FACE('',(#2447),#816,.T.);
#38251=ADVANCED_FACE('',(#2448),#582,.T.);
#38252=ADVANCED_FACE('',(#2449),#817,.T.);
#38253=ADVANCED_FACE('',(#2450),#37349,.T.);
#38254=ADVANCED_FACE('',(#2451),#37350,.T.);
#38255=ADVANCED_FACE('',(#2452),#1991,.F.);
#38256=ADVANCED_FACE('',(#2453),#324,.T.);
#38257=ADVANCED_FACE('',(#2454),#37351,.T.);
#38258=ADVANCED_FACE('',(#2455),#325,.T.);
#38259=ADVANCED_FACE('',(#2456),#818,.T.);
#38260=ADVANCED_FACE('',(#2457),#583,.T.);
#38261=ADVANCED_FACE('',(#2458),#819,.T.);
#38262=ADVANCED_FACE('',(#2459),#37352,.T.);
#38263=ADVANCED_FACE('',(#2460),#37353,.T.);
#38264=ADVANCED_FACE('',(#2461),#1992,.F.);
#38265=ADVANCED_FACE('',(#2462),#326,.T.);
#38266=ADVANCED_FACE('',(#2463),#37354,.T.);
#38267=ADVANCED_FACE('',(#2464),#327,.T.);
#38268=ADVANCED_FACE('',(#2465),#820,.T.);
#38269=ADVANCED_FACE('',(#2466),#584,.T.);
#38270=ADVANCED_FACE('',(#2467),#821,.T.);
#38271=ADVANCED_FACE('',(#2468),#37355,.T.);
#38272=ADVANCED_FACE('',(#2469),#37356,.T.);
#38273=ADVANCED_FACE('',(#2470),#37357,.T.);
#38274=ADVANCED_FACE('',(#2471),#1993,.F.);
#38275=ADVANCED_FACE('',(#2472),#328,.T.);
#38276=ADVANCED_FACE('',(#2473),#822,.T.);
#38277=ADVANCED_FACE('',(#2474),#37358,.T.);
#38278=ADVANCED_FACE('',(#2475),#329,.T.);
#38279=ADVANCED_FACE('',(#2476),#1994,.F.);
#38280=ADVANCED_FACE('',(#2477),#330,.T.);
#38281=ADVANCED_FACE('',(#2478),#331,.T.);
#38282=ADVANCED_FACE('',(#2479),#37359,.T.);
#38283=ADVANCED_FACE('',(#2480),#37360,.T.);
#38284=ADVANCED_FACE('',(#2481),#1163,.F.);
#38285=ADVANCED_FACE('',(#2482),#823,.T.);
#38286=ADVANCED_FACE('',(#2483),#585,.T.);
#38287=ADVANCED_FACE('',(#2484),#37361,.T.);
#38288=ADVANCED_FACE('',(#2485),#1995,.F.);
#38289=ADVANCED_FACE('',(#2486),#332,.T.);
#38290=ADVANCED_FACE('',(#2487),#37362,.T.);
#38291=ADVANCED_FACE('',(#2488),#333,.T.);
#38292=ADVANCED_FACE('',(#2489),#824,.T.);
#38293=ADVANCED_FACE('',(#2490),#586,.T.);
#38294=ADVANCED_FACE('',(#2491),#825,.T.);
#38295=ADVANCED_FACE('',(#2492),#37363,.T.);
#38296=ADVANCED_FACE('',(#2493),#37364,.T.);
#38297=ADVANCED_FACE('',(#2494),#1996,.F.);
#38298=ADVANCED_FACE('',(#2495),#334,.T.);
#38299=ADVANCED_FACE('',(#2496),#37365,.T.);
#38300=ADVANCED_FACE('',(#2497),#335,.T.);
#38301=ADVANCED_FACE('',(#2498),#826,.T.);
#38302=ADVANCED_FACE('',(#2499),#587,.T.);
#38303=ADVANCED_FACE('',(#2500),#827,.T.);
#38304=ADVANCED_FACE('',(#2501),#37366,.T.);
#38305=ADVANCED_FACE('',(#2502),#37367,.T.);
#38306=ADVANCED_FACE('',(#2503),#1997,.F.);
#38307=ADVANCED_FACE('',(#2504),#336,.T.);
#38308=ADVANCED_FACE('',(#2505),#37368,.T.);
#38309=ADVANCED_FACE('',(#2506),#337,.T.);
#38310=ADVANCED_FACE('',(#2507),#828,.T.);
#38311=ADVANCED_FACE('',(#2508),#588,.T.);
#38312=ADVANCED_FACE('',(#2509),#37369,.T.);
#38313=ADVANCED_FACE('',(#2510),#37370,.T.);
#38314=ADVANCED_FACE('',(#2511),#1998,.F.);
#38315=ADVANCED_FACE('',(#2512),#338,.T.);
#38316=ADVANCED_FACE('',(#2513),#829,.T.);
#38317=ADVANCED_FACE('',(#2514),#37371,.T.);
#38318=ADVANCED_FACE('',(#2515),#339,.T.);
#38319=ADVANCED_FACE('',(#2516),#1999,.F.);
#38320=ADVANCED_FACE('',(#2517),#340,.T.);
#38321=ADVANCED_FACE('',(#2518),#341,.T.);
#38322=ADVANCED_FACE('',(#2519),#37372,.T.);
#38323=ADVANCED_FACE('',(#2520),#37373,.T.);
#38324=ADVANCED_FACE('',(#2521),#1164,.F.);
#38325=ADVANCED_FACE('',(#2522),#830,.T.);
#38326=ADVANCED_FACE('',(#2523),#589,.T.);
#38327=ADVANCED_FACE('',(#2524),#2000,.F.);
#38328=ADVANCED_FACE('',(#2525),#831,.T.);
#38329=ADVANCED_FACE('',(#2526),#342,.T.);
#38330=ADVANCED_FACE('',(#2527),#37374,.T.);
#38331=ADVANCED_FACE('',(#2528),#343,.T.);
#38332=ADVANCED_FACE('',(#2529),#1165,.F.);
#38333=ADVANCED_FACE('',(#2530),#2001,.F.);
#38334=ADVANCED_FACE('',(#2531),#37375,.T.);
#38335=ADVANCED_FACE('',(#2532),#344,.T.);
#38336=ADVANCED_FACE('',(#2533),#345,.T.);
#38337=ADVANCED_FACE('',(#2534),#1166,.F.);
#38338=ADVANCED_FACE('',(#2535),#37376,.T.);
#38339=ADVANCED_FACE('',(#2536),#2002,.F.);
#38340=ADVANCED_FACE('',(#2537),#346,.T.);
#38341=ADVANCED_FACE('',(#2538),#37377,.T.);
#38342=ADVANCED_FACE('',(#2539),#347,.T.);
#38343=ADVANCED_FACE('',(#2540),#832,.T.);
#38344=ADVANCED_FACE('',(#2541),#590,.T.);
#38345=ADVANCED_FACE('',(#2542),#833,.T.);
#38346=ADVANCED_FACE('',(#2543),#37378,.T.);
#38347=ADVANCED_FACE('',(#2544),#2003,.F.);
#38348=ADVANCED_FACE('',(#2545),#37379,.T.);
#38349=ADVANCED_FACE('',(#2546),#348,.T.);
#38350=ADVANCED_FACE('',(#2547),#349,.T.);
#38351=ADVANCED_FACE('',(#2548),#1167,.F.);
#38352=ADVANCED_FACE('',(#2549),#37380,.T.);
#38353=ADVANCED_FACE('',(#2550),#2004,.F.);
#38354=ADVANCED_FACE('',(#2551),#350,.T.);
#38355=ADVANCED_FACE('',(#2552),#37381,.T.);
#38356=ADVANCED_FACE('',(#2553),#351,.T.);
#38357=ADVANCED_FACE('',(#2554),#834,.T.);
#38358=ADVANCED_FACE('',(#2555),#591,.T.);
#38359=ADVANCED_FACE('',(#2556),#2005,.F.);
#38360=ADVANCED_FACE('',(#2557),#37382,.T.);
#38361=ADVANCED_FACE('',(#2558),#352,.T.);
#38362=ADVANCED_FACE('',(#2559),#353,.T.);
#38363=ADVANCED_FACE('',(#2560),#37383,.T.);
#38364=ADVANCED_FACE('',(#2561),#1168,.F.);
#38365=ADVANCED_FACE('',(#2562),#2006,.F.);
#38366=ADVANCED_FACE('',(#2563),#835,.T.);
#38367=ADVANCED_FACE('',(#2564),#354,.T.);
#38368=ADVANCED_FACE('',(#2565),#37384,.T.);
#38369=ADVANCED_FACE('',(#2566),#355,.T.);
#38370=ADVANCED_FACE('',(#2567),#1169,.F.);
#38371=ADVANCED_FACE('',(#2568),#37385,.T.);
#38372=ADVANCED_FACE('',(#2569),#1170,.F.);
#38373=ADVANCED_FACE('',(#2570),#37386,.T.);
#38374=ADVANCED_FACE('',(#2571),#2007,.F.);
#38375=ADVANCED_FACE('',(#2572),#356,.T.);
#38376=ADVANCED_FACE('',(#2573),#37387,.T.);
#38377=ADVANCED_FACE('',(#2574),#357,.T.);
#38378=ADVANCED_FACE('',(#2575),#836,.T.);
#38379=ADVANCED_FACE('',(#2576),#592,.T.);
#38380=ADVANCED_FACE('',(#2577),#37388,.T.);
#38381=ADVANCED_FACE('',(#2578),#2008,.F.);
#38382=ADVANCED_FACE('',(#2579),#358,.T.);
#38383=ADVANCED_FACE('',(#2580),#37389,.T.);
#38384=ADVANCED_FACE('',(#2581),#359,.T.);
#38385=ADVANCED_FACE('',(#2582),#837,.T.);
#38386=ADVANCED_FACE('',(#2583),#593,.T.);
#38387=ADVANCED_FACE('',(#2584),#838,.T.);
#38388=ADVANCED_FACE('',(#2585),#37390,.T.);
#38389=ADVANCED_FACE('',(#2586),#37391,.T.);
#38390=ADVANCED_FACE('',(#2587),#2009,.F.);
#38391=ADVANCED_FACE('',(#2588),#360,.T.);
#38392=ADVANCED_FACE('',(#2589),#37392,.T.);
#38393=ADVANCED_FACE('',(#2590),#361,.T.);
#38394=ADVANCED_FACE('',(#2591),#839,.T.);
#38395=ADVANCED_FACE('',(#2592),#594,.T.);
#38396=ADVANCED_FACE('',(#2593),#840,.T.);
#38397=ADVANCED_FACE('',(#2594),#37393,.T.);
#38398=ADVANCED_FACE('',(#2595),#2010,.F.);
#38399=ADVANCED_FACE('',(#2596),#37394,.T.);
#38400=ADVANCED_FACE('',(#2597),#362,.T.);
#38401=ADVANCED_FACE('',(#2598),#363,.T.);
#38402=ADVANCED_FACE('',(#2599),#1171,.F.);
#38403=ADVANCED_FACE('',(#2600),#37395,.T.);
#38404=ADVANCED_FACE('',(#2601),#2011,.F.);
#38405=ADVANCED_FACE('',(#2602),#364,.T.);
#38406=ADVANCED_FACE('',(#2603),#37396,.T.);
#38407=ADVANCED_FACE('',(#2604),#365,.T.);
#38408=ADVANCED_FACE('',(#2605),#841,.T.);
#38409=ADVANCED_FACE('',(#2606),#595,.T.);
#38410=ADVANCED_FACE('',(#2607),#842,.T.);
#38411=ADVANCED_FACE('',(#2608),#37397,.T.);
#38412=ADVANCED_FACE('',(#2609),#2012,.F.);
#38413=ADVANCED_FACE('',(#2610),#37398,.T.);
#38414=ADVANCED_FACE('',(#2611),#366,.T.);
#38415=ADVANCED_FACE('',(#2612),#367,.T.);
#38416=ADVANCED_FACE('',(#2613),#1172,.F.);
#38417=ADVANCED_FACE('',(#2614),#37399,.T.);
#38418=ADVANCED_FACE('',(#2615),#1173,.F.);
#38419=ADVANCED_FACE('',(#2616),#37400,.T.);
#38420=ADVANCED_FACE('',(#2617),#2013,.F.);
#38421=ADVANCED_FACE('',(#2618),#368,.T.);
#38422=ADVANCED_FACE('',(#2619),#37401,.T.);
#38423=ADVANCED_FACE('',(#2620),#369,.T.);
#38424=ADVANCED_FACE('',(#2621),#843,.T.);
#38425=ADVANCED_FACE('',(#2622),#596,.T.);
#38426=ADVANCED_FACE('',(#2623),#844,.T.);
#38427=ADVANCED_FACE('',(#2624),#37402,.T.);
#38428=ADVANCED_FACE('',(#2625),#37403,.T.);
#38429=ADVANCED_FACE('',(#2626),#2014,.F.);
#38430=ADVANCED_FACE('',(#2627),#370,.T.);
#38431=ADVANCED_FACE('',(#2628),#37404,.T.);
#38432=ADVANCED_FACE('',(#2629),#371,.T.);
#38433=ADVANCED_FACE('',(#2630),#845,.T.);
#38434=ADVANCED_FACE('',(#2631),#597,.T.);
#38435=ADVANCED_FACE('',(#2632),#846,.T.);
#38436=ADVANCED_FACE('',(#2633),#37405,.T.);
#38437=ADVANCED_FACE('',(#2634),#37406,.T.);
#38438=ADVANCED_FACE('',(#2635),#2015,.F.);
#38439=ADVANCED_FACE('',(#2636),#372,.T.);
#38440=ADVANCED_FACE('',(#2637),#37407,.T.);
#38441=ADVANCED_FACE('',(#2638),#373,.T.);
#38442=ADVANCED_FACE('',(#2639),#847,.T.);
#38443=ADVANCED_FACE('',(#2640),#598,.T.);
#38444=ADVANCED_FACE('',(#2641),#2016,.F.);
#38445=ADVANCED_FACE('',(#2642),#37408,.T.);
#38446=ADVANCED_FACE('',(#2643),#374,.T.);
#38447=ADVANCED_FACE('',(#2644),#375,.T.);
#38448=ADVANCED_FACE('',(#2645),#1174,.F.);
#38449=ADVANCED_FACE('',(#2646),#2017,.F.);
#38450=ADVANCED_FACE('',(#2647),#37409,.T.);
#38451=ADVANCED_FACE('',(#2648),#376,.T.);
#38452=ADVANCED_FACE('',(#2649),#377,.T.);
#38453=ADVANCED_FACE('',(#2650),#1175,.F.);
#38454=ADVANCED_FACE('',(#2651),#37410,.T.);
#38455=ADVANCED_FACE('',(#2652),#2018,.F.);
#38456=ADVANCED_FACE('',(#2653),#378,.T.);
#38457=ADVANCED_FACE('',(#2654),#37411,.T.);
#38458=ADVANCED_FACE('',(#2655),#379,.T.);
#38459=ADVANCED_FACE('',(#2656),#848,.T.);
#38460=ADVANCED_FACE('',(#2657),#599,.T.);
#38461=ADVANCED_FACE('',(#2658),#849,.T.);
#38462=ADVANCED_FACE('',(#2659),#37412,.T.);
#38463=ADVANCED_FACE('',(#2660),#2019,.F.);
#38464=ADVANCED_FACE('',(#2661),#37413,.T.);
#38465=ADVANCED_FACE('',(#2662),#380,.T.);
#38466=ADVANCED_FACE('',(#2663),#381,.T.);
#38467=ADVANCED_FACE('',(#2664),#1176,.F.);
#38468=ADVANCED_FACE('',(#2665),#37414,.T.);
#38469=ADVANCED_FACE('',(#2666),#1177,.F.);
#38470=ADVANCED_FACE('',(#2667),#37415,.T.);
#38471=ADVANCED_FACE('',(#2668),#1178,.F.);
#38472=ADVANCED_FACE('',(#2669),#2020,.F.);
#38473=ADVANCED_FACE('',(#2670),#850,.T.);
#38474=ADVANCED_FACE('',(#2671),#382,.T.);
#38475=ADVANCED_FACE('',(#2672),#37416,.T.);
#38476=ADVANCED_FACE('',(#2673),#383,.T.);
#38477=ADVANCED_FACE('',(#2674),#1179,.F.);
#38478=ADVANCED_FACE('',(#2675),#2021,.F.);
#38479=ADVANCED_FACE('',(#2676),#37417,.T.);
#38480=ADVANCED_FACE('',(#2677),#384,.T.);
#38481=ADVANCED_FACE('',(#2678),#385,.T.);
#38482=ADVANCED_FACE('',(#2679),#1180,.F.);
#38483=ADVANCED_FACE('',(#2680),#37418,.T.);
#38484=ADVANCED_FACE('',(#2681),#2022,.F.);
#38485=ADVANCED_FACE('',(#2682),#386,.T.);
#38486=ADVANCED_FACE('',(#2683),#37419,.T.);
#38487=ADVANCED_FACE('',(#2684),#387,.T.);
#38488=ADVANCED_FACE('',(#2685),#851,.T.);
#38489=ADVANCED_FACE('',(#2686),#600,.T.);
#38490=ADVANCED_FACE('',(#2687),#2023,.F.);
#38491=ADVANCED_FACE('',(#2688),#37420,.T.);
#38492=ADVANCED_FACE('',(#2689),#388,.T.);
#38493=ADVANCED_FACE('',(#2690),#389,.T.);
#38494=ADVANCED_FACE('',(#2691),#1181,.F.);
#38495=ADVANCED_FACE('',(#2692),#37421,.T.);
#38496=ADVANCED_FACE('',(#2693),#2024,.F.);
#38497=ADVANCED_FACE('',(#2694),#390,.T.);
#38498=ADVANCED_FACE('',(#2695),#37422,.T.);
#38499=ADVANCED_FACE('',(#2696),#391,.T.);
#38500=ADVANCED_FACE('',(#2697),#852,.T.);
#38501=ADVANCED_FACE('',(#2698),#601,.T.);
#38502=ADVANCED_FACE('',(#2699),#853,.T.);
#38503=ADVANCED_FACE('',(#2700),#37423,.T.);
#38504=ADVANCED_FACE('',(#2701),#2025,.F.);
#38505=ADVANCED_FACE('',(#2702),#37424,.T.);
#38506=ADVANCED_FACE('',(#2703),#392,.T.);
#38507=ADVANCED_FACE('',(#2704),#393,.T.);
#38508=ADVANCED_FACE('',(#2705),#1182,.F.);
#38509=ADVANCED_FACE('',(#2706),#37425,.T.);
#38510=ADVANCED_FACE('',(#2707),#1183,.F.);
#38511=ADVANCED_FACE('',(#2708),#2026,.F.);
#38512=ADVANCED_FACE('',(#2709),#854,.T.);
#38513=ADVANCED_FACE('',(#2710),#394,.T.);
#38514=ADVANCED_FACE('',(#2711),#37426,.T.);
#38515=ADVANCED_FACE('',(#2712),#395,.T.);
#38516=ADVANCED_FACE('',(#2713),#1184,.F.);
#38517=ADVANCED_FACE('',(#2714),#37427,.T.);
#38518=ADVANCED_FACE('',(#2715),#1185,.F.);
#38519=ADVANCED_FACE('',(#2716),#37428,.T.);
#38520=ADVANCED_FACE('',(#2717),#2027,.F.);
#38521=ADVANCED_FACE('',(#2718),#396,.T.);
#38522=ADVANCED_FACE('',(#2719),#37429,.T.);
#38523=ADVANCED_FACE('',(#2720),#397,.T.);
#38524=ADVANCED_FACE('',(#2721),#855,.T.);
#38525=ADVANCED_FACE('',(#2722),#602,.T.);
#38526=ADVANCED_FACE('',(#2723),#856,.T.);
#38527=ADVANCED_FACE('',(#2724),#37430,.T.);
#38528=ADVANCED_FACE('',(#2725),#37431,.T.);
#38529=ADVANCED_FACE('',(#2726),#2028,.F.);
#38530=ADVANCED_FACE('',(#2727),#398,.T.);
#38531=ADVANCED_FACE('',(#2728),#37432,.T.);
#38532=ADVANCED_FACE('',(#2729),#399,.T.);
#38533=ADVANCED_FACE('',(#2730),#857,.T.);
#38534=ADVANCED_FACE('',(#2731),#603,.T.);
#38535=ADVANCED_FACE('',(#2732),#858,.T.);
#38536=ADVANCED_FACE('',(#2733),#37433,.T.);
#38537=ADVANCED_FACE('',(#2734),#37434,.T.);
#38538=ADVANCED_FACE('',(#2735),#2029,.F.);
#38539=ADVANCED_FACE('',(#2736),#400,.T.);
#38540=ADVANCED_FACE('',(#2737),#37435,.T.);
#38541=ADVANCED_FACE('',(#2738),#401,.T.);
#38542=ADVANCED_FACE('',(#2739),#859,.T.);
#38543=ADVANCED_FACE('',(#2740),#604,.T.);
#38544=ADVANCED_FACE('',(#2741),#37436,.T.);
#38545=ADVANCED_FACE('',(#2742),#2030,.F.);
#38546=ADVANCED_FACE('',(#2743),#402,.T.);
#38547=ADVANCED_FACE('',(#2744),#37437,.T.);
#38548=ADVANCED_FACE('',(#2745),#403,.T.);
#38549=ADVANCED_FACE('',(#2746),#860,.T.);
#38550=ADVANCED_FACE('',(#2747),#605,.T.);
#38551=ADVANCED_FACE('',(#2748),#861,.T.);
#38552=ADVANCED_FACE('',(#2749),#37438,.T.);
#38553=ADVANCED_FACE('',(#2750),#2031,.F.);
#38554=ADVANCED_FACE('',(#2751),#37439,.T.);
#38555=ADVANCED_FACE('',(#2752),#404,.T.);
#38556=ADVANCED_FACE('',(#2753),#405,.T.);
#38557=ADVANCED_FACE('',(#2754),#1186,.F.);
#38558=ADVANCED_FACE('',(#2755),#2032,.F.);
#38559=ADVANCED_FACE('',(#2756),#862,.T.);
#38560=ADVANCED_FACE('',(#2757),#406,.T.);
#38561=ADVANCED_FACE('',(#2758),#37440,.T.);
#38562=ADVANCED_FACE('',(#2759),#407,.T.);
#38563=ADVANCED_FACE('',(#2760),#1187,.F.);
#38564=ADVANCED_FACE('',(#2761),#37441,.T.);
#38565=ADVANCED_FACE('',(#2762),#2033,.F.);
#38566=ADVANCED_FACE('',(#2763),#408,.T.);
#38567=ADVANCED_FACE('',(#2764),#37442,.T.);
#38568=ADVANCED_FACE('',(#2765),#409,.T.);
#38569=ADVANCED_FACE('',(#2766),#863,.T.);
#38570=ADVANCED_FACE('',(#2767),#606,.T.);
#38571=ADVANCED_FACE('',(#2768),#864,.T.);
#38572=ADVANCED_FACE('',(#2769),#37443,.T.);
#38573=ADVANCED_FACE('',(#2770),#37444,.T.);
#38574=ADVANCED_FACE('',(#2771),#2034,.F.);
#38575=ADVANCED_FACE('',(#2772),#410,.T.);
#38576=ADVANCED_FACE('',(#2773),#37445,.T.);
#38577=ADVANCED_FACE('',(#2774),#411,.T.);
#38578=ADVANCED_FACE('',(#2775),#865,.T.);
#38579=ADVANCED_FACE('',(#2776),#607,.T.);
#38580=ADVANCED_FACE('',(#2777),#2035,.F.);
#38581=ADVANCED_FACE('',(#2778),#37446,.T.);
#38582=ADVANCED_FACE('',(#2779),#412,.T.);
#38583=ADVANCED_FACE('',(#2780),#413,.T.);
#38584=ADVANCED_FACE('',(#2781),#1188,.F.);
#38585=ADVANCED_FACE('',(#2782),#2036,.F.);
#38586=ADVANCED_FACE('',(#2783),#37447,.T.);
#38587=ADVANCED_FACE('',(#2784),#414,.T.);
#38588=ADVANCED_FACE('',(#2785),#415,.T.);
#38589=ADVANCED_FACE('',(#2786),#1189,.F.);
#38590=ADVANCED_FACE('',(#2787),#37448,.T.);
#38591=ADVANCED_FACE('',(#2788),#2037,.F.);
#38592=ADVANCED_FACE('',(#2789),#416,.T.);
#38593=ADVANCED_FACE('',(#2790),#37449,.T.);
#38594=ADVANCED_FACE('',(#2791),#417,.T.);
#38595=ADVANCED_FACE('',(#2792),#866,.T.);
#38596=ADVANCED_FACE('',(#2793),#608,.T.);
#38597=ADVANCED_FACE('',(#2794),#867,.T.);
#38598=ADVANCED_FACE('',(#2795),#37450,.T.);
#38599=ADVANCED_FACE('',(#2796),#2038,.F.);
#38600=ADVANCED_FACE('',(#2797),#37451,.T.);
#38601=ADVANCED_FACE('',(#2798),#418,.T.);
#38602=ADVANCED_FACE('',(#2799),#419,.T.);
#38603=ADVANCED_FACE('',(#2800),#37452,.T.);
#38604=ADVANCED_FACE('',(#2801),#1190,.F.);
#38605=ADVANCED_FACE('',(#2802),#2039,.F.);
#38606=ADVANCED_FACE('',(#2803),#37453,.T.);
#38607=ADVANCED_FACE('',(#2804),#420,.T.);
#38608=ADVANCED_FACE('',(#2805),#421,.T.);
#38609=ADVANCED_FACE('',(#2806),#1191,.F.);
#38610=ADVANCED_FACE('',(#2807),#37454,.T.);
#38611=ADVANCED_FACE('',(#2808),#1192,.F.);
#38612=ADVANCED_FACE('',(#2809),#37455,.T.);
#38613=ADVANCED_FACE('',(#2810),#1193,.F.);
#38614=ADVANCED_FACE('',(#2811),#2040,.F.);
#38615=ADVANCED_FACE('',(#2812),#868,.T.);
#38616=ADVANCED_FACE('',(#2813),#422,.T.);
#38617=ADVANCED_FACE('',(#2814),#37456,.T.);
#38618=ADVANCED_FACE('',(#2815),#423,.T.);
#38619=ADVANCED_FACE('',(#2816),#1194,.F.);
#38620=ADVANCED_FACE('',(#2817),#2041,.F.);
#38621=ADVANCED_FACE('',(#2818),#37457,.T.);
#38622=ADVANCED_FACE('',(#2819),#424,.T.);
#38623=ADVANCED_FACE('',(#2820),#425,.T.);
#38624=ADVANCED_FACE('',(#2821),#1195,.F.);
#38625=ADVANCED_FACE('',(#2822),#37458,.T.);
#38626=ADVANCED_FACE('',(#2823),#2042,.F.);
#38627=ADVANCED_FACE('',(#2824),#426,.T.);
#38628=ADVANCED_FACE('',(#2825),#37459,.T.);
#38629=ADVANCED_FACE('',(#2826),#427,.T.);
#38630=ADVANCED_FACE('',(#2827),#869,.T.);
#38631=ADVANCED_FACE('',(#2828),#609,.T.);
#38632=ADVANCED_FACE('',(#2829),#870,.T.);
#38633=ADVANCED_FACE('',(#2830),#37460,.T.);
#38634=ADVANCED_FACE('',(#2831),#2043,.F.);
#38635=ADVANCED_FACE('',(#2832),#37461,.T.);
#38636=ADVANCED_FACE('',(#2833),#428,.T.);
#38637=ADVANCED_FACE('',(#2834),#429,.T.);
#38638=ADVANCED_FACE('',(#2835),#37462,.T.);
#38639=ADVANCED_FACE('',(#2836),#1196,.F.);
#38640=ADVANCED_FACE('',(#2837),#37463,.T.);
#38641=ADVANCED_FACE('',(#2838),#2044,.F.);
#38642=ADVANCED_FACE('',(#2839),#430,.T.);
#38643=ADVANCED_FACE('',(#2840),#37464,.T.);
#38644=ADVANCED_FACE('',(#2841),#431,.T.);
#38645=ADVANCED_FACE('',(#2842),#871,.T.);
#38646=ADVANCED_FACE('',(#2843),#610,.T.);
#38647=ADVANCED_FACE('',(#2844),#872,.T.);
#38648=ADVANCED_FACE('',(#2845),#37465,.T.);
#38649=ADVANCED_FACE('',(#2846),#37466,.T.);
#38650=ADVANCED_FACE('',(#2847),#2045,.F.);
#38651=ADVANCED_FACE('',(#2848),#432,.T.);
#38652=ADVANCED_FACE('',(#2849),#37467,.T.);
#38653=ADVANCED_FACE('',(#2850),#433,.T.);
#38654=ADVANCED_FACE('',(#2851),#873,.T.);
#38655=ADVANCED_FACE('',(#2852),#611,.T.);
#38656=ADVANCED_FACE('',(#2853),#874,.T.);
#38657=ADVANCED_FACE('',(#2854),#37468,.T.);
#38658=ADVANCED_FACE('',(#2855),#2046,.F.);
#38659=ADVANCED_FACE('',(#2856),#37469,.T.);
#38660=ADVANCED_FACE('',(#2857),#434,.T.);
#38661=ADVANCED_FACE('',(#2858),#435,.T.);
#38662=ADVANCED_FACE('',(#2859),#1197,.F.);
#38663=ADVANCED_FACE('',(#2860),#37470,.T.);
#38664=ADVANCED_FACE('',(#2861),#2047,.F.);
#38665=ADVANCED_FACE('',(#2862),#436,.T.);
#38666=ADVANCED_FACE('',(#2863),#37471,.T.);
#38667=ADVANCED_FACE('',(#2864),#437,.T.);
#38668=ADVANCED_FACE('',(#2865),#875,.T.);
#38669=ADVANCED_FACE('',(#2866),#612,.T.);
#38670=ADVANCED_FACE('',(#2867),#37472,.T.);
#38671=ADVANCED_FACE('',(#2868),#2048,.F.);
#38672=ADVANCED_FACE('',(#2869),#438,.T.);
#38673=ADVANCED_FACE('',(#2870),#37473,.T.);
#38674=ADVANCED_FACE('',(#2871),#439,.T.);
#38675=ADVANCED_FACE('',(#2872),#876,.T.);
#38676=ADVANCED_FACE('',(#2873),#613,.T.);
#38677=ADVANCED_FACE('',(#2874),#877,.T.);
#38678=ADVANCED_FACE('',(#2875),#37474,.T.);
#38679=ADVANCED_FACE('',(#2876),#2049,.F.);
#38680=ADVANCED_FACE('',(#2877),#37475,.T.);
#38681=ADVANCED_FACE('',(#2878),#440,.T.);
#38682=ADVANCED_FACE('',(#2879),#441,.T.);
#38683=ADVANCED_FACE('',(#2880),#37476,.T.);
#38684=ADVANCED_FACE('',(#2881),#2050,.F.);
#38685=ADVANCED_FACE('',(#2882),#442,.T.);
#38686=ADVANCED_FACE('',(#2883),#37477,.T.);
#38687=ADVANCED_FACE('',(#2884),#443,.T.);
#38688=ADVANCED_FACE('',(#2885),#878,.T.);
#38689=ADVANCED_FACE('',(#2886),#614,.T.);
#38690=ADVANCED_FACE('',(#2887),#2051,.F.);
#38691=ADVANCED_FACE('',(#2888),#879,.T.);
#38692=ADVANCED_FACE('',(#2889),#444,.T.);
#38693=ADVANCED_FACE('',(#2890),#37478,.T.);
#38694=ADVANCED_FACE('',(#2891),#445,.T.);
#38695=ADVANCED_FACE('',(#2892),#1198,.F.);
#38696=ADVANCED_FACE('',(#2893),#2052,.F.);
#38697=ADVANCED_FACE('',(#2894),#37479,.T.);
#38698=ADVANCED_FACE('',(#2895),#446,.T.);
#38699=ADVANCED_FACE('',(#2896),#447,.T.);
#38700=ADVANCED_FACE('',(#2897),#1199,.F.);
#38701=ADVANCED_FACE('',(#2898),#2053,.F.);
#38702=ADVANCED_FACE('',(#2899),#880,.T.);
#38703=ADVANCED_FACE('',(#2900),#448,.T.);
#38704=ADVANCED_FACE('',(#2901),#37480,.T.);
#38705=ADVANCED_FACE('',(#2902),#449,.T.);
#38706=ADVANCED_FACE('',(#2903),#1200,.F.);
#38707=ADVANCED_FACE('',(#2904),#37481,.T.);
#38708=ADVANCED_FACE('',(#2905),#1201,.F.);
#38709=ADVANCED_FACE('',(#2906),#2054,.F.);
#38710=ADVANCED_FACE('',(#2907),#37482,.T.);
#38711=ADVANCED_FACE('',(#2908),#450,.T.);
#38712=ADVANCED_FACE('',(#2909),#451,.T.);
#38713=ADVANCED_FACE('',(#2910),#1202,.F.);
#38714=ADVANCED_FACE('',(#2911),#2055,.F.);
#38715=ADVANCED_FACE('',(#2912),#37483,.T.);
#38716=ADVANCED_FACE('',(#2913),#452,.T.);
#38717=ADVANCED_FACE('',(#2914),#453,.T.);
#38718=ADVANCED_FACE('',(#2915),#1203,.F.);
#38719=ADVANCED_FACE('',(#2916),#37484,.T.);
#38720=ADVANCED_FACE('',(#2917),#2056,.F.);
#38721=ADVANCED_FACE('',(#2918),#454,.T.);
#38722=ADVANCED_FACE('',(#2919),#37485,.T.);
#38723=ADVANCED_FACE('',(#2920),#455,.T.);
#38724=ADVANCED_FACE('',(#2921),#881,.T.);
#38725=ADVANCED_FACE('',(#2922),#615,.T.);
#38726=ADVANCED_FACE('',(#2923),#882,.T.);
#38727=ADVANCED_FACE('',(#2924),#37486,.T.);
#38728=ADVANCED_FACE('',(#2925),#2057,.F.);
#38729=ADVANCED_FACE('',(#2926),#37487,.T.);
#38730=ADVANCED_FACE('',(#2927),#456,.T.);
#38731=ADVANCED_FACE('',(#2928),#457,.T.);
#38732=ADVANCED_FACE('',(#2929),#1204,.F.);
#38733=ADVANCED_FACE('',(#2930),#37488,.T.);
#38734=ADVANCED_FACE('',(#2931),#1205,.F.);
#38735=ADVANCED_FACE('',(#2932),#37489,.T.);
#38736=ADVANCED_FACE('',(#2933),#1206,.F.);
#38737=ADVANCED_FACE('',(#2934),#37490,.T.);
#38738=ADVANCED_FACE('',(#2935),#2058,.F.);
#38739=ADVANCED_FACE('',(#2936),#458,.T.);
#38740=ADVANCED_FACE('',(#2937),#37491,.T.);
#38741=ADVANCED_FACE('',(#2938),#459,.T.);
#38742=ADVANCED_FACE('',(#2939),#883,.T.);
#38743=ADVANCED_FACE('',(#2940),#616,.T.);
#38744=ADVANCED_FACE('',(#2941),#884,.T.);
#38745=ADVANCED_FACE('',(#2942),#37492,.T.);
#38746=ADVANCED_FACE('',(#2943),#37493,.T.);
#38747=ADVANCED_FACE('',(#2944),#2059,.F.);
#38748=ADVANCED_FACE('',(#2945),#460,.T.);
#38749=ADVANCED_FACE('',(#2946),#37494,.T.);
#38750=ADVANCED_FACE('',(#2947),#461,.T.);
#38751=ADVANCED_FACE('',(#2948),#885,.T.);
#38752=ADVANCED_FACE('',(#2949),#617,.T.);
#38753=ADVANCED_FACE('',(#2950),#37495,.T.);
#38754=ADVANCED_FACE('',(#2951),#2060,.F.);
#38755=ADVANCED_FACE('',(#2952),#462,.T.);
#38756=ADVANCED_FACE('',(#2953),#37496,.T.);
#38757=ADVANCED_FACE('',(#2954),#463,.T.);
#38758=ADVANCED_FACE('',(#2955),#886,.T.);
#38759=ADVANCED_FACE('',(#2956),#618,.T.);
#38760=ADVANCED_FACE('',(#2957),#887,.T.);
#38761=ADVANCED_FACE('',(#2958),#37497,.T.);
#38762=ADVANCED_FACE('',(#2959),#37498,.T.);
#38763=ADVANCED_FACE('',(#2960),#2061,.F.);
#38764=ADVANCED_FACE('',(#2961),#464,.T.);
#38765=ADVANCED_FACE('',(#2962),#37499,.T.);
#38766=ADVANCED_FACE('',(#2963),#465,.T.);
#38767=ADVANCED_FACE('',(#2964),#888,.T.);
#38768=ADVANCED_FACE('',(#2965),#619,.T.);
#38769=ADVANCED_FACE('',(#2966),#889,.T.);
#38770=ADVANCED_FACE('',(#2967),#37500,.T.);
#38771=ADVANCED_FACE('',(#2968),#37501,.T.);
#38772=ADVANCED_FACE('',(#2969),#2062,.F.);
#38773=ADVANCED_FACE('',(#2970),#466,.T.);
#38774=ADVANCED_FACE('',(#2971),#37502,.T.);
#38775=ADVANCED_FACE('',(#2972),#467,.T.);
#38776=ADVANCED_FACE('',(#2973),#890,.T.);
#38777=ADVANCED_FACE('',(#2974),#620,.T.);
#38778=ADVANCED_FACE('',(#2975),#2063,.F.);
#38779=ADVANCED_FACE('',(#2976),#891,.T.);
#38780=ADVANCED_FACE('',(#2977),#468,.T.);
#38781=ADVANCED_FACE('',(#2978),#37503,.T.);
#38782=ADVANCED_FACE('',(#2979),#469,.T.);
#38783=ADVANCED_FACE('',(#2980),#1207,.F.);
#38784=ADVANCED_FACE('',(#2981),#2064,.F.);
#38785=ADVANCED_FACE('',(#2982),#37504,.T.);
#38786=ADVANCED_FACE('',(#2983),#470,.T.);
#38787=ADVANCED_FACE('',(#2984),#471,.T.);
#38788=ADVANCED_FACE('',(#2985),#1208,.F.);
#38789=ADVANCED_FACE('',(#2986),#2065,.F.);
#38790=ADVANCED_FACE('',(#2987),#37505,.T.);
#38791=ADVANCED_FACE('',(#2988),#472,.T.);
#38792=ADVANCED_FACE('',(#2989),#473,.T.);
#38793=ADVANCED_FACE('',(#2990),#1209,.F.);
#38794=ADVANCED_FACE('',(#2991),#2066,.F.);
#38795=ADVANCED_FACE('',(#2992),#892,.T.);
#38796=ADVANCED_FACE('',(#2993),#474,.T.);
#38797=ADVANCED_FACE('',(#2994),#37506,.T.);
#38798=ADVANCED_FACE('',(#2995),#475,.T.);
#38799=ADVANCED_FACE('',(#2996),#1210,.F.);
#38800=ADVANCED_FACE('',(#2997),#37507,.T.);
#38801=ADVANCED_FACE('',(#2998),#621,.T.);
#38802=ADVANCED_FACE('',(#2999),#1211,.F.);
#38803=ADVANCED_FACE('',(#3000),#2067,.F.);
#38804=ADVANCED_FACE('',(#3001),#37508,.T.);
#38805=ADVANCED_FACE('',(#3002),#476,.T.);
#38806=ADVANCED_FACE('',(#3003),#477,.T.);
#38807=ADVANCED_FACE('',(#3004),#1212,.F.);
#38808=ADVANCED_FACE('',(#3005),#37509,.T.);
#38809=ADVANCED_FACE('',(#3006),#2068,.F.);
#38810=ADVANCED_FACE('',(#3007),#478,.T.);
#38811=ADVANCED_FACE('',(#3008),#37510,.T.);
#38812=ADVANCED_FACE('',(#3009),#479,.T.);
#38813=ADVANCED_FACE('',(#3010),#893,.T.);
#38814=ADVANCED_FACE('',(#3011),#622,.T.);
#38815=ADVANCED_FACE('',(#3012),#2069,.F.);
#38816=ADVANCED_FACE('',(#3013),#37511,.T.);
#38817=ADVANCED_FACE('',(#3014),#480,.T.);
#38818=ADVANCED_FACE('',(#3015),#481,.T.);
#38819=ADVANCED_FACE('',(#3016),#2070,.F.);
#38820=ADVANCED_FACE('',(#3017),#894,.T.);
#38821=ADVANCED_FACE('',(#3018),#482,.T.);
#38822=ADVANCED_FACE('',(#3019),#37512,.T.);
#38823=ADVANCED_FACE('',(#3020),#483,.T.);
#38824=ADVANCED_FACE('',(#3021),#1213,.F.);
#38825=ADVANCED_FACE('',(#3022),#37513,.T.);
#38826=ADVANCED_FACE('',(#3023),#1214,.F.);
#38827=ADVANCED_FACE('',(#3024),#895,.T.);
#38828=ADVANCED_FACE('',(#3025),#37514,.T.);
#38829=ADVANCED_FACE('',(#3026),#484,.T.);
#38830=ADVANCED_FACE('',(#3027),#2071,.F.);
#38831=ADVANCED_FACE('',(#3028),#1215,.F.);
#38832=ADVANCED_FACE('',(#3029),#896,.T.);
#38833=ADVANCED_FACE('',(#3030),#37515,.T.);
#38834=ADVANCED_FACE('',(#3031),#1216,.F.);
#38835=ADVANCED_FACE('',(#3032),#1217,.F.);
#38836=ADVANCED_FACE('',(#3033),#37516,.T.);
#38837=ADVANCED_FACE('',(#3034),#1218,.F.);
#38838=ADVANCED_FACE('',(#3035),#897,.T.);
#38839=ADVANCED_FACE('',(#3036),#37517,.T.);
#38840=ADVANCED_FACE('',(#3037),#1219,.F.);
#38841=ADVANCED_FACE('',(#3038),#898,.T.);
#38842=ADVANCED_FACE('',(#3039),#37518,.T.);
#38843=ADVANCED_FACE('',(#3040),#1220,.F.);
#38844=ADVANCED_FACE('',(#3041),#1221,.F.);
#38845=ADVANCED_FACE('',(#3042),#899,.T.);
#38846=ADVANCED_FACE('',(#3043),#37519,.T.);
#38847=ADVANCED_FACE('',(#3044),#1222,.F.);
#38848=ADVANCED_FACE('',(#3045),#37520,.T.);
#38849=ADVANCED_FACE('',(#3046),#1223,.F.);
#38850=ADVANCED_FACE('',(#3047),#900,.T.);
#38851=ADVANCED_FACE('',(#3048),#37521,.T.);
#38852=ADVANCED_FACE('',(#3049),#1224,.F.);
#38853=ADVANCED_FACE('',(#3050),#1225,.F.);
#38854=ADVANCED_FACE('',(#3051),#901,.T.);
#38855=ADVANCED_FACE('',(#3052),#37522,.T.);
#38856=ADVANCED_FACE('',(#3053),#1226,.F.);
#38857=ADVANCED_FACE('',(#3054),#902,.T.);
#38858=ADVANCED_FACE('',(#3055),#37523,.T.);
#38859=ADVANCED_FACE('',(#3056),#1227,.F.);
#38860=ADVANCED_FACE('',(#3057),#2072,.F.);
#38861=ADVANCED_FACE('',(#3058),#485,.T.);
#38862=ADVANCED_FACE('',(#3059),#37524,.T.);
#38863=ADVANCED_FACE('',(#3060),#486,.T.);
#38864=ADVANCED_FACE('',(#3061),#37525,.T.);
#38865=ADVANCED_FACE('',(#3062),#1228,.F.);
#38866=ADVANCED_FACE('',(#3063),#1229,.F.);
#38867=ADVANCED_FACE('',(#3064),#903,.T.);
#38868=ADVANCED_FACE('',(#3065),#37526,.T.);
#38869=ADVANCED_FACE('',(#3066),#1230,.F.);
#38870=ADVANCED_FACE('',(#3067),#904,.T.);
#38871=ADVANCED_FACE('',(#3068),#37527,.T.);
#38872=ADVANCED_FACE('',(#3069),#1231,.F.);
#38873=ADVANCED_FACE('',(#3070),#1232,.F.);
#38874=ADVANCED_FACE('',(#3071),#37528,.T.);
#38875=ADVANCED_FACE('',(#3072),#1233,.F.);
#38876=ADVANCED_FACE('',(#3073),#905,.T.);
#38877=ADVANCED_FACE('',(#3074),#37529,.T.);
#38878=ADVANCED_FACE('',(#3075),#1234,.F.);
#38879=ADVANCED_FACE('',(#3076),#906,.T.);
#38880=ADVANCED_FACE('',(#3077),#37530,.T.);
#38881=ADVANCED_FACE('',(#3078),#1235,.F.);
#38882=ADVANCED_FACE('',(#3079),#1236,.F.);
#38883=ADVANCED_FACE('',(#3080),#907,.T.);
#38884=ADVANCED_FACE('',(#3081),#37531,.T.);
#38885=ADVANCED_FACE('',(#3082),#1237,.F.);
#38886=ADVANCED_FACE('',(#3083),#37532,.T.);
#38887=ADVANCED_FACE('',(#3084),#1238,.F.);
#38888=ADVANCED_FACE('',(#3085),#908,.T.);
#38889=ADVANCED_FACE('',(#3086),#37533,.T.);
#38890=ADVANCED_FACE('',(#3087),#1239,.F.);
#38891=ADVANCED_FACE('',(#3088),#1240,.F.);
#38892=ADVANCED_FACE('',(#3089),#909,.T.);
#38893=ADVANCED_FACE('',(#3090),#37534,.T.);
#38894=ADVANCED_FACE('',(#3091),#1241,.F.);
#38895=ADVANCED_FACE('',(#3092),#910,.T.);
#38896=ADVANCED_FACE('',(#3093),#37535,.T.);
#38897=ADVANCED_FACE('',(#3094),#1242,.F.);
#38898=ADVANCED_FACE('',(#3095),#2073,.F.);
#38899=ADVANCED_FACE('',(#3096),#487,.T.);
#38900=ADVANCED_FACE('',(#3097),#37536,.T.);
#38901=ADVANCED_FACE('',(#3098),#488,.T.);
#38902=ADVANCED_FACE('',(#3099),#37537,.T.);
#38903=ADVANCED_FACE('',(#3100),#1243,.F.);
#38904=ADVANCED_FACE('',(#3101),#1244,.F.);
#38905=ADVANCED_FACE('',(#3102),#911,.T.);
#38906=ADVANCED_FACE('',(#3103),#37538,.T.);
#38907=ADVANCED_FACE('',(#3104),#1245,.F.);
#38908=ADVANCED_FACE('',(#3105),#912,.T.);
#38909=ADVANCED_FACE('',(#3106),#37539,.T.);
#38910=ADVANCED_FACE('',(#3107),#1246,.F.);
#38911=ADVANCED_FACE('',(#3108),#1247,.F.);
#38912=ADVANCED_FACE('',(#3109),#37540,.T.);
#38913=ADVANCED_FACE('',(#3110),#1248,.F.);
#38914=ADVANCED_FACE('',(#3111),#913,.T.);
#38915=ADVANCED_FACE('',(#3112),#37541,.T.);
#38916=ADVANCED_FACE('',(#3113),#1249,.F.);
#38917=ADVANCED_FACE('',(#3114),#914,.T.);
#38918=ADVANCED_FACE('',(#3115),#37542,.T.);
#38919=ADVANCED_FACE('',(#3116),#1250,.F.);
#38920=ADVANCED_FACE('',(#3117),#1251,.F.);
#38921=ADVANCED_FACE('',(#3118),#915,.T.);
#38922=ADVANCED_FACE('',(#3119),#37543,.T.);
#38923=ADVANCED_FACE('',(#3120),#1252,.F.);
#38924=ADVANCED_FACE('',(#3121),#37544,.T.);
#38925=ADVANCED_FACE('',(#3122),#1253,.F.);
#38926=ADVANCED_FACE('',(#3123),#916,.T.);
#38927=ADVANCED_FACE('',(#3124),#37545,.T.);
#38928=ADVANCED_FACE('',(#3125),#1254,.F.);
#38929=ADVANCED_FACE('',(#3126),#1255,.F.);
#38930=ADVANCED_FACE('',(#3127),#917,.T.);
#38931=ADVANCED_FACE('',(#3128),#37546,.T.);
#38932=ADVANCED_FACE('',(#3129),#1256,.F.);
#38933=ADVANCED_FACE('',(#3130),#918,.T.);
#38934=ADVANCED_FACE('',(#3131),#37547,.T.);
#38935=ADVANCED_FACE('',(#3132),#1257,.F.);
#38936=ADVANCED_FACE('',(#3133),#2074,.F.);
#38937=ADVANCED_FACE('',(#3134),#489,.T.);
#38938=ADVANCED_FACE('',(#3135),#37548,.T.);
#38939=ADVANCED_FACE('',(#3136),#490,.T.);
#38940=ADVANCED_FACE('',(#3137),#37549,.T.);
#38941=ADVANCED_FACE('',(#3138),#1258,.F.);
#38942=ADVANCED_FACE('',(#3139),#1259,.F.);
#38943=ADVANCED_FACE('',(#3140),#919,.T.);
#38944=ADVANCED_FACE('',(#3141),#37550,.T.);
#38945=ADVANCED_FACE('',(#3142),#1260,.F.);
#38946=ADVANCED_FACE('',(#3143),#920,.T.);
#38947=ADVANCED_FACE('',(#3144),#37551,.T.);
#38948=ADVANCED_FACE('',(#3145),#1261,.F.);
#38949=ADVANCED_FACE('',(#3146),#2075,.F.);
#38950=ADVANCED_FACE('',(#3147),#921,.T.);
#38951=ADVANCED_FACE('',(#3148),#491,.T.);
#38952=ADVANCED_FACE('',(#3149),#37552,.T.);
#38953=ADVANCED_FACE('',(#3150),#37553,.T.);
#38954=ADVANCED_FACE('',(#3151),#492,.T.);
#38955=ADVANCED_FACE('',(#3152),#1262,.F.);
#38956=ADVANCED_FACE('',(#3153),#1263,.F.);
#38957=ADVANCED_FACE('',(#3154),#922,.T.);
#38958=ADVANCED_FACE('',(#3155),#37554,.T.);
#38959=ADVANCED_FACE('',(#3156),#1264,.F.);
#38960=ADVANCED_FACE('',(#3157),#923,.T.);
#38961=ADVANCED_FACE('',(#3158),#37555,.T.);
#38962=ADVANCED_FACE('',(#3159),#1265,.F.);
#38963=ADVANCED_FACE('',(#3160),#1266,.F.);
#38964=ADVANCED_FACE('',(#3161),#924,.T.);
#38965=ADVANCED_FACE('',(#3162),#37556,.T.);
#38966=ADVANCED_FACE('',(#3163),#1267,.F.);
#38967=ADVANCED_FACE('',(#3164),#37557,.T.);
#38968=ADVANCED_FACE('',(#3165),#1268,.F.);
#38969=ADVANCED_FACE('',(#3166),#925,.T.);
#38970=ADVANCED_FACE('',(#3167),#37558,.T.);
#38971=ADVANCED_FACE('',(#3168),#1269,.F.);
#38972=ADVANCED_FACE('',(#3169),#1270,.F.);
#38973=ADVANCED_FACE('',(#3170),#37559,.T.);
#38974=ADVANCED_FACE('',(#3171),#2076,.F.);
#38975=ADVANCED_FACE('',(#3172),#493,.T.);
#38976=ADVANCED_FACE('',(#3173),#37560,.T.);
#38977=ADVANCED_FACE('',(#3174),#926,.T.);
#38978=ADVANCED_FACE('',(#3175),#494,.T.);
#38979=ADVANCED_FACE('',(#3176),#495,.T.);
#38980=ADVANCED_FACE('',(#3177),#927,.T.);
#38981=ADVANCED_FACE('',(#3178),#623,.T.);
#38982=ADVANCED_FACE('',(#3179),#928,.T.);
#38983=ADVANCED_FACE('',(#3180),#37561,.T.);
#38984=ADVANCED_FACE('',(#3181),#37562,.T.);
#38985=ADVANCED_FACE('',(#3182),#37563,.T.);
#38986=ADVANCED_FACE('',(#3183),#37564,.T.);
#38987=ADVANCED_FACE('',(#3184),#2077,.F.);
#38988=ADVANCED_FACE('',(#3185),#496,.T.);
#38989=ADVANCED_FACE('',(#3186),#929,.T.);
#38990=ADVANCED_FACE('',(#3187),#37565,.T.);
#38991=ADVANCED_FACE('',(#3188),#497,.T.);
#38992=ADVANCED_FACE('',(#3189),#2078,.F.);
#38993=ADVANCED_FACE('',(#3190),#498,.T.);
#38994=ADVANCED_FACE('',(#3191),#499,.T.);
#38995=ADVANCED_FACE('',(#3192),#37566,.T.);
#38996=ADVANCED_FACE('',(#3193),#37567,.T.);
#38997=ADVANCED_FACE('',(#3194),#1271,.F.);
#38998=ADVANCED_FACE('',(#3195),#930,.T.);
#38999=ADVANCED_FACE('',(#3196),#624,.T.);
#39000=ADVANCED_FACE('',(#3197),#931,.T.);
#39001=ADVANCED_FACE('',(#3198),#2079,.F.);
#39002=ADVANCED_FACE('',(#3199),#932,.T.);
#39003=ADVANCED_FACE('',(#3200),#500,.T.);
#39004=ADVANCED_FACE('',(#3201),#625,.T.);
#39005=ADVANCED_FACE('',(#3202),#1272,.F.);
#39006=ADVANCED_FACE('',(#3203),#2080,.F.);
#39007=ADVANCED_FACE('',(#3204),#37568,.T.);
#39008=ADVANCED_FACE('',(#3205),#501,.T.);
#39009=ADVANCED_FACE('',(#3206),#502,.T.);
#39010=ADVANCED_FACE('',(#3207),#933,.T.);
#39011=ADVANCED_FACE('',(#3208),#37569,.F.);
#39012=ADVANCED_FACE('',(#3209),#934,.T.);
#39013=ADVANCED_FACE('',(#3210),#2081,.F.);
#39014=ADVANCED_FACE('',(#3211),#935,.T.);
#39015=ADVANCED_FACE('',(#3212),#503,.T.);
#39016=ADVANCED_FACE('',(#3213),#936,.T.);
#39017=ADVANCED_FACE('',(#3214),#2082,.F.);
#39018=ADVANCED_FACE('',(#3215),#937,.T.);
#39019=ADVANCED_FACE('',(#3216),#504,.T.);
#39020=ADVANCED_FACE('',(#3217),#626,.T.);
#39021=ADVANCED_FACE('',(#3218),#37570,.T.);
#39022=ADVANCED_FACE('',(#3219),#1273,.F.);
#39023=ADVANCED_FACE('',(#3220),#627,.T.);
#39024=ADVANCED_FACE('',(#3221),#37571,.T.);
#39025=ADVANCED_FACE('',(#3222),#1274,.F.);
#39026=ADVANCED_FACE('',(#3223),#938,.T.);
#39027=ADVANCED_FACE('',(#3224),#37572,.T.);
#39028=ADVANCED_FACE('',(#3225),#1275,.F.);
#39029=ADVANCED_FACE('',(#3226),#37573,.T.);
#39030=ADVANCED_FACE('',(#3227),#37574,.T.);
#39031=ADVANCED_FACE('',(#3228),#37575,.T.);
#39032=ADVANCED_FACE('',(#3229),#37576,.T.);
#39033=ADVANCED_FACE('',(#3230),#37577,.T.);
#39034=ADVANCED_FACE('',(#3231),#1276,.F.);
#39035=ADVANCED_FACE('',(#3232),#37578,.T.);
#39036=ADVANCED_FACE('',(#3233),#939,.T.);
#39037=ADVANCED_FACE('',(#3234),#37579,.T.);
#39038=ADVANCED_FACE('',(#3235),#37580,.T.);
#39039=ADVANCED_FACE('',(#3236),#1277,.F.);
#39040=ADVANCED_FACE('',(#3237),#37581,.T.);
#39041=ADVANCED_FACE('',(#3238),#37582,.T.);
#39042=ADVANCED_FACE('',(#3239),#1278,.F.);
#39043=ADVANCED_FACE('',(#3240),#37583,.T.);
#39044=ADVANCED_FACE('',(#3241),#940,.T.);
#39045=ADVANCED_FACE('',(#3242),#37584,.T.);
#39046=ADVANCED_FACE('',(#3243),#37585,.T.);
#39047=ADVANCED_FACE('',(#3244),#37586,.T.);
#39048=ADVANCED_FACE('',(#3245),#37587,.T.);
#39049=ADVANCED_FACE('',(#3246),#1279,.F.);
#39050=ADVANCED_FACE('',(#3247),#37588,.T.);
#39051=ADVANCED_FACE('',(#3248),#941,.T.);
#39052=ADVANCED_FACE('',(#3249),#37589,.T.);
#39053=ADVANCED_FACE('',(#3250),#1280,.F.);
#39054=ADVANCED_FACE('',(#3251),#37590,.T.);
#39055=ADVANCED_FACE('',(#3252),#37591,.T.);
#39056=ADVANCED_FACE('',(#3253),#37592,.T.);
#39057=ADVANCED_FACE('',(#3254),#1281,.F.);
#39058=ADVANCED_FACE('',(#3255),#37593,.T.);
#39059=ADVANCED_FACE('',(#3256),#942,.T.);
#39060=ADVANCED_FACE('',(#3257),#37594,.T.);
#39061=ADVANCED_FACE('',(#3258),#37595,.T.);
#39062=ADVANCED_FACE('',(#3259),#37596,.T.);
#39063=ADVANCED_FACE('',(#3260),#37597,.T.);
#39064=ADVANCED_FACE('',(#3261),#1282,.F.);
#39065=ADVANCED_FACE('',(#3262),#37598,.T.);
#39066=ADVANCED_FACE('',(#3263),#943,.T.);
#39067=ADVANCED_FACE('',(#3264),#37599,.T.);
#39068=ADVANCED_FACE('',(#3265),#37600,.T.);
#39069=ADVANCED_FACE('',(#3266),#37601,.T.);
#39070=ADVANCED_FACE('',(#3267),#37602,.T.);
#39071=ADVANCED_FACE('',(#3268),#1283,.F.);
#39072=ADVANCED_FACE('',(#3269),#37603,.T.);
#39073=ADVANCED_FACE('',(#3270),#944,.T.);
#39074=ADVANCED_FACE('',(#3271),#37604,.T.);
#39075=ADVANCED_FACE('',(#3272),#37605,.T.);
#39076=ADVANCED_FACE('',(#3273),#37606,.T.);
#39077=ADVANCED_FACE('',(#3274),#37607,.T.);
#39078=ADVANCED_FACE('',(#3275),#1284,.F.);
#39079=ADVANCED_FACE('',(#3276),#37608,.T.);
#39080=ADVANCED_FACE('',(#3277),#945,.T.);
#39081=ADVANCED_FACE('',(#3278),#37609,.T.);
#39082=ADVANCED_FACE('',(#3279),#1285,.F.);
#39083=ADVANCED_FACE('',(#3280),#37610,.T.);
#39084=ADVANCED_FACE('',(#3281),#37611,.T.);
#39085=ADVANCED_FACE('',(#3282),#37612,.T.);
#39086=ADVANCED_FACE('',(#3283),#1286,.F.);
#39087=ADVANCED_FACE('',(#3284),#37613,.T.);
#39088=ADVANCED_FACE('',(#3285),#946,.T.);
#39089=ADVANCED_FACE('',(#3286),#37614,.T.);
#39090=ADVANCED_FACE('',(#3287),#37615,.T.);
#39091=ADVANCED_FACE('',(#3288),#37616,.T.);
#39092=ADVANCED_FACE('',(#3289),#37617,.T.);
#39093=ADVANCED_FACE('',(#3290),#1287,.F.);
#39094=ADVANCED_FACE('',(#3291),#37618,.T.);
#39095=ADVANCED_FACE('',(#3292),#947,.T.);
#39096=ADVANCED_FACE('',(#3293),#37619,.T.);
#39097=ADVANCED_FACE('',(#3294),#37620,.T.);
#39098=ADVANCED_FACE('',(#3295),#1288,.F.);
#39099=ADVANCED_FACE('',(#3296),#37621,.T.);
#39100=ADVANCED_FACE('',(#3297),#37622,.T.);
#39101=ADVANCED_FACE('',(#3298),#1289,.F.);
#39102=ADVANCED_FACE('',(#3299),#37623,.T.);
#39103=ADVANCED_FACE('',(#3300),#948,.T.);
#39104=ADVANCED_FACE('',(#3301),#37624,.T.);
#39105=ADVANCED_FACE('',(#3302),#1290,.F.);
#39106=ADVANCED_FACE('',(#3303),#37625,.T.);
#39107=ADVANCED_FACE('',(#3304),#37626,.T.);
#39108=ADVANCED_FACE('',(#3305),#37627,.T.);
#39109=ADVANCED_FACE('',(#3306),#1291,.F.);
#39110=ADVANCED_FACE('',(#3307),#37628,.T.);
#39111=ADVANCED_FACE('',(#3308),#949,.T.);
#39112=ADVANCED_FACE('',(#3309),#37629,.T.);
#39113=ADVANCED_FACE('',(#3310),#37630,.T.);
#39114=ADVANCED_FACE('',(#3311),#37631,.T.);
#39115=ADVANCED_FACE('',(#3312),#37632,.T.);
#39116=ADVANCED_FACE('',(#3313),#1292,.F.);
#39117=ADVANCED_FACE('',(#3314),#37633,.T.);
#39118=ADVANCED_FACE('',(#3315),#950,.T.);
#39119=ADVANCED_FACE('',(#3316),#37634,.T.);
#39120=ADVANCED_FACE('',(#3317),#37635,.T.);
#39121=ADVANCED_FACE('',(#3318),#37636,.T.);
#39122=ADVANCED_FACE('',(#3319),#37637,.T.);
#39123=ADVANCED_FACE('',(#3320),#1293,.F.);
#39124=ADVANCED_FACE('',(#3321),#37638,.T.);
#39125=ADVANCED_FACE('',(#3322),#951,.T.);
#39126=ADVANCED_FACE('',(#3323),#37639,.T.);
#39127=ADVANCED_FACE('',(#3324),#37640,.T.);
#39128=ADVANCED_FACE('',(#3325),#1294,.F.);
#39129=ADVANCED_FACE('',(#3326),#37641,.T.);
#39130=ADVANCED_FACE('',(#3327),#37642,.T.);
#39131=ADVANCED_FACE('',(#3328),#1295,.F.);
#39132=ADVANCED_FACE('',(#3329),#37643,.T.);
#39133=ADVANCED_FACE('',(#3330),#952,.T.);
#39134=ADVANCED_FACE('',(#3331),#37644,.T.);
#39135=ADVANCED_FACE('',(#3332),#37645,.T.);
#39136=ADVANCED_FACE('',(#3333),#37646,.T.);
#39137=ADVANCED_FACE('',(#3334),#37647,.T.);
#39138=ADVANCED_FACE('',(#3335),#1296,.F.);
#39139=ADVANCED_FACE('',(#3336),#37648,.T.);
#39140=ADVANCED_FACE('',(#3337),#953,.T.);
#39141=ADVANCED_FACE('',(#3338),#37649,.T.);
#39142=ADVANCED_FACE('',(#3339),#954,.T.);
#39143=ADVANCED_FACE('',(#3340),#1297,.F.);
#39144=ADVANCED_FACE('',(#3341),#37650,.T.);
#39145=ADVANCED_FACE('',(#3342),#1298,.F.);
#39146=ADVANCED_FACE('',(#3343),#37651,.T.);
#39147=ADVANCED_FACE('',(#3344),#37652,.T.);
#39148=ADVANCED_FACE('',(#3345),#628,.T.);
#39149=ADVANCED_FACE('',(#3346),#37653,.T.);
#39150=ADVANCED_FACE('',(#3347),#629,.T.);
#39151=ADVANCED_FACE('',(#3348),#37654,.T.);
#39152=ADVANCED_FACE('',(#3349),#630,.T.);
#39153=ADVANCED_FACE('',(#3350),#631,.T.);
#39154=ADVANCED_FACE('',(#3351),#632,.T.);
#39155=ADVANCED_FACE('',(#3352),#37655,.T.);
#39156=ADVANCED_FACE('',(#3353),#633,.T.);
#39157=ADVANCED_FACE('',(#3354),#634,.T.);
#39158=ADVANCED_FACE('',(#3355),#635,.T.);
#39159=ADVANCED_FACE('',(#3356),#37656,.T.);
#39160=ADVANCED_FACE('',(#3357),#636,.T.);
#39161=ADVANCED_FACE('',(#3358),#637,.T.);
#39162=ADVANCED_FACE('',(#3359),#638,.T.);
#39163=ADVANCED_FACE('',(#3360),#639,.T.);
#39164=ADVANCED_FACE('',(#3361),#640,.T.);
#39165=ADVANCED_FACE('',(#3362),#641,.T.);
#39166=ADVANCED_FACE('',(#3363),#37657,.T.);
#39167=ADVANCED_FACE('',(#3364),#642,.T.);
#39168=ADVANCED_FACE('',(#3365),#643,.T.);
#39169=ADVANCED_FACE('',(#3366),#644,.T.);
#39170=ADVANCED_FACE('',(#3367),#37658,.T.);
#39171=ADVANCED_FACE('',(#3368),#645,.T.);
#39172=ADVANCED_FACE('',(#3369),#646,.T.);
#39173=ADVANCED_FACE('',(#3370),#647,.T.);
#39174=ADVANCED_FACE('',(#3371),#37659,.T.);
#39175=ADVANCED_FACE('',(#3372),#648,.T.);
#39176=ADVANCED_FACE('',(#3373),#649,.T.);
#39177=ADVANCED_FACE('',(#3374),#650,.T.);
#39178=ADVANCED_FACE('',(#3375),#651,.T.);
#39179=ADVANCED_FACE('',(#3376),#652,.T.);
#39180=ADVANCED_FACE('',(#3377),#653,.T.);
#39181=ADVANCED_FACE('',(#3378),#37660,.T.);
#39182=ADVANCED_FACE('',(#3379),#654,.T.);
#39183=ADVANCED_FACE('',(#3380),#655,.T.);
#39184=ADVANCED_FACE('',(#3381),#656,.T.);
#39185=ADVANCED_FACE('',(#3382),#37661,.T.);
#39186=ADVANCED_FACE('',(#3383),#657,.T.);
#39187=ADVANCED_FACE('',(#3384),#658,.T.);
#39188=ADVANCED_FACE('',(#3385),#659,.T.);
#39189=ADVANCED_FACE('',(#3386),#37662,.T.);
#39190=ADVANCED_FACE('',(#3387),#660,.T.);
#39191=ADVANCED_FACE('',(#3388),#661,.T.);
#39192=ADVANCED_FACE('',(#3389),#662,.T.);
#39193=ADVANCED_FACE('',(#3390),#663,.T.);
#39194=ADVANCED_FACE('',(#3391),#664,.T.);
#39195=ADVANCED_FACE('',(#3392),#665,.T.);
#39196=ADVANCED_FACE('',(#3393),#37663,.T.);
#39197=ADVANCED_FACE('',(#3394),#666,.T.);
#39198=ADVANCED_FACE('',(#3395),#667,.T.);
#39199=ADVANCED_FACE('',(#3396),#668,.T.);
#39200=ADVANCED_FACE('',(#3397),#37664,.T.);
#39201=ADVANCED_FACE('',(#3398),#669,.T.);
#39202=ADVANCED_FACE('',(#3399),#670,.T.);
#39203=ADVANCED_FACE('',(#3400),#671,.T.);
#39204=ADVANCED_FACE('',(#3401),#37665,.T.);
#39205=ADVANCED_FACE('',(#3402),#1299,.F.);
#39206=ADVANCED_FACE('',(#3403),#1300,.F.);
#39207=ADVANCED_FACE('',(#3404),#672,.T.);
#39208=ADVANCED_FACE('',(#3405),#1301,.F.);
#40346=CLOSED_SHELL('',(#38166,#38167,#38168,#38169,#38170,#38171,#38172,
#38173,#38174,#38175,#38176,#38177,#38178,#38179,#38180,#38181,#38182,#38183,
#38184,#38185,#38186,#38187,#38188,#38189,#38190,#38191,#38192,#38193,#38194,
#38195,#38196,#38197,#38198,#38199,#38200,#38201,#38202,#38203,#38204,#38205,
#38206,#38207,#38208,#38209,#38210,#38211,#38212,#38213,#38214,#38215,#38216,
#38217,#38218,#38219,#38220,#38221,#38222,#38223,#38224,#38225,#38226,#38227,
#38228,#38229,#38230,#38231,#38232,#38233,#38234,#38235,#38236,#38237,#38238,
#38239,#38240,#38241,#38242,#38243,#38244,#38245,#38246,#38247,#38248,#38249,
#38250,#38251,#38252,#38253,#38254,#38255,#38256,#38257,#38258,#38259,#38260,
#38261,#38262,#38263,#38264,#38265,#38266,#38267,#38268,#38269,#38270,#38271,
#38272,#38273,#38274,#38275,#38276,#38277,#38278,#38279,#38280,#38281,#38282,
#38283,#38284,#38285,#38286,#38287,#38288,#38289,#38290,#38291,#38292,#38293,
#38294,#38295,#38296,#38297,#38298,#38299,#38300,#38301,#38302,#38303,#38304,
#38305,#38306,#38307,#38308,#38309,#38310,#38311,#38312,#38313,#38314,#38315,
#38316,#38317,#38318,#38319,#38320,#38321,#38322,#38323,#38324,#38325,#38326,
#38327,#38328,#38329,#38330,#38331,#38332,#38333,#38334,#38335,#38336,#38337,
#38338,#38339,#38340,#38341,#38342,#38343,#38344,#38345,#38346,#38347,#38348,
#38349,#38350,#38351,#38352,#38353,#38354,#38355,#38356,#38357,#38358,#38359,
#38360,#38361,#38362,#38363,#38364,#38365,#38366,#38367,#38368,#38369,#38370,
#38371,#38372,#38373,#38374,#38375,#38376,#38377,#38378,#38379,#38380,#38381,
#38382,#38383,#38384,#38385,#38386,#38387,#38388,#38389,#38390,#38391,#38392,
#38393,#38394,#38395,#38396,#38397,#38398,#38399,#38400,#38401,#38402,#38403,
#38404,#38405,#38406,#38407,#38408,#38409,#38410,#38411,#38412,#38413,#38414,
#38415,#38416,#38417,#38418,#38419,#38420,#38421,#38422,#38423,#38424,#38425,
#38426,#38427,#38428,#38429,#38430,#38431,#38432,#38433,#38434,#38435,#38436,
#38437,#38438,#38439,#38440,#38441,#38442,#38443,#38444,#38445,#38446,#38447,
#38448,#38449,#38450,#38451,#38452,#38453,#38454,#38455,#38456,#38457,#38458,
#38459,#38460,#38461,#38462,#38463,#38464,#38465,#38466,#38467,#38468,#38469,
#38470,#38471,#38472,#38473,#38474,#38475,#38476,#38477,#38478,#38479,#38480,
#38481,#38482,#38483,#38484,#38485,#38486,#38487,#38488,#38489,#38490,#38491,
#38492,#38493,#38494,#38495,#38496,#38497,#38498,#38499,#38500,#38501,#38502,
#38503,#38504,#38505,#38506,#38507,#38508,#38509,#38510,#38511,#38512,#38513,
#38514,#38515,#38516,#38517,#38518,#38519,#38520,#38521,#38522,#38523,#38524,
#38525,#38526,#38527,#38528,#38529,#38530,#38531,#38532,#38533,#38534,#38535,
#38536,#38537,#38538,#38539,#38540,#38541,#38542,#38543,#38544,#38545,#38546,
#38547,#38548,#38549,#38550,#38551,#38552,#38553,#38554,#38555,#38556,#38557,
#38558,#38559,#38560,#38561,#38562,#38563,#38564,#38565,#38566,#38567,#38568,
#38569,#38570,#38571,#38572,#38573,#38574,#38575,#38576,#38577,#38578,#38579,
#38580,#38581,#38582,#38583,#38584,#38585,#38586,#38587,#38588,#38589,#38590,
#38591,#38592,#38593,#38594,#38595,#38596,#38597,#38598,#38599,#38600,#38601,
#38602,#38603,#38604,#38605,#38606,#38607,#38608,#38609,#38610,#38611,#38612,
#38613,#38614,#38615,#38616,#38617,#38618,#38619,#38620,#38621,#38622,#38623,
#38624,#38625,#38626,#38627,#38628,#38629,#38630,#38631,#38632,#38633,#38634,
#38635,#38636,#38637,#38638,#38639,#38640,#38641,#38642,#38643,#38644,#38645,
#38646,#38647,#38648,#38649,#38650,#38651,#38652,#38653,#38654,#38655,#38656,
#38657,#38658,#38659,#38660,#38661,#38662,#38663,#38664,#38665,#38666,#38667,
#38668,#38669,#38670,#38671,#38672,#38673,#38674,#38675,#38676,#38677,#38678,
#38679,#38680,#38681,#38682,#38683,#38684,#38685,#38686,#38687,#38688,#38689,
#38690,#38691,#38692,#38693,#38694,#38695,#38696,#38697,#38698,#38699,#38700,
#38701,#38702,#38703,#38704,#38705,#38706,#38707,#38708,#38709,#38710,#38711,
#38712,#38713,#38714,#38715,#38716,#38717,#38718,#38719,#38720,#38721,#38722,
#38723,#38724,#38725,#38726,#38727,#38728,#38729,#38730,#38731,#38732,#38733,
#38734,#38735,#38736,#38737,#38738,#38739,#38740,#38741,#38742,#38743,#38744,
#38745,#38746,#38747,#38748,#38749,#38750,#38751,#38752,#38753,#38754,#38755,
#38756,#38757,#38758,#38759,#38760,#38761,#38762,#38763,#38764,#38765,#38766,
#38767,#38768,#38769,#38770,#38771,#38772,#38773,#38774,#38775,#38776,#38777,
#38778,#38779,#38780,#38781,#38782,#38783,#38784,#38785,#38786,#38787,#38788,
#38789,#38790,#38791,#38792,#38793,#38794,#38795,#38796,#38797,#38798,#38799,
#38800,#38801,#38802,#38803,#38804,#38805,#38806,#38807,#38808,#38809,#38810,
#38811,#38812,#38813,#38814,#38815,#38816,#38817,#38818,#38819,#38820,#38821,
#38822,#38823,#38824,#38825,#38826,#38827,#38828,#38829,#38830,#38831,#38832,
#38833,#38834,#38835,#38836,#38837,#38838,#38839,#38840,#38841,#38842,#38843,
#38844,#38845,#38846,#38847,#38848,#38849,#38850,#38851,#38852,#38853,#38854,
#38855,#38856,#38857,#38858,#38859,#38860,#38861,#38862,#38863,#38864,#38865,
#38866,#38867,#38868,#38869,#38870,#38871,#38872,#38873,#38874,#38875,#38876,
#38877,#38878,#38879,#38880,#38881,#38882,#38883,#38884,#38885,#38886,#38887,
#38888,#38889,#38890,#38891,#38892,#38893,#38894,#38895,#38896,#38897,#38898,
#38899,#38900,#38901,#38902,#38903,#38904,#38905,#38906,#38907,#38908,#38909,
#38910,#38911,#38912,#38913,#38914,#38915,#38916,#38917,#38918,#38919,#38920,
#38921,#38922,#38923,#38924,#38925,#38926,#38927,#38928,#38929,#38930,#38931,
#38932,#38933,#38934,#38935,#38936,#38937,#38938,#38939,#38940,#38941,#38942,
#38943,#38944,#38945,#38946,#38947,#38948,#38949,#38950,#38951,#38952,#38953,
#38954,#38955,#38956,#38957,#38958,#38959,#38960,#38961,#38962,#38963,#38964,
#38965,#38966,#38967,#38968,#38969,#38970,#38971,#38972,#38973,#38974,#38975,
#38976,#38977,#38978,#38979,#38980,#38981,#38982,#38983,#38984,#38985,#38986,
#38987,#38988,#38989,#38990,#38991,#38992,#38993,#38994,#38995,#38996,#38997,
#38998,#38999,#39000,#39001,#39002,#39003,#39004,#39005,#39006,#39007,#39008,
#39009,#39010,#39011,#39012,#39013,#39014,#39015,#39016,#39017,#39018,#39019,
#39020,#39021,#39022,#39023,#39024,#39025,#39026,#39027,#39028,#39029,#39030,
#39031,#39032,#39033,#39034,#39035,#39036,#39037,#39038,#39039,#39040,#39041,
#39042,#39043,#39044,#39045,#39046,#39047,#39048,#39049,#39050,#39051,#39052,
#39053,#39054,#39055,#39056,#39057,#39058,#39059,#39060,#39061,#39062,#39063,
#39064,#39065,#39066,#39067,#39068,#39069,#39070,#39071,#39072,#39073,#39074,
#39075,#39076,#39077,#39078,#39079,#39080,#39081,#39082,#39083,#39084,#39085,
#39086,#39087,#39088,#39089,#39090,#39091,#39092,#39093,#39094,#39095,#39096,
#39097,#39098,#39099,#39100,#39101,#39102,#39103,#39104,#39105,#39106,#39107,
#39108,#39109,#39110,#39111,#39112,#39113,#39114,#39115,#39116,#39117,#39118,
#39119,#39120,#39121,#39122,#39123,#39124,#39125,#39126,#39127,#39128,#39129,
#39130,#39131,#39132,#39133,#39134,#39135,#39136,#39137,#39138,#39139,#39140,
#39141,#39142,#39143,#39144,#39145,#39146,#39147,#39148,#39149,#39150,#39151,
#39152,#39153,#39154,#39155,#39156,#39157,#39158,#39159,#39160,#39161,#39162,
#39163,#39164,#39165,#39166,#39167,#39168,#39169,#39170,#39171,#39172,#39173,
#39174,#39175,#39176,#39177,#39178,#39179,#39180,#39181,#39182,#39183,#39184,
#39185,#39186,#39187,#39188,#39189,#39190,#39191,#39192,#39193,#39194,#39195,
#39196,#39197,#39198,#39199,#39200,#39201,#39202,#39203,#39204,#39205,#39206,
#39207,#39208));
#40904=AXIS2_PLACEMENT_3D('',#68016,#46177,#46178);
#40905=AXIS2_PLACEMENT_3D('',#68017,#46179,#46180);
#40906=AXIS2_PLACEMENT_3D('',#68020,#46181,#46182);
#40907=AXIS2_PLACEMENT_3D('',#68024,#46184,#46185);
#40908=AXIS2_PLACEMENT_3D('',#68048,#46187,#46188);
#40909=AXIS2_PLACEMENT_3D('',#68054,#46189,#46190);
#40910=AXIS2_PLACEMENT_3D('',#68059,#46191,#46192);
#40911=AXIS2_PLACEMENT_3D('',#68060,#46193,#46194);
#40912=AXIS2_PLACEMENT_3D('',#68061,#46195,#46196);
#40913=AXIS2_PLACEMENT_3D('',#68064,#46197,#46198);
#40914=AXIS2_PLACEMENT_3D('',#68068,#46200,#46201);
#40915=AXIS2_PLACEMENT_3D('',#68070,#46203,#46204);
#40916=AXIS2_PLACEMENT_3D('',#68073,#46205,#46206);
#40917=AXIS2_PLACEMENT_3D('',#68075,#46207,#46208);
#40918=AXIS2_PLACEMENT_3D('',#68077,#46209,#46210);
#40919=AXIS2_PLACEMENT_3D('',#68086,#46211,#46212);
#40920=AXIS2_PLACEMENT_3D('',#68089,#46214,#46215);
#40921=AXIS2_PLACEMENT_3D('',#68123,#46217,#46218);
#40922=AXIS2_PLACEMENT_3D('',#68129,#46219,#46220);
#40923=AXIS2_PLACEMENT_3D('',#68134,#46221,#46222);
#40924=AXIS2_PLACEMENT_3D('',#68135,#46223,#46224);
#40925=AXIS2_PLACEMENT_3D('',#68136,#46225,#46226);
#40926=AXIS2_PLACEMENT_3D('',#68137,#46227,#46228);
#40927=AXIS2_PLACEMENT_3D('',#68138,#46229,#46230);
#40928=AXIS2_PLACEMENT_3D('',#68139,#46231,#46232);
#40929=AXIS2_PLACEMENT_3D('',#68140,#46233,#46234);
#40930=AXIS2_PLACEMENT_3D('',#68144,#46236,#46237);
#40931=AXIS2_PLACEMENT_3D('',#68155,#46240,#46241);
#40932=AXIS2_PLACEMENT_3D('',#68159,#46243,#46244);
#40933=AXIS2_PLACEMENT_3D('',#68167,#46248,#46249);
#40934=AXIS2_PLACEMENT_3D('',#68175,#46253,#46254);
#40935=AXIS2_PLACEMENT_3D('',#68183,#46258,#46259);
#40936=AXIS2_PLACEMENT_3D('',#68191,#46263,#46264);
#40937=AXIS2_PLACEMENT_3D('',#68199,#46268,#46269);
#40938=AXIS2_PLACEMENT_3D('',#68207,#46273,#46274);
#40939=AXIS2_PLACEMENT_3D('',#68215,#46278,#46279);
#40940=AXIS2_PLACEMENT_3D('',#68223,#46283,#46284);
#40941=AXIS2_PLACEMENT_3D('',#68231,#46288,#46289);
#40942=AXIS2_PLACEMENT_3D('',#68239,#46293,#46294);
#40943=AXIS2_PLACEMENT_3D('',#68247,#46298,#46299);
#40944=AXIS2_PLACEMENT_3D('',#68255,#46303,#46304);
#40945=AXIS2_PLACEMENT_3D('',#68263,#46308,#46309);
#40946=AXIS2_PLACEMENT_3D('',#68271,#46313,#46314);
#40947=AXIS2_PLACEMENT_3D('',#68279,#46318,#46319);
#40948=AXIS2_PLACEMENT_3D('',#68287,#46323,#46324);
#40949=AXIS2_PLACEMENT_3D('',#68295,#46328,#46329);
#40950=AXIS2_PLACEMENT_3D('',#68303,#46333,#46334);
#40951=AXIS2_PLACEMENT_3D('',#68311,#46338,#46339);
#40952=AXIS2_PLACEMENT_3D('',#68319,#46343,#46344);
#40953=AXIS2_PLACEMENT_3D('',#68327,#46348,#46349);
#40954=AXIS2_PLACEMENT_3D('',#68335,#46353,#46354);
#40955=AXIS2_PLACEMENT_3D('',#68343,#46358,#46359);
#40956=AXIS2_PLACEMENT_3D('',#68351,#46363,#46364);
#40957=AXIS2_PLACEMENT_3D('',#68359,#46368,#46369);
#40958=AXIS2_PLACEMENT_3D('',#68367,#46373,#46374);
#40959=AXIS2_PLACEMENT_3D('',#68375,#46378,#46379);
#40960=AXIS2_PLACEMENT_3D('',#68383,#46383,#46384);
#40961=AXIS2_PLACEMENT_3D('',#68391,#46388,#46389);
#40962=AXIS2_PLACEMENT_3D('',#68399,#46393,#46394);
#40963=AXIS2_PLACEMENT_3D('',#68407,#46398,#46399);
#40964=AXIS2_PLACEMENT_3D('',#68415,#46403,#46404);
#40965=AXIS2_PLACEMENT_3D('',#68423,#46408,#46409);
#40966=AXIS2_PLACEMENT_3D('',#68431,#46413,#46414);
#40967=AXIS2_PLACEMENT_3D('',#68439,#46418,#46419);
#40968=AXIS2_PLACEMENT_3D('',#68447,#46423,#46424);
#40969=AXIS2_PLACEMENT_3D('',#68475,#46428,#46429);
#40970=AXIS2_PLACEMENT_3D('',#68503,#46433,#46434);
#40971=AXIS2_PLACEMENT_3D('',#68531,#46438,#46439);
#40972=AXIS2_PLACEMENT_3D('',#68539,#46443,#46444);
#40973=AXIS2_PLACEMENT_3D('',#68547,#46448,#46449);
#40974=AXIS2_PLACEMENT_3D('',#68555,#46453,#46454);
#40975=AXIS2_PLACEMENT_3D('',#68563,#46458,#46459);
#40976=AXIS2_PLACEMENT_3D('',#68571,#46463,#46464);
#40977=AXIS2_PLACEMENT_3D('',#68579,#46468,#46469);
#40978=AXIS2_PLACEMENT_3D('',#68587,#46473,#46474);
#40979=AXIS2_PLACEMENT_3D('',#68595,#46478,#46479);
#40980=AXIS2_PLACEMENT_3D('',#68598,#46481,#46482);
#40981=AXIS2_PLACEMENT_3D('',#68599,#46483,#46484);
#40982=AXIS2_PLACEMENT_3D('',#68601,#46485,#46486);
#40983=AXIS2_PLACEMENT_3D('',#68602,#46487,#46488);
#40984=AXIS2_PLACEMENT_3D('',#68603,#46489,#46490);
#40985=AXIS2_PLACEMENT_3D('',#68605,#46491,#46492);
#40986=AXIS2_PLACEMENT_3D('',#68610,#46493,#46494);
#40987=AXIS2_PLACEMENT_3D('',#68612,#46495,#46496);
#40988=AXIS2_PLACEMENT_3D('',#68613,#46497,#46498);
#40989=AXIS2_PLACEMENT_3D('',#68614,#46499,#46500);
#40990=AXIS2_PLACEMENT_3D('',#68616,#46502,#46503);
#40991=AXIS2_PLACEMENT_3D('',#68618,#46504,#46505);
#40992=AXIS2_PLACEMENT_3D('',#68620,#46506,#46507);
#40993=AXIS2_PLACEMENT_3D('',#68644,#46509,#46510);
#40994=AXIS2_PLACEMENT_3D('',#68650,#46511,#46512);
#40995=AXIS2_PLACEMENT_3D('',#68655,#46513,#46514);
#40996=AXIS2_PLACEMENT_3D('',#68656,#46515,#46516);
#40997=AXIS2_PLACEMENT_3D('',#68657,#46517,#46518);
#40998=AXIS2_PLACEMENT_3D('',#68660,#46519,#46520);
#40999=AXIS2_PLACEMENT_3D('',#68664,#46522,#46523);
#41000=AXIS2_PLACEMENT_3D('',#68666,#46525,#46526);
#41001=AXIS2_PLACEMENT_3D('',#68669,#46527,#46528);
#41002=AXIS2_PLACEMENT_3D('',#68671,#46529,#46530);
#41003=AXIS2_PLACEMENT_3D('',#68673,#46531,#46532);
#41004=AXIS2_PLACEMENT_3D('',#68682,#46533,#46534);
#41005=AXIS2_PLACEMENT_3D('',#68685,#46536,#46537);
#41006=AXIS2_PLACEMENT_3D('',#68719,#46539,#46540);
#41007=AXIS2_PLACEMENT_3D('',#68725,#46541,#46542);
#41008=AXIS2_PLACEMENT_3D('',#68730,#46543,#46544);
#41009=AXIS2_PLACEMENT_3D('',#68731,#46545,#46546);
#41010=AXIS2_PLACEMENT_3D('',#68732,#46547,#46548);
#41011=AXIS2_PLACEMENT_3D('',#68733,#46549,#46550);
#41012=AXIS2_PLACEMENT_3D('',#68734,#46551,#46552);
#41013=AXIS2_PLACEMENT_3D('',#68735,#46553,#46554);
#41014=AXIS2_PLACEMENT_3D('',#68736,#46555,#46556);
#41015=AXIS2_PLACEMENT_3D('',#68740,#46558,#46559);
#41016=AXIS2_PLACEMENT_3D('',#68751,#46562,#46563);
#41017=AXIS2_PLACEMENT_3D('',#68753,#46564,#46565);
#41018=AXIS2_PLACEMENT_3D('',#68754,#46566,#46567);
#41019=AXIS2_PLACEMENT_3D('',#68755,#46568,#46569);
#41020=AXIS2_PLACEMENT_3D('',#68757,#46570,#46571);
#41021=AXIS2_PLACEMENT_3D('',#68762,#46572,#46573);
#41022=AXIS2_PLACEMENT_3D('',#68764,#46574,#46575);
#41023=AXIS2_PLACEMENT_3D('',#68765,#46576,#46577);
#41024=AXIS2_PLACEMENT_3D('',#68766,#46578,#46579);
#41025=AXIS2_PLACEMENT_3D('',#68768,#46581,#46582);
#41026=AXIS2_PLACEMENT_3D('',#68770,#46583,#46584);
#41027=AXIS2_PLACEMENT_3D('',#68772,#46585,#46586);
#41028=AXIS2_PLACEMENT_3D('',#68796,#46588,#46589);
#41029=AXIS2_PLACEMENT_3D('',#68802,#46590,#46591);
#41030=AXIS2_PLACEMENT_3D('',#68807,#46592,#46593);
#41031=AXIS2_PLACEMENT_3D('',#68808,#46594,#46595);
#41032=AXIS2_PLACEMENT_3D('',#68809,#46596,#46597);
#41033=AXIS2_PLACEMENT_3D('',#68812,#46598,#46599);
#41034=AXIS2_PLACEMENT_3D('',#68816,#46601,#46602);
#41035=AXIS2_PLACEMENT_3D('',#68818,#46604,#46605);
#41036=AXIS2_PLACEMENT_3D('',#68821,#46606,#46607);
#41037=AXIS2_PLACEMENT_3D('',#68823,#46608,#46609);
#41038=AXIS2_PLACEMENT_3D('',#68825,#46610,#46611);
#41039=AXIS2_PLACEMENT_3D('',#68834,#46612,#46613);
#41040=AXIS2_PLACEMENT_3D('',#68837,#46615,#46616);
#41041=AXIS2_PLACEMENT_3D('',#68871,#46618,#46619);
#41042=AXIS2_PLACEMENT_3D('',#68877,#46620,#46621);
#41043=AXIS2_PLACEMENT_3D('',#68882,#46622,#46623);
#41044=AXIS2_PLACEMENT_3D('',#68883,#46624,#46625);
#41045=AXIS2_PLACEMENT_3D('',#68884,#46626,#46627);
#41046=AXIS2_PLACEMENT_3D('',#68885,#46628,#46629);
#41047=AXIS2_PLACEMENT_3D('',#68886,#46630,#46631);
#41048=AXIS2_PLACEMENT_3D('',#68887,#46632,#46633);
#41049=AXIS2_PLACEMENT_3D('',#68888,#46634,#46635);
#41050=AXIS2_PLACEMENT_3D('',#68892,#46637,#46638);
#41051=AXIS2_PLACEMENT_3D('',#68903,#46641,#46642);
#41052=AXIS2_PLACEMENT_3D('',#68905,#46643,#46644);
#41053=AXIS2_PLACEMENT_3D('',#68906,#46645,#46646);
#41054=AXIS2_PLACEMENT_3D('',#68907,#46647,#46648);
#41055=AXIS2_PLACEMENT_3D('',#68909,#46649,#46650);
#41056=AXIS2_PLACEMENT_3D('',#68914,#46651,#46652);
#41057=AXIS2_PLACEMENT_3D('',#68916,#46653,#46654);
#41058=AXIS2_PLACEMENT_3D('',#68917,#46655,#46656);
#41059=AXIS2_PLACEMENT_3D('',#68918,#46657,#46658);
#41060=AXIS2_PLACEMENT_3D('',#68920,#46660,#46661);
#41061=AXIS2_PLACEMENT_3D('',#68923,#46662,#46663);
#41062=AXIS2_PLACEMENT_3D('',#68927,#46665,#46666);
#41063=AXIS2_PLACEMENT_3D('',#68951,#46668,#46669);
#41064=AXIS2_PLACEMENT_3D('',#68957,#46670,#46671);
#41065=AXIS2_PLACEMENT_3D('',#68962,#46672,#46673);
#41066=AXIS2_PLACEMENT_3D('',#68963,#46674,#46675);
#41067=AXIS2_PLACEMENT_3D('',#68964,#46676,#46677);
#41068=AXIS2_PLACEMENT_3D('',#68967,#46678,#46679);
#41069=AXIS2_PLACEMENT_3D('',#68969,#46680,#46681);
#41070=AXIS2_PLACEMENT_3D('',#68971,#46682,#46683);
#41071=AXIS2_PLACEMENT_3D('',#68980,#46684,#46685);
#41072=AXIS2_PLACEMENT_3D('',#68983,#46687,#46688);
#41073=AXIS2_PLACEMENT_3D('',#68996,#46690,#46691);
#41074=AXIS2_PLACEMENT_3D('',#68997,#46692,#46693);
#41075=AXIS2_PLACEMENT_3D('',#68998,#46694,#46695);
#41076=AXIS2_PLACEMENT_3D('',#69000,#46696,#46697);
#41077=AXIS2_PLACEMENT_3D('',#69002,#46698,#46699);
#41078=AXIS2_PLACEMENT_3D('',#69025,#46701,#46702);
#41079=AXIS2_PLACEMENT_3D('',#69031,#46703,#46704);
#41080=AXIS2_PLACEMENT_3D('',#69036,#46705,#46706);
#41081=AXIS2_PLACEMENT_3D('',#69037,#46707,#46708);
#41082=AXIS2_PLACEMENT_3D('',#69038,#46709,#46710);
#41083=AXIS2_PLACEMENT_3D('',#69039,#46711,#46712);
#41084=AXIS2_PLACEMENT_3D('',#69040,#46713,#46714);
#41085=AXIS2_PLACEMENT_3D('',#69042,#46715,#46716);
#41086=AXIS2_PLACEMENT_3D('',#69044,#46717,#46718);
#41087=AXIS2_PLACEMENT_3D('',#69045,#46719,#46720);
#41088=AXIS2_PLACEMENT_3D('',#69046,#46721,#46722);
#41089=AXIS2_PLACEMENT_3D('',#69048,#46723,#46724);
#41090=AXIS2_PLACEMENT_3D('',#69053,#46725,#46726);
#41091=AXIS2_PLACEMENT_3D('',#69055,#46727,#46728);
#41092=AXIS2_PLACEMENT_3D('',#69056,#46729,#46730);
#41093=AXIS2_PLACEMENT_3D('',#69057,#46731,#46732);
#41094=AXIS2_PLACEMENT_3D('',#69059,#46734,#46735);
#41095=AXIS2_PLACEMENT_3D('',#69062,#46737,#46738);
#41096=AXIS2_PLACEMENT_3D('',#69063,#46739,#46740);
#41097=AXIS2_PLACEMENT_3D('',#69072,#46743,#46744);
#41098=AXIS2_PLACEMENT_3D('',#69075,#46745,#46746);
#41099=AXIS2_PLACEMENT_3D('',#69079,#46748,#46749);
#41100=AXIS2_PLACEMENT_3D('',#69103,#46751,#46752);
#41101=AXIS2_PLACEMENT_3D('',#69109,#46753,#46754);
#41102=AXIS2_PLACEMENT_3D('',#69114,#46755,#46756);
#41103=AXIS2_PLACEMENT_3D('',#69115,#46757,#46758);
#41104=AXIS2_PLACEMENT_3D('',#69116,#46759,#46760);
#41105=AXIS2_PLACEMENT_3D('',#69119,#46761,#46762);
#41106=AXIS2_PLACEMENT_3D('',#69121,#46763,#46764);
#41107=AXIS2_PLACEMENT_3D('',#69123,#46765,#46766);
#41108=AXIS2_PLACEMENT_3D('',#69132,#46767,#46768);
#41109=AXIS2_PLACEMENT_3D('',#69135,#46770,#46771);
#41110=AXIS2_PLACEMENT_3D('',#69148,#46773,#46774);
#41111=AXIS2_PLACEMENT_3D('',#69149,#46775,#46776);
#41112=AXIS2_PLACEMENT_3D('',#69150,#46777,#46778);
#41113=AXIS2_PLACEMENT_3D('',#69152,#46779,#46780);
#41114=AXIS2_PLACEMENT_3D('',#69154,#46781,#46782);
#41115=AXIS2_PLACEMENT_3D('',#69177,#46784,#46785);
#41116=AXIS2_PLACEMENT_3D('',#69183,#46786,#46787);
#41117=AXIS2_PLACEMENT_3D('',#69188,#46788,#46789);
#41118=AXIS2_PLACEMENT_3D('',#69189,#46790,#46791);
#41119=AXIS2_PLACEMENT_3D('',#69190,#46792,#46793);
#41120=AXIS2_PLACEMENT_3D('',#69191,#46794,#46795);
#41121=AXIS2_PLACEMENT_3D('',#69192,#46796,#46797);
#41122=AXIS2_PLACEMENT_3D('',#69194,#46798,#46799);
#41123=AXIS2_PLACEMENT_3D('',#69196,#46800,#46801);
#41124=AXIS2_PLACEMENT_3D('',#69197,#46802,#46803);
#41125=AXIS2_PLACEMENT_3D('',#69198,#46804,#46805);
#41126=AXIS2_PLACEMENT_3D('',#69200,#46806,#46807);
#41127=AXIS2_PLACEMENT_3D('',#69205,#46808,#46809);
#41128=AXIS2_PLACEMENT_3D('',#69207,#46810,#46811);
#41129=AXIS2_PLACEMENT_3D('',#69208,#46812,#46813);
#41130=AXIS2_PLACEMENT_3D('',#69209,#46814,#46815);
#41131=AXIS2_PLACEMENT_3D('',#69211,#46817,#46818);
#41132=AXIS2_PLACEMENT_3D('',#69214,#46820,#46821);
#41133=AXIS2_PLACEMENT_3D('',#69215,#46822,#46823);
#41134=AXIS2_PLACEMENT_3D('',#69224,#46826,#46827);
#41135=AXIS2_PLACEMENT_3D('',#69227,#46828,#46829);
#41136=AXIS2_PLACEMENT_3D('',#69231,#46831,#46832);
#41137=AXIS2_PLACEMENT_3D('',#69255,#46834,#46835);
#41138=AXIS2_PLACEMENT_3D('',#69261,#46836,#46837);
#41139=AXIS2_PLACEMENT_3D('',#69266,#46838,#46839);
#41140=AXIS2_PLACEMENT_3D('',#69267,#46840,#46841);
#41141=AXIS2_PLACEMENT_3D('',#69268,#46842,#46843);
#41142=AXIS2_PLACEMENT_3D('',#69287,#46845,#46846);
#41143=AXIS2_PLACEMENT_3D('',#69289,#46848,#46849);
#41144=AXIS2_PLACEMENT_3D('',#69290,#46850,#46851);
#41145=AXIS2_PLACEMENT_3D('',#69291,#46852,#46853);
#41146=AXIS2_PLACEMENT_3D('',#69292,#46854,#46855);
#41147=AXIS2_PLACEMENT_3D('',#69298,#46858,#46859);
#41148=AXIS2_PLACEMENT_3D('',#69306,#46863,#46864);
#41149=AXIS2_PLACEMENT_3D('',#69314,#46868,#46869);
#41150=AXIS2_PLACEMENT_3D('',#69322,#46873,#46874);
#41151=AXIS2_PLACEMENT_3D('',#69330,#46878,#46879);
#41152=AXIS2_PLACEMENT_3D('',#69338,#46883,#46884);
#41153=AXIS2_PLACEMENT_3D('',#69346,#46888,#46889);
#41154=AXIS2_PLACEMENT_3D('',#69354,#46893,#46894);
#41155=AXIS2_PLACEMENT_3D('',#69362,#46898,#46899);
#41156=AXIS2_PLACEMENT_3D('',#69370,#46903,#46904);
#41157=AXIS2_PLACEMENT_3D('',#69378,#46908,#46909);
#41158=AXIS2_PLACEMENT_3D('',#69386,#46913,#46914);
#41159=AXIS2_PLACEMENT_3D('',#69394,#46918,#46919);
#41160=AXIS2_PLACEMENT_3D('',#69402,#46923,#46924);
#41161=AXIS2_PLACEMENT_3D('',#69410,#46928,#46929);
#41162=AXIS2_PLACEMENT_3D('',#69418,#46933,#46934);
#41163=AXIS2_PLACEMENT_3D('',#69426,#46938,#46939);
#41164=AXIS2_PLACEMENT_3D('',#69434,#46943,#46944);
#41165=AXIS2_PLACEMENT_3D('',#69445,#46950,#46951);
#41166=AXIS2_PLACEMENT_3D('',#69453,#46955,#46956);
#41167=AXIS2_PLACEMENT_3D('',#69461,#46960,#46961);
#41168=AXIS2_PLACEMENT_3D('',#69469,#46965,#46966);
#41169=AXIS2_PLACEMENT_3D('',#69473,#46969,#46970);
#41170=AXIS2_PLACEMENT_3D('',#69479,#46973,#46974);
#41171=AXIS2_PLACEMENT_3D('',#69487,#46978,#46979);
#41172=AXIS2_PLACEMENT_3D('',#69495,#46983,#46984);
#41173=AXIS2_PLACEMENT_3D('',#69503,#46988,#46989);
#41174=AXIS2_PLACEMENT_3D('',#69514,#46995,#46996);
#41175=AXIS2_PLACEMENT_3D('',#69519,#46999,#47000);
#41176=AXIS2_PLACEMENT_3D('',#69527,#47004,#47005);
#41177=AXIS2_PLACEMENT_3D('',#69535,#47009,#47010);
#41178=AXIS2_PLACEMENT_3D('',#69543,#47014,#47015);
#41179=AXIS2_PLACEMENT_3D('',#69551,#47019,#47020);
#41180=AXIS2_PLACEMENT_3D('',#69555,#47023,#47024);
#41181=AXIS2_PLACEMENT_3D('',#69561,#47027,#47028);
#41182=AXIS2_PLACEMENT_3D('',#69569,#47032,#47033);
#41183=AXIS2_PLACEMENT_3D('',#69577,#47037,#47038);
#41184=AXIS2_PLACEMENT_3D('',#69585,#47042,#47043);
#41185=AXIS2_PLACEMENT_3D('',#69593,#47047,#47048);
#41186=AXIS2_PLACEMENT_3D('',#69601,#47052,#47053);
#41187=AXIS2_PLACEMENT_3D('',#69609,#47057,#47058);
#41188=AXIS2_PLACEMENT_3D('',#69617,#47062,#47063);
#41189=AXIS2_PLACEMENT_3D('',#69625,#47067,#47068);
#41190=AXIS2_PLACEMENT_3D('',#69633,#47072,#47073);
#41191=AXIS2_PLACEMENT_3D('',#69641,#47077,#47078);
#41192=AXIS2_PLACEMENT_3D('',#69646,#47081,#47082);
#41193=AXIS2_PLACEMENT_3D('',#69647,#47083,#47084);
#41194=AXIS2_PLACEMENT_3D('',#69649,#47085,#47086);
#41195=AXIS2_PLACEMENT_3D('',#69650,#47087,#47088);
#41196=AXIS2_PLACEMENT_3D('',#69651,#47089,#47090);
#41197=AXIS2_PLACEMENT_3D('',#69653,#47091,#47092);
#41198=AXIS2_PLACEMENT_3D('',#69658,#47093,#47094);
#41199=AXIS2_PLACEMENT_3D('',#69660,#47095,#47096);
#41200=AXIS2_PLACEMENT_3D('',#69661,#47097,#47098);
#41201=AXIS2_PLACEMENT_3D('',#69662,#47099,#47100);
#41202=AXIS2_PLACEMENT_3D('',#69664,#47101,#47102);
#41203=AXIS2_PLACEMENT_3D('',#69666,#47104,#47105);
#41204=AXIS2_PLACEMENT_3D('',#69668,#47106,#47107);
#41205=AXIS2_PLACEMENT_3D('',#69670,#47108,#47109);
#41206=AXIS2_PLACEMENT_3D('',#69694,#47111,#47112);
#41207=AXIS2_PLACEMENT_3D('',#69700,#47113,#47114);
#41208=AXIS2_PLACEMENT_3D('',#69705,#47115,#47116);
#41209=AXIS2_PLACEMENT_3D('',#69706,#47117,#47118);
#41210=AXIS2_PLACEMENT_3D('',#69707,#47119,#47120);
#41211=AXIS2_PLACEMENT_3D('',#69726,#47122,#47123);
#41212=AXIS2_PLACEMENT_3D('',#69728,#47125,#47126);
#41213=AXIS2_PLACEMENT_3D('',#69729,#47127,#47128);
#41214=AXIS2_PLACEMENT_3D('',#69730,#47129,#47130);
#41215=AXIS2_PLACEMENT_3D('',#69732,#47131,#47132);
#41216=AXIS2_PLACEMENT_3D('',#69733,#47133,#47134);
#41217=AXIS2_PLACEMENT_3D('',#69734,#47135,#47136);
#41218=AXIS2_PLACEMENT_3D('',#69736,#47137,#47138);
#41219=AXIS2_PLACEMENT_3D('',#69741,#47139,#47140);
#41220=AXIS2_PLACEMENT_3D('',#69743,#47141,#47142);
#41221=AXIS2_PLACEMENT_3D('',#69744,#47143,#47144);
#41222=AXIS2_PLACEMENT_3D('',#69745,#47145,#47146);
#41223=AXIS2_PLACEMENT_3D('',#69747,#47147,#47148);
#41224=AXIS2_PLACEMENT_3D('',#69749,#47150,#47151);
#41225=AXIS2_PLACEMENT_3D('',#69751,#47152,#47153);
#41226=AXIS2_PLACEMENT_3D('',#69753,#47154,#47155);
#41227=AXIS2_PLACEMENT_3D('',#69777,#47157,#47158);
#41228=AXIS2_PLACEMENT_3D('',#69783,#47159,#47160);
#41229=AXIS2_PLACEMENT_3D('',#69788,#47161,#47162);
#41230=AXIS2_PLACEMENT_3D('',#69789,#47163,#47164);
#41231=AXIS2_PLACEMENT_3D('',#69790,#47165,#47166);
#41232=AXIS2_PLACEMENT_3D('',#69809,#47168,#47169);
#41233=AXIS2_PLACEMENT_3D('',#69811,#47171,#47172);
#41234=AXIS2_PLACEMENT_3D('',#69812,#47173,#47174);
#41235=AXIS2_PLACEMENT_3D('',#69813,#47175,#47176);
#41236=AXIS2_PLACEMENT_3D('',#69815,#47177,#47178);
#41237=AXIS2_PLACEMENT_3D('',#69816,#47179,#47180);
#41238=AXIS2_PLACEMENT_3D('',#69817,#47181,#47182);
#41239=AXIS2_PLACEMENT_3D('',#69819,#47183,#47184);
#41240=AXIS2_PLACEMENT_3D('',#69824,#47185,#47186);
#41241=AXIS2_PLACEMENT_3D('',#69826,#47187,#47188);
#41242=AXIS2_PLACEMENT_3D('',#69827,#47189,#47190);
#41243=AXIS2_PLACEMENT_3D('',#69828,#47191,#47192);
#41244=AXIS2_PLACEMENT_3D('',#69830,#47193,#47194);
#41245=AXIS2_PLACEMENT_3D('',#69832,#47196,#47197);
#41246=AXIS2_PLACEMENT_3D('',#69834,#47198,#47199);
#41247=AXIS2_PLACEMENT_3D('',#69836,#47200,#47201);
#41248=AXIS2_PLACEMENT_3D('',#69838,#47203,#47204);
#41249=AXIS2_PLACEMENT_3D('',#69840,#47205,#47206);
#41250=AXIS2_PLACEMENT_3D('',#69842,#47207,#47208);
#41251=AXIS2_PLACEMENT_3D('',#69866,#47210,#47211);
#41252=AXIS2_PLACEMENT_3D('',#69872,#47212,#47213);
#41253=AXIS2_PLACEMENT_3D('',#69877,#47214,#47215);
#41254=AXIS2_PLACEMENT_3D('',#69878,#47216,#47217);
#41255=AXIS2_PLACEMENT_3D('',#69879,#47218,#47219);
#41256=AXIS2_PLACEMENT_3D('',#69882,#47220,#47221);
#41257=AXIS2_PLACEMENT_3D('',#69884,#47222,#47223);
#41258=AXIS2_PLACEMENT_3D('',#69886,#47224,#47225);
#41259=AXIS2_PLACEMENT_3D('',#69895,#47226,#47227);
#41260=AXIS2_PLACEMENT_3D('',#69898,#47229,#47230);
#41261=AXIS2_PLACEMENT_3D('',#69911,#47232,#47233);
#41262=AXIS2_PLACEMENT_3D('',#69912,#47234,#47235);
#41263=AXIS2_PLACEMENT_3D('',#69934,#47236,#47237);
#41264=AXIS2_PLACEMENT_3D('',#69940,#47238,#47239);
#41265=AXIS2_PLACEMENT_3D('',#69945,#47240,#47241);
#41266=AXIS2_PLACEMENT_3D('',#69946,#47242,#47243);
#41267=AXIS2_PLACEMENT_3D('',#69947,#47244,#47245);
#41268=AXIS2_PLACEMENT_3D('',#69948,#47246,#47247);
#41269=AXIS2_PLACEMENT_3D('',#69949,#47248,#47249);
#41270=AXIS2_PLACEMENT_3D('',#69952,#47251,#47252);
#41271=AXIS2_PLACEMENT_3D('',#69953,#47253,#47254);
#41272=AXIS2_PLACEMENT_3D('',#69956,#47256,#47257);
#41273=AXIS2_PLACEMENT_3D('',#69957,#47258,#47259);
#41274=AXIS2_PLACEMENT_3D('',#69960,#47261,#47262);
#41275=AXIS2_PLACEMENT_3D('',#69965,#47263,#47264);
#41276=AXIS2_PLACEMENT_3D('',#69967,#47265,#47266);
#41277=AXIS2_PLACEMENT_3D('',#69974,#47267,#47268);
#41278=AXIS2_PLACEMENT_3D('',#69976,#47270,#47271);
#41279=AXIS2_PLACEMENT_3D('',#69978,#47272,#47273);
#41280=AXIS2_PLACEMENT_3D('',#69980,#47274,#47275);
#41281=AXIS2_PLACEMENT_3D('',#70004,#47277,#47278);
#41282=AXIS2_PLACEMENT_3D('',#70010,#47279,#47280);
#41283=AXIS2_PLACEMENT_3D('',#70015,#47281,#47282);
#41284=AXIS2_PLACEMENT_3D('',#70016,#47283,#47284);
#41285=AXIS2_PLACEMENT_3D('',#70017,#47285,#47286);
#41286=AXIS2_PLACEMENT_3D('',#70036,#47288,#47289);
#41287=AXIS2_PLACEMENT_3D('',#70038,#47291,#47292);
#41288=AXIS2_PLACEMENT_3D('',#70039,#47293,#47294);
#41289=AXIS2_PLACEMENT_3D('',#70040,#47295,#47296);
#41290=AXIS2_PLACEMENT_3D('',#70042,#47297,#47298);
#41291=AXIS2_PLACEMENT_3D('',#70043,#47299,#47300);
#41292=AXIS2_PLACEMENT_3D('',#70044,#47301,#47302);
#41293=AXIS2_PLACEMENT_3D('',#70046,#47303,#47304);
#41294=AXIS2_PLACEMENT_3D('',#70051,#47305,#47306);
#41295=AXIS2_PLACEMENT_3D('',#70053,#47307,#47308);
#41296=AXIS2_PLACEMENT_3D('',#70054,#47309,#47310);
#41297=AXIS2_PLACEMENT_3D('',#70055,#47311,#47312);
#41298=AXIS2_PLACEMENT_3D('',#70057,#47313,#47314);
#41299=AXIS2_PLACEMENT_3D('',#70059,#47316,#47317);
#41300=AXIS2_PLACEMENT_3D('',#70061,#47318,#47319);
#41301=AXIS2_PLACEMENT_3D('',#70063,#47320,#47321);
#41302=AXIS2_PLACEMENT_3D('',#70087,#47323,#47324);
#41303=AXIS2_PLACEMENT_3D('',#70093,#47325,#47326);
#41304=AXIS2_PLACEMENT_3D('',#70098,#47327,#47328);
#41305=AXIS2_PLACEMENT_3D('',#70099,#47329,#47330);
#41306=AXIS2_PLACEMENT_3D('',#70100,#47331,#47332);
#41307=AXIS2_PLACEMENT_3D('',#70119,#47334,#47335);
#41308=AXIS2_PLACEMENT_3D('',#70121,#47337,#47338);
#41309=AXIS2_PLACEMENT_3D('',#70122,#47339,#47340);
#41310=AXIS2_PLACEMENT_3D('',#70123,#47341,#47342);
#41311=AXIS2_PLACEMENT_3D('',#70125,#47343,#47344);
#41312=AXIS2_PLACEMENT_3D('',#70126,#47345,#47346);
#41313=AXIS2_PLACEMENT_3D('',#70127,#47347,#47348);
#41314=AXIS2_PLACEMENT_3D('',#70129,#47349,#47350);
#41315=AXIS2_PLACEMENT_3D('',#70134,#47351,#47352);
#41316=AXIS2_PLACEMENT_3D('',#70136,#47353,#47354);
#41317=AXIS2_PLACEMENT_3D('',#70137,#47355,#47356);
#41318=AXIS2_PLACEMENT_3D('',#70138,#47357,#47358);
#41319=AXIS2_PLACEMENT_3D('',#70140,#47359,#47360);
#41320=AXIS2_PLACEMENT_3D('',#70142,#47362,#47363);
#41321=AXIS2_PLACEMENT_3D('',#70144,#47364,#47365);
#41322=AXIS2_PLACEMENT_3D('',#70146,#47366,#47367);
#41323=AXIS2_PLACEMENT_3D('',#70170,#47369,#47370);
#41324=AXIS2_PLACEMENT_3D('',#70176,#47371,#47372);
#41325=AXIS2_PLACEMENT_3D('',#70181,#47373,#47374);
#41326=AXIS2_PLACEMENT_3D('',#70182,#47375,#47376);
#41327=AXIS2_PLACEMENT_3D('',#70183,#47377,#47378);
#41328=AXIS2_PLACEMENT_3D('',#70202,#47380,#47381);
#41329=AXIS2_PLACEMENT_3D('',#70204,#47383,#47384);
#41330=AXIS2_PLACEMENT_3D('',#70205,#47385,#47386);
#41331=AXIS2_PLACEMENT_3D('',#70206,#47387,#47388);
#41332=AXIS2_PLACEMENT_3D('',#70208,#47389,#47390);
#41333=AXIS2_PLACEMENT_3D('',#70209,#47391,#47392);
#41334=AXIS2_PLACEMENT_3D('',#70210,#47393,#47394);
#41335=AXIS2_PLACEMENT_3D('',#70212,#47395,#47396);
#41336=AXIS2_PLACEMENT_3D('',#70217,#47397,#47398);
#41337=AXIS2_PLACEMENT_3D('',#70219,#47399,#47400);
#41338=AXIS2_PLACEMENT_3D('',#70221,#47401,#47402);
#41339=AXIS2_PLACEMENT_3D('',#70223,#47404,#47405);
#41340=AXIS2_PLACEMENT_3D('',#70225,#47406,#47407);
#41341=AXIS2_PLACEMENT_3D('',#70227,#47408,#47409);
#41342=AXIS2_PLACEMENT_3D('',#70251,#47411,#47412);
#41343=AXIS2_PLACEMENT_3D('',#70257,#47413,#47414);
#41344=AXIS2_PLACEMENT_3D('',#70262,#47415,#47416);
#41345=AXIS2_PLACEMENT_3D('',#70263,#47417,#47418);
#41346=AXIS2_PLACEMENT_3D('',#70264,#47419,#47420);
#41347=AXIS2_PLACEMENT_3D('',#70267,#47421,#47422);
#41348=AXIS2_PLACEMENT_3D('',#70269,#47423,#47424);
#41349=AXIS2_PLACEMENT_3D('',#70271,#47425,#47426);
#41350=AXIS2_PLACEMENT_3D('',#70280,#47427,#47428);
#41351=AXIS2_PLACEMENT_3D('',#70283,#47430,#47431);
#41352=AXIS2_PLACEMENT_3D('',#70296,#47433,#47434);
#41353=AXIS2_PLACEMENT_3D('',#70297,#47435,#47436);
#41354=AXIS2_PLACEMENT_3D('',#70319,#47437,#47438);
#41355=AXIS2_PLACEMENT_3D('',#70325,#47439,#47440);
#41356=AXIS2_PLACEMENT_3D('',#70330,#47441,#47442);
#41357=AXIS2_PLACEMENT_3D('',#70331,#47443,#47444);
#41358=AXIS2_PLACEMENT_3D('',#70332,#47445,#47446);
#41359=AXIS2_PLACEMENT_3D('',#70333,#47447,#47448);
#41360=AXIS2_PLACEMENT_3D('',#70334,#47449,#47450);
#41361=AXIS2_PLACEMENT_3D('',#70337,#47452,#47453);
#41362=AXIS2_PLACEMENT_3D('',#70338,#47454,#47455);
#41363=AXIS2_PLACEMENT_3D('',#70341,#47457,#47458);
#41364=AXIS2_PLACEMENT_3D('',#70342,#47459,#47460);
#41365=AXIS2_PLACEMENT_3D('',#70345,#47462,#47463);
#41366=AXIS2_PLACEMENT_3D('',#70350,#47464,#47465);
#41367=AXIS2_PLACEMENT_3D('',#70352,#47466,#47467);
#41368=AXIS2_PLACEMENT_3D('',#70359,#47468,#47469);
#41369=AXIS2_PLACEMENT_3D('',#70382,#47471,#47472);
#41370=AXIS2_PLACEMENT_3D('',#70384,#47473,#47474);
#41371=AXIS2_PLACEMENT_3D('',#70389,#47475,#47476);
#41372=AXIS2_PLACEMENT_3D('',#70391,#47477,#47478);
#41373=AXIS2_PLACEMENT_3D('',#70392,#47479,#47480);
#41374=AXIS2_PLACEMENT_3D('',#70393,#47481,#47482);
#41375=AXIS2_PLACEMENT_3D('',#70394,#47483,#47484);
#41376=AXIS2_PLACEMENT_3D('',#70395,#47485,#47486);
#41377=AXIS2_PLACEMENT_3D('',#70396,#47487,#47488);
#41378=AXIS2_PLACEMENT_3D('',#70399,#47490,#47491);
#41379=AXIS2_PLACEMENT_3D('',#70400,#47492,#47493);
#41380=AXIS2_PLACEMENT_3D('',#70401,#47494,#47495);
#41381=AXIS2_PLACEMENT_3D('',#70404,#47497,#47498);
#41382=AXIS2_PLACEMENT_3D('',#70434,#47500,#47501);
#41383=AXIS2_PLACEMENT_3D('',#70436,#47502,#47503);
#41384=AXIS2_PLACEMENT_3D('',#70441,#47504,#47505);
#41385=AXIS2_PLACEMENT_3D('',#70442,#47506,#47507);
#41386=AXIS2_PLACEMENT_3D('',#70445,#47509,#47510);
#41387=AXIS2_PLACEMENT_3D('',#70446,#47511,#47512);
#41388=AXIS2_PLACEMENT_3D('',#70447,#47513,#47514);
#41389=AXIS2_PLACEMENT_3D('',#70448,#47515,#47516);
#41390=AXIS2_PLACEMENT_3D('',#70449,#47517,#47518);
#41391=AXIS2_PLACEMENT_3D('',#70452,#47520,#47521);
#41392=AXIS2_PLACEMENT_3D('',#70461,#47523,#47524);
#41393=AXIS2_PLACEMENT_3D('',#70463,#47525,#47526);
#41394=AXIS2_PLACEMENT_3D('',#70465,#47527,#47528);
#41395=AXIS2_PLACEMENT_3D('',#70489,#47530,#47531);
#41396=AXIS2_PLACEMENT_3D('',#70495,#47532,#47533);
#41397=AXIS2_PLACEMENT_3D('',#70500,#47534,#47535);
#41398=AXIS2_PLACEMENT_3D('',#70501,#47536,#47537);
#41399=AXIS2_PLACEMENT_3D('',#70502,#47538,#47539);
#41400=AXIS2_PLACEMENT_3D('',#70521,#47541,#47542);
#41401=AXIS2_PLACEMENT_3D('',#70523,#47544,#47545);
#41402=AXIS2_PLACEMENT_3D('',#70524,#47546,#47547);
#41403=AXIS2_PLACEMENT_3D('',#70525,#47548,#47549);
#41404=AXIS2_PLACEMENT_3D('',#70527,#47550,#47551);
#41405=AXIS2_PLACEMENT_3D('',#70528,#47552,#47553);
#41406=AXIS2_PLACEMENT_3D('',#70529,#47554,#47555);
#41407=AXIS2_PLACEMENT_3D('',#70531,#47556,#47557);
#41408=AXIS2_PLACEMENT_3D('',#70536,#47558,#47559);
#41409=AXIS2_PLACEMENT_3D('',#70538,#47560,#47561);
#41410=AXIS2_PLACEMENT_3D('',#70539,#47562,#47563);
#41411=AXIS2_PLACEMENT_3D('',#70540,#47564,#47565);
#41412=AXIS2_PLACEMENT_3D('',#70542,#47566,#47567);
#41413=AXIS2_PLACEMENT_3D('',#70565,#47569,#47570);
#41414=AXIS2_PLACEMENT_3D('',#70567,#47571,#47572);
#41415=AXIS2_PLACEMENT_3D('',#70572,#47573,#47574);
#41416=AXIS2_PLACEMENT_3D('',#70573,#47575,#47576);
#41417=AXIS2_PLACEMENT_3D('',#70576,#47578,#47579);
#41418=AXIS2_PLACEMENT_3D('',#70577,#47580,#47581);
#41419=AXIS2_PLACEMENT_3D('',#70578,#47582,#47583);
#41420=AXIS2_PLACEMENT_3D('',#70579,#47584,#47585);
#41421=AXIS2_PLACEMENT_3D('',#70580,#47586,#47587);
#41422=AXIS2_PLACEMENT_3D('',#70583,#47589,#47590);
#41423=AXIS2_PLACEMENT_3D('',#70592,#47592,#47593);
#41424=AXIS2_PLACEMENT_3D('',#70594,#47594,#47595);
#41425=AXIS2_PLACEMENT_3D('',#70596,#47596,#47597);
#41426=AXIS2_PLACEMENT_3D('',#70620,#47599,#47600);
#41427=AXIS2_PLACEMENT_3D('',#70626,#47601,#47602);
#41428=AXIS2_PLACEMENT_3D('',#70631,#47603,#47604);
#41429=AXIS2_PLACEMENT_3D('',#70632,#47605,#47606);
#41430=AXIS2_PLACEMENT_3D('',#70633,#47607,#47608);
#41431=AXIS2_PLACEMENT_3D('',#70652,#47610,#47611);
#41432=AXIS2_PLACEMENT_3D('',#70654,#47613,#47614);
#41433=AXIS2_PLACEMENT_3D('',#70655,#47615,#47616);
#41434=AXIS2_PLACEMENT_3D('',#70656,#47617,#47618);
#41435=AXIS2_PLACEMENT_3D('',#70658,#47619,#47620);
#41436=AXIS2_PLACEMENT_3D('',#70659,#47621,#47622);
#41437=AXIS2_PLACEMENT_3D('',#70660,#47623,#47624);
#41438=AXIS2_PLACEMENT_3D('',#70662,#47625,#47626);
#41439=AXIS2_PLACEMENT_3D('',#70688,#47627,#47628);
#41440=AXIS2_PLACEMENT_3D('',#70690,#47629,#47630);
#41441=AXIS2_PLACEMENT_3D('',#70695,#47631,#47632);
#41442=AXIS2_PLACEMENT_3D('',#70696,#47633,#47634);
#41443=AXIS2_PLACEMENT_3D('',#70699,#47636,#47637);
#41444=AXIS2_PLACEMENT_3D('',#70700,#47638,#47639);
#41445=AXIS2_PLACEMENT_3D('',#70701,#47640,#47641);
#41446=AXIS2_PLACEMENT_3D('',#70702,#47642,#47643);
#41447=AXIS2_PLACEMENT_3D('',#70703,#47644,#47645);
#41448=AXIS2_PLACEMENT_3D('',#70720,#47647,#47648);
#41449=AXIS2_PLACEMENT_3D('',#70730,#47650,#47651);
#41450=AXIS2_PLACEMENT_3D('',#70753,#47653,#47654);
#41451=AXIS2_PLACEMENT_3D('',#70755,#47655,#47656);
#41452=AXIS2_PLACEMENT_3D('',#70760,#47657,#47658);
#41453=AXIS2_PLACEMENT_3D('',#70762,#47659,#47660);
#41454=AXIS2_PLACEMENT_3D('',#70763,#47661,#47662);
#41455=AXIS2_PLACEMENT_3D('',#70764,#47663,#47664);
#41456=AXIS2_PLACEMENT_3D('',#70765,#47665,#47666);
#41457=AXIS2_PLACEMENT_3D('',#70766,#47667,#47668);
#41458=AXIS2_PLACEMENT_3D('',#70767,#47669,#47670);
#41459=AXIS2_PLACEMENT_3D('',#70770,#47672,#47673);
#41460=AXIS2_PLACEMENT_3D('',#70771,#47674,#47675);
#41461=AXIS2_PLACEMENT_3D('',#70772,#47676,#47677);
#41462=AXIS2_PLACEMENT_3D('',#70775,#47679,#47680);
#41463=AXIS2_PLACEMENT_3D('',#70784,#47682,#47683);
#41464=AXIS2_PLACEMENT_3D('',#70801,#47685,#47686);
#41465=AXIS2_PLACEMENT_3D('',#70811,#47688,#47689);
#41466=AXIS2_PLACEMENT_3D('',#70813,#47691,#47692);
#41467=AXIS2_PLACEMENT_3D('',#70815,#47693,#47694);
#41468=AXIS2_PLACEMENT_3D('',#70817,#47695,#47696);
#41469=AXIS2_PLACEMENT_3D('',#70841,#47698,#47699);
#41470=AXIS2_PLACEMENT_3D('',#70847,#47700,#47701);
#41471=AXIS2_PLACEMENT_3D('',#70852,#47702,#47703);
#41472=AXIS2_PLACEMENT_3D('',#70853,#47704,#47705);
#41473=AXIS2_PLACEMENT_3D('',#70854,#47706,#47707);
#41474=AXIS2_PLACEMENT_3D('',#70873,#47709,#47710);
#41475=AXIS2_PLACEMENT_3D('',#70875,#47712,#47713);
#41476=AXIS2_PLACEMENT_3D('',#70876,#47714,#47715);
#41477=AXIS2_PLACEMENT_3D('',#70877,#47716,#47717);
#41478=AXIS2_PLACEMENT_3D('',#70879,#47718,#47719);
#41479=AXIS2_PLACEMENT_3D('',#70880,#47720,#47721);
#41480=AXIS2_PLACEMENT_3D('',#70881,#47722,#47723);
#41481=AXIS2_PLACEMENT_3D('',#70883,#47724,#47725);
#41482=AXIS2_PLACEMENT_3D('',#70888,#47726,#47727);
#41483=AXIS2_PLACEMENT_3D('',#70890,#47728,#47729);
#41484=AXIS2_PLACEMENT_3D('',#70892,#47730,#47731);
#41485=AXIS2_PLACEMENT_3D('',#70916,#47733,#47734);
#41486=AXIS2_PLACEMENT_3D('',#70922,#47735,#47736);
#41487=AXIS2_PLACEMENT_3D('',#70927,#47737,#47738);
#41488=AXIS2_PLACEMENT_3D('',#70928,#47739,#47740);
#41489=AXIS2_PLACEMENT_3D('',#70929,#47741,#47742);
#41490=AXIS2_PLACEMENT_3D('',#70948,#47744,#47745);
#41491=AXIS2_PLACEMENT_3D('',#70950,#47747,#47748);
#41492=AXIS2_PLACEMENT_3D('',#70951,#47749,#47750);
#41493=AXIS2_PLACEMENT_3D('',#70952,#47751,#47752);
#41494=AXIS2_PLACEMENT_3D('',#70954,#47753,#47754);
#41495=AXIS2_PLACEMENT_3D('',#70955,#47755,#47756);
#41496=AXIS2_PLACEMENT_3D('',#70956,#47757,#47758);
#41497=AXIS2_PLACEMENT_3D('',#70958,#47759,#47760);
#41498=AXIS2_PLACEMENT_3D('',#70963,#47761,#47762);
#41499=AXIS2_PLACEMENT_3D('',#70965,#47763,#47764);
#41500=AXIS2_PLACEMENT_3D('',#70966,#47765,#47766);
#41501=AXIS2_PLACEMENT_3D('',#70967,#47767,#47768);
#41502=AXIS2_PLACEMENT_3D('',#70969,#47769,#47770);
#41503=AXIS2_PLACEMENT_3D('',#70971,#47772,#47773);
#41504=AXIS2_PLACEMENT_3D('',#70973,#47774,#47775);
#41505=AXIS2_PLACEMENT_3D('',#70975,#47776,#47777);
#41506=AXIS2_PLACEMENT_3D('',#70999,#47779,#47780);
#41507=AXIS2_PLACEMENT_3D('',#71005,#47781,#47782);
#41508=AXIS2_PLACEMENT_3D('',#71010,#47783,#47784);
#41509=AXIS2_PLACEMENT_3D('',#71011,#47785,#47786);
#41510=AXIS2_PLACEMENT_3D('',#71012,#47787,#47788);
#41511=AXIS2_PLACEMENT_3D('',#71031,#47790,#47791);
#41512=AXIS2_PLACEMENT_3D('',#71033,#47793,#47794);
#41513=AXIS2_PLACEMENT_3D('',#71034,#47795,#47796);
#41514=AXIS2_PLACEMENT_3D('',#71035,#47797,#47798);
#41515=AXIS2_PLACEMENT_3D('',#71037,#47799,#47800);
#41516=AXIS2_PLACEMENT_3D('',#71038,#47801,#47802);
#41517=AXIS2_PLACEMENT_3D('',#71039,#47803,#47804);
#41518=AXIS2_PLACEMENT_3D('',#71041,#47805,#47806);
#41519=AXIS2_PLACEMENT_3D('',#71046,#47807,#47808);
#41520=AXIS2_PLACEMENT_3D('',#71048,#47809,#47810);
#41521=AXIS2_PLACEMENT_3D('',#71049,#47811,#47812);
#41522=AXIS2_PLACEMENT_3D('',#71050,#47813,#47814);
#41523=AXIS2_PLACEMENT_3D('',#71052,#47815,#47816);
#41524=AXIS2_PLACEMENT_3D('',#71075,#47818,#47819);
#41525=AXIS2_PLACEMENT_3D('',#71077,#47820,#47821);
#41526=AXIS2_PLACEMENT_3D('',#71082,#47822,#47823);
#41527=AXIS2_PLACEMENT_3D('',#71083,#47824,#47825);
#41528=AXIS2_PLACEMENT_3D('',#71086,#47827,#47828);
#41529=AXIS2_PLACEMENT_3D('',#71087,#47829,#47830);
#41530=AXIS2_PLACEMENT_3D('',#71088,#47831,#47832);
#41531=AXIS2_PLACEMENT_3D('',#71089,#47833,#47834);
#41532=AXIS2_PLACEMENT_3D('',#71090,#47835,#47836);
#41533=AXIS2_PLACEMENT_3D('',#71093,#47838,#47839);
#41534=AXIS2_PLACEMENT_3D('',#71102,#47841,#47842);
#41535=AXIS2_PLACEMENT_3D('',#71104,#47843,#47844);
#41536=AXIS2_PLACEMENT_3D('',#71106,#47845,#47846);
#41537=AXIS2_PLACEMENT_3D('',#71130,#47848,#47849);
#41538=AXIS2_PLACEMENT_3D('',#71136,#47850,#47851);
#41539=AXIS2_PLACEMENT_3D('',#71141,#47852,#47853);
#41540=AXIS2_PLACEMENT_3D('',#71142,#47854,#47855);
#41541=AXIS2_PLACEMENT_3D('',#71143,#47856,#47857);
#41542=AXIS2_PLACEMENT_3D('',#71162,#47859,#47860);
#41543=AXIS2_PLACEMENT_3D('',#71164,#47862,#47863);
#41544=AXIS2_PLACEMENT_3D('',#71165,#47864,#47865);
#41545=AXIS2_PLACEMENT_3D('',#71166,#47866,#47867);
#41546=AXIS2_PLACEMENT_3D('',#71168,#47868,#47869);
#41547=AXIS2_PLACEMENT_3D('',#71169,#47870,#47871);
#41548=AXIS2_PLACEMENT_3D('',#71170,#47872,#47873);
#41549=AXIS2_PLACEMENT_3D('',#71172,#47874,#47875);
#41550=AXIS2_PLACEMENT_3D('',#71177,#47876,#47877);
#41551=AXIS2_PLACEMENT_3D('',#71179,#47878,#47879);
#41552=AXIS2_PLACEMENT_3D('',#71180,#47880,#47881);
#41553=AXIS2_PLACEMENT_3D('',#71181,#47882,#47883);
#41554=AXIS2_PLACEMENT_3D('',#71183,#47884,#47885);
#41555=AXIS2_PLACEMENT_3D('',#71206,#47887,#47888);
#41556=AXIS2_PLACEMENT_3D('',#71208,#47889,#47890);
#41557=AXIS2_PLACEMENT_3D('',#71213,#47891,#47892);
#41558=AXIS2_PLACEMENT_3D('',#71214,#47893,#47894);
#41559=AXIS2_PLACEMENT_3D('',#71217,#47896,#47897);
#41560=AXIS2_PLACEMENT_3D('',#71218,#47898,#47899);
#41561=AXIS2_PLACEMENT_3D('',#71219,#47900,#47901);
#41562=AXIS2_PLACEMENT_3D('',#71220,#47902,#47903);
#41563=AXIS2_PLACEMENT_3D('',#71221,#47904,#47905);
#41564=AXIS2_PLACEMENT_3D('',#71224,#47907,#47908);
#41565=AXIS2_PLACEMENT_3D('',#71233,#47910,#47911);
#41566=AXIS2_PLACEMENT_3D('',#71250,#47913,#47914);
#41567=AXIS2_PLACEMENT_3D('',#71260,#47916,#47917);
#41568=AXIS2_PLACEMENT_3D('',#71262,#47919,#47920);
#41569=AXIS2_PLACEMENT_3D('',#71264,#47921,#47922);
#41570=AXIS2_PLACEMENT_3D('',#71266,#47923,#47924);
#41571=AXIS2_PLACEMENT_3D('',#71290,#47926,#47927);
#41572=AXIS2_PLACEMENT_3D('',#71296,#47928,#47929);
#41573=AXIS2_PLACEMENT_3D('',#71301,#47930,#47931);
#41574=AXIS2_PLACEMENT_3D('',#71302,#47932,#47933);
#41575=AXIS2_PLACEMENT_3D('',#71303,#47934,#47935);
#41576=AXIS2_PLACEMENT_3D('',#71322,#47937,#47938);
#41577=AXIS2_PLACEMENT_3D('',#71324,#47940,#47941);
#41578=AXIS2_PLACEMENT_3D('',#71325,#47942,#47943);
#41579=AXIS2_PLACEMENT_3D('',#71326,#47944,#47945);
#41580=AXIS2_PLACEMENT_3D('',#71328,#47946,#47947);
#41581=AXIS2_PLACEMENT_3D('',#71329,#47948,#47949);
#41582=AXIS2_PLACEMENT_3D('',#71330,#47950,#47951);
#41583=AXIS2_PLACEMENT_3D('',#71332,#47952,#47953);
#41584=AXIS2_PLACEMENT_3D('',#71337,#47954,#47955);
#41585=AXIS2_PLACEMENT_3D('',#71339,#47956,#47957);
#41586=AXIS2_PLACEMENT_3D('',#71340,#47958,#47959);
#41587=AXIS2_PLACEMENT_3D('',#71341,#47960,#47961);
#41588=AXIS2_PLACEMENT_3D('',#71343,#47962,#47963);
#41589=AXIS2_PLACEMENT_3D('',#71345,#47965,#47966);
#41590=AXIS2_PLACEMENT_3D('',#71347,#47967,#47968);
#41591=AXIS2_PLACEMENT_3D('',#71349,#47969,#47970);
#41592=AXIS2_PLACEMENT_3D('',#71373,#47972,#47973);
#41593=AXIS2_PLACEMENT_3D('',#71379,#47974,#47975);
#41594=AXIS2_PLACEMENT_3D('',#71384,#47976,#47977);
#41595=AXIS2_PLACEMENT_3D('',#71385,#47978,#47979);
#41596=AXIS2_PLACEMENT_3D('',#71386,#47980,#47981);
#41597=AXIS2_PLACEMENT_3D('',#71405,#47983,#47984);
#41598=AXIS2_PLACEMENT_3D('',#71407,#47986,#47987);
#41599=AXIS2_PLACEMENT_3D('',#71408,#47988,#47989);
#41600=AXIS2_PLACEMENT_3D('',#71409,#47990,#47991);
#41601=AXIS2_PLACEMENT_3D('',#71411,#47992,#47993);
#41602=AXIS2_PLACEMENT_3D('',#71412,#47994,#47995);
#41603=AXIS2_PLACEMENT_3D('',#71413,#47996,#47997);
#41604=AXIS2_PLACEMENT_3D('',#71415,#47998,#47999);
#41605=AXIS2_PLACEMENT_3D('',#71420,#48000,#48001);
#41606=AXIS2_PLACEMENT_3D('',#71422,#48002,#48003);
#41607=AXIS2_PLACEMENT_3D('',#71423,#48004,#48005);
#41608=AXIS2_PLACEMENT_3D('',#71424,#48006,#48007);
#41609=AXIS2_PLACEMENT_3D('',#71426,#48008,#48009);
#41610=AXIS2_PLACEMENT_3D('',#71428,#48011,#48012);
#41611=AXIS2_PLACEMENT_3D('',#71430,#48013,#48014);
#41612=AXIS2_PLACEMENT_3D('',#71432,#48015,#48016);
#41613=AXIS2_PLACEMENT_3D('',#71456,#48018,#48019);
#41614=AXIS2_PLACEMENT_3D('',#71462,#48020,#48021);
#41615=AXIS2_PLACEMENT_3D('',#71467,#48022,#48023);
#41616=AXIS2_PLACEMENT_3D('',#71468,#48024,#48025);
#41617=AXIS2_PLACEMENT_3D('',#71469,#48026,#48027);
#41618=AXIS2_PLACEMENT_3D('',#71488,#48029,#48030);
#41619=AXIS2_PLACEMENT_3D('',#71490,#48032,#48033);
#41620=AXIS2_PLACEMENT_3D('',#71491,#48034,#48035);
#41621=AXIS2_PLACEMENT_3D('',#71492,#48036,#48037);
#41622=AXIS2_PLACEMENT_3D('',#71494,#48038,#48039);
#41623=AXIS2_PLACEMENT_3D('',#71495,#48040,#48041);
#41624=AXIS2_PLACEMENT_3D('',#71496,#48042,#48043);
#41625=AXIS2_PLACEMENT_3D('',#71498,#48044,#48045);
#41626=AXIS2_PLACEMENT_3D('',#71524,#48046,#48047);
#41627=AXIS2_PLACEMENT_3D('',#71526,#48048,#48049);
#41628=AXIS2_PLACEMENT_3D('',#71531,#48050,#48051);
#41629=AXIS2_PLACEMENT_3D('',#71532,#48052,#48053);
#41630=AXIS2_PLACEMENT_3D('',#71535,#48055,#48056);
#41631=AXIS2_PLACEMENT_3D('',#71536,#48057,#48058);
#41632=AXIS2_PLACEMENT_3D('',#71537,#48059,#48060);
#41633=AXIS2_PLACEMENT_3D('',#71538,#48061,#48062);
#41634=AXIS2_PLACEMENT_3D('',#71539,#48063,#48064);
#41635=AXIS2_PLACEMENT_3D('',#71542,#48066,#48067);
#41636=AXIS2_PLACEMENT_3D('',#71572,#48069,#48070);
#41637=AXIS2_PLACEMENT_3D('',#71574,#48071,#48072);
#41638=AXIS2_PLACEMENT_3D('',#71579,#48073,#48074);
#41639=AXIS2_PLACEMENT_3D('',#71580,#48075,#48076);
#41640=AXIS2_PLACEMENT_3D('',#71583,#48078,#48079);
#41641=AXIS2_PLACEMENT_3D('',#71584,#48080,#48081);
#41642=AXIS2_PLACEMENT_3D('',#71585,#48082,#48083);
#41643=AXIS2_PLACEMENT_3D('',#71586,#48084,#48085);
#41644=AXIS2_PLACEMENT_3D('',#71587,#48086,#48087);
#41645=AXIS2_PLACEMENT_3D('',#71590,#48089,#48090);
#41646=AXIS2_PLACEMENT_3D('',#71599,#48092,#48093);
#41647=AXIS2_PLACEMENT_3D('',#71601,#48094,#48095);
#41648=AXIS2_PLACEMENT_3D('',#71603,#48096,#48097);
#41649=AXIS2_PLACEMENT_3D('',#71627,#48099,#48100);
#41650=AXIS2_PLACEMENT_3D('',#71633,#48101,#48102);
#41651=AXIS2_PLACEMENT_3D('',#71638,#48103,#48104);
#41652=AXIS2_PLACEMENT_3D('',#71639,#48105,#48106);
#41653=AXIS2_PLACEMENT_3D('',#71640,#48107,#48108);
#41654=AXIS2_PLACEMENT_3D('',#71659,#48110,#48111);
#41655=AXIS2_PLACEMENT_3D('',#71661,#48113,#48114);
#41656=AXIS2_PLACEMENT_3D('',#71662,#48115,#48116);
#41657=AXIS2_PLACEMENT_3D('',#71663,#48117,#48118);
#41658=AXIS2_PLACEMENT_3D('',#71665,#48119,#48120);
#41659=AXIS2_PLACEMENT_3D('',#71666,#48121,#48122);
#41660=AXIS2_PLACEMENT_3D('',#71667,#48123,#48124);
#41661=AXIS2_PLACEMENT_3D('',#71669,#48125,#48126);
#41662=AXIS2_PLACEMENT_3D('',#71674,#48127,#48128);
#41663=AXIS2_PLACEMENT_3D('',#71676,#48129,#48130);
#41664=AXIS2_PLACEMENT_3D('',#71677,#48131,#48132);
#41665=AXIS2_PLACEMENT_3D('',#71678,#48133,#48134);
#41666=AXIS2_PLACEMENT_3D('',#71680,#48135,#48136);
#41667=AXIS2_PLACEMENT_3D('',#71703,#48138,#48139);
#41668=AXIS2_PLACEMENT_3D('',#71705,#48140,#48141);
#41669=AXIS2_PLACEMENT_3D('',#71710,#48142,#48143);
#41670=AXIS2_PLACEMENT_3D('',#71711,#48144,#48145);
#41671=AXIS2_PLACEMENT_3D('',#71714,#48147,#48148);
#41672=AXIS2_PLACEMENT_3D('',#71715,#48149,#48150);
#41673=AXIS2_PLACEMENT_3D('',#71716,#48151,#48152);
#41674=AXIS2_PLACEMENT_3D('',#71717,#48153,#48154);
#41675=AXIS2_PLACEMENT_3D('',#71718,#48155,#48156);
#41676=AXIS2_PLACEMENT_3D('',#71721,#48158,#48159);
#41677=AXIS2_PLACEMENT_3D('',#71730,#48161,#48162);
#41678=AXIS2_PLACEMENT_3D('',#71747,#48164,#48165);
#41679=AXIS2_PLACEMENT_3D('',#71757,#48167,#48168);
#41680=AXIS2_PLACEMENT_3D('',#71759,#48170,#48171);
#41681=AXIS2_PLACEMENT_3D('',#71776,#48173,#48174);
#41682=AXIS2_PLACEMENT_3D('',#71786,#48176,#48177);
#41683=AXIS2_PLACEMENT_3D('',#71809,#48179,#48180);
#41684=AXIS2_PLACEMENT_3D('',#71811,#48181,#48182);
#41685=AXIS2_PLACEMENT_3D('',#71816,#48183,#48184);
#41686=AXIS2_PLACEMENT_3D('',#71818,#48185,#48186);
#41687=AXIS2_PLACEMENT_3D('',#71819,#48187,#48188);
#41688=AXIS2_PLACEMENT_3D('',#71820,#48189,#48190);
#41689=AXIS2_PLACEMENT_3D('',#71821,#48191,#48192);
#41690=AXIS2_PLACEMENT_3D('',#71822,#48193,#48194);
#41691=AXIS2_PLACEMENT_3D('',#71823,#48195,#48196);
#41692=AXIS2_PLACEMENT_3D('',#71826,#48198,#48199);
#41693=AXIS2_PLACEMENT_3D('',#71827,#48200,#48201);
#41694=AXIS2_PLACEMENT_3D('',#71828,#48202,#48203);
#41695=AXIS2_PLACEMENT_3D('',#71831,#48205,#48206);
#41696=AXIS2_PLACEMENT_3D('',#71861,#48208,#48209);
#41697=AXIS2_PLACEMENT_3D('',#71863,#48210,#48211);
#41698=AXIS2_PLACEMENT_3D('',#71868,#48212,#48213);
#41699=AXIS2_PLACEMENT_3D('',#71869,#48214,#48215);
#41700=AXIS2_PLACEMENT_3D('',#71872,#48217,#48218);
#41701=AXIS2_PLACEMENT_3D('',#71873,#48219,#48220);
#41702=AXIS2_PLACEMENT_3D('',#71874,#48221,#48222);
#41703=AXIS2_PLACEMENT_3D('',#71875,#48223,#48224);
#41704=AXIS2_PLACEMENT_3D('',#71876,#48225,#48226);
#41705=AXIS2_PLACEMENT_3D('',#71879,#48228,#48229);
#41706=AXIS2_PLACEMENT_3D('',#71888,#48231,#48232);
#41707=AXIS2_PLACEMENT_3D('',#71890,#48233,#48234);
#41708=AXIS2_PLACEMENT_3D('',#71892,#48235,#48236);
#41709=AXIS2_PLACEMENT_3D('',#71916,#48238,#48239);
#41710=AXIS2_PLACEMENT_3D('',#71922,#48240,#48241);
#41711=AXIS2_PLACEMENT_3D('',#71927,#48242,#48243);
#41712=AXIS2_PLACEMENT_3D('',#71928,#48244,#48245);
#41713=AXIS2_PLACEMENT_3D('',#71929,#48246,#48247);
#41714=AXIS2_PLACEMENT_3D('',#71948,#48249,#48250);
#41715=AXIS2_PLACEMENT_3D('',#71950,#48252,#48253);
#41716=AXIS2_PLACEMENT_3D('',#71951,#48254,#48255);
#41717=AXIS2_PLACEMENT_3D('',#71952,#48256,#48257);
#41718=AXIS2_PLACEMENT_3D('',#71954,#48258,#48259);
#41719=AXIS2_PLACEMENT_3D('',#71955,#48260,#48261);
#41720=AXIS2_PLACEMENT_3D('',#71956,#48262,#48263);
#41721=AXIS2_PLACEMENT_3D('',#71958,#48264,#48265);
#41722=AXIS2_PLACEMENT_3D('',#71984,#48266,#48267);
#41723=AXIS2_PLACEMENT_3D('',#71986,#48268,#48269);
#41724=AXIS2_PLACEMENT_3D('',#71991,#48270,#48271);
#41725=AXIS2_PLACEMENT_3D('',#71992,#48272,#48273);
#41726=AXIS2_PLACEMENT_3D('',#71995,#48275,#48276);
#41727=AXIS2_PLACEMENT_3D('',#71996,#48277,#48278);
#41728=AXIS2_PLACEMENT_3D('',#71997,#48279,#48280);
#41729=AXIS2_PLACEMENT_3D('',#71998,#48281,#48282);
#41730=AXIS2_PLACEMENT_3D('',#71999,#48283,#48284);
#41731=AXIS2_PLACEMENT_3D('',#72002,#48286,#48287);
#41732=AXIS2_PLACEMENT_3D('',#72011,#48289,#48290);
#41733=AXIS2_PLACEMENT_3D('',#72013,#48291,#48292);
#41734=AXIS2_PLACEMENT_3D('',#72015,#48293,#48294);
#41735=AXIS2_PLACEMENT_3D('',#72039,#48296,#48297);
#41736=AXIS2_PLACEMENT_3D('',#72045,#48298,#48299);
#41737=AXIS2_PLACEMENT_3D('',#72050,#48300,#48301);
#41738=AXIS2_PLACEMENT_3D('',#72051,#48302,#48303);
#41739=AXIS2_PLACEMENT_3D('',#72052,#48304,#48305);
#41740=AXIS2_PLACEMENT_3D('',#72071,#48307,#48308);
#41741=AXIS2_PLACEMENT_3D('',#72073,#48310,#48311);
#41742=AXIS2_PLACEMENT_3D('',#72074,#48312,#48313);
#41743=AXIS2_PLACEMENT_3D('',#72075,#48314,#48315);
#41744=AXIS2_PLACEMENT_3D('',#72077,#48316,#48317);
#41745=AXIS2_PLACEMENT_3D('',#72078,#48318,#48319);
#41746=AXIS2_PLACEMENT_3D('',#72079,#48320,#48321);
#41747=AXIS2_PLACEMENT_3D('',#72081,#48322,#48323);
#41748=AXIS2_PLACEMENT_3D('',#72086,#48324,#48325);
#41749=AXIS2_PLACEMENT_3D('',#72088,#48326,#48327);
#41750=AXIS2_PLACEMENT_3D('',#72089,#48328,#48329);
#41751=AXIS2_PLACEMENT_3D('',#72090,#48330,#48331);
#41752=AXIS2_PLACEMENT_3D('',#72092,#48332,#48333);
#41753=AXIS2_PLACEMENT_3D('',#72115,#48335,#48336);
#41754=AXIS2_PLACEMENT_3D('',#72117,#48337,#48338);
#41755=AXIS2_PLACEMENT_3D('',#72122,#48339,#48340);
#41756=AXIS2_PLACEMENT_3D('',#72123,#48341,#48342);
#41757=AXIS2_PLACEMENT_3D('',#72126,#48344,#48345);
#41758=AXIS2_PLACEMENT_3D('',#72127,#48346,#48347);
#41759=AXIS2_PLACEMENT_3D('',#72128,#48348,#48349);
#41760=AXIS2_PLACEMENT_3D('',#72129,#48350,#48351);
#41761=AXIS2_PLACEMENT_3D('',#72130,#48352,#48353);
#41762=AXIS2_PLACEMENT_3D('',#72133,#48355,#48356);
#41763=AXIS2_PLACEMENT_3D('',#72142,#48358,#48359);
#41764=AXIS2_PLACEMENT_3D('',#72159,#48361,#48362);
#41765=AXIS2_PLACEMENT_3D('',#72169,#48364,#48365);
#41766=AXIS2_PLACEMENT_3D('',#72192,#48367,#48368);
#41767=AXIS2_PLACEMENT_3D('',#72194,#48369,#48370);
#41768=AXIS2_PLACEMENT_3D('',#72199,#48371,#48372);
#41769=AXIS2_PLACEMENT_3D('',#72201,#48373,#48374);
#41770=AXIS2_PLACEMENT_3D('',#72202,#48375,#48376);
#41771=AXIS2_PLACEMENT_3D('',#72203,#48377,#48378);
#41772=AXIS2_PLACEMENT_3D('',#72204,#48379,#48380);
#41773=AXIS2_PLACEMENT_3D('',#72205,#48381,#48382);
#41774=AXIS2_PLACEMENT_3D('',#72206,#48383,#48384);
#41775=AXIS2_PLACEMENT_3D('',#72209,#48386,#48387);
#41776=AXIS2_PLACEMENT_3D('',#72210,#48388,#48389);
#41777=AXIS2_PLACEMENT_3D('',#72211,#48390,#48391);
#41778=AXIS2_PLACEMENT_3D('',#72214,#48393,#48394);
#41779=AXIS2_PLACEMENT_3D('',#72223,#48396,#48397);
#41780=AXIS2_PLACEMENT_3D('',#72240,#48399,#48400);
#41781=AXIS2_PLACEMENT_3D('',#72250,#48402,#48403);
#41782=AXIS2_PLACEMENT_3D('',#72252,#48405,#48406);
#41783=AXIS2_PLACEMENT_3D('',#72254,#48407,#48408);
#41784=AXIS2_PLACEMENT_3D('',#72256,#48409,#48410);
#41785=AXIS2_PLACEMENT_3D('',#72280,#48412,#48413);
#41786=AXIS2_PLACEMENT_3D('',#72286,#48414,#48415);
#41787=AXIS2_PLACEMENT_3D('',#72291,#48416,#48417);
#41788=AXIS2_PLACEMENT_3D('',#72292,#48418,#48419);
#41789=AXIS2_PLACEMENT_3D('',#72293,#48420,#48421);
#41790=AXIS2_PLACEMENT_3D('',#72312,#48423,#48424);
#41791=AXIS2_PLACEMENT_3D('',#72314,#48426,#48427);
#41792=AXIS2_PLACEMENT_3D('',#72315,#48428,#48429);
#41793=AXIS2_PLACEMENT_3D('',#72316,#48430,#48431);
#41794=AXIS2_PLACEMENT_3D('',#72318,#48432,#48433);
#41795=AXIS2_PLACEMENT_3D('',#72319,#48434,#48435);
#41796=AXIS2_PLACEMENT_3D('',#72320,#48436,#48437);
#41797=AXIS2_PLACEMENT_3D('',#72322,#48438,#48439);
#41798=AXIS2_PLACEMENT_3D('',#72327,#48440,#48441);
#41799=AXIS2_PLACEMENT_3D('',#72329,#48442,#48443);
#41800=AXIS2_PLACEMENT_3D('',#72330,#48444,#48445);
#41801=AXIS2_PLACEMENT_3D('',#72331,#48446,#48447);
#41802=AXIS2_PLACEMENT_3D('',#72333,#48448,#48449);
#41803=AXIS2_PLACEMENT_3D('',#72335,#48451,#48452);
#41804=AXIS2_PLACEMENT_3D('',#72337,#48453,#48454);
#41805=AXIS2_PLACEMENT_3D('',#72339,#48455,#48456);
#41806=AXIS2_PLACEMENT_3D('',#72363,#48458,#48459);
#41807=AXIS2_PLACEMENT_3D('',#72369,#48460,#48461);
#41808=AXIS2_PLACEMENT_3D('',#72374,#48462,#48463);
#41809=AXIS2_PLACEMENT_3D('',#72375,#48464,#48465);
#41810=AXIS2_PLACEMENT_3D('',#72376,#48466,#48467);
#41811=AXIS2_PLACEMENT_3D('',#72395,#48469,#48470);
#41812=AXIS2_PLACEMENT_3D('',#72397,#48472,#48473);
#41813=AXIS2_PLACEMENT_3D('',#72398,#48474,#48475);
#41814=AXIS2_PLACEMENT_3D('',#72399,#48476,#48477);
#41815=AXIS2_PLACEMENT_3D('',#72401,#48478,#48479);
#41816=AXIS2_PLACEMENT_3D('',#72402,#48480,#48481);
#41817=AXIS2_PLACEMENT_3D('',#72403,#48482,#48483);
#41818=AXIS2_PLACEMENT_3D('',#72405,#48484,#48485);
#41819=AXIS2_PLACEMENT_3D('',#72410,#48486,#48487);
#41820=AXIS2_PLACEMENT_3D('',#72412,#48488,#48489);
#41821=AXIS2_PLACEMENT_3D('',#72413,#48490,#48491);
#41822=AXIS2_PLACEMENT_3D('',#72414,#48492,#48493);
#41823=AXIS2_PLACEMENT_3D('',#72416,#48494,#48495);
#41824=AXIS2_PLACEMENT_3D('',#72418,#48497,#48498);
#41825=AXIS2_PLACEMENT_3D('',#72420,#48499,#48500);
#41826=AXIS2_PLACEMENT_3D('',#72422,#48501,#48502);
#41827=AXIS2_PLACEMENT_3D('',#72446,#48504,#48505);
#41828=AXIS2_PLACEMENT_3D('',#72452,#48506,#48507);
#41829=AXIS2_PLACEMENT_3D('',#72457,#48508,#48509);
#41830=AXIS2_PLACEMENT_3D('',#72458,#48510,#48511);
#41831=AXIS2_PLACEMENT_3D('',#72459,#48512,#48513);
#41832=AXIS2_PLACEMENT_3D('',#72478,#48515,#48516);
#41833=AXIS2_PLACEMENT_3D('',#72480,#48518,#48519);
#41834=AXIS2_PLACEMENT_3D('',#72481,#48520,#48521);
#41835=AXIS2_PLACEMENT_3D('',#72482,#48522,#48523);
#41836=AXIS2_PLACEMENT_3D('',#72484,#48524,#48525);
#41837=AXIS2_PLACEMENT_3D('',#72485,#48526,#48527);
#41838=AXIS2_PLACEMENT_3D('',#72486,#48528,#48529);
#41839=AXIS2_PLACEMENT_3D('',#72488,#48530,#48531);
#41840=AXIS2_PLACEMENT_3D('',#72493,#48532,#48533);
#41841=AXIS2_PLACEMENT_3D('',#72495,#48534,#48535);
#41842=AXIS2_PLACEMENT_3D('',#72497,#48536,#48537);
#41843=AXIS2_PLACEMENT_3D('',#72521,#48539,#48540);
#41844=AXIS2_PLACEMENT_3D('',#72527,#48541,#48542);
#41845=AXIS2_PLACEMENT_3D('',#72532,#48543,#48544);
#41846=AXIS2_PLACEMENT_3D('',#72533,#48545,#48546);
#41847=AXIS2_PLACEMENT_3D('',#72534,#48547,#48548);
#41848=AXIS2_PLACEMENT_3D('',#72553,#48550,#48551);
#41849=AXIS2_PLACEMENT_3D('',#72555,#48553,#48554);
#41850=AXIS2_PLACEMENT_3D('',#72556,#48555,#48556);
#41851=AXIS2_PLACEMENT_3D('',#72557,#48557,#48558);
#41852=AXIS2_PLACEMENT_3D('',#72559,#48559,#48560);
#41853=AXIS2_PLACEMENT_3D('',#72560,#48561,#48562);
#41854=AXIS2_PLACEMENT_3D('',#72561,#48563,#48564);
#41855=AXIS2_PLACEMENT_3D('',#72563,#48565,#48566);
#41856=AXIS2_PLACEMENT_3D('',#72568,#48567,#48568);
#41857=AXIS2_PLACEMENT_3D('',#72570,#48569,#48570);
#41858=AXIS2_PLACEMENT_3D('',#72571,#48571,#48572);
#41859=AXIS2_PLACEMENT_3D('',#72572,#48573,#48574);
#41860=AXIS2_PLACEMENT_3D('',#72574,#48575,#48576);
#41861=AXIS2_PLACEMENT_3D('',#72597,#48578,#48579);
#41862=AXIS2_PLACEMENT_3D('',#72599,#48580,#48581);
#41863=AXIS2_PLACEMENT_3D('',#72604,#48582,#48583);
#41864=AXIS2_PLACEMENT_3D('',#72605,#48584,#48585);
#41865=AXIS2_PLACEMENT_3D('',#72608,#48587,#48588);
#41866=AXIS2_PLACEMENT_3D('',#72609,#48589,#48590);
#41867=AXIS2_PLACEMENT_3D('',#72610,#48591,#48592);
#41868=AXIS2_PLACEMENT_3D('',#72611,#48593,#48594);
#41869=AXIS2_PLACEMENT_3D('',#72612,#48595,#48596);
#41870=AXIS2_PLACEMENT_3D('',#72615,#48598,#48599);
#41871=AXIS2_PLACEMENT_3D('',#72645,#48601,#48602);
#41872=AXIS2_PLACEMENT_3D('',#72647,#48603,#48604);
#41873=AXIS2_PLACEMENT_3D('',#72652,#48605,#48606);
#41874=AXIS2_PLACEMENT_3D('',#72654,#48607,#48608);
#41875=AXIS2_PLACEMENT_3D('',#72655,#48609,#48610);
#41876=AXIS2_PLACEMENT_3D('',#72656,#48611,#48612);
#41877=AXIS2_PLACEMENT_3D('',#72657,#48613,#48614);
#41878=AXIS2_PLACEMENT_3D('',#72658,#48615,#48616);
#41879=AXIS2_PLACEMENT_3D('',#72659,#48617,#48618);
#41880=AXIS2_PLACEMENT_3D('',#72662,#48620,#48621);
#41881=AXIS2_PLACEMENT_3D('',#72663,#48622,#48623);
#41882=AXIS2_PLACEMENT_3D('',#72664,#48624,#48625);
#41883=AXIS2_PLACEMENT_3D('',#72667,#48627,#48628);
#41884=AXIS2_PLACEMENT_3D('',#72676,#48630,#48631);
#41885=AXIS2_PLACEMENT_3D('',#72678,#48632,#48633);
#41886=AXIS2_PLACEMENT_3D('',#72680,#48634,#48635);
#41887=AXIS2_PLACEMENT_3D('',#72704,#48637,#48638);
#41888=AXIS2_PLACEMENT_3D('',#72710,#48639,#48640);
#41889=AXIS2_PLACEMENT_3D('',#72715,#48641,#48642);
#41890=AXIS2_PLACEMENT_3D('',#72716,#48643,#48644);
#41891=AXIS2_PLACEMENT_3D('',#72717,#48645,#48646);
#41892=AXIS2_PLACEMENT_3D('',#72736,#48648,#48649);
#41893=AXIS2_PLACEMENT_3D('',#72738,#48651,#48652);
#41894=AXIS2_PLACEMENT_3D('',#72739,#48653,#48654);
#41895=AXIS2_PLACEMENT_3D('',#72740,#48655,#48656);
#41896=AXIS2_PLACEMENT_3D('',#72742,#48657,#48658);
#41897=AXIS2_PLACEMENT_3D('',#72743,#48659,#48660);
#41898=AXIS2_PLACEMENT_3D('',#72744,#48661,#48662);
#41899=AXIS2_PLACEMENT_3D('',#72746,#48663,#48664);
#41900=AXIS2_PLACEMENT_3D('',#72751,#48665,#48666);
#41901=AXIS2_PLACEMENT_3D('',#72753,#48667,#48668);
#41902=AXIS2_PLACEMENT_3D('',#72754,#48669,#48670);
#41903=AXIS2_PLACEMENT_3D('',#72755,#48671,#48672);
#41904=AXIS2_PLACEMENT_3D('',#72757,#48673,#48674);
#41905=AXIS2_PLACEMENT_3D('',#72759,#48676,#48677);
#41906=AXIS2_PLACEMENT_3D('',#72761,#48678,#48679);
#41907=AXIS2_PLACEMENT_3D('',#72763,#48680,#48681);
#41908=AXIS2_PLACEMENT_3D('',#72787,#48683,#48684);
#41909=AXIS2_PLACEMENT_3D('',#72793,#48685,#48686);
#41910=AXIS2_PLACEMENT_3D('',#72798,#48687,#48688);
#41911=AXIS2_PLACEMENT_3D('',#72799,#48689,#48690);
#41912=AXIS2_PLACEMENT_3D('',#72800,#48691,#48692);
#41913=AXIS2_PLACEMENT_3D('',#72819,#48694,#48695);
#41914=AXIS2_PLACEMENT_3D('',#72821,#48697,#48698);
#41915=AXIS2_PLACEMENT_3D('',#72822,#48699,#48700);
#41916=AXIS2_PLACEMENT_3D('',#72823,#48701,#48702);
#41917=AXIS2_PLACEMENT_3D('',#72825,#48703,#48704);
#41918=AXIS2_PLACEMENT_3D('',#72826,#48705,#48706);
#41919=AXIS2_PLACEMENT_3D('',#72827,#48707,#48708);
#41920=AXIS2_PLACEMENT_3D('',#72829,#48709,#48710);
#41921=AXIS2_PLACEMENT_3D('',#72855,#48711,#48712);
#41922=AXIS2_PLACEMENT_3D('',#72857,#48713,#48714);
#41923=AXIS2_PLACEMENT_3D('',#72862,#48715,#48716);
#41924=AXIS2_PLACEMENT_3D('',#72863,#48717,#48718);
#41925=AXIS2_PLACEMENT_3D('',#72866,#48720,#48721);
#41926=AXIS2_PLACEMENT_3D('',#72867,#48722,#48723);
#41927=AXIS2_PLACEMENT_3D('',#72868,#48724,#48725);
#41928=AXIS2_PLACEMENT_3D('',#72869,#48726,#48727);
#41929=AXIS2_PLACEMENT_3D('',#72870,#48728,#48729);
#41930=AXIS2_PLACEMENT_3D('',#72873,#48731,#48732);
#41931=AXIS2_PLACEMENT_3D('',#72903,#48734,#48735);
#41932=AXIS2_PLACEMENT_3D('',#72905,#48736,#48737);
#41933=AXIS2_PLACEMENT_3D('',#72910,#48738,#48739);
#41934=AXIS2_PLACEMENT_3D('',#72911,#48740,#48741);
#41935=AXIS2_PLACEMENT_3D('',#72914,#48743,#48744);
#41936=AXIS2_PLACEMENT_3D('',#72915,#48745,#48746);
#41937=AXIS2_PLACEMENT_3D('',#72916,#48747,#48748);
#41938=AXIS2_PLACEMENT_3D('',#72917,#48749,#48750);
#41939=AXIS2_PLACEMENT_3D('',#72918,#48751,#48752);
#41940=AXIS2_PLACEMENT_3D('',#72921,#48754,#48755);
#41941=AXIS2_PLACEMENT_3D('',#72930,#48757,#48758);
#41942=AXIS2_PLACEMENT_3D('',#72932,#48759,#48760);
#41943=AXIS2_PLACEMENT_3D('',#72934,#48761,#48762);
#41944=AXIS2_PLACEMENT_3D('',#72958,#48764,#48765);
#41945=AXIS2_PLACEMENT_3D('',#72964,#48766,#48767);
#41946=AXIS2_PLACEMENT_3D('',#72969,#48768,#48769);
#41947=AXIS2_PLACEMENT_3D('',#72970,#48770,#48771);
#41948=AXIS2_PLACEMENT_3D('',#72971,#48772,#48773);
#41949=AXIS2_PLACEMENT_3D('',#72990,#48775,#48776);
#41950=AXIS2_PLACEMENT_3D('',#72992,#48778,#48779);
#41951=AXIS2_PLACEMENT_3D('',#72993,#48780,#48781);
#41952=AXIS2_PLACEMENT_3D('',#72994,#48782,#48783);
#41953=AXIS2_PLACEMENT_3D('',#72996,#48784,#48785);
#41954=AXIS2_PLACEMENT_3D('',#72997,#48786,#48787);
#41955=AXIS2_PLACEMENT_3D('',#72998,#48788,#48789);
#41956=AXIS2_PLACEMENT_3D('',#73000,#48790,#48791);
#41957=AXIS2_PLACEMENT_3D('',#73005,#48792,#48793);
#41958=AXIS2_PLACEMENT_3D('',#73007,#48794,#48795);
#41959=AXIS2_PLACEMENT_3D('',#73008,#48796,#48797);
#41960=AXIS2_PLACEMENT_3D('',#73009,#48798,#48799);
#41961=AXIS2_PLACEMENT_3D('',#73011,#48800,#48801);
#41962=AXIS2_PLACEMENT_3D('',#73034,#48803,#48804);
#41963=AXIS2_PLACEMENT_3D('',#73036,#48805,#48806);
#41964=AXIS2_PLACEMENT_3D('',#73041,#48807,#48808);
#41965=AXIS2_PLACEMENT_3D('',#73042,#48809,#48810);
#41966=AXIS2_PLACEMENT_3D('',#73045,#48812,#48813);
#41967=AXIS2_PLACEMENT_3D('',#73046,#48814,#48815);
#41968=AXIS2_PLACEMENT_3D('',#73047,#48816,#48817);
#41969=AXIS2_PLACEMENT_3D('',#73048,#48818,#48819);
#41970=AXIS2_PLACEMENT_3D('',#73049,#48820,#48821);
#41971=AXIS2_PLACEMENT_3D('',#73066,#48823,#48824);
#41972=AXIS2_PLACEMENT_3D('',#73076,#48826,#48827);
#41973=AXIS2_PLACEMENT_3D('',#73099,#48829,#48830);
#41974=AXIS2_PLACEMENT_3D('',#73101,#48831,#48832);
#41975=AXIS2_PLACEMENT_3D('',#73106,#48833,#48834);
#41976=AXIS2_PLACEMENT_3D('',#73107,#48835,#48836);
#41977=AXIS2_PLACEMENT_3D('',#73110,#48838,#48839);
#41978=AXIS2_PLACEMENT_3D('',#73111,#48840,#48841);
#41979=AXIS2_PLACEMENT_3D('',#73112,#48842,#48843);
#41980=AXIS2_PLACEMENT_3D('',#73113,#48844,#48845);
#41981=AXIS2_PLACEMENT_3D('',#73114,#48846,#48847);
#41982=AXIS2_PLACEMENT_3D('',#73117,#48849,#48850);
#41983=AXIS2_PLACEMENT_3D('',#73126,#48852,#48853);
#41984=AXIS2_PLACEMENT_3D('',#73143,#48855,#48856);
#41985=AXIS2_PLACEMENT_3D('',#73153,#48858,#48859);
#41986=AXIS2_PLACEMENT_3D('',#73155,#48861,#48862);
#41987=AXIS2_PLACEMENT_3D('',#73172,#48864,#48865);
#41988=AXIS2_PLACEMENT_3D('',#73182,#48867,#48868);
#41989=AXIS2_PLACEMENT_3D('',#73205,#48870,#48871);
#41990=AXIS2_PLACEMENT_3D('',#73207,#48872,#48873);
#41991=AXIS2_PLACEMENT_3D('',#73212,#48874,#48875);
#41992=AXIS2_PLACEMENT_3D('',#73214,#48876,#48877);
#41993=AXIS2_PLACEMENT_3D('',#73215,#48878,#48879);
#41994=AXIS2_PLACEMENT_3D('',#73216,#48880,#48881);
#41995=AXIS2_PLACEMENT_3D('',#73217,#48882,#48883);
#41996=AXIS2_PLACEMENT_3D('',#73218,#48884,#48885);
#41997=AXIS2_PLACEMENT_3D('',#73219,#48886,#48887);
#41998=AXIS2_PLACEMENT_3D('',#73222,#48889,#48890);
#41999=AXIS2_PLACEMENT_3D('',#73223,#48891,#48892);
#42000=AXIS2_PLACEMENT_3D('',#73224,#48893,#48894);
#42001=AXIS2_PLACEMENT_3D('',#73227,#48896,#48897);
#42002=AXIS2_PLACEMENT_3D('',#73257,#48899,#48900);
#42003=AXIS2_PLACEMENT_3D('',#73259,#48901,#48902);
#42004=AXIS2_PLACEMENT_3D('',#73264,#48903,#48904);
#42005=AXIS2_PLACEMENT_3D('',#73265,#48905,#48906);
#42006=AXIS2_PLACEMENT_3D('',#73268,#48908,#48909);
#42007=AXIS2_PLACEMENT_3D('',#73269,#48910,#48911);
#42008=AXIS2_PLACEMENT_3D('',#73270,#48912,#48913);
#42009=AXIS2_PLACEMENT_3D('',#73271,#48914,#48915);
#42010=AXIS2_PLACEMENT_3D('',#73272,#48916,#48917);
#42011=AXIS2_PLACEMENT_3D('',#73275,#48919,#48920);
#42012=AXIS2_PLACEMENT_3D('',#73284,#48922,#48923);
#42013=AXIS2_PLACEMENT_3D('',#73286,#48924,#48925);
#42014=AXIS2_PLACEMENT_3D('',#73288,#48926,#48927);
#42015=AXIS2_PLACEMENT_3D('',#73312,#48929,#48930);
#42016=AXIS2_PLACEMENT_3D('',#73318,#48931,#48932);
#42017=AXIS2_PLACEMENT_3D('',#73323,#48933,#48934);
#42018=AXIS2_PLACEMENT_3D('',#73324,#48935,#48936);
#42019=AXIS2_PLACEMENT_3D('',#73325,#48937,#48938);
#42020=AXIS2_PLACEMENT_3D('',#73344,#48940,#48941);
#42021=AXIS2_PLACEMENT_3D('',#73346,#48943,#48944);
#42022=AXIS2_PLACEMENT_3D('',#73347,#48945,#48946);
#42023=AXIS2_PLACEMENT_3D('',#73348,#48947,#48948);
#42024=AXIS2_PLACEMENT_3D('',#73350,#48949,#48950);
#42025=AXIS2_PLACEMENT_3D('',#73351,#48951,#48952);
#42026=AXIS2_PLACEMENT_3D('',#73352,#48953,#48954);
#42027=AXIS2_PLACEMENT_3D('',#73354,#48955,#48956);
#42028=AXIS2_PLACEMENT_3D('',#73359,#48957,#48958);
#42029=AXIS2_PLACEMENT_3D('',#73361,#48959,#48960);
#42030=AXIS2_PLACEMENT_3D('',#73362,#48961,#48962);
#42031=AXIS2_PLACEMENT_3D('',#73363,#48963,#48964);
#42032=AXIS2_PLACEMENT_3D('',#73365,#48965,#48966);
#42033=AXIS2_PLACEMENT_3D('',#73388,#48968,#48969);
#42034=AXIS2_PLACEMENT_3D('',#73390,#48970,#48971);
#42035=AXIS2_PLACEMENT_3D('',#73395,#48972,#48973);
#42036=AXIS2_PLACEMENT_3D('',#73396,#48974,#48975);
#42037=AXIS2_PLACEMENT_3D('',#73399,#48977,#48978);
#42038=AXIS2_PLACEMENT_3D('',#73400,#48979,#48980);
#42039=AXIS2_PLACEMENT_3D('',#73401,#48981,#48982);
#42040=AXIS2_PLACEMENT_3D('',#73402,#48983,#48984);
#42041=AXIS2_PLACEMENT_3D('',#73403,#48985,#48986);
#42042=AXIS2_PLACEMENT_3D('',#73420,#48988,#48989);
#42043=AXIS2_PLACEMENT_3D('',#73430,#48991,#48992);
#42044=AXIS2_PLACEMENT_3D('',#73432,#48994,#48995);
#42045=AXIS2_PLACEMENT_3D('',#73434,#48996,#48997);
#42046=AXIS2_PLACEMENT_3D('',#73436,#48998,#48999);
#42047=AXIS2_PLACEMENT_3D('',#73460,#49001,#49002);
#42048=AXIS2_PLACEMENT_3D('',#73466,#49003,#49004);
#42049=AXIS2_PLACEMENT_3D('',#73471,#49005,#49006);
#42050=AXIS2_PLACEMENT_3D('',#73472,#49007,#49008);
#42051=AXIS2_PLACEMENT_3D('',#73473,#49009,#49010);
#42052=AXIS2_PLACEMENT_3D('',#73492,#49012,#49013);
#42053=AXIS2_PLACEMENT_3D('',#73494,#49015,#49016);
#42054=AXIS2_PLACEMENT_3D('',#73495,#49017,#49018);
#42055=AXIS2_PLACEMENT_3D('',#73496,#49019,#49020);
#42056=AXIS2_PLACEMENT_3D('',#73498,#49021,#49022);
#42057=AXIS2_PLACEMENT_3D('',#73499,#49023,#49024);
#42058=AXIS2_PLACEMENT_3D('',#73500,#49025,#49026);
#42059=AXIS2_PLACEMENT_3D('',#73502,#49027,#49028);
#42060=AXIS2_PLACEMENT_3D('',#73507,#49029,#49030);
#42061=AXIS2_PLACEMENT_3D('',#73509,#49031,#49032);
#42062=AXIS2_PLACEMENT_3D('',#73510,#49033,#49034);
#42063=AXIS2_PLACEMENT_3D('',#73511,#49035,#49036);
#42064=AXIS2_PLACEMENT_3D('',#73513,#49037,#49038);
#42065=AXIS2_PLACEMENT_3D('',#73515,#49040,#49041);
#42066=AXIS2_PLACEMENT_3D('',#73517,#49042,#49043);
#42067=AXIS2_PLACEMENT_3D('',#73519,#49044,#49045);
#42068=AXIS2_PLACEMENT_3D('',#73543,#49047,#49048);
#42069=AXIS2_PLACEMENT_3D('',#73549,#49049,#49050);
#42070=AXIS2_PLACEMENT_3D('',#73554,#49051,#49052);
#42071=AXIS2_PLACEMENT_3D('',#73555,#49053,#49054);
#42072=AXIS2_PLACEMENT_3D('',#73556,#49055,#49056);
#42073=AXIS2_PLACEMENT_3D('',#73575,#49058,#49059);
#42074=AXIS2_PLACEMENT_3D('',#73577,#49061,#49062);
#42075=AXIS2_PLACEMENT_3D('',#73578,#49063,#49064);
#42076=AXIS2_PLACEMENT_3D('',#73579,#49065,#49066);
#42077=AXIS2_PLACEMENT_3D('',#73581,#49067,#49068);
#42078=AXIS2_PLACEMENT_3D('',#73582,#49069,#49070);
#42079=AXIS2_PLACEMENT_3D('',#73583,#49071,#49072);
#42080=AXIS2_PLACEMENT_3D('',#73585,#49073,#49074);
#42081=AXIS2_PLACEMENT_3D('',#73590,#49075,#49076);
#42082=AXIS2_PLACEMENT_3D('',#73592,#49077,#49078);
#42083=AXIS2_PLACEMENT_3D('',#73593,#49079,#49080);
#42084=AXIS2_PLACEMENT_3D('',#73594,#49081,#49082);
#42085=AXIS2_PLACEMENT_3D('',#73596,#49083,#49084);
#42086=AXIS2_PLACEMENT_3D('',#73619,#49086,#49087);
#42087=AXIS2_PLACEMENT_3D('',#73621,#49088,#49089);
#42088=AXIS2_PLACEMENT_3D('',#73626,#49090,#49091);
#42089=AXIS2_PLACEMENT_3D('',#73627,#49092,#49093);
#42090=AXIS2_PLACEMENT_3D('',#73630,#49095,#49096);
#42091=AXIS2_PLACEMENT_3D('',#73631,#49097,#49098);
#42092=AXIS2_PLACEMENT_3D('',#73632,#49099,#49100);
#42093=AXIS2_PLACEMENT_3D('',#73633,#49101,#49102);
#42094=AXIS2_PLACEMENT_3D('',#73634,#49103,#49104);
#42095=AXIS2_PLACEMENT_3D('',#73637,#49106,#49107);
#42096=AXIS2_PLACEMENT_3D('',#73646,#49109,#49110);
#42097=AXIS2_PLACEMENT_3D('',#73648,#49111,#49112);
#42098=AXIS2_PLACEMENT_3D('',#73650,#49113,#49114);
#42099=AXIS2_PLACEMENT_3D('',#73674,#49116,#49117);
#42100=AXIS2_PLACEMENT_3D('',#73680,#49118,#49119);
#42101=AXIS2_PLACEMENT_3D('',#73685,#49120,#49121);
#42102=AXIS2_PLACEMENT_3D('',#73686,#49122,#49123);
#42103=AXIS2_PLACEMENT_3D('',#73687,#49124,#49125);
#42104=AXIS2_PLACEMENT_3D('',#73706,#49127,#49128);
#42105=AXIS2_PLACEMENT_3D('',#73708,#49130,#49131);
#42106=AXIS2_PLACEMENT_3D('',#73709,#49132,#49133);
#42107=AXIS2_PLACEMENT_3D('',#73710,#49134,#49135);
#42108=AXIS2_PLACEMENT_3D('',#73712,#49136,#49137);
#42109=AXIS2_PLACEMENT_3D('',#73713,#49138,#49139);
#42110=AXIS2_PLACEMENT_3D('',#73714,#49140,#49141);
#42111=AXIS2_PLACEMENT_3D('',#73716,#49142,#49143);
#42112=AXIS2_PLACEMENT_3D('',#73721,#49144,#49145);
#42113=AXIS2_PLACEMENT_3D('',#73723,#49146,#49147);
#42114=AXIS2_PLACEMENT_3D('',#73725,#49148,#49149);
#42115=AXIS2_PLACEMENT_3D('',#73749,#49151,#49152);
#42116=AXIS2_PLACEMENT_3D('',#73755,#49153,#49154);
#42117=AXIS2_PLACEMENT_3D('',#73760,#49155,#49156);
#42118=AXIS2_PLACEMENT_3D('',#73761,#49157,#49158);
#42119=AXIS2_PLACEMENT_3D('',#73762,#49159,#49160);
#42120=AXIS2_PLACEMENT_3D('',#73781,#49162,#49163);
#42121=AXIS2_PLACEMENT_3D('',#73783,#49165,#49166);
#42122=AXIS2_PLACEMENT_3D('',#73784,#49167,#49168);
#42123=AXIS2_PLACEMENT_3D('',#73785,#49169,#49170);
#42124=AXIS2_PLACEMENT_3D('',#73787,#49171,#49172);
#42125=AXIS2_PLACEMENT_3D('',#73788,#49173,#49174);
#42126=AXIS2_PLACEMENT_3D('',#73789,#49175,#49176);
#42127=AXIS2_PLACEMENT_3D('',#73791,#49177,#49178);
#42128=AXIS2_PLACEMENT_3D('',#73796,#49179,#49180);
#42129=AXIS2_PLACEMENT_3D('',#73798,#49181,#49182);
#42130=AXIS2_PLACEMENT_3D('',#73799,#49183,#49184);
#42131=AXIS2_PLACEMENT_3D('',#73800,#49185,#49186);
#42132=AXIS2_PLACEMENT_3D('',#73802,#49187,#49188);
#42133=AXIS2_PLACEMENT_3D('',#73824,#49190,#49191);
#42134=AXIS2_PLACEMENT_3D('',#73825,#49192,#49193);
#42135=AXIS2_PLACEMENT_3D('',#73826,#49194,#49195);
#42136=AXIS2_PLACEMENT_3D('',#73827,#49196,#49197);
#42137=AXIS2_PLACEMENT_3D('',#73828,#49198,#49199);
#42138=AXIS2_PLACEMENT_3D('',#73829,#49200,#49201);
#42139=AXIS2_PLACEMENT_3D('',#73830,#49202,#49203);
#42140=AXIS2_PLACEMENT_3D('',#73831,#49204,#49205);
#42141=AXIS2_PLACEMENT_3D('',#73833,#49206,#49207);
#42142=AXIS2_PLACEMENT_3D('',#73835,#49208,#49209);
#42143=AXIS2_PLACEMENT_3D('',#73859,#49211,#49212);
#42144=AXIS2_PLACEMENT_3D('',#73865,#49213,#49214);
#42145=AXIS2_PLACEMENT_3D('',#73870,#49215,#49216);
#42146=AXIS2_PLACEMENT_3D('',#73871,#49217,#49218);
#42147=AXIS2_PLACEMENT_3D('',#73872,#49219,#49220);
#42148=AXIS2_PLACEMENT_3D('',#73891,#49222,#49223);
#42149=AXIS2_PLACEMENT_3D('',#73893,#49225,#49226);
#42150=AXIS2_PLACEMENT_3D('',#73894,#49227,#49228);
#42151=AXIS2_PLACEMENT_3D('',#73895,#49229,#49230);
#42152=AXIS2_PLACEMENT_3D('',#73897,#49231,#49232);
#42153=AXIS2_PLACEMENT_3D('',#73898,#49233,#49234);
#42154=AXIS2_PLACEMENT_3D('',#73899,#49235,#49236);
#42155=AXIS2_PLACEMENT_3D('',#73901,#49237,#49238);
#42156=AXIS2_PLACEMENT_3D('',#73927,#49239,#49240);
#42157=AXIS2_PLACEMENT_3D('',#73929,#49241,#49242);
#42158=AXIS2_PLACEMENT_3D('',#73934,#49243,#49244);
#42159=AXIS2_PLACEMENT_3D('',#73936,#49245,#49246);
#42160=AXIS2_PLACEMENT_3D('',#73937,#49247,#49248);
#42161=AXIS2_PLACEMENT_3D('',#73938,#49249,#49250);
#42162=AXIS2_PLACEMENT_3D('',#73939,#49251,#49252);
#42163=AXIS2_PLACEMENT_3D('',#73940,#49253,#49254);
#42164=AXIS2_PLACEMENT_3D('',#73941,#49255,#49256);
#42165=AXIS2_PLACEMENT_3D('',#73944,#49258,#49259);
#42166=AXIS2_PLACEMENT_3D('',#73945,#49260,#49261);
#42167=AXIS2_PLACEMENT_3D('',#73946,#49262,#49263);
#42168=AXIS2_PLACEMENT_3D('',#73949,#49265,#49266);
#42169=AXIS2_PLACEMENT_3D('',#73979,#49268,#49269);
#42170=AXIS2_PLACEMENT_3D('',#73981,#49270,#49271);
#42171=AXIS2_PLACEMENT_3D('',#73986,#49272,#49273);
#42172=AXIS2_PLACEMENT_3D('',#73987,#49274,#49275);
#42173=AXIS2_PLACEMENT_3D('',#73990,#49277,#49278);
#42174=AXIS2_PLACEMENT_3D('',#73991,#49279,#49280);
#42175=AXIS2_PLACEMENT_3D('',#73992,#49281,#49282);
#42176=AXIS2_PLACEMENT_3D('',#73993,#49283,#49284);
#42177=AXIS2_PLACEMENT_3D('',#73994,#49285,#49286);
#42178=AXIS2_PLACEMENT_3D('',#73997,#49288,#49289);
#42179=AXIS2_PLACEMENT_3D('',#74027,#49291,#49292);
#42180=AXIS2_PLACEMENT_3D('',#74029,#49293,#49294);
#42181=AXIS2_PLACEMENT_3D('',#74034,#49295,#49296);
#42182=AXIS2_PLACEMENT_3D('',#74036,#49297,#49298);
#42183=AXIS2_PLACEMENT_3D('',#74037,#49299,#49300);
#42184=AXIS2_PLACEMENT_3D('',#74038,#49301,#49302);
#42185=AXIS2_PLACEMENT_3D('',#74039,#49303,#49304);
#42186=AXIS2_PLACEMENT_3D('',#74040,#49305,#49306);
#42187=AXIS2_PLACEMENT_3D('',#74041,#49307,#49308);
#42188=AXIS2_PLACEMENT_3D('',#74044,#49310,#49311);
#42189=AXIS2_PLACEMENT_3D('',#74045,#49312,#49313);
#42190=AXIS2_PLACEMENT_3D('',#74046,#49314,#49315);
#42191=AXIS2_PLACEMENT_3D('',#74049,#49317,#49318);
#42192=AXIS2_PLACEMENT_3D('',#74058,#49320,#49321);
#42193=AXIS2_PLACEMENT_3D('',#74075,#49323,#49324);
#42194=AXIS2_PLACEMENT_3D('',#74085,#49326,#49327);
#42195=AXIS2_PLACEMENT_3D('',#74108,#49329,#49330);
#42196=AXIS2_PLACEMENT_3D('',#74110,#49331,#49332);
#42197=AXIS2_PLACEMENT_3D('',#74115,#49333,#49334);
#42198=AXIS2_PLACEMENT_3D('',#74116,#49335,#49336);
#42199=AXIS2_PLACEMENT_3D('',#74119,#49338,#49339);
#42200=AXIS2_PLACEMENT_3D('',#74120,#49340,#49341);
#42201=AXIS2_PLACEMENT_3D('',#74121,#49342,#49343);
#42202=AXIS2_PLACEMENT_3D('',#74122,#49344,#49345);
#42203=AXIS2_PLACEMENT_3D('',#74123,#49346,#49347);
#42204=AXIS2_PLACEMENT_3D('',#74126,#49349,#49350);
#42205=AXIS2_PLACEMENT_3D('',#74156,#49352,#49353);
#42206=AXIS2_PLACEMENT_3D('',#74158,#49354,#49355);
#42207=AXIS2_PLACEMENT_3D('',#74163,#49356,#49357);
#42208=AXIS2_PLACEMENT_3D('',#74164,#49358,#49359);
#42209=AXIS2_PLACEMENT_3D('',#74167,#49361,#49362);
#42210=AXIS2_PLACEMENT_3D('',#74168,#49363,#49364);
#42211=AXIS2_PLACEMENT_3D('',#74169,#49365,#49366);
#42212=AXIS2_PLACEMENT_3D('',#74170,#49367,#49368);
#42213=AXIS2_PLACEMENT_3D('',#74171,#49369,#49370);
#42214=AXIS2_PLACEMENT_3D('',#74174,#49372,#49373);
#42215=AXIS2_PLACEMENT_3D('',#74183,#49375,#49376);
#42216=AXIS2_PLACEMENT_3D('',#74185,#49377,#49378);
#42217=AXIS2_PLACEMENT_3D('',#74187,#49379,#49380);
#42218=AXIS2_PLACEMENT_3D('',#74211,#49382,#49383);
#42219=AXIS2_PLACEMENT_3D('',#74217,#49384,#49385);
#42220=AXIS2_PLACEMENT_3D('',#74222,#49386,#49387);
#42221=AXIS2_PLACEMENT_3D('',#74223,#49388,#49389);
#42222=AXIS2_PLACEMENT_3D('',#74224,#49390,#49391);
#42223=AXIS2_PLACEMENT_3D('',#74243,#49393,#49394);
#42224=AXIS2_PLACEMENT_3D('',#74245,#49396,#49397);
#42225=AXIS2_PLACEMENT_3D('',#74246,#49398,#49399);
#42226=AXIS2_PLACEMENT_3D('',#74247,#49400,#49401);
#42227=AXIS2_PLACEMENT_3D('',#74249,#49402,#49403);
#42228=AXIS2_PLACEMENT_3D('',#74250,#49404,#49405);
#42229=AXIS2_PLACEMENT_3D('',#74251,#49406,#49407);
#42230=AXIS2_PLACEMENT_3D('',#74253,#49408,#49409);
#42231=AXIS2_PLACEMENT_3D('',#74258,#49410,#49411);
#42232=AXIS2_PLACEMENT_3D('',#74260,#49412,#49413);
#42233=AXIS2_PLACEMENT_3D('',#74261,#49414,#49415);
#42234=AXIS2_PLACEMENT_3D('',#74262,#49416,#49417);
#42235=AXIS2_PLACEMENT_3D('',#74264,#49418,#49419);
#42236=AXIS2_PLACEMENT_3D('',#74287,#49421,#49422);
#42237=AXIS2_PLACEMENT_3D('',#74289,#49423,#49424);
#42238=AXIS2_PLACEMENT_3D('',#74294,#49425,#49426);
#42239=AXIS2_PLACEMENT_3D('',#74295,#49427,#49428);
#42240=AXIS2_PLACEMENT_3D('',#74298,#49430,#49431);
#42241=AXIS2_PLACEMENT_3D('',#74299,#49432,#49433);
#42242=AXIS2_PLACEMENT_3D('',#74300,#49434,#49435);
#42243=AXIS2_PLACEMENT_3D('',#74301,#49436,#49437);
#42244=AXIS2_PLACEMENT_3D('',#74302,#49438,#49439);
#42245=AXIS2_PLACEMENT_3D('',#74305,#49441,#49442);
#42246=AXIS2_PLACEMENT_3D('',#74314,#49444,#49445);
#42247=AXIS2_PLACEMENT_3D('',#74331,#49447,#49448);
#42248=AXIS2_PLACEMENT_3D('',#74341,#49450,#49451);
#42249=AXIS2_PLACEMENT_3D('',#74343,#49453,#49454);
#42250=AXIS2_PLACEMENT_3D('',#74360,#49456,#49457);
#42251=AXIS2_PLACEMENT_3D('',#74370,#49459,#49460);
#42252=AXIS2_PLACEMENT_3D('',#74372,#49462,#49463);
#42253=AXIS2_PLACEMENT_3D('',#74374,#49464,#49465);
#42254=AXIS2_PLACEMENT_3D('',#74376,#49466,#49467);
#42255=AXIS2_PLACEMENT_3D('',#74400,#49469,#49470);
#42256=AXIS2_PLACEMENT_3D('',#74406,#49471,#49472);
#42257=AXIS2_PLACEMENT_3D('',#74411,#49473,#49474);
#42258=AXIS2_PLACEMENT_3D('',#74412,#49475,#49476);
#42259=AXIS2_PLACEMENT_3D('',#74413,#49477,#49478);
#42260=AXIS2_PLACEMENT_3D('',#74432,#49480,#49481);
#42261=AXIS2_PLACEMENT_3D('',#74434,#49483,#49484);
#42262=AXIS2_PLACEMENT_3D('',#74435,#49485,#49486);
#42263=AXIS2_PLACEMENT_3D('',#74436,#49487,#49488);
#42264=AXIS2_PLACEMENT_3D('',#74438,#49489,#49490);
#42265=AXIS2_PLACEMENT_3D('',#74439,#49491,#49492);
#42266=AXIS2_PLACEMENT_3D('',#74440,#49493,#49494);
#42267=AXIS2_PLACEMENT_3D('',#74442,#49495,#49496);
#42268=AXIS2_PLACEMENT_3D('',#74447,#49497,#49498);
#42269=AXIS2_PLACEMENT_3D('',#74449,#49499,#49500);
#42270=AXIS2_PLACEMENT_3D('',#74450,#49501,#49502);
#42271=AXIS2_PLACEMENT_3D('',#74451,#49503,#49504);
#42272=AXIS2_PLACEMENT_3D('',#74453,#49505,#49506);
#42273=AXIS2_PLACEMENT_3D('',#74455,#49508,#49509);
#42274=AXIS2_PLACEMENT_3D('',#74457,#49510,#49511);
#42275=AXIS2_PLACEMENT_3D('',#74459,#49512,#49513);
#42276=AXIS2_PLACEMENT_3D('',#74483,#49515,#49516);
#42277=AXIS2_PLACEMENT_3D('',#74489,#49517,#49518);
#42278=AXIS2_PLACEMENT_3D('',#74494,#49519,#49520);
#42279=AXIS2_PLACEMENT_3D('',#74495,#49521,#49522);
#42280=AXIS2_PLACEMENT_3D('',#74496,#49523,#49524);
#42281=AXIS2_PLACEMENT_3D('',#74515,#49526,#49527);
#42282=AXIS2_PLACEMENT_3D('',#74517,#49529,#49530);
#42283=AXIS2_PLACEMENT_3D('',#74518,#49531,#49532);
#42284=AXIS2_PLACEMENT_3D('',#74519,#49533,#49534);
#42285=AXIS2_PLACEMENT_3D('',#74521,#49535,#49536);
#42286=AXIS2_PLACEMENT_3D('',#74522,#49537,#49538);
#42287=AXIS2_PLACEMENT_3D('',#74523,#49539,#49540);
#42288=AXIS2_PLACEMENT_3D('',#74525,#49541,#49542);
#42289=AXIS2_PLACEMENT_3D('',#74530,#49543,#49544);
#42290=AXIS2_PLACEMENT_3D('',#74532,#49545,#49546);
#42291=AXIS2_PLACEMENT_3D('',#74534,#49547,#49548);
#42292=AXIS2_PLACEMENT_3D('',#74558,#49550,#49551);
#42293=AXIS2_PLACEMENT_3D('',#74564,#49552,#49553);
#42294=AXIS2_PLACEMENT_3D('',#74569,#49554,#49555);
#42295=AXIS2_PLACEMENT_3D('',#74570,#49556,#49557);
#42296=AXIS2_PLACEMENT_3D('',#74571,#49558,#49559);
#42297=AXIS2_PLACEMENT_3D('',#74590,#49561,#49562);
#42298=AXIS2_PLACEMENT_3D('',#74592,#49564,#49565);
#42299=AXIS2_PLACEMENT_3D('',#74593,#49566,#49567);
#42300=AXIS2_PLACEMENT_3D('',#74594,#49568,#49569);
#42301=AXIS2_PLACEMENT_3D('',#74596,#49570,#49571);
#42302=AXIS2_PLACEMENT_3D('',#74597,#49572,#49573);
#42303=AXIS2_PLACEMENT_3D('',#74598,#49574,#49575);
#42304=AXIS2_PLACEMENT_3D('',#74600,#49576,#49577);
#42305=AXIS2_PLACEMENT_3D('',#74605,#49578,#49579);
#42306=AXIS2_PLACEMENT_3D('',#74607,#49580,#49581);
#42307=AXIS2_PLACEMENT_3D('',#74608,#49582,#49583);
#42308=AXIS2_PLACEMENT_3D('',#74609,#49584,#49585);
#42309=AXIS2_PLACEMENT_3D('',#74611,#49586,#49587);
#42310=AXIS2_PLACEMENT_3D('',#74613,#49589,#49590);
#42311=AXIS2_PLACEMENT_3D('',#74615,#49591,#49592);
#42312=AXIS2_PLACEMENT_3D('',#74617,#49593,#49594);
#42313=AXIS2_PLACEMENT_3D('',#74641,#49596,#49597);
#42314=AXIS2_PLACEMENT_3D('',#74647,#49598,#49599);
#42315=AXIS2_PLACEMENT_3D('',#74652,#49600,#49601);
#42316=AXIS2_PLACEMENT_3D('',#74653,#49602,#49603);
#42317=AXIS2_PLACEMENT_3D('',#74654,#49604,#49605);
#42318=AXIS2_PLACEMENT_3D('',#74673,#49607,#49608);
#42319=AXIS2_PLACEMENT_3D('',#74675,#49610,#49611);
#42320=AXIS2_PLACEMENT_3D('',#74676,#49612,#49613);
#42321=AXIS2_PLACEMENT_3D('',#74677,#49614,#49615);
#42322=AXIS2_PLACEMENT_3D('',#74679,#49616,#49617);
#42323=AXIS2_PLACEMENT_3D('',#74680,#49618,#49619);
#42324=AXIS2_PLACEMENT_3D('',#74681,#49620,#49621);
#42325=AXIS2_PLACEMENT_3D('',#74683,#49622,#49623);
#42326=AXIS2_PLACEMENT_3D('',#74688,#49624,#49625);
#42327=AXIS2_PLACEMENT_3D('',#74690,#49626,#49627);
#42328=AXIS2_PLACEMENT_3D('',#74691,#49628,#49629);
#42329=AXIS2_PLACEMENT_3D('',#74692,#49630,#49631);
#42330=AXIS2_PLACEMENT_3D('',#74694,#49632,#49633);
#42331=AXIS2_PLACEMENT_3D('',#74696,#49635,#49636);
#42332=AXIS2_PLACEMENT_3D('',#74698,#49637,#49638);
#42333=AXIS2_PLACEMENT_3D('',#74700,#49639,#49640);
#42334=AXIS2_PLACEMENT_3D('',#74724,#49642,#49643);
#42335=AXIS2_PLACEMENT_3D('',#74730,#49644,#49645);
#42336=AXIS2_PLACEMENT_3D('',#74735,#49646,#49647);
#42337=AXIS2_PLACEMENT_3D('',#74736,#49648,#49649);
#42338=AXIS2_PLACEMENT_3D('',#74737,#49650,#49651);
#42339=AXIS2_PLACEMENT_3D('',#74756,#49653,#49654);
#42340=AXIS2_PLACEMENT_3D('',#74758,#49656,#49657);
#42341=AXIS2_PLACEMENT_3D('',#74759,#49658,#49659);
#42342=AXIS2_PLACEMENT_3D('',#74760,#49660,#49661);
#42343=AXIS2_PLACEMENT_3D('',#74762,#49662,#49663);
#42344=AXIS2_PLACEMENT_3D('',#74763,#49664,#49665);
#42345=AXIS2_PLACEMENT_3D('',#74764,#49666,#49667);
#42346=AXIS2_PLACEMENT_3D('',#74766,#49668,#49669);
#42347=AXIS2_PLACEMENT_3D('',#74792,#49670,#49671);
#42348=AXIS2_PLACEMENT_3D('',#74794,#49672,#49673);
#42349=AXIS2_PLACEMENT_3D('',#74799,#49674,#49675);
#42350=AXIS2_PLACEMENT_3D('',#74801,#49676,#49677);
#42351=AXIS2_PLACEMENT_3D('',#74802,#49678,#49679);
#42352=AXIS2_PLACEMENT_3D('',#74803,#49680,#49681);
#42353=AXIS2_PLACEMENT_3D('',#74804,#49682,#49683);
#42354=AXIS2_PLACEMENT_3D('',#74805,#49684,#49685);
#42355=AXIS2_PLACEMENT_3D('',#74806,#49686,#49687);
#42356=AXIS2_PLACEMENT_3D('',#74809,#49689,#49690);
#42357=AXIS2_PLACEMENT_3D('',#74810,#49691,#49692);
#42358=AXIS2_PLACEMENT_3D('',#74811,#49693,#49694);
#42359=AXIS2_PLACEMENT_3D('',#74814,#49696,#49697);
#42360=AXIS2_PLACEMENT_3D('',#74844,#49699,#49700);
#42361=AXIS2_PLACEMENT_3D('',#74846,#49701,#49702);
#42362=AXIS2_PLACEMENT_3D('',#74851,#49703,#49704);
#42363=AXIS2_PLACEMENT_3D('',#74852,#49705,#49706);
#42364=AXIS2_PLACEMENT_3D('',#74855,#49708,#49709);
#42365=AXIS2_PLACEMENT_3D('',#74856,#49710,#49711);
#42366=AXIS2_PLACEMENT_3D('',#74857,#49712,#49713);
#42367=AXIS2_PLACEMENT_3D('',#74858,#49714,#49715);
#42368=AXIS2_PLACEMENT_3D('',#74859,#49716,#49717);
#42369=AXIS2_PLACEMENT_3D('',#74862,#49719,#49720);
#42370=AXIS2_PLACEMENT_3D('',#74892,#49722,#49723);
#42371=AXIS2_PLACEMENT_3D('',#74894,#49724,#49725);
#42372=AXIS2_PLACEMENT_3D('',#74899,#49726,#49727);
#42373=AXIS2_PLACEMENT_3D('',#74900,#49728,#49729);
#42374=AXIS2_PLACEMENT_3D('',#74903,#49731,#49732);
#42375=AXIS2_PLACEMENT_3D('',#74904,#49733,#49734);
#42376=AXIS2_PLACEMENT_3D('',#74905,#49735,#49736);
#42377=AXIS2_PLACEMENT_3D('',#74906,#49737,#49738);
#42378=AXIS2_PLACEMENT_3D('',#74907,#49739,#49740);
#42379=AXIS2_PLACEMENT_3D('',#74910,#49742,#49743);
#42380=AXIS2_PLACEMENT_3D('',#74940,#49745,#49746);
#42381=AXIS2_PLACEMENT_3D('',#74942,#49747,#49748);
#42382=AXIS2_PLACEMENT_3D('',#74947,#49749,#49750);
#42383=AXIS2_PLACEMENT_3D('',#74949,#49751,#49752);
#42384=AXIS2_PLACEMENT_3D('',#74950,#49753,#49754);
#42385=AXIS2_PLACEMENT_3D('',#74951,#49755,#49756);
#42386=AXIS2_PLACEMENT_3D('',#74952,#49757,#49758);
#42387=AXIS2_PLACEMENT_3D('',#74953,#49759,#49760);
#42388=AXIS2_PLACEMENT_3D('',#74954,#49761,#49762);
#42389=AXIS2_PLACEMENT_3D('',#74957,#49764,#49765);
#42390=AXIS2_PLACEMENT_3D('',#74958,#49766,#49767);
#42391=AXIS2_PLACEMENT_3D('',#74959,#49768,#49769);
#42392=AXIS2_PLACEMENT_3D('',#74962,#49771,#49772);
#42393=AXIS2_PLACEMENT_3D('',#74971,#49774,#49775);
#42394=AXIS2_PLACEMENT_3D('',#75006,#49778,#49779);
#42395=AXIS2_PLACEMENT_3D('',#75010,#49781,#49782);
#42396=AXIS2_PLACEMENT_3D('',#75028,#49784,#49785);
#42397=AXIS2_PLACEMENT_3D('',#75029,#49786,#49787);
#42398=AXIS2_PLACEMENT_3D('',#75039,#49789,#49790);
#42399=AXIS2_PLACEMENT_3D('',#75042,#49792,#49793);
#42400=AXIS2_PLACEMENT_3D('',#75070,#49794,#49795);
#42401=AXIS2_PLACEMENT_3D('',#75072,#49796,#49797);
#42402=AXIS2_PLACEMENT_3D('',#75077,#49798,#49799);
#42403=AXIS2_PLACEMENT_3D('',#75078,#49800,#49801);
#42404=AXIS2_PLACEMENT_3D('',#75081,#49803,#49804);
#42405=AXIS2_PLACEMENT_3D('',#75082,#49805,#49806);
#42406=AXIS2_PLACEMENT_3D('',#75083,#49807,#49808);
#42407=AXIS2_PLACEMENT_3D('',#75084,#49809,#49810);
#42408=AXIS2_PLACEMENT_3D('',#75085,#49811,#49812);
#42409=AXIS2_PLACEMENT_3D('',#75088,#49814,#49815);
#42410=AXIS2_PLACEMENT_3D('',#75097,#49817,#49818);
#42411=AXIS2_PLACEMENT_3D('',#75099,#49819,#49820);
#42412=AXIS2_PLACEMENT_3D('',#75101,#49821,#49822);
#42413=AXIS2_PLACEMENT_3D('',#75125,#49824,#49825);
#42414=AXIS2_PLACEMENT_3D('',#75131,#49826,#49827);
#42415=AXIS2_PLACEMENT_3D('',#75136,#49828,#49829);
#42416=AXIS2_PLACEMENT_3D('',#75137,#49830,#49831);
#42417=AXIS2_PLACEMENT_3D('',#75138,#49832,#49833);
#42418=AXIS2_PLACEMENT_3D('',#75157,#49835,#49836);
#42419=AXIS2_PLACEMENT_3D('',#75159,#49838,#49839);
#42420=AXIS2_PLACEMENT_3D('',#75160,#49840,#49841);
#42421=AXIS2_PLACEMENT_3D('',#75161,#49842,#49843);
#42422=AXIS2_PLACEMENT_3D('',#75163,#49844,#49845);
#42423=AXIS2_PLACEMENT_3D('',#75164,#49846,#49847);
#42424=AXIS2_PLACEMENT_3D('',#75165,#49848,#49849);
#42425=AXIS2_PLACEMENT_3D('',#75167,#49850,#49851);
#42426=AXIS2_PLACEMENT_3D('',#75192,#49852,#49853);
#42427=AXIS2_PLACEMENT_3D('',#75193,#49854,#49855);
#42428=AXIS2_PLACEMENT_3D('',#75194,#49856,#49857);
#42429=AXIS2_PLACEMENT_3D('',#75195,#49858,#49859);
#42430=AXIS2_PLACEMENT_3D('',#75196,#49860,#49861);
#42431=AXIS2_PLACEMENT_3D('',#75197,#49862,#49863);
#42432=AXIS2_PLACEMENT_3D('',#75198,#49864,#49865);
#42433=AXIS2_PLACEMENT_3D('',#75220,#49866,#49867);
#42434=AXIS2_PLACEMENT_3D('',#75222,#49868,#49869);
#42435=AXIS2_PLACEMENT_3D('',#75227,#49870,#49871);
#42436=AXIS2_PLACEMENT_3D('',#75229,#49872,#49873);
#42437=AXIS2_PLACEMENT_3D('',#75230,#49874,#49875);
#42438=AXIS2_PLACEMENT_3D('',#75231,#49876,#49877);
#42439=AXIS2_PLACEMENT_3D('',#75232,#49878,#49879);
#42440=AXIS2_PLACEMENT_3D('',#75233,#49880,#49881);
#42441=AXIS2_PLACEMENT_3D('',#75234,#49882,#49883);
#42442=AXIS2_PLACEMENT_3D('',#75237,#49885,#49886);
#42443=AXIS2_PLACEMENT_3D('',#75238,#49887,#49888);
#42444=AXIS2_PLACEMENT_3D('',#75239,#49889,#49890);
#42445=AXIS2_PLACEMENT_3D('',#75242,#49892,#49893);
#42446=AXIS2_PLACEMENT_3D('',#75251,#49895,#49896);
#42447=AXIS2_PLACEMENT_3D('',#75268,#49898,#49899);
#42448=AXIS2_PLACEMENT_3D('',#75278,#49901,#49902);
#42449=AXIS2_PLACEMENT_3D('',#75280,#49904,#49905);
#42450=AXIS2_PLACEMENT_3D('',#75289,#49906,#49907);
#42451=AXIS2_PLACEMENT_3D('',#75290,#49908,#49909);
#42452=AXIS2_PLACEMENT_3D('',#75291,#49910,#49911);
#42453=AXIS2_PLACEMENT_3D('',#75293,#49912,#49913);
#42454=AXIS2_PLACEMENT_3D('',#75295,#49914,#49915);
#42455=AXIS2_PLACEMENT_3D('',#75297,#49917,#49918);
#42456=AXIS2_PLACEMENT_3D('',#75298,#49919,#49920);
#42457=AXIS2_PLACEMENT_3D('',#75325,#49921,#49922);
#42458=AXIS2_PLACEMENT_3D('',#75330,#49923,#49924);
#42459=AXIS2_PLACEMENT_3D('',#75341,#49928,#49929);
#42460=AXIS2_PLACEMENT_3D('',#75349,#49930,#49931);
#42461=AXIS2_PLACEMENT_3D('',#75350,#49932,#49933);
#42462=AXIS2_PLACEMENT_3D('',#75352,#49935,#49936);
#42463=AXIS2_PLACEMENT_3D('',#75356,#49939,#49940);
#42464=AXIS2_PLACEMENT_3D('',#75367,#49943,#49944);
#42465=AXIS2_PLACEMENT_3D('',#75368,#49945,#49946);
#42466=AXIS2_PLACEMENT_3D('',#75385,#49948,#49949);
#42467=AXIS2_PLACEMENT_3D('',#75395,#49951,#49952);
#42468=AXIS2_PLACEMENT_3D('',#75397,#49954,#49955);
#42469=AXIS2_PLACEMENT_3D('',#75398,#49956,#49957);
#42470=AXIS2_PLACEMENT_3D('',#75399,#49958,#49959);
#42471=AXIS2_PLACEMENT_3D('',#75401,#49961,#49962);
#42472=AXIS2_PLACEMENT_3D('',#75403,#49964,#49965);
#42473=AXIS2_PLACEMENT_3D('',#75404,#49966,#49967);
#42474=AXIS2_PLACEMENT_3D('',#75405,#49968,#49969);
#42475=AXIS2_PLACEMENT_3D('',#75407,#49971,#49972);
#42476=AXIS2_PLACEMENT_3D('',#75411,#49975,#49976);
#42477=AXIS2_PLACEMENT_3D('',#75422,#49979,#49980);
#42478=AXIS2_PLACEMENT_3D('',#75423,#49981,#49982);
#42479=AXIS2_PLACEMENT_3D('',#75425,#49983,#49984);
#42480=AXIS2_PLACEMENT_3D('',#75432,#49985,#49986);
#42481=AXIS2_PLACEMENT_3D('',#75434,#49988,#49989);
#42482=AXIS2_PLACEMENT_3D('',#75436,#49991,#49992);
#42483=AXIS2_PLACEMENT_3D('',#75453,#49994,#49995);
#42484=AXIS2_PLACEMENT_3D('',#75463,#49997,#49998);
#42485=AXIS2_PLACEMENT_3D('',#75465,#50000,#50001);
#42486=AXIS2_PLACEMENT_3D('',#75466,#50002,#50003);
#42487=AXIS2_PLACEMENT_3D('',#75467,#50004,#50005);
#42488=AXIS2_PLACEMENT_3D('',#75469,#50007,#50008);
#42489=AXIS2_PLACEMENT_3D('',#75473,#50011,#50012);
#42490=AXIS2_PLACEMENT_3D('',#75484,#50015,#50016);
#42491=AXIS2_PLACEMENT_3D('',#75485,#50017,#50018);
#42492=AXIS2_PLACEMENT_3D('',#75486,#50019,#50020);
#42493=AXIS2_PLACEMENT_3D('',#75487,#50021,#50022);
#42494=AXIS2_PLACEMENT_3D('',#75489,#50024,#50025);
#42495=AXIS2_PLACEMENT_3D('',#75491,#50027,#50028);
#42496=AXIS2_PLACEMENT_3D('',#75492,#50029,#50030);
#42497=AXIS2_PLACEMENT_3D('',#75493,#50031,#50032);
#42498=AXIS2_PLACEMENT_3D('',#75510,#50034,#50035);
#42499=AXIS2_PLACEMENT_3D('',#75520,#50037,#50038);
#42500=AXIS2_PLACEMENT_3D('',#75543,#50040,#50041);
#42501=AXIS2_PLACEMENT_3D('',#75545,#50042,#50043);
#42502=AXIS2_PLACEMENT_3D('',#75550,#50044,#50045);
#42503=AXIS2_PLACEMENT_3D('',#75551,#50046,#50047);
#42504=AXIS2_PLACEMENT_3D('',#75552,#50048,#50049);
#42505=AXIS2_PLACEMENT_3D('',#75553,#50050,#50051);
#42506=AXIS2_PLACEMENT_3D('',#75556,#50053,#50054);
#42507=AXIS2_PLACEMENT_3D('',#75557,#50055,#50056);
#42508=AXIS2_PLACEMENT_3D('',#75558,#50057,#50058);
#42509=AXIS2_PLACEMENT_3D('',#75560,#50060,#50061);
#42510=AXIS2_PLACEMENT_3D('',#75563,#50064,#50065);
#42511=AXIS2_PLACEMENT_3D('',#75565,#50067,#50068);
#42512=AXIS2_PLACEMENT_3D('',#75566,#50069,#50070);
#42513=AXIS2_PLACEMENT_3D('',#75567,#50071,#50072);
#42514=AXIS2_PLACEMENT_3D('',#75569,#50074,#50075);
#42515=AXIS2_PLACEMENT_3D('',#75571,#50077,#50078);
#42516=AXIS2_PLACEMENT_3D('',#75572,#50079,#50080);
#42517=AXIS2_PLACEMENT_3D('',#75573,#50081,#50082);
#42518=AXIS2_PLACEMENT_3D('',#75575,#50084,#50085);
#42519=AXIS2_PLACEMENT_3D('',#75579,#50088,#50089);
#42520=AXIS2_PLACEMENT_3D('',#75590,#50092,#50093);
#42521=AXIS2_PLACEMENT_3D('',#75591,#50094,#50095);
#42522=AXIS2_PLACEMENT_3D('',#75608,#50097,#50098);
#42523=AXIS2_PLACEMENT_3D('',#75618,#50100,#50101);
#42524=AXIS2_PLACEMENT_3D('',#75620,#50103,#50104);
#42525=AXIS2_PLACEMENT_3D('',#75621,#50105,#50106);
#42526=AXIS2_PLACEMENT_3D('',#75622,#50107,#50108);
#42527=AXIS2_PLACEMENT_3D('',#75624,#50109,#50110);
#42528=AXIS2_PLACEMENT_3D('',#75626,#50112,#50113);
#42529=AXIS2_PLACEMENT_3D('',#75629,#50116,#50117);
#42530=AXIS2_PLACEMENT_3D('',#75631,#50118,#50119);
#42531=AXIS2_PLACEMENT_3D('',#75638,#50120,#50121);
#42532=AXIS2_PLACEMENT_3D('',#75640,#50123,#50124);
#42533=AXIS2_PLACEMENT_3D('',#75644,#50127,#50128);
#42534=AXIS2_PLACEMENT_3D('',#75655,#50131,#50132);
#42535=AXIS2_PLACEMENT_3D('',#75656,#50133,#50134);
#42536=AXIS2_PLACEMENT_3D('',#75664,#50135,#50136);
#42537=AXIS2_PLACEMENT_3D('',#75665,#50137,#50138);
#42538=AXIS2_PLACEMENT_3D('',#75667,#50140,#50141);
#42539=AXIS2_PLACEMENT_3D('',#75669,#50143,#50144);
#42540=AXIS2_PLACEMENT_3D('',#75686,#50146,#50147);
#42541=AXIS2_PLACEMENT_3D('',#75696,#50149,#50150);
#42542=AXIS2_PLACEMENT_3D('',#75698,#50152,#50153);
#42543=AXIS2_PLACEMENT_3D('',#75699,#50154,#50155);
#42544=AXIS2_PLACEMENT_3D('',#75700,#50156,#50157);
#42545=AXIS2_PLACEMENT_3D('',#75702,#50159,#50160);
#42546=AXIS2_PLACEMENT_3D('',#75706,#50163,#50164);
#42547=AXIS2_PLACEMENT_3D('',#75717,#50167,#50168);
#42548=AXIS2_PLACEMENT_3D('',#75718,#50169,#50170);
#42549=AXIS2_PLACEMENT_3D('',#75719,#50171,#50172);
#42550=AXIS2_PLACEMENT_3D('',#75720,#50173,#50174);
#42551=AXIS2_PLACEMENT_3D('',#75722,#50176,#50177);
#42552=AXIS2_PLACEMENT_3D('',#75724,#50179,#50180);
#42553=AXIS2_PLACEMENT_3D('',#75725,#50181,#50182);
#42554=AXIS2_PLACEMENT_3D('',#75726,#50183,#50184);
#42555=AXIS2_PLACEMENT_3D('',#75743,#50186,#50187);
#42556=AXIS2_PLACEMENT_3D('',#75753,#50189,#50190);
#42557=AXIS2_PLACEMENT_3D('',#75776,#50192,#50193);
#42558=AXIS2_PLACEMENT_3D('',#75778,#50194,#50195);
#42559=AXIS2_PLACEMENT_3D('',#75783,#50196,#50197);
#42560=AXIS2_PLACEMENT_3D('',#75784,#50198,#50199);
#42561=AXIS2_PLACEMENT_3D('',#75785,#50200,#50201);
#42562=AXIS2_PLACEMENT_3D('',#75786,#50202,#50203);
#42563=AXIS2_PLACEMENT_3D('',#75789,#50205,#50206);
#42564=AXIS2_PLACEMENT_3D('',#75790,#50207,#50208);
#42565=AXIS2_PLACEMENT_3D('',#75791,#50209,#50210);
#42566=AXIS2_PLACEMENT_3D('',#75793,#50212,#50213);
#42567=AXIS2_PLACEMENT_3D('',#75796,#50216,#50217);
#42568=AXIS2_PLACEMENT_3D('',#75798,#50219,#50220);
#42569=AXIS2_PLACEMENT_3D('',#75799,#50221,#50222);
#42570=AXIS2_PLACEMENT_3D('',#75800,#50223,#50224);
#42571=AXIS2_PLACEMENT_3D('',#75802,#50225,#50226);
#42572=AXIS2_PLACEMENT_3D('',#75804,#50228,#50229);
#42573=AXIS2_PLACEMENT_3D('',#75807,#50232,#50233);
#42574=AXIS2_PLACEMENT_3D('',#75815,#50234,#50235);
#42575=AXIS2_PLACEMENT_3D('',#75816,#50236,#50237);
#42576=AXIS2_PLACEMENT_3D('',#75818,#50239,#50240);
#42577=AXIS2_PLACEMENT_3D('',#75822,#50243,#50244);
#42578=AXIS2_PLACEMENT_3D('',#75833,#50247,#50248);
#42579=AXIS2_PLACEMENT_3D('',#75834,#50249,#50250);
#42580=AXIS2_PLACEMENT_3D('',#75851,#50252,#50253);
#42581=AXIS2_PLACEMENT_3D('',#75861,#50255,#50256);
#42582=AXIS2_PLACEMENT_3D('',#75863,#50258,#50259);
#42583=AXIS2_PLACEMENT_3D('',#75864,#50260,#50261);
#42584=AXIS2_PLACEMENT_3D('',#75865,#50262,#50263);
#42585=AXIS2_PLACEMENT_3D('',#75867,#50265,#50266);
#42586=AXIS2_PLACEMENT_3D('',#75869,#50268,#50269);
#42587=AXIS2_PLACEMENT_3D('',#75870,#50270,#50271);
#42588=AXIS2_PLACEMENT_3D('',#75871,#50272,#50273);
#42589=AXIS2_PLACEMENT_3D('',#75873,#50275,#50276);
#42590=AXIS2_PLACEMENT_3D('',#75877,#50279,#50280);
#42591=AXIS2_PLACEMENT_3D('',#75888,#50283,#50284);
#42592=AXIS2_PLACEMENT_3D('',#75889,#50285,#50286);
#42593=AXIS2_PLACEMENT_3D('',#75890,#50287,#50288);
#42594=AXIS2_PLACEMENT_3D('',#75891,#50289,#50290);
#42595=AXIS2_PLACEMENT_3D('',#75893,#50292,#50293);
#42596=AXIS2_PLACEMENT_3D('',#75895,#50295,#50296);
#42597=AXIS2_PLACEMENT_3D('',#75912,#50298,#50299);
#42598=AXIS2_PLACEMENT_3D('',#75922,#50301,#50302);
#42599=AXIS2_PLACEMENT_3D('',#75924,#50304,#50305);
#42600=AXIS2_PLACEMENT_3D('',#75925,#50306,#50307);
#42601=AXIS2_PLACEMENT_3D('',#75926,#50308,#50309);
#42602=AXIS2_PLACEMENT_3D('',#75928,#50311,#50312);
#42603=AXIS2_PLACEMENT_3D('',#75932,#50315,#50316);
#42604=AXIS2_PLACEMENT_3D('',#75943,#50319,#50320);
#42605=AXIS2_PLACEMENT_3D('',#75944,#50321,#50322);
#42606=AXIS2_PLACEMENT_3D('',#75945,#50323,#50324);
#42607=AXIS2_PLACEMENT_3D('',#75946,#50325,#50326);
#42608=AXIS2_PLACEMENT_3D('',#75948,#50328,#50329);
#42609=AXIS2_PLACEMENT_3D('',#75950,#50331,#50332);
#42610=AXIS2_PLACEMENT_3D('',#75951,#50333,#50334);
#42611=AXIS2_PLACEMENT_3D('',#75952,#50335,#50336);
#42612=AXIS2_PLACEMENT_3D('',#75969,#50338,#50339);
#42613=AXIS2_PLACEMENT_3D('',#75979,#50341,#50342);
#42614=AXIS2_PLACEMENT_3D('',#76002,#50344,#50345);
#42615=AXIS2_PLACEMENT_3D('',#76004,#50346,#50347);
#42616=AXIS2_PLACEMENT_3D('',#76009,#50348,#50349);
#42617=AXIS2_PLACEMENT_3D('',#76010,#50350,#50351);
#42618=AXIS2_PLACEMENT_3D('',#76011,#50352,#50353);
#42619=AXIS2_PLACEMENT_3D('',#76012,#50354,#50355);
#42620=AXIS2_PLACEMENT_3D('',#76015,#50357,#50358);
#42621=AXIS2_PLACEMENT_3D('',#76016,#50359,#50360);
#42622=AXIS2_PLACEMENT_3D('',#76017,#50361,#50362);
#42623=AXIS2_PLACEMENT_3D('',#76019,#50364,#50365);
#42624=AXIS2_PLACEMENT_3D('',#76022,#50368,#50369);
#42625=AXIS2_PLACEMENT_3D('',#76024,#50371,#50372);
#42626=AXIS2_PLACEMENT_3D('',#76025,#50373,#50374);
#42627=AXIS2_PLACEMENT_3D('',#76026,#50375,#50376);
#42628=AXIS2_PLACEMENT_3D('',#76028,#50378,#50379);
#42629=AXIS2_PLACEMENT_3D('',#76030,#50381,#50382);
#42630=AXIS2_PLACEMENT_3D('',#76031,#50383,#50384);
#42631=AXIS2_PLACEMENT_3D('',#76032,#50385,#50386);
#42632=AXIS2_PLACEMENT_3D('',#76049,#50388,#50389);
#42633=AXIS2_PLACEMENT_3D('',#76059,#50391,#50392);
#42634=AXIS2_PLACEMENT_3D('',#76082,#50394,#50395);
#42635=AXIS2_PLACEMENT_3D('',#76084,#50396,#50397);
#42636=AXIS2_PLACEMENT_3D('',#76089,#50398,#50399);
#42637=AXIS2_PLACEMENT_3D('',#76091,#50400,#50401);
#42638=AXIS2_PLACEMENT_3D('',#76092,#50402,#50403);
#42639=AXIS2_PLACEMENT_3D('',#76093,#50404,#50405);
#42640=AXIS2_PLACEMENT_3D('',#76094,#50406,#50407);
#42641=AXIS2_PLACEMENT_3D('',#76095,#50408,#50409);
#42642=AXIS2_PLACEMENT_3D('',#76096,#50410,#50411);
#42643=AXIS2_PLACEMENT_3D('',#76099,#50413,#50414);
#42644=AXIS2_PLACEMENT_3D('',#76100,#50415,#50416);
#42645=AXIS2_PLACEMENT_3D('',#76102,#50418,#50419);
#42646=AXIS2_PLACEMENT_3D('',#76103,#50420,#50421);
#42647=AXIS2_PLACEMENT_3D('',#76106,#50423,#50424);
#42648=AXIS2_PLACEMENT_3D('',#76115,#50426,#50427);
#42649=AXIS2_PLACEMENT_3D('',#76127,#50430,#50431);
#42650=AXIS2_PLACEMENT_3D('',#76129,#50433,#50434);
#42651=AXIS2_PLACEMENT_3D('',#76130,#50435,#50436);
#42652=AXIS2_PLACEMENT_3D('',#76131,#50437,#50438);
#42653=AXIS2_PLACEMENT_3D('',#76133,#50440,#50441);
#42654=AXIS2_PLACEMENT_3D('',#76135,#50443,#50444);
#42655=AXIS2_PLACEMENT_3D('',#76136,#50445,#50446);
#42656=AXIS2_PLACEMENT_3D('',#76137,#50447,#50448);
#42657=AXIS2_PLACEMENT_3D('',#76139,#50450,#50451);
#42658=AXIS2_PLACEMENT_3D('',#76143,#50454,#50455);
#42659=AXIS2_PLACEMENT_3D('',#76154,#50458,#50459);
#42660=AXIS2_PLACEMENT_3D('',#76155,#50460,#50461);
#42661=AXIS2_PLACEMENT_3D('',#76163,#50462,#50463);
#42662=AXIS2_PLACEMENT_3D('',#76164,#50464,#50465);
#42663=AXIS2_PLACEMENT_3D('',#76181,#50467,#50468);
#42664=AXIS2_PLACEMENT_3D('',#76191,#50470,#50471);
#42665=AXIS2_PLACEMENT_3D('',#76193,#50473,#50474);
#42666=AXIS2_PLACEMENT_3D('',#76195,#50476,#50477);
#42667=AXIS2_PLACEMENT_3D('',#76197,#50479,#50480);
#42668=AXIS2_PLACEMENT_3D('',#76198,#50481,#50482);
#42669=AXIS2_PLACEMENT_3D('',#76199,#50483,#50484);
#42670=AXIS2_PLACEMENT_3D('',#76201,#50486,#50487);
#42671=AXIS2_PLACEMENT_3D('',#76205,#50490,#50491);
#42672=AXIS2_PLACEMENT_3D('',#76216,#50494,#50495);
#42673=AXIS2_PLACEMENT_3D('',#76217,#50496,#50497);
#42674=AXIS2_PLACEMENT_3D('',#76219,#50498,#50499);
#42675=AXIS2_PLACEMENT_3D('',#76221,#50500,#50501);
#42676=AXIS2_PLACEMENT_3D('',#76245,#50503,#50504);
#42677=AXIS2_PLACEMENT_3D('',#76251,#50505,#50506);
#42678=AXIS2_PLACEMENT_3D('',#76256,#50507,#50508);
#42679=AXIS2_PLACEMENT_3D('',#76257,#50509,#50510);
#42680=AXIS2_PLACEMENT_3D('',#76258,#50511,#50512);
#42681=AXIS2_PLACEMENT_3D('',#76262,#50514,#50515);
#42682=AXIS2_PLACEMENT_3D('',#76284,#50517,#50518);
#42683=AXIS2_PLACEMENT_3D('',#76285,#50519,#50520);
#42684=AXIS2_PLACEMENT_3D('',#76287,#50521,#50522);
#42685=AXIS2_PLACEMENT_3D('',#76288,#50523,#50524);
#42686=AXIS2_PLACEMENT_3D('',#76289,#50525,#50526);
#42687=AXIS2_PLACEMENT_3D('',#76290,#50527,#50528);
#42688=AXIS2_PLACEMENT_3D('',#76291,#50529,#50530);
#42689=AXIS2_PLACEMENT_3D('',#76292,#50531,#50532);
#42690=AXIS2_PLACEMENT_3D('',#76293,#50533,#50534);
#42691=AXIS2_PLACEMENT_3D('',#76295,#50535,#50536);
#42692=AXIS2_PLACEMENT_3D('',#76296,#50537,#50538);
#42693=AXIS2_PLACEMENT_3D('',#76297,#50539,#50540);
#42694=AXIS2_PLACEMENT_3D('',#76299,#50541,#50542);
#42695=AXIS2_PLACEMENT_3D('',#76304,#50543,#50544);
#42696=AXIS2_PLACEMENT_3D('',#76306,#50545,#50546);
#42697=AXIS2_PLACEMENT_3D('',#76307,#50547,#50548);
#42698=AXIS2_PLACEMENT_3D('',#76308,#50549,#50550);
#42699=AXIS2_PLACEMENT_3D('',#76310,#50552,#50553);
#42700=AXIS2_PLACEMENT_3D('',#76311,#50554,#50555);
#42701=AXIS2_PLACEMENT_3D('',#76312,#50556,#50557);
#42702=AXIS2_PLACEMENT_3D('',#76314,#50558,#50559);
#42703=AXIS2_PLACEMENT_3D('',#76316,#50560,#50561);
#42704=AXIS2_PLACEMENT_3D('',#76318,#50563,#50564);
#42705=AXIS2_PLACEMENT_3D('',#76320,#50565,#50566);
#42706=AXIS2_PLACEMENT_3D('',#76322,#50567,#50568);
#42707=AXIS2_PLACEMENT_3D('',#76346,#50570,#50571);
#42708=AXIS2_PLACEMENT_3D('',#76352,#50572,#50573);
#42709=AXIS2_PLACEMENT_3D('',#76357,#50574,#50575);
#42710=AXIS2_PLACEMENT_3D('',#76358,#50576,#50577);
#42711=AXIS2_PLACEMENT_3D('',#76359,#50578,#50579);
#42712=AXIS2_PLACEMENT_3D('',#76362,#50580,#50581);
#42713=AXIS2_PLACEMENT_3D('',#76364,#50582,#50583);
#42714=AXIS2_PLACEMENT_3D('',#76366,#50584,#50585);
#42715=AXIS2_PLACEMENT_3D('',#76375,#50586,#50587);
#42716=AXIS2_PLACEMENT_3D('',#76378,#50589,#50590);
#42717=AXIS2_PLACEMENT_3D('',#76391,#50592,#50593);
#42718=AXIS2_PLACEMENT_3D('',#76392,#50594,#50595);
#42719=AXIS2_PLACEMENT_3D('',#76414,#50596,#50597);
#42720=AXIS2_PLACEMENT_3D('',#76420,#50598,#50599);
#42721=AXIS2_PLACEMENT_3D('',#76425,#50600,#50601);
#42722=AXIS2_PLACEMENT_3D('',#76426,#50602,#50603);
#42723=AXIS2_PLACEMENT_3D('',#76427,#50604,#50605);
#42724=AXIS2_PLACEMENT_3D('',#76428,#50606,#50607);
#42725=AXIS2_PLACEMENT_3D('',#76429,#50608,#50609);
#42726=AXIS2_PLACEMENT_3D('',#76432,#50611,#50612);
#42727=AXIS2_PLACEMENT_3D('',#76433,#50613,#50614);
#42728=AXIS2_PLACEMENT_3D('',#76436,#50616,#50617);
#42729=AXIS2_PLACEMENT_3D('',#76437,#50618,#50619);
#42730=AXIS2_PLACEMENT_3D('',#76440,#50621,#50622);
#42731=AXIS2_PLACEMENT_3D('',#76445,#50623,#50624);
#42732=AXIS2_PLACEMENT_3D('',#76447,#50625,#50626);
#42733=AXIS2_PLACEMENT_3D('',#76454,#50627,#50628);
#42734=AXIS2_PLACEMENT_3D('',#76456,#50630,#50631);
#42735=AXIS2_PLACEMENT_3D('',#76458,#50632,#50633);
#42736=AXIS2_PLACEMENT_3D('',#76492,#50634,#50635);
#42737=AXIS2_PLACEMENT_3D('',#76493,#50636,#50637);
#42738=AXIS2_PLACEMENT_3D('',#76494,#50638,#50639);
#42739=AXIS2_PLACEMENT_3D('',#76495,#50640,#50641);
#42740=AXIS2_PLACEMENT_3D('',#76496,#50642,#50643);
#42741=AXIS2_PLACEMENT_3D('',#76497,#50644,#50645);
#42742=AXIS2_PLACEMENT_3D('',#76498,#50646,#50647);
#42743=AXIS2_PLACEMENT_3D('',#76501,#50649,#50650);
#42744=AXIS2_PLACEMENT_3D('',#76522,#50651,#50652);
#42745=AXIS2_PLACEMENT_3D('',#76523,#50653,#50654);
#42746=AXIS2_PLACEMENT_3D('',#76524,#50655,#50656);
#42747=AXIS2_PLACEMENT_3D('',#76525,#50657,#50658);
#42748=AXIS2_PLACEMENT_3D('',#76526,#50659,#50660);
#42749=AXIS2_PLACEMENT_3D('',#76527,#50661,#50662);
#42750=AXIS2_PLACEMENT_3D('',#76528,#50663,#50664);
#42751=AXIS2_PLACEMENT_3D('',#76529,#50665,#50666);
#42752=AXIS2_PLACEMENT_3D('',#76532,#50667,#50668);
#42753=AXIS2_PLACEMENT_3D('',#76533,#50669,#50670);
#42754=AXIS2_PLACEMENT_3D('',#76534,#50671,#50672);
#42755=AXIS2_PLACEMENT_3D('',#76535,#50673,#50674);
#42756=AXIS2_PLACEMENT_3D('',#76539,#50676,#50677);
#42757=AXIS2_PLACEMENT_3D('',#76540,#50678,#50679);
#42758=AXIS2_PLACEMENT_3D('',#76541,#50680,#50681);
#42759=AXIS2_PLACEMENT_3D('',#76543,#50682,#50683);
#42760=AXIS2_PLACEMENT_3D('',#76577,#50684,#50685);
#42761=AXIS2_PLACEMENT_3D('',#76578,#50686,#50687);
#42762=AXIS2_PLACEMENT_3D('',#76579,#50688,#50689);
#42763=AXIS2_PLACEMENT_3D('',#76580,#50690,#50691);
#42764=AXIS2_PLACEMENT_3D('',#76581,#50692,#50693);
#42765=AXIS2_PLACEMENT_3D('',#76582,#50694,#50695);
#42766=AXIS2_PLACEMENT_3D('',#76584,#50696,#50697);
#42767=AXIS2_PLACEMENT_3D('',#76618,#50698,#50699);
#42768=AXIS2_PLACEMENT_3D('',#76619,#50700,#50701);
#42769=AXIS2_PLACEMENT_3D('',#76620,#50702,#50703);
#42770=AXIS2_PLACEMENT_3D('',#76621,#50704,#50705);
#42771=AXIS2_PLACEMENT_3D('',#76622,#50706,#50707);
#42772=AXIS2_PLACEMENT_3D('',#76623,#50708,#50709);
#42773=AXIS2_PLACEMENT_3D('',#76624,#50710,#50711);
#42774=AXIS2_PLACEMENT_3D('',#76626,#50713,#50714);
#42775=AXIS2_PLACEMENT_3D('',#76630,#50717,#50718);
#42776=AXIS2_PLACEMENT_3D('',#76631,#50719,#50720);
#42777=AXIS2_PLACEMENT_3D('',#76633,#50722,#50723);
#42778=AXIS2_PLACEMENT_3D('',#76637,#50726,#50727);
#42779=AXIS2_PLACEMENT_3D('',#76638,#50728,#50729);
#42780=AXIS2_PLACEMENT_3D('',#76639,#50730,#50731);
#42781=AXIS2_PLACEMENT_3D('',#76641,#50732,#50733);
#42782=AXIS2_PLACEMENT_3D('',#76643,#50735,#50736);
#42783=AXIS2_PLACEMENT_3D('',#76646,#50739,#50740);
#42784=AXIS2_PLACEMENT_3D('',#76647,#50741,#50742);
#42785=AXIS2_PLACEMENT_3D('',#76648,#50743,#50744);
#42786=AXIS2_PLACEMENT_3D('',#76649,#50745,#50746);
#42787=AXIS2_PLACEMENT_3D('',#76650,#50747,#50748);
#42788=AXIS2_PLACEMENT_3D('',#76651,#50749,#50750);
#42789=AXIS2_PLACEMENT_3D('',#76668,#50752,#50753);
#42790=AXIS2_PLACEMENT_3D('',#76670,#50755,#50756);
#42791=AXIS2_PLACEMENT_3D('',#76672,#50758,#50759);
#42792=AXIS2_PLACEMENT_3D('',#76673,#50760,#50761);
#42793=AXIS2_PLACEMENT_3D('',#76674,#50762,#50763);
#42794=AXIS2_PLACEMENT_3D('',#76675,#50764,#50765);
#42795=AXIS2_PLACEMENT_3D('',#76676,#50766,#50767);
#42796=AXIS2_PLACEMENT_3D('',#76677,#50768,#50769);
#42797=AXIS2_PLACEMENT_3D('',#76680,#50771,#50772);
#42798=AXIS2_PLACEMENT_3D('',#76682,#50774,#50775);
#42799=AXIS2_PLACEMENT_3D('',#76699,#50777,#50778);
#42800=AXIS2_PLACEMENT_3D('',#76701,#50780,#50781);
#42801=AXIS2_PLACEMENT_3D('',#76703,#50783,#50784);
#42802=AXIS2_PLACEMENT_3D('',#76704,#50785,#50786);
#42803=AXIS2_PLACEMENT_3D('',#76705,#50787,#50788);
#42804=AXIS2_PLACEMENT_3D('',#76706,#50789,#50790);
#42805=AXIS2_PLACEMENT_3D('',#76707,#50791,#50792);
#42806=AXIS2_PLACEMENT_3D('',#76708,#50793,#50794);
#42807=AXIS2_PLACEMENT_3D('',#76725,#50796,#50797);
#42808=AXIS2_PLACEMENT_3D('',#76727,#50799,#50800);
#42809=AXIS2_PLACEMENT_3D('',#76729,#50802,#50803);
#42810=AXIS2_PLACEMENT_3D('',#76730,#50804,#50805);
#42811=AXIS2_PLACEMENT_3D('',#76731,#50806,#50807);
#42812=AXIS2_PLACEMENT_3D('',#76732,#50808,#50809);
#42813=AXIS2_PLACEMENT_3D('',#76734,#50811,#50812);
#42814=AXIS2_PLACEMENT_3D('',#76735,#50813,#50814);
#42815=AXIS2_PLACEMENT_3D('',#76736,#50815,#50816);
#42816=AXIS2_PLACEMENT_3D('',#76737,#50817,#50818);
#42817=AXIS2_PLACEMENT_3D('',#76739,#50820,#50821);
#42818=AXIS2_PLACEMENT_3D('',#76741,#50823,#50824);
#42819=AXIS2_PLACEMENT_3D('',#76742,#50825,#50826);
#42820=AXIS2_PLACEMENT_3D('',#76743,#50827,#50828);
#42821=AXIS2_PLACEMENT_3D('',#76744,#50829,#50830);
#42822=AXIS2_PLACEMENT_3D('',#76745,#50831,#50832);
#42823=AXIS2_PLACEMENT_3D('',#76746,#50833,#50834);
#42824=AXIS2_PLACEMENT_3D('',#76763,#50836,#50837);
#42825=AXIS2_PLACEMENT_3D('',#76765,#50839,#50840);
#42826=AXIS2_PLACEMENT_3D('',#76767,#50842,#50843);
#42827=AXIS2_PLACEMENT_3D('',#76768,#50844,#50845);
#42828=AXIS2_PLACEMENT_3D('',#76769,#50846,#50847);
#42829=AXIS2_PLACEMENT_3D('',#76770,#50848,#50849);
#42830=AXIS2_PLACEMENT_3D('',#76771,#50850,#50851);
#42831=AXIS2_PLACEMENT_3D('',#76772,#50852,#50853);
#42832=AXIS2_PLACEMENT_3D('',#76789,#50855,#50856);
#42833=AXIS2_PLACEMENT_3D('',#76791,#50858,#50859);
#42834=AXIS2_PLACEMENT_3D('',#76793,#50861,#50862);
#42835=AXIS2_PLACEMENT_3D('',#76794,#50863,#50864);
#42836=AXIS2_PLACEMENT_3D('',#76795,#50865,#50866);
#42837=AXIS2_PLACEMENT_3D('',#76796,#50867,#50868);
#42838=AXIS2_PLACEMENT_3D('',#76797,#50869,#50870);
#42839=AXIS2_PLACEMENT_3D('',#76798,#50871,#50872);
#42840=AXIS2_PLACEMENT_3D('',#76815,#50874,#50875);
#42841=AXIS2_PLACEMENT_3D('',#76817,#50877,#50878);
#42842=AXIS2_PLACEMENT_3D('',#76819,#50880,#50881);
#42843=AXIS2_PLACEMENT_3D('',#76820,#50882,#50883);
#42844=AXIS2_PLACEMENT_3D('',#76821,#50884,#50885);
#42845=AXIS2_PLACEMENT_3D('',#76822,#50886,#50887);
#42846=AXIS2_PLACEMENT_3D('',#76823,#50888,#50889);
#42847=AXIS2_PLACEMENT_3D('',#76825,#50891,#50892);
#42848=AXIS2_PLACEMENT_3D('',#76826,#50893,#50894);
#42849=AXIS2_PLACEMENT_3D('',#76827,#50895,#50896);
#42850=AXIS2_PLACEMENT_3D('',#76829,#50898,#50899);
#42851=AXIS2_PLACEMENT_3D('',#76831,#50901,#50902);
#42852=AXIS2_PLACEMENT_3D('',#76832,#50903,#50904);
#42853=AXIS2_PLACEMENT_3D('',#76833,#50905,#50906);
#42854=AXIS2_PLACEMENT_3D('',#76834,#50907,#50908);
#42855=AXIS2_PLACEMENT_3D('',#76835,#50909,#50910);
#42856=AXIS2_PLACEMENT_3D('',#76836,#50911,#50912);
#42857=AXIS2_PLACEMENT_3D('',#76853,#50914,#50915);
#42858=AXIS2_PLACEMENT_3D('',#76855,#50917,#50918);
#42859=AXIS2_PLACEMENT_3D('',#76857,#50920,#50921);
#42860=AXIS2_PLACEMENT_3D('',#76858,#50922,#50923);
#42861=AXIS2_PLACEMENT_3D('',#76859,#50924,#50925);
#42862=AXIS2_PLACEMENT_3D('',#76860,#50926,#50927);
#42863=AXIS2_PLACEMENT_3D('',#76861,#50928,#50929);
#42864=AXIS2_PLACEMENT_3D('',#76862,#50930,#50931);
#42865=AXIS2_PLACEMENT_3D('',#76865,#50933,#50934);
#42866=AXIS2_PLACEMENT_3D('',#76867,#50936,#50937);
#42867=AXIS2_PLACEMENT_3D('',#76884,#50939,#50940);
#42868=AXIS2_PLACEMENT_3D('',#76886,#50942,#50943);
#42869=AXIS2_PLACEMENT_3D('',#76888,#50945,#50946);
#42870=AXIS2_PLACEMENT_3D('',#76889,#50947,#50948);
#42871=AXIS2_PLACEMENT_3D('',#76890,#50949,#50950);
#42872=AXIS2_PLACEMENT_3D('',#76891,#50951,#50952);
#42873=AXIS2_PLACEMENT_3D('',#76892,#50953,#50954);
#42874=AXIS2_PLACEMENT_3D('',#76894,#50956,#50957);
#42875=AXIS2_PLACEMENT_3D('',#76895,#50958,#50959);
#42876=AXIS2_PLACEMENT_3D('',#76912,#50961,#50962);
#42877=AXIS2_PLACEMENT_3D('',#76914,#50964,#50965);
#42878=AXIS2_PLACEMENT_3D('',#76916,#50967,#50968);
#42879=AXIS2_PLACEMENT_3D('',#76917,#50969,#50970);
#42880=AXIS2_PLACEMENT_3D('',#76918,#50971,#50972);
#42881=AXIS2_PLACEMENT_3D('',#76919,#50973,#50974);
#42882=AXIS2_PLACEMENT_3D('',#76920,#50975,#50976);
#42883=AXIS2_PLACEMENT_3D('',#76921,#50977,#50978);
#42884=AXIS2_PLACEMENT_3D('',#76922,#50979,#50980);
#42885=AXIS2_PLACEMENT_3D('',#76924,#50982,#50983);
#42886=AXIS2_PLACEMENT_3D('',#76926,#50985,#50986);
#42887=AXIS2_PLACEMENT_3D('',#76927,#50987,#50988);
#42888=AXIS2_PLACEMENT_3D('',#76928,#50989,#50990);
#42889=AXIS2_PLACEMENT_3D('',#76929,#50991,#50992);
#42890=AXIS2_PLACEMENT_3D('',#76930,#50993,#50994);
#42891=AXIS2_PLACEMENT_3D('',#76931,#50995,#50996);
#42892=AXIS2_PLACEMENT_3D('',#76948,#50998,#50999);
#42893=AXIS2_PLACEMENT_3D('',#76950,#51001,#51002);
#42894=AXIS2_PLACEMENT_3D('',#76952,#51004,#51005);
#42895=AXIS2_PLACEMENT_3D('',#76953,#51006,#51007);
#42896=AXIS2_PLACEMENT_3D('',#76954,#51008,#51009);
#42897=AXIS2_PLACEMENT_3D('',#76955,#51010,#51011);
#42898=AXIS2_PLACEMENT_3D('',#76956,#51012,#51013);
#42899=AXIS2_PLACEMENT_3D('',#76957,#51014,#51015);
#42900=AXIS2_PLACEMENT_3D('',#76960,#51017,#51018);
#42901=AXIS2_PLACEMENT_3D('',#76962,#51020,#51021);
#42902=AXIS2_PLACEMENT_3D('',#76979,#51023,#51024);
#42903=AXIS2_PLACEMENT_3D('',#76981,#51026,#51027);
#42904=AXIS2_PLACEMENT_3D('',#76983,#51029,#51030);
#42905=AXIS2_PLACEMENT_3D('',#76984,#51031,#51032);
#42906=AXIS2_PLACEMENT_3D('',#76985,#51033,#51034);
#42907=AXIS2_PLACEMENT_3D('',#76986,#51035,#51036);
#42908=AXIS2_PLACEMENT_3D('',#76987,#51037,#51038);
#42909=AXIS2_PLACEMENT_3D('',#76988,#51039,#51040);
#42910=AXIS2_PLACEMENT_3D('',#77005,#51042,#51043);
#42911=AXIS2_PLACEMENT_3D('',#77007,#51045,#51046);
#42912=AXIS2_PLACEMENT_3D('',#77009,#51048,#51049);
#42913=AXIS2_PLACEMENT_3D('',#77010,#51050,#51051);
#42914=AXIS2_PLACEMENT_3D('',#77011,#51052,#51053);
#42915=AXIS2_PLACEMENT_3D('',#77012,#51054,#51055);
#42916=AXIS2_PLACEMENT_3D('',#77013,#51056,#51057);
#42917=AXIS2_PLACEMENT_3D('',#77020,#51058,#51059);
#42918=AXIS2_PLACEMENT_3D('',#77025,#51062,#51063);
#42919=AXIS2_PLACEMENT_3D('',#77028,#51065,#51066);
#42920=AXIS2_PLACEMENT_3D('',#77029,#51067,#51068);
#42921=AXIS2_PLACEMENT_3D('',#77031,#51070,#51071);
#42922=AXIS2_PLACEMENT_3D('',#77033,#51073,#51074);
#42923=AXIS2_PLACEMENT_3D('',#77034,#51075,#51076);
#42924=AXIS2_PLACEMENT_3D('',#77051,#51078,#51079);
#42925=AXIS2_PLACEMENT_3D('',#77052,#51080,#51081);
#42926=AXIS2_PLACEMENT_3D('',#77053,#51082,#51083);
#42927=AXIS2_PLACEMENT_3D('',#77054,#51084,#51085);
#42928=AXIS2_PLACEMENT_3D('',#77055,#51086,#51087);
#42929=AXIS2_PLACEMENT_3D('',#77056,#51088,#51089);
#42930=AXIS2_PLACEMENT_3D('',#77057,#51090,#51091);
#42931=AXIS2_PLACEMENT_3D('',#77058,#51092,#51093);
#42932=AXIS2_PLACEMENT_3D('',#77059,#51094,#51095);
#42933=AXIS2_PLACEMENT_3D('',#77060,#51096,#51097);
#42934=AXIS2_PLACEMENT_3D('',#77061,#51098,#51099);
#42935=AXIS2_PLACEMENT_3D('',#77062,#51100,#51101);
#42936=AXIS2_PLACEMENT_3D('',#77063,#51102,#51103);
#42937=AXIS2_PLACEMENT_3D('',#77064,#51104,#51105);
#42938=AXIS2_PLACEMENT_3D('',#77065,#51106,#51107);
#42939=AXIS2_PLACEMENT_3D('',#77066,#51108,#51109);
#42940=AXIS2_PLACEMENT_3D('',#77067,#51110,#51111);
#42941=AXIS2_PLACEMENT_3D('',#77068,#51112,#51113);
#42942=AXIS2_PLACEMENT_3D('',#77069,#51114,#51115);
#42943=AXIS2_PLACEMENT_3D('',#77070,#51116,#51117);
#42944=AXIS2_PLACEMENT_3D('',#77071,#51118,#51119);
#42945=AXIS2_PLACEMENT_3D('',#77072,#51120,#51121);
#42946=AXIS2_PLACEMENT_3D('',#77073,#51122,#51123);
#42947=AXIS2_PLACEMENT_3D('',#77074,#51124,#51125);
#42948=AXIS2_PLACEMENT_3D('',#77075,#51126,#51127);
#42949=AXIS2_PLACEMENT_3D('',#77076,#51128,#51129);
#42950=AXIS2_PLACEMENT_3D('',#77077,#51130,#51131);
#42951=AXIS2_PLACEMENT_3D('',#77078,#51132,#51133);
#42952=AXIS2_PLACEMENT_3D('',#77079,#51134,#51135);
#42953=AXIS2_PLACEMENT_3D('',#77080,#51136,#51137);
#42954=AXIS2_PLACEMENT_3D('',#77081,#51138,#51139);
#42955=AXIS2_PLACEMENT_3D('',#77082,#51140,#51141);
#42956=AXIS2_PLACEMENT_3D('',#77083,#51142,#51143);
#42957=AXIS2_PLACEMENT_3D('',#77084,#51144,#51145);
#42958=AXIS2_PLACEMENT_3D('',#77085,#51146,#51147);
#42959=AXIS2_PLACEMENT_3D('',#77086,#51148,#51149);
#42960=AXIS2_PLACEMENT_3D('',#77087,#51150,#51151);
#42961=AXIS2_PLACEMENT_3D('',#77088,#51152,#51153);
#42962=AXIS2_PLACEMENT_3D('',#77089,#51154,#51155);
#42963=AXIS2_PLACEMENT_3D('',#77090,#51156,#51157);
#42964=AXIS2_PLACEMENT_3D('',#77091,#51158,#51159);
#42965=AXIS2_PLACEMENT_3D('',#77092,#51160,#51161);
#42966=AXIS2_PLACEMENT_3D('',#77093,#51162,#51163);
#42967=AXIS2_PLACEMENT_3D('',#77094,#51164,#51165);
#42968=AXIS2_PLACEMENT_3D('',#77095,#51166,#51167);
#42969=AXIS2_PLACEMENT_3D('',#77096,#51168,#51169);
#42970=AXIS2_PLACEMENT_3D('',#77097,#51170,#51171);
#42971=AXIS2_PLACEMENT_3D('',#77098,#51172,#51173);
#42972=AXIS2_PLACEMENT_3D('',#77099,#51174,#51175);
#42973=AXIS2_PLACEMENT_3D('',#77100,#51176,#51177);
#42974=AXIS2_PLACEMENT_3D('',#77101,#51178,#51179);
#42975=AXIS2_PLACEMENT_3D('',#77102,#51180,#51181);
#42976=AXIS2_PLACEMENT_3D('',#77103,#51182,#51183);
#42977=AXIS2_PLACEMENT_3D('',#77104,#51184,#51185);
#42978=AXIS2_PLACEMENT_3D('',#77105,#51186,#51187);
#42979=AXIS2_PLACEMENT_3D('',#77106,#51188,#51189);
#42980=AXIS2_PLACEMENT_3D('',#77107,#51190,#51191);
#42981=AXIS2_PLACEMENT_3D('',#77108,#51192,#51193);
#42982=AXIS2_PLACEMENT_3D('',#77109,#51194,#51195);
#42983=AXIS2_PLACEMENT_3D('',#77110,#51196,#51197);
#42984=AXIS2_PLACEMENT_3D('',#77111,#51198,#51199);
#42985=AXIS2_PLACEMENT_3D('',#77112,#51200,#51201);
#42986=AXIS2_PLACEMENT_3D('',#77113,#51202,#51203);
#42987=AXIS2_PLACEMENT_3D('',#77114,#51204,#51205);
#42988=AXIS2_PLACEMENT_3D('',#77115,#51206,#51207);
#42989=AXIS2_PLACEMENT_3D('',#77116,#51208,#51209);
#42990=AXIS2_PLACEMENT_3D('',#77117,#51210,#51211);
#42991=AXIS2_PLACEMENT_3D('',#77118,#51212,#51213);
#42992=AXIS2_PLACEMENT_3D('',#77119,#51214,#51215);
#42993=AXIS2_PLACEMENT_3D('',#77120,#51216,#51217);
#42994=AXIS2_PLACEMENT_3D('',#77121,#51218,#51219);
#42995=AXIS2_PLACEMENT_3D('',#77122,#51220,#51221);
#42996=AXIS2_PLACEMENT_3D('',#77123,#51222,#51223);
#42997=AXIS2_PLACEMENT_3D('',#77125,#51225,#51226);
#46177=DIRECTION('axis',(0.,0.,1.));
#46178=DIRECTION('refdir',(1.,0.,0.));
#46179=DIRECTION('center_axis',(0.,6.12323399573677E-17,1.));
#46180=DIRECTION('ref_axis',(0.707106781186561,0.707106781186534,0.));
#46181=DIRECTION('center_axis',(0.,0.,-1.));
#46182=DIRECTION('ref_axis',(0.,1.,0.));
#46183=DIRECTION('',(0.,-6.12323399573677E-17,-1.));
#46184=DIRECTION('center_axis',(0.,0.707106781186544,-0.707106781186551));
#46185=DIRECTION('ref_axis',(4.08878244448902E-17,0.707106781186551,0.707106781186544));
#46186=DIRECTION('',(0.,6.12323399573677E-17,1.));
#46187=DIRECTION('center_axis',(0.706796314700322,0.,-0.707417111417333));
#46188=DIRECTION('ref_axis',(0.,1.,0.));
#46189=DIRECTION('center_axis',(-0.706790970013431,0.,0.707422451373628));
#46190=DIRECTION('ref_axis',(0.707106781191854,-0.0298705971533445,0.706475581614962));
#46191=DIRECTION('center_axis',(0.,0.,1.));
#46192=DIRECTION('ref_axis',(1.,0.,0.));
#46193=DIRECTION('center_axis',(0.,0.999107349012797,0.0422434036107608));
#46194=DIRECTION('ref_axis',(0.,-0.0422434036107608,0.999107349012797));
#46195=DIRECTION('center_axis',(0.,-0.130526192220051,0.99144486137381));
#46196=DIRECTION('ref_axis',(-0.707106781186556,-0.701057384649969,-0.0922959556412579));
#46197=DIRECTION('center_axis',(0.,0.130526192220054,-0.99144486137381));
#46198=DIRECTION('ref_axis',(0.,-0.99144486137381,-0.130526192220054));
#46199=DIRECTION('',(0.,0.130526192220051,-0.991444861373811));
#46200=DIRECTION('center_axis',(0.,-0.608761429008712,-0.793353340291242));
#46201=DIRECTION('ref_axis',(-1.63551297779562E-16,-0.793353340291242,0.608761429008711));
#46202=DIRECTION('',(0.,-0.130526192220051,0.991444861373811));
#46203=DIRECTION('center_axis',(1.,0.,0.));
#46204=DIRECTION('ref_axis',(0.,0.,-1.));
#46205=DIRECTION('center_axis',(1.,0.,0.));
#46206=DIRECTION('ref_axis',(0.,-0.0613490884647565,0.998116370642494));
#46207=DIRECTION('center_axis',(-1.22556994625176E-14,0.996041880624797,
0.0888851620992961));
#46208=DIRECTION('ref_axis',(-0.707106781186568,-0.0628513008672846,0.704307968135574));
#46209=DIRECTION('center_axis',(-1.,0.,0.));
#46210=DIRECTION('ref_axis',(0.,-0.0613490884647565,0.998116370642494));
#46211=DIRECTION('center_axis',(-1.,0.,0.));
#46212=DIRECTION('ref_axis',(0.,0.692139864205962,0.721763401937888));
#46213=DIRECTION('',(1.,0.,0.));
#46214=DIRECTION('center_axis',(-1.,0.,0.));
#46215=DIRECTION('ref_axis',(0.,-0.0418848167539273,0.999122446012244));
#46216=DIRECTION('',(-1.,0.,0.));
#46217=DIRECTION('center_axis',(-0.70679631470526,0.0923364618639821,-0.701365059957726));
#46218=DIRECTION('ref_axis',(0.,-0.991444861373808,-0.130526192220071));
#46219=DIRECTION('center_axis',(0.706790970014367,-0.0923371588686554,0.70137035423392));
#46220=DIRECTION('ref_axis',(-0.707106781190918,-0.0625985175108842,0.704330480384924));
#46221=DIRECTION('center_axis',(0.,0.,1.));
#46222=DIRECTION('ref_axis',(1.,0.,0.));
#46223=DIRECTION('center_axis',(-1.,0.,0.));
#46224=DIRECTION('ref_axis',(0.,-0.780427540257714,0.625246235020487));
#46225=DIRECTION('center_axis',(0.,0.,1.));
#46226=DIRECTION('ref_axis',(1.,0.,0.));
#46227=DIRECTION('center_axis',(0.,-0.996073717759274,-0.0885276724488873));
#46228=DIRECTION('ref_axis',(0.,-0.0885276724488874,0.996073717759274));
#46229=DIRECTION('center_axis',(0.172056328312398,-0.893396984377419,0.415016202325873));
#46230=DIRECTION('ref_axis',(0.34214448757159,0.449268102924444,0.825284993998464));
#46231=DIRECTION('center_axis',(0.,0.999122446012245,0.0418848167539202));
#46232=DIRECTION('ref_axis',(0.,-0.0418848167539202,0.999122446012244));
#46233=DIRECTION('center_axis',(0.,-1.,6.12323399573677E-17));
#46234=DIRECTION('ref_axis',(1.,0.,0.));
#46235=DIRECTION('',(1.,0.,0.));
#46236=DIRECTION('center_axis',(0.,-1.,6.12323399573677E-17));
#46237=DIRECTION('ref_axis',(-0.707106781186568,0.,0.707106781186527));
#46238=DIRECTION('',(0.,-6.12323399573677E-17,-1.));
#46239=DIRECTION('',(-0.706902428155817,0.,-0.707311075176552));
#46240=DIRECTION('center_axis',(1.,0.,0.));
#46241=DIRECTION('ref_axis',(0.,0.,-1.));
#46242=DIRECTION('',(0.,1.,-6.12323399573677E-17));
#46243=DIRECTION('center_axis',(-1.,0.,0.));
#46244=DIRECTION('ref_axis',(0.,-0.0654031292301429,0.997858923238603));
#46245=DIRECTION('',(0.,-0.130526192220051,0.991444861373811));
#46246=DIRECTION('',(0.,0.991444861373811,0.130526192220051));
#46247=DIRECTION('',(0.,-0.130526192220051,0.991444861373811));
#46248=DIRECTION('center_axis',(-1.,0.,0.));
#46249=DIRECTION('ref_axis',(0.,-0.195090322016128,0.98078528040323));
#46250=DIRECTION('',(0.,0.258819045102521,-0.965925826289068));
#46251=DIRECTION('',(0.,0.965925826289068,0.258819045102521));
#46252=DIRECTION('',(0.,-0.258819045102521,0.965925826289068));
#46253=DIRECTION('center_axis',(-1.,0.,0.));
#46254=DIRECTION('ref_axis',(0.,-0.321439465303161,0.946930129495106));
#46255=DIRECTION('',(0.,0.38268343236509,-0.923879532511287));
#46256=DIRECTION('',(0.,0.923879532511287,0.38268343236509));
#46257=DIRECTION('',(0.,0.38268343236509,-0.923879532511287));
#46258=DIRECTION('center_axis',(-1.,0.,0.));
#46259=DIRECTION('ref_axis',(0.,-0.442288690219001,0.896872741532688));
#46260=DIRECTION('',(0.,-0.5,0.866025403784439));
#46261=DIRECTION('',(0.,0.866025403784439,0.5));
#46262=DIRECTION('',(0.,-0.5,0.866025403784439));
#46263=DIRECTION('center_axis',(-1.,0.,0.));
#46264=DIRECTION('ref_axis',(0.,-0.555570233019602,0.831469612302545));
#46265=DIRECTION('',(0.,0.60876142900872,-0.793353340291235));
#46266=DIRECTION('',(0.,0.793353340291235,0.60876142900872));
#46267=DIRECTION('',(0.,-0.60876142900872,0.793353340291235));
#46268=DIRECTION('center_axis',(-1.,0.,0.));
#46269=DIRECTION('ref_axis',(0.,-0.659345815100068,0.751839807478978));
#46270=DIRECTION('',(0.,0.707106781186547,-0.707106781186548));
#46271=DIRECTION('',(0.,0.707106781186548,0.707106781186547));
#46272=DIRECTION('',(0.,0.707106781186547,-0.707106781186548));
#46273=DIRECTION('center_axis',(-1.,0.,0.));
#46274=DIRECTION('ref_axis',(0.,-0.751839807478977,0.659345815100069));
#46275=DIRECTION('',(0.,-0.793353340291235,0.608761429008721));
#46276=DIRECTION('',(0.,0.608761429008721,0.793353340291235));
#46277=DIRECTION('',(0.,-0.793353340291235,0.608761429008721));
#46278=DIRECTION('center_axis',(-1.,0.,0.));
#46279=DIRECTION('ref_axis',(0.,-0.831469612302545,0.555570233019602));
#46280=DIRECTION('',(0.,0.866025403784438,-0.5));
#46281=DIRECTION('',(0.,0.5,0.866025403784438));
#46282=DIRECTION('',(0.,-0.866025403784438,0.5));
#46283=DIRECTION('center_axis',(-1.,0.,0.));
#46284=DIRECTION('ref_axis',(0.,-0.896872741532688,0.442288690219002));
#46285=DIRECTION('',(0.,0.923879532511287,-0.38268343236509));
#46286=DIRECTION('',(0.,0.38268343236509,0.923879532511287));
#46287=DIRECTION('',(0.,0.923879532511287,-0.38268343236509));
#46288=DIRECTION('center_axis',(-1.,0.,0.));
#46289=DIRECTION('ref_axis',(0.,-0.946930129495106,0.321439465303162));
#46290=DIRECTION('',(0.,-0.965925826289068,0.258819045102521));
#46291=DIRECTION('',(0.,0.258819045102521,0.965925826289068));
#46292=DIRECTION('',(0.,-0.965925826289068,0.258819045102521));
#46293=DIRECTION('center_axis',(-1.,0.,0.));
#46294=DIRECTION('ref_axis',(0.,-0.98078528040323,0.195090322016129));
#46295=DIRECTION('',(0.,0.99144486137381,-0.130526192220052));
#46296=DIRECTION('',(0.,0.130526192220052,0.99144486137381));
#46297=DIRECTION('',(0.,-0.99144486137381,0.130526192220052));
#46298=DIRECTION('center_axis',(-1.,0.,0.));
#46299=DIRECTION('ref_axis',(0.,-0.997858923238603,0.0654031292301436));
#46300=DIRECTION('',(0.,1.,-1.22464679914735E-16));
#46301=DIRECTION('',(0.,1.22464679914735E-16,1.));
#46302=DIRECTION('',(0.,1.,-1.22464679914735E-16));
#46303=DIRECTION('center_axis',(-1.,0.,0.));
#46304=DIRECTION('ref_axis',(0.,-0.997858923238603,-0.0654031292301433));
#46305=DIRECTION('',(0.,-0.991444861373811,-0.130526192220051));
#46306=DIRECTION('',(0.,-0.130526192220051,0.991444861373811));
#46307=DIRECTION('',(0.,-0.991444861373811,-0.130526192220051));
#46308=DIRECTION('center_axis',(-1.,0.,0.));
#46309=DIRECTION('ref_axis',(0.,-0.980785280403231,-0.195090322016127));
#46310=DIRECTION('',(0.,0.965925826289068,0.25881904510252));
#46311=DIRECTION('',(0.,-0.25881904510252,0.965925826289068));
#46312=DIRECTION('',(0.,-0.965925826289068,-0.25881904510252));
#46313=DIRECTION('center_axis',(-1.,0.,0.));
#46314=DIRECTION('ref_axis',(0.,-0.946930129495106,-0.321439465303161));
#46315=DIRECTION('',(0.,0.923879532511287,0.382683432365089));
#46316=DIRECTION('',(0.,-0.382683432365089,0.923879532511287));
#46317=DIRECTION('',(0.,0.923879532511287,0.382683432365089));
#46318=DIRECTION('center_axis',(-1.,0.,0.));
#46319=DIRECTION('ref_axis',(0.,-0.896872741532689,-0.442288690219));
#46320=DIRECTION('',(0.,-0.866025403784439,-0.5));
#46321=DIRECTION('',(0.,-0.5,0.866025403784439));
#46322=DIRECTION('',(0.,-0.866025403784439,-0.5));
#46323=DIRECTION('center_axis',(-1.,0.,0.));
#46324=DIRECTION('ref_axis',(0.,-0.831469612302545,-0.555570233019602));
#46325=DIRECTION('',(0.,0.793353340291235,0.60876142900872));
#46326=DIRECTION('',(0.,-0.60876142900872,0.793353340291235));
#46327=DIRECTION('',(0.,-0.793353340291235,-0.60876142900872));
#46328=DIRECTION('center_axis',(-1.,0.,0.));
#46329=DIRECTION('ref_axis',(0.,-0.751839807478978,-0.659345815100068));
#46330=DIRECTION('',(0.,0.707106781186548,0.707106781186547));
#46331=DIRECTION('',(0.,-0.707106781186547,0.707106781186548));
#46332=DIRECTION('',(0.,0.707106781186548,0.707106781186547));
#46333=DIRECTION('center_axis',(-1.,0.,0.));
#46334=DIRECTION('ref_axis',(0.,-0.659345815100069,-0.751839807478977));
#46335=DIRECTION('',(0.,-0.608761429008721,-0.793353340291235));
#46336=DIRECTION('',(0.,-0.793353340291235,0.608761429008721));
#46337=DIRECTION('',(0.,0.608761429008721,0.793353340291235));
#46338=DIRECTION('center_axis',(-1.,0.,0.));
#46339=DIRECTION('ref_axis',(0.,-0.555570233019602,-0.831469612302545));
#46340=DIRECTION('',(0.,0.5,0.866025403784438));
#46341=DIRECTION('',(0.,-0.866025403784438,0.5));
#46342=DIRECTION('',(0.,-0.5,-0.866025403784438));
#46343=DIRECTION('center_axis',(-1.,0.,0.));
#46344=DIRECTION('ref_axis',(0.,-0.442288690219002,-0.896872741532688));
#46345=DIRECTION('',(0.,0.38268343236509,0.923879532511286));
#46346=DIRECTION('',(0.,-0.923879532511286,0.38268343236509));
#46347=DIRECTION('',(0.,0.38268343236509,0.923879532511286));
#46348=DIRECTION('center_axis',(-1.,0.,0.));
#46349=DIRECTION('ref_axis',(0.,-0.321439465303162,-0.946930129495106));
#46350=DIRECTION('',(0.,-0.258819045102522,-0.965925826289068));
#46351=DIRECTION('',(0.,-0.965925826289068,0.258819045102522));
#46352=DIRECTION('',(0.,-0.258819045102522,-0.965925826289068));
#46353=DIRECTION('center_axis',(-1.,0.,0.));
#46354=DIRECTION('ref_axis',(0.,-0.19509032201613,-0.98078528040323));
#46355=DIRECTION('',(0.,0.130526192220052,0.99144486137381));
#46356=DIRECTION('',(0.,-0.99144486137381,0.130526192220052));
#46357=DIRECTION('',(0.,-0.130526192220052,-0.99144486137381));
#46358=DIRECTION('center_axis',(-1.,0.,0.));
#46359=DIRECTION('ref_axis',(0.,-0.0654031292301437,-0.997858923238603));
#46360=DIRECTION('',(0.,1.83697019872103E-16,1.));
#46361=DIRECTION('',(0.,-1.,1.83697019872103E-16));
#46362=DIRECTION('',(0.,1.83697019872103E-16,1.));
#46363=DIRECTION('center_axis',(-1.,0.,0.));
#46364=DIRECTION('ref_axis',(0.,0.0654031292301432,-0.997858923238603));
#46365=DIRECTION('',(0.,0.130526192220051,-0.991444861373811));
#46366=DIRECTION('',(0.,-0.991444861373811,-0.130526192220051));
#46367=DIRECTION('',(0.,0.130526192220051,-0.991444861373811));
#46368=DIRECTION('center_axis',(-1.,0.,0.));
#46369=DIRECTION('ref_axis',(0.,0.195090322016127,-0.980785280403231));
#46370=DIRECTION('',(0.,-0.25881904510252,0.965925826289068));
#46371=DIRECTION('',(0.,-0.965925826289068,-0.25881904510252));
#46372=DIRECTION('',(0.,0.25881904510252,-0.965925826289068));
#46373=DIRECTION('center_axis',(-1.,0.,0.));
#46374=DIRECTION('ref_axis',(0.,0.321439465303161,-0.946930129495106));
#46375=DIRECTION('',(0.,-0.382683432365089,0.923879532511287));
#46376=DIRECTION('',(0.,-0.923879532511287,-0.382683432365089));
#46377=DIRECTION('',(0.,-0.382683432365089,0.923879532511287));
#46378=DIRECTION('center_axis',(-1.,0.,0.));
#46379=DIRECTION('ref_axis',(0.,0.442288690219,-0.896872741532689));
#46380=DIRECTION('',(0.,0.499999999999999,-0.866025403784439));
#46381=DIRECTION('',(0.,-0.866025403784439,-0.499999999999999));
#46382=DIRECTION('',(0.,0.499999999999999,-0.866025403784439));
#46383=DIRECTION('center_axis',(-1.,0.,0.));
#46384=DIRECTION('ref_axis',(0.,0.555570233019602,-0.831469612302546));
#46385=DIRECTION('',(0.,-0.60876142900872,0.793353340291236));
#46386=DIRECTION('',(0.,-0.793353340291236,-0.60876142900872));
#46387=DIRECTION('',(0.,-0.60876142900872,0.793353340291236));
#46388=DIRECTION('center_axis',(-1.,0.,0.));
#46389=DIRECTION('ref_axis',(0.,0.659345815100068,-0.751839807478978));
#46390=DIRECTION('',(0.,-0.707106781186547,0.707106781186548));
#46391=DIRECTION('',(0.,-0.707106781186548,-0.707106781186547));
#46392=DIRECTION('',(0.,-0.707106781186547,0.707106781186548));
#46393=DIRECTION('center_axis',(-1.,0.,0.));
#46394=DIRECTION('ref_axis',(0.,0.751839807478977,-0.65934581510007));
#46395=DIRECTION('',(0.,0.793353340291235,-0.608761429008721));
#46396=DIRECTION('',(0.,-0.608761429008721,-0.793353340291235));
#46397=DIRECTION('',(0.,0.793353340291235,-0.608761429008721));
#46398=DIRECTION('center_axis',(-1.,0.,0.));
#46399=DIRECTION('ref_axis',(0.,0.831469612302545,-0.555570233019602));
#46400=DIRECTION('',(0.,-0.866025403784438,0.5));
#46401=DIRECTION('',(0.,-0.5,-0.866025403784438));
#46402=DIRECTION('',(0.,0.866025403784438,-0.5));
#46403=DIRECTION('center_axis',(-1.,0.,0.));
#46404=DIRECTION('ref_axis',(0.,0.896872741532688,-0.442288690219002));
#46405=DIRECTION('',(0.,-0.923879532511286,0.38268343236509));
#46406=DIRECTION('',(0.,-0.38268343236509,-0.923879532511286));
#46407=DIRECTION('',(0.,-0.923879532511286,0.38268343236509));
#46408=DIRECTION('center_axis',(-1.,0.,0.));
#46409=DIRECTION('ref_axis',(0.,0.946930129495106,-0.321439465303162));
#46410=DIRECTION('',(0.,0.965925826289068,-0.258819045102522));
#46411=DIRECTION('',(0.,-0.258819045102522,-0.965925826289068));
#46412=DIRECTION('',(0.,0.965925826289068,-0.258819045102522));
#46413=DIRECTION('center_axis',(-1.,0.,0.));
#46414=DIRECTION('ref_axis',(0.,0.98078528040323,-0.19509032201613));
#46415=DIRECTION('',(0.,-0.99144486137381,0.130526192220053));
#46416=DIRECTION('',(0.,-0.130526192220053,-0.99144486137381));
#46417=DIRECTION('',(0.,-0.99144486137381,0.130526192220053));
#46418=DIRECTION('center_axis',(-1.,0.,0.));
#46419=DIRECTION('ref_axis',(0.,0.998116759314604,-0.0613427646533231));
#46420=DIRECTION('',(0.,-1.,0.));
#46421=DIRECTION('',(0.,0.,-1.));
#46422=DIRECTION('',(0.,-1.,0.));
#46423=DIRECTION('center_axis',(-1.,0.,0.));
#46424=DIRECTION('ref_axis',(0.,0.997858923238603,0.0654031292301429));
#46425=DIRECTION('',(0.,-0.99144486137381,-0.130526192220052));
#46426=DIRECTION('',(0.,0.130526192220052,-0.99144486137381));
#46427=DIRECTION('',(0.,-0.99144486137381,-0.130526192220052));
#46428=DIRECTION('center_axis',(-1.,0.,0.));
#46429=DIRECTION('ref_axis',(0.,0.98078528040323,0.195090322016128));
#46430=DIRECTION('',(0.,-0.965925826289068,-0.258819045102521));
#46431=DIRECTION('',(0.,0.258819045102521,-0.965925826289068));
#46432=DIRECTION('',(0.,-0.965925826289068,-0.258819045102521));
#46433=DIRECTION('center_axis',(-1.,0.,0.));
#46434=DIRECTION('ref_axis',(0.,0.946930129495106,0.321439465303162));
#46435=DIRECTION('',(0.,-0.923879532511287,-0.38268343236509));
#46436=DIRECTION('',(0.,0.38268343236509,-0.923879532511287));
#46437=DIRECTION('',(0.,-0.923879532511287,-0.38268343236509));
#46438=DIRECTION('center_axis',(-1.,0.,0.));
#46439=DIRECTION('ref_axis',(0.,0.896872741532688,0.442288690219001));
#46440=DIRECTION('',(0.,0.866025403784439,0.5));
#46441=DIRECTION('',(0.,0.5,-0.866025403784439));
#46442=DIRECTION('',(0.,0.866025403784439,0.5));
#46443=DIRECTION('center_axis',(-1.,0.,0.));
#46444=DIRECTION('ref_axis',(0.,0.831469612302545,0.555570233019602));
#46445=DIRECTION('',(0.,-0.793353340291235,-0.608761429008721));
#46446=DIRECTION('',(0.,0.608761429008721,-0.793353340291235));
#46447=DIRECTION('',(0.,0.793353340291235,0.608761429008721));
#46448=DIRECTION('center_axis',(-1.,0.,0.));
#46449=DIRECTION('ref_axis',(0.,0.751839807478977,0.659345815100069));
#46450=DIRECTION('',(0.,-0.707106781186548,-0.707106781186548));
#46451=DIRECTION('',(0.,0.707106781186548,-0.707106781186548));
#46452=DIRECTION('',(0.,-0.707106781186548,-0.707106781186548));
#46453=DIRECTION('center_axis',(-1.,0.,0.));
#46454=DIRECTION('ref_axis',(0.,0.659345815100069,0.751839807478978));
#46455=DIRECTION('',(0.,0.608761429008721,0.793353340291235));
#46456=DIRECTION('',(0.,0.793353340291235,-0.608761429008721));
#46457=DIRECTION('',(0.,0.608761429008721,0.793353340291235));
#46458=DIRECTION('center_axis',(-1.,0.,0.));
#46459=DIRECTION('ref_axis',(0.,0.555570233019602,0.831469612302545));
#46460=DIRECTION('',(0.,-0.5,-0.866025403784439));
#46461=DIRECTION('',(0.,0.866025403784439,-0.5));
#46462=DIRECTION('',(0.,0.5,0.866025403784439));
#46463=DIRECTION('center_axis',(-1.,0.,0.));
#46464=DIRECTION('ref_axis',(0.,0.442288690219001,0.896872741532688));
#46465=DIRECTION('',(0.,-0.38268343236509,-0.923879532511287));
#46466=DIRECTION('',(0.,0.923879532511287,-0.38268343236509));
#46467=DIRECTION('',(0.,-0.38268343236509,-0.923879532511287));
#46468=DIRECTION('center_axis',(-1.,0.,0.));
#46469=DIRECTION('ref_axis',(0.,0.321439465303162,0.946930129495106));
#46470=DIRECTION('',(0.,0.258819045102521,0.965925826289068));
#46471=DIRECTION('',(0.,0.965925826289068,-0.258819045102521));
#46472=DIRECTION('',(0.,0.258819045102521,0.965925826289068));
#46473=DIRECTION('center_axis',(-1.,0.,0.));
#46474=DIRECTION('ref_axis',(0.,0.195090322016129,0.98078528040323));
#46475=DIRECTION('',(0.,-0.130526192220052,-0.99144486137381));
#46476=DIRECTION('',(0.,0.99144486137381,-0.130526192220052));
#46477=DIRECTION('',(0.,0.130526192220052,0.99144486137381));
#46478=DIRECTION('center_axis',(-1.,0.,0.));
#46479=DIRECTION('ref_axis',(0.,0.0654031292301431,0.997858923238603));
#46480=DIRECTION('',(0.,-6.12323399573677E-17,-1.));
#46481=DIRECTION('center_axis',(1.,0.,0.));
#46482=DIRECTION('ref_axis',(0.,-1.,1.83697019872103E-16));
#46483=DIRECTION('center_axis',(1.,0.,0.));
#46484=DIRECTION('ref_axis',(0.,0.,-1.));
#46485=DIRECTION('center_axis',(1.,0.,0.));
#46486=DIRECTION('ref_axis',(0.,-0.0654031292301429,0.997858923238603));
#46487=DIRECTION('center_axis',(0.,-0.996073717759274,-0.0885276724488873));
#46488=DIRECTION('ref_axis',(0.,-0.0885276724488873,0.996073717759274));
#46489=DIRECTION('center_axis',(-1.,0.,0.));
#46490=DIRECTION('ref_axis',(0.,1.,0.));
#46491=DIRECTION('center_axis',(-1.,0.,0.));
#46492=DIRECTION('ref_axis',(0.,-0.0613490884647565,0.998116370642494));
#46493=DIRECTION('center_axis',(1.,0.,0.));
#46494=DIRECTION('ref_axis',(0.,0.,-1.));
#46495=DIRECTION('center_axis',(1.,0.,0.));
#46496=DIRECTION('ref_axis',(0.,-0.0613490884647565,0.998116370642494));
#46497=DIRECTION('center_axis',(1.22556994625176E-14,0.996041880624797,
0.0888851620992961));
#46498=DIRECTION('ref_axis',(0.,-0.0888851620992961,0.996041880624797));
#46499=DIRECTION('center_axis',(1.,0.,0.));
#46500=DIRECTION('ref_axis',(0.,1.,0.));
#46501=DIRECTION('',(-1.,0.,0.));
#46502=DIRECTION('center_axis',(0.,-1.,1.22464679914735E-16));
#46503=DIRECTION('ref_axis',(0.707106781186561,0.,0.707106781186534));
#46504=DIRECTION('center_axis',(0.,1.,0.));
#46505=DIRECTION('ref_axis',(0.,0.,1.));
#46506=DIRECTION('center_axis',(0.,0.70710678118655,0.707106781186545));
#46507=DIRECTION('ref_axis',(4.08878244448901E-17,-0.707106781186545,0.70710678118655));
#46508=DIRECTION('',(0.,-1.,1.22464679914735E-16));
#46509=DIRECTION('center_axis',(0.706796314700278,0.707417111417378,0.));
#46510=DIRECTION('ref_axis',(0.,0.,1.));
#46511=DIRECTION('center_axis',(-0.706790970013365,-0.707422451373694,0.));
#46512=DIRECTION('ref_axis',(0.707106781191921,-0.706475581614895,-0.0298705971533335));
#46513=DIRECTION('center_axis',(0.429570054990526,-0.177774910040256,-0.885361874724463));
#46514=DIRECTION('ref_axis',(0.818074617559245,-0.33855512006305,0.464902517507045));
#46515=DIRECTION('center_axis',(0.,-0.0422434036107607,0.999107349012797));
#46516=DIRECTION('ref_axis',(0.,-0.999107349012797,-0.0422434036107607));
#46517=DIRECTION('center_axis',(0.,-0.99144486137381,-0.130526192220051));
#46518=DIRECTION('ref_axis',(-0.707106781186561,0.0922959556412554,-0.701057384649965));
#46519=DIRECTION('center_axis',(1.46763321699137E-14,0.991444861373812,
0.130526192220041));
#46520=DIRECTION('ref_axis',(0.,0.130526192220041,-0.991444861373812));
#46521=DIRECTION('',(0.,0.991444861373811,0.130526192220051));
#46522=DIRECTION('center_axis',(0.,0.793353340291235,-0.608761429008721));
#46523=DIRECTION('ref_axis',(-8.17756488897799E-17,-0.608761429008721,-0.793353340291235));
#46524=DIRECTION('',(0.,-0.991444861373811,-0.130526192220051));
#46525=DIRECTION('center_axis',(1.,0.,0.));
#46526=DIRECTION('ref_axis',(0.,0.,-1.));
#46527=DIRECTION('center_axis',(1.,0.,0.));
#46528=DIRECTION('ref_axis',(0.,-0.998116370642494,-0.0613490884647563));
#46529=DIRECTION('center_axis',(2.68645784048061E-14,-0.0888851620992943,
0.996041880624797));
#46530=DIRECTION('ref_axis',(-0.707106781186562,-0.704307968135583,-0.0628513008672563));
#46531=DIRECTION('center_axis',(-1.,0.,0.));
#46532=DIRECTION('ref_axis',(0.,-0.998116370642494,-0.0613490884647564));
#46533=DIRECTION('center_axis',(-1.,0.,0.));
#46534=DIRECTION('ref_axis',(0.,-0.721763401937886,0.692139864205963));
#46535=DIRECTION('',(1.,0.,0.));
#46536=DIRECTION('center_axis',(-1.,0.,0.));
#46537=DIRECTION('ref_axis',(0.,-0.999122446012244,-0.0418848167539273));
#46538=DIRECTION('',(-1.,0.,0.));
#46539=DIRECTION('center_axis',(-0.70679631470526,0.701365059957728,0.0923364618639608));
#46540=DIRECTION('ref_axis',(0.,0.130526192220041,-0.991444861373812));
#46541=DIRECTION('center_axis',(0.706790970014397,-0.701370354233891,-0.0923371588686514));
#46542=DIRECTION('ref_axis',(-0.707106781190889,-0.704330480384954,-0.0625985175108834));
#46543=DIRECTION('center_axis',(-0.939647353856842,0.276579550719404,0.201411525275212));
#46544=DIRECTION('ref_axis',(-0.34214448759234,-0.759583311697392,-0.553145859788354));
#46545=DIRECTION('center_axis',(-1.,0.,0.));
#46546=DIRECTION('ref_axis',(0.,-0.625246235020487,-0.780427540257714));
#46547=DIRECTION('center_axis',(0.,0.,1.));
#46548=DIRECTION('ref_axis',(-0.923502716556039,0.38359188275251,0.));
#46549=DIRECTION('center_axis',(0.,0.0885276724488872,-0.996073717759274));
#46550=DIRECTION('ref_axis',(0.,-0.996073717759274,-0.0885276724488872));
#46551=DIRECTION('center_axis',(-0.93964735386447,-0.300502853768194,0.163587546141727));
#46552=DIRECTION('ref_axis',(0.3421444875714,-0.825284993998558,0.449268102924417));
#46553=DIRECTION('center_axis',(0.,-0.04188481675392,0.999122446012245));
#46554=DIRECTION('ref_axis',(0.,-0.999122446012244,-0.04188481675392));
#46555=DIRECTION('center_axis',(0.,-1.22464679914735E-16,-1.));
#46556=DIRECTION('ref_axis',(1.,0.,0.));
#46557=DIRECTION('',(1.,0.,0.));
#46558=DIRECTION('center_axis',(0.,-1.22464679914735E-16,-1.));
#46559=DIRECTION('ref_axis',(-0.707106781186568,-0.707106781186527,8.65956056235502E-17));
#46560=DIRECTION('',(0.,1.,-1.22464679914735E-16));
#46561=DIRECTION('',(-0.706902428155817,0.707311075176552,0.));
#46562=DIRECTION('center_axis',(1.,0.,0.));
#46563=DIRECTION('ref_axis',(0.,0.,-1.));
#46564=DIRECTION('center_axis',(1.,0.,0.));
#46565=DIRECTION('ref_axis',(0.,-0.997858923238603,-0.0654031292301432));
#46566=DIRECTION('center_axis',(0.,0.0885276724488872,-0.996073717759274));
#46567=DIRECTION('ref_axis',(0.,-0.996073717759274,-0.0885276724488872));
#46568=DIRECTION('center_axis',(-1.,0.,0.));
#46569=DIRECTION('ref_axis',(0.,1.,0.));
#46570=DIRECTION('center_axis',(-1.,0.,0.));
#46571=DIRECTION('ref_axis',(0.,-0.998116370642494,-0.0613490884647563));
#46572=DIRECTION('center_axis',(1.,0.,0.));
#46573=DIRECTION('ref_axis',(0.,0.,-1.));
#46574=DIRECTION('center_axis',(1.,0.,0.));
#46575=DIRECTION('ref_axis',(0.,-0.998116370642494,-0.0613490884647564));
#46576=DIRECTION('center_axis',(-2.68645784048061E-14,-0.0888851620992943,
0.996041880624797));
#46577=DIRECTION('ref_axis',(0.,-0.996041880624797,-0.0888851620992943));
#46578=DIRECTION('center_axis',(1.,0.,0.));
#46579=DIRECTION('ref_axis',(0.,1.,0.));
#46580=DIRECTION('',(-1.,0.,0.));
#46581=DIRECTION('center_axis',(0.,-1.83697019872103E-16,-1.));
#46582=DIRECTION('ref_axis',(0.707106781186561,-0.707106781186534,0.));
#46583=DIRECTION('center_axis',(0.,0.,1.));
#46584=DIRECTION('ref_axis',(0.,-1.,0.));
#46585=DIRECTION('center_axis',(0.,-0.707106781186549,0.707106781186546));
#46586=DIRECTION('ref_axis',(4.08878244448899E-17,-0.707106781186546,-0.707106781186549));
#46587=DIRECTION('',(0.,-1.83697019872103E-16,-1.));
#46588=DIRECTION('center_axis',(0.706796314700315,0.,0.70741711141734));
#46589=DIRECTION('ref_axis',(0.,-1.,0.));
#46590=DIRECTION('center_axis',(-0.706790970013431,0.,-0.707422451373628));
#46591=DIRECTION('ref_axis',(0.707106781191854,0.0298705971533399,-0.706475581614962));
#46592=DIRECTION('center_axis',(0.,0.,1.));
#46593=DIRECTION('ref_axis',(1.,0.,0.));
#46594=DIRECTION('center_axis',(0.,-0.999107349012797,-0.0422434036107607));
#46595=DIRECTION('ref_axis',(0.,0.0422434036107607,-0.999107349012797));
#46596=DIRECTION('center_axis',(0.,0.130526192220051,-0.99144486137381));
#46597=DIRECTION('ref_axis',(-0.707106781186559,0.701057384649968,0.0922959556412478));
#46598=DIRECTION('center_axis',(1.46763321699136E-14,-0.13052619222007,
0.991444861373808));
#46599=DIRECTION('ref_axis',(0.,0.991444861373808,0.13052619222007));
#46600=DIRECTION('',(0.,-0.130526192220051,0.991444861373811));
#46601=DIRECTION('center_axis',(0.,0.60876142900872,0.793353340291235));
#46602=DIRECTION('ref_axis',(0.,0.793353340291235,-0.60876142900872));
#46603=DIRECTION('',(0.,0.130526192220051,-0.991444861373811));
#46604=DIRECTION('center_axis',(1.,0.,0.));
#46605=DIRECTION('ref_axis',(0.,0.,-1.));
#46606=DIRECTION('center_axis',(1.,0.,0.));
#46607=DIRECTION('ref_axis',(0.,0.0613490884647572,-0.998116370642493));
#46608=DIRECTION('center_axis',(-1.30223461708592E-14,-0.996041880624797,
-0.088885162099298));
#46609=DIRECTION('ref_axis',(-0.707106781186568,0.0628513008672865,-0.704307968135574));
#46610=DIRECTION('center_axis',(-1.,0.,0.));
#46611=DIRECTION('ref_axis',(0.,0.0613490884647572,-0.998116370642494));
#46612=DIRECTION('center_axis',(-1.,0.,0.));
#46613=DIRECTION('ref_axis',(0.,-0.692139864205963,-0.721763401937886));
#46614=DIRECTION('',(1.,0.,0.));
#46615=DIRECTION('center_axis',(-1.,0.,0.));
#46616=DIRECTION('ref_axis',(0.,0.0418848167539273,-0.999122446012244));
#46617=DIRECTION('',(-1.,0.,0.));
#46618=DIRECTION('center_axis',(-0.706796314705261,-0.0923364618639611,
0.701365059957728));
#46619=DIRECTION('ref_axis',(0.,0.991444861373812,0.130526192220041));
#46620=DIRECTION('center_axis',(0.706790970014412,0.0923371588686494,-0.701370354233876));
#46621=DIRECTION('ref_axis',(-0.707106781190874,0.062598517510891,-0.704330480384968));
#46622=DIRECTION('center_axis',(0.,0.,1.));
#46623=DIRECTION('ref_axis',(1.,0.,0.));
#46624=DIRECTION('center_axis',(-1.,0.,0.));
#46625=DIRECTION('ref_axis',(0.,0.780427540257703,-0.625246235020501));
#46626=DIRECTION('center_axis',(0.,0.,1.));
#46627=DIRECTION('ref_axis',(1.,0.,0.));
#46628=DIRECTION('center_axis',(0.,0.996073717759274,0.0885276724488872));
#46629=DIRECTION('ref_axis',(0.,0.0885276724488872,-0.996073717759274));
#46630=DIRECTION('center_axis',(-0.172056328312399,-0.893396984377419,0.415016202325874));
#46631=DIRECTION('ref_axis',(0.342144487571596,-0.449268102924457,-0.825284993998455));
#46632=DIRECTION('center_axis',(0.,-0.999122446012245,-0.04188481675392));
#46633=DIRECTION('ref_axis',(0.,0.04188481675392,-0.999122446012244));
#46634=DIRECTION('center_axis',(0.,1.,-1.83697019872103E-16));
#46635=DIRECTION('ref_axis',(1.,0.,0.));
#46636=DIRECTION('',(1.,0.,0.));
#46637=DIRECTION('center_axis',(0.,1.,-1.83697019872103E-16));
#46638=DIRECTION('ref_axis',(-0.707106781186558,0.,-0.707106781186537));
#46639=DIRECTION('',(0.,1.83697019872103E-16,1.));
#46640=DIRECTION('',(-0.706902428155817,0.,0.707311075176552));
#46641=DIRECTION('center_axis',(1.,0.,0.));
#46642=DIRECTION('ref_axis',(0.,0.,-1.));
#46643=DIRECTION('center_axis',(1.,0.,0.));
#46644=DIRECTION('ref_axis',(0.,0.0654031292301432,-0.997858923238603));
#46645=DIRECTION('center_axis',(0.,0.996073717759274,0.0885276724488872));
#46646=DIRECTION('ref_axis',(0.,0.0885276724488872,-0.996073717759274));
#46647=DIRECTION('center_axis',(-1.,0.,0.));
#46648=DIRECTION('ref_axis',(0.,1.,0.));
#46649=DIRECTION('center_axis',(-1.,0.,0.));
#46650=DIRECTION('ref_axis',(0.,0.0613490884647572,-0.998116370642493));
#46651=DIRECTION('center_axis',(1.,0.,0.));
#46652=DIRECTION('ref_axis',(0.,0.,-1.));
#46653=DIRECTION('center_axis',(1.,0.,0.));
#46654=DIRECTION('ref_axis',(0.,0.0613490884647572,-0.998116370642494));
#46655=DIRECTION('center_axis',(1.30223461708592E-14,-0.996041880624797,
-0.088885162099298));
#46656=DIRECTION('ref_axis',(0.,0.088885162099298,-0.996041880624797));
#46657=DIRECTION('center_axis',(1.,0.,0.));
#46658=DIRECTION('ref_axis',(0.,1.,0.));
#46659=DIRECTION('',(-1.,0.,0.));
#46660=DIRECTION('center_axis',(0.,0.707106781186547,-0.707106781186548));
#46661=DIRECTION('ref_axis',(-0.707106781186556,0.499999999999994,0.499999999999994));
#46662=DIRECTION('center_axis',(0.,-0.707106781186548,0.707106781186548));
#46663=DIRECTION('ref_axis',(0.,0.707106781186547,0.707106781186547));
#46664=DIRECTION('',(0.,-0.707106781186547,0.707106781186548));
#46665=DIRECTION('center_axis',(0.,0.,1.));
#46666=DIRECTION('ref_axis',(4.088782444489E-17,1.,6.76379601470668E-31));
#46667=DIRECTION('',(0.,0.707106781186547,-0.707106781186548));
#46668=DIRECTION('center_axis',(-0.706796314703387,-0.50021943660843,0.50021943660843));
#46669=DIRECTION('ref_axis',(0.,0.707106781186547,0.707106781186547));
#46670=DIRECTION('center_axis',(0.706790970016761,0.500223212527551,-0.500223212527551));
#46671=DIRECTION('ref_axis',(-0.707106781188526,0.478431972699673,-0.520675376310329));
#46672=DIRECTION('center_axis',(0.,0.,1.));
#46673=DIRECTION('ref_axis',(1.,0.,0.));
#46674=DIRECTION('center_axis',(0.,0.736346178773833,0.676604984466694));
#46675=DIRECTION('ref_axis',(0.,0.676604984466694,-0.736346178773833));
#46676=DIRECTION('center_axis',(1.,0.,0.));
#46677=DIRECTION('ref_axis',(0.,0.,-1.));
#46678=DIRECTION('center_axis',(-1.,0.,0.));
#46679=DIRECTION('ref_axis',(0.,0.662394497621569,-0.749155210567656));
#46680=DIRECTION('center_axis',(3.37324551670366E-14,0.767159269002869,
0.641456667268323));
#46681=DIRECTION('ref_axis',(0.707106781186531,0.453578359262747,-0.542463521362071));
#46682=DIRECTION('center_axis',(1.,0.,0.));
#46683=DIRECTION('ref_axis',(0.,0.662394497621569,-0.749155210567656));
#46684=DIRECTION('center_axis',(1.,0.,0.));
#46685=DIRECTION('ref_axis',(0.,0.999780587432123,-0.0209470044130192));
#46686=DIRECTION('',(-1.,0.,0.));
#46687=DIRECTION('center_axis',(1.,0.,0.));
#46688=DIRECTION('ref_axis',(0.,0.676869218855479,-0.736103294766417));
#46689=DIRECTION('',(1.,0.,0.));
#46690=DIRECTION('center_axis',(0.,0.,1.));
#46691=DIRECTION('ref_axis',(1.,0.,0.));
#46692=DIRECTION('center_axis',(0.,0.736103294766404,0.676869218855492));
#46693=DIRECTION('ref_axis',(0.,0.676869218855492,-0.736103294766404));
#46694=DIRECTION('center_axis',(0.,0.60876142900872,-0.793353340291236));
#46695=DIRECTION('ref_axis',(0.707106781186568,-0.560985526796924,-0.430459334576854));
#46696=DIRECTION('center_axis',(0.,-0.60876142900871,0.793353340291244));
#46697=DIRECTION('ref_axis',(0.,-0.793353340291244,-0.60876142900871));
#46698=DIRECTION('center_axis',(0.,-0.991444861373811,0.130526192220051));
#46699=DIRECTION('ref_axis',(-1.2266347333467E-16,-0.130526192220051,-0.99144486137381));
#46700=DIRECTION('',(0.,0.60876142900872,-0.793353340291236));
#46701=DIRECTION('center_axis',(0.706796314705257,-0.430648251648579,0.561231728318249));
#46702=DIRECTION('ref_axis',(5.92118946466749E-14,-0.79335334029126,-0.608761429008688));
#46703=DIRECTION('center_axis',(-0.706790970016562,0.430651502409158,-0.5612359647918));
#46704=DIRECTION('ref_axis',(0.707106781188724,0.453773022653805,-0.542300695102404));
#46705=DIRECTION('center_axis',(0.,0.,1.));
#46706=DIRECTION('ref_axis',(1.,0.,0.));
#46707=DIRECTION('center_axis',(0.,-0.766928997900545,-0.641731962878012));
#46708=DIRECTION('ref_axis',(0.,0.641731962878012,-0.766928997900545));
#46709=DIRECTION('center_axis',(0.050484733373679,-0.98928852678309,-0.136965333101232));
#46710=DIRECTION('ref_axis',(0.342144487592483,0.145973322135736,-0.92823969901892));
#46711=DIRECTION('center_axis',(1.,0.,0.));
#46712=DIRECTION('ref_axis',(0.,-0.109729753246606,-0.993961458635313));
#46713=DIRECTION('center_axis',(1.,0.,0.));
#46714=DIRECTION('ref_axis',(0.,0.,-1.));
#46715=DIRECTION('center_axis',(-1.,0.,0.));
#46716=DIRECTION('ref_axis',(0.,0.659345815100069,-0.751839807478978));
#46717=DIRECTION('center_axis',(0.,-0.766928997900545,-0.641731962878012));
#46718=DIRECTION('ref_axis',(0.,0.641731962878012,-0.766928997900545));
#46719=DIRECTION('center_axis',(1.,0.,0.));
#46720=DIRECTION('ref_axis',(0.,0.659345815100068,-0.751839807478978));
#46721=DIRECTION('center_axis',(1.,0.,0.));
#46722=DIRECTION('ref_axis',(0.,1.,0.));
#46723=DIRECTION('center_axis',(1.,0.,0.));
#46724=DIRECTION('ref_axis',(0.,0.662394497621569,-0.749155210567656));
#46725=DIRECTION('center_axis',(1.,0.,0.));
#46726=DIRECTION('ref_axis',(0.,0.,-1.));
#46727=DIRECTION('center_axis',(-1.,0.,0.));
#46728=DIRECTION('ref_axis',(0.,0.662394497621569,-0.749155210567656));
#46729=DIRECTION('center_axis',(-3.37324551670366E-14,0.767159269002869,
0.641456667268323));
#46730=DIRECTION('ref_axis',(0.,0.641456667268323,-0.767159269002869));
#46731=DIRECTION('center_axis',(1.,0.,0.));
#46732=DIRECTION('ref_axis',(0.,1.,0.));
#46733=DIRECTION('',(1.,0.,0.));
#46734=DIRECTION('center_axis',(-1.,0.,0.));
#46735=DIRECTION('ref_axis',(0.,-0.109729753246601,-0.993961458635313));
#46736=DIRECTION('',(-1.,0.,0.));
#46737=DIRECTION('center_axis',(-1.,0.,0.));
#46738=DIRECTION('ref_axis',(0.,-0.109729753246606,-0.993961458635313));
#46739=DIRECTION('center_axis',(0.,0.793353340291236,0.60876142900872));
#46740=DIRECTION('ref_axis',(1.,0.,0.));
#46741=DIRECTION('',(1.,0.,0.));
#46742=DIRECTION('',(0.,-0.60876142900872,0.793353340291236));
#46743=DIRECTION('center_axis',(0.,-0.5,-0.866025403784438));
#46744=DIRECTION('ref_axis',(-0.70710678118656,0.612372435695785,-0.353553390593264));
#46745=DIRECTION('center_axis',(-7.40148683083439E-15,0.49999999999999,
0.866025403784444));
#46746=DIRECTION('ref_axis',(0.,0.866025403784444,-0.49999999999999));
#46747=DIRECTION('',(0.,0.5,0.866025403784438));
#46748=DIRECTION('center_axis',(0.,0.96592582628907,0.258819045102514));
#46749=DIRECTION('ref_axis',(4.08878244448897E-17,0.258819045102514,-0.96592582628907));
#46750=DIRECTION('',(0.,-0.5,-0.866025403784438));
#46751=DIRECTION('center_axis',(-0.706796314703078,0.353708555707291,0.612641189556832));
#46752=DIRECTION('ref_axis',(0.,0.866025403784438,-0.500000000000001));
#46753=DIRECTION('center_axis',(0.706790970016422,-0.353711225685321,-0.612645814094435));
#46754=DIRECTION('ref_axis',(-0.707106781188865,-0.379106486770089,-0.596890502257795));
#46755=DIRECTION('center_axis',(0.,0.,1.));
#46756=DIRECTION('ref_axis',(-0.858053385943048,0.513560499719041,0.));
#46757=DIRECTION('center_axis',(0.,0.844130643547427,-0.536137535175637));
#46758=DIRECTION('ref_axis',(0.,-0.536137535175637,-0.844130643547427));
#46759=DIRECTION('center_axis',(1.,0.,0.));
#46760=DIRECTION('ref_axis',(0.,0.,-1.));
#46761=DIRECTION('center_axis',(-1.,0.,0.));
#46762=DIRECTION('ref_axis',(0.,-0.552188054430745,-0.833719588677145));
#46763=DIRECTION('center_axis',(-5.53689289357882E-14,0.818154990804658,
-0.57499774870988));
#46764=DIRECTION('ref_axis',(0.707106781186565,-0.406584807279713,-0.578522942059599));
#46765=DIRECTION('center_axis',(1.,0.,0.));
#46766=DIRECTION('ref_axis',(0.,-0.552188054430745,-0.833719588677145));
#46767=DIRECTION('center_axis',(1.,0.,0.));
#46768=DIRECTION('ref_axis',(0.,0.238529004405318,-0.971135373703073));
#46769=DIRECTION('',(-1.,0.,0.));
#46770=DIRECTION('center_axis',(1.,0.,0.));
#46771=DIRECTION('ref_axis',(0.,-0.535834538347885,-0.844323011360882));
#46772=DIRECTION('',(1.,0.,0.));
#46773=DIRECTION('center_axis',(0.00806484247964557,-0.999722309028741,
0.0221418866861002));
#46774=DIRECTION('ref_axis',(-0.34214448758315,-0.0235649067522203,-0.93935182162288));
#46775=DIRECTION('center_axis',(0.,0.844323011360888,-0.535834538347877));
#46776=DIRECTION('ref_axis',(0.,-0.535834538347877,-0.844323011360888));
#46777=DIRECTION('center_axis',(0.,-0.608761429008721,-0.793353340291235));
#46778=DIRECTION('ref_axis',(0.707106781186559,-0.56098552679692,0.430459334576875));
#46779=DIRECTION('center_axis',(0.,0.608761429008721,0.793353340291235));
#46780=DIRECTION('ref_axis',(0.,-0.793353340291235,0.608761429008721));
#46781=DIRECTION('center_axis',(0.,-0.130526192220041,0.991444861373812));
#46782=DIRECTION('ref_axis',(-8.17756488897808E-17,-0.991444861373812,-0.130526192220041));
#46783=DIRECTION('',(0.,-0.608761429008721,-0.793353340291235));
#46784=DIRECTION('center_axis',(0.706796314705256,0.430648251648625,0.561231728318216));
#46785=DIRECTION('ref_axis',(0.,-0.793353340291247,0.608761429008705));
#46786=DIRECTION('center_axis',(-0.706790970016491,-0.430651502409201,-0.561235964791856));
#46787=DIRECTION('ref_axis',(0.707106781188796,-0.406377146597353,-0.578668829919337));
#46788=DIRECTION('center_axis',(0.,0.,1.));
#46789=DIRECTION('ref_axis',(1.,0.,0.));
#46790=DIRECTION('center_axis',(0.,-0.818361307397102,0.574704072158277));
#46791=DIRECTION('ref_axis',(0.,-0.574704072158277,-0.818361307397102));
#46792=DIRECTION('center_axis',(0.,0.,1.));
#46793=DIRECTION('ref_axis',(1.,0.,0.));
#46794=DIRECTION('center_axis',(1.,0.,0.));
#46795=DIRECTION('ref_axis',(0.,-0.988493193186426,-0.151265353019466));
#46796=DIRECTION('center_axis',(1.,0.,0.));
#46797=DIRECTION('ref_axis',(0.,0.,-1.));
#46798=DIRECTION('center_axis',(-1.,0.,0.));
#46799=DIRECTION('ref_axis',(0.,-0.555570233019602,-0.831469612302545));
#46800=DIRECTION('center_axis',(0.,-0.818361307397102,0.574704072158277));
#46801=DIRECTION('ref_axis',(0.,-0.574704072158277,-0.818361307397102));
#46802=DIRECTION('center_axis',(1.,0.,0.));
#46803=DIRECTION('ref_axis',(0.,-0.555570233019602,-0.831469612302545));
#46804=DIRECTION('center_axis',(1.,0.,0.));
#46805=DIRECTION('ref_axis',(0.,1.,0.));
#46806=DIRECTION('center_axis',(1.,0.,0.));
#46807=DIRECTION('ref_axis',(0.,-0.552188054430745,-0.833719588677145));
#46808=DIRECTION('center_axis',(1.,0.,0.));
#46809=DIRECTION('ref_axis',(0.,0.,-1.));
#46810=DIRECTION('center_axis',(-1.,0.,0.));
#46811=DIRECTION('ref_axis',(0.,-0.552188054430745,-0.833719588677145));
#46812=DIRECTION('center_axis',(5.53689289357882E-14,0.818154990804658,
-0.57499774870988));
#46813=DIRECTION('ref_axis',(0.,-0.57499774870988,-0.818154990804658));
#46814=DIRECTION('center_axis',(1.,0.,0.));
#46815=DIRECTION('ref_axis',(0.,1.,0.));
#46816=DIRECTION('',(1.,0.,0.));
#46817=DIRECTION('center_axis',(-1.,0.,0.));
#46818=DIRECTION('ref_axis',(0.,-0.988493193186426,-0.151265353019465));
#46819=DIRECTION('',(-1.,0.,0.));
#46820=DIRECTION('center_axis',(-1.,0.,0.));
#46821=DIRECTION('ref_axis',(0.,-0.988493193186426,-0.151265353019466));
#46822=DIRECTION('center_axis',(0.,0.793353340291235,-0.608761429008721));
#46823=DIRECTION('ref_axis',(1.,0.,0.));
#46824=DIRECTION('',(1.,0.,0.));
#46825=DIRECTION('',(0.,0.608761429008721,0.793353340291235));
#46826=DIRECTION('center_axis',(0.,-0.707106781186548,-0.707106781186547));
#46827=DIRECTION('ref_axis',(-0.707106781186569,0.499999999999985,-0.499999999999985));
#46828=DIRECTION('center_axis',(0.,0.70710678118654,0.707106781186555));
#46829=DIRECTION('ref_axis',(0.,0.707106781186555,-0.70710678118654));
#46830=DIRECTION('',(0.,0.707106781186548,0.707106781186547));
#46831=DIRECTION('center_axis',(0.,1.,0.));
#46832=DIRECTION('ref_axis',(0.,0.,-1.));
#46833=DIRECTION('',(0.,-0.707106781186548,-0.707106781186547));
#46834=DIRECTION('center_axis',(-0.706796314703392,0.500219436608432,0.500219436608421));
#46835=DIRECTION('ref_axis',(0.,0.70710678118654,-0.707106781186555));
#46836=DIRECTION('center_axis',(0.706790970016731,-0.500223212527577,-0.500223212527566));
#46837=DIRECTION('ref_axis',(-0.707106781188556,-0.520675376310292,-0.478431972699668));
#46838=DIRECTION('center_axis',(0.,0.,1.));
#46839=DIRECTION('ref_axis',(-0.89245173180272,0.451142889118653,0.));
#46840=DIRECTION('center_axis',(0.,0.676604984466694,-0.736346178773833));
#46841=DIRECTION('ref_axis',(0.,-0.736346178773833,-0.676604984466694));
#46842=DIRECTION('center_axis',(1.,0.,0.));
#46843=DIRECTION('ref_axis',(0.,-0.0209470044129978,-0.999780587432124));
#46844=DIRECTION('',(-1.,0.,0.));
#46845=DIRECTION('center_axis',(1.,0.,0.));
#46846=DIRECTION('ref_axis',(0.,-0.736103294766409,-0.676869218855487));
#46847=DIRECTION('',(1.,0.,0.));
#46848=DIRECTION('center_axis',(0.0943675359584503,-0.964005004559974,0.248574172714011));
#46849=DIRECTION('ref_axis',(-0.342144487584525,-0.265884093513182,-0.901245137813346));
#46850=DIRECTION('center_axis',(0.,0.676869218855492,-0.736103294766404));
#46851=DIRECTION('ref_axis',(0.,-0.736103294766404,-0.676869218855492));
#46852=DIRECTION('center_axis',(-1.,0.,0.));
#46853=DIRECTION('ref_axis',(0.,0.,1.));
#46854=DIRECTION('center_axis',(1.,0.,0.));
#46855=DIRECTION('ref_axis',(0.,-0.0654031292301429,0.997858923238603));
#46856=DIRECTION('',(0.,-1.,6.12323399573677E-17));
#46857=DIRECTION('',(0.,-6.12323399573677E-17,-1.));
#46858=DIRECTION('center_axis',(1.,0.,0.));
#46859=DIRECTION('ref_axis',(0.,0.0654031292301431,0.997858923238603));
#46860=DIRECTION('',(0.,0.130526192220052,0.99144486137381));
#46861=DIRECTION('',(0.,-0.99144486137381,0.130526192220052));
#46862=DIRECTION('',(0.,-0.130526192220052,-0.99144486137381));
#46863=DIRECTION('center_axis',(1.,0.,0.));
#46864=DIRECTION('ref_axis',(0.,0.195090322016129,0.98078528040323));
#46865=DIRECTION('',(0.,0.258819045102521,0.965925826289068));
#46866=DIRECTION('',(0.,-0.965925826289068,0.258819045102521));
#46867=DIRECTION('',(0.,0.258819045102521,0.965925826289068));
#46868=DIRECTION('center_axis',(1.,0.,0.));
#46869=DIRECTION('ref_axis',(0.,0.321439465303162,0.946930129495106));
#46870=DIRECTION('',(0.,-0.38268343236509,-0.923879532511287));
#46871=DIRECTION('',(0.,-0.923879532511287,0.38268343236509));
#46872=DIRECTION('',(0.,-0.38268343236509,-0.923879532511287));
#46873=DIRECTION('center_axis',(1.,0.,0.));
#46874=DIRECTION('ref_axis',(0.,0.442288690219001,0.896872741532688));
#46875=DIRECTION('',(0.,0.5,0.866025403784439));
#46876=DIRECTION('',(0.,-0.866025403784439,0.5));
#46877=DIRECTION('',(0.,-0.5,-0.866025403784439));
#46878=DIRECTION('center_axis',(1.,0.,0.));
#46879=DIRECTION('ref_axis',(0.,0.555570233019602,0.831469612302545));
#46880=DIRECTION('',(0.,0.608761429008721,0.793353340291235));
#46881=DIRECTION('',(0.,-0.793353340291235,0.608761429008721));
#46882=DIRECTION('',(0.,0.608761429008721,0.793353340291235));
#46883=DIRECTION('center_axis',(1.,0.,0.));
#46884=DIRECTION('ref_axis',(0.,0.659345815100069,0.751839807478978));
#46885=DIRECTION('',(0.,-0.707106781186548,-0.707106781186548));
#46886=DIRECTION('',(0.,-0.707106781186548,0.707106781186548));
#46887=DIRECTION('',(0.,-0.707106781186548,-0.707106781186548));
#46888=DIRECTION('center_axis',(1.,0.,0.));
#46889=DIRECTION('ref_axis',(0.,0.751839807478977,0.659345815100069));
#46890=DIRECTION('',(0.,0.793353340291235,0.608761429008721));
#46891=DIRECTION('',(0.,-0.608761429008721,0.793353340291235));
#46892=DIRECTION('',(0.,-0.793353340291235,-0.608761429008721));
#46893=DIRECTION('center_axis',(1.,0.,0.));
#46894=DIRECTION('ref_axis',(0.,0.831469612302545,0.555570233019602));
#46895=DIRECTION('',(0.,0.866025403784439,0.5));
#46896=DIRECTION('',(0.,-0.5,0.866025403784439));
#46897=DIRECTION('',(0.,0.866025403784439,0.5));
#46898=DIRECTION('center_axis',(1.,0.,0.));
#46899=DIRECTION('ref_axis',(0.,0.896872741532688,0.442288690219001));
#46900=DIRECTION('',(0.,-0.923879532511287,-0.38268343236509));
#46901=DIRECTION('',(0.,-0.38268343236509,0.923879532511287));
#46902=DIRECTION('',(0.,-0.923879532511287,-0.38268343236509));
#46903=DIRECTION('center_axis',(1.,0.,0.));
#46904=DIRECTION('ref_axis',(0.,0.946930129495106,0.321439465303162));
#46905=DIRECTION('',(0.,-0.965925826289068,-0.258819045102521));
#46906=DIRECTION('',(0.,-0.258819045102521,0.965925826289068));
#46907=DIRECTION('',(0.,-0.965925826289068,-0.258819045102521));
#46908=DIRECTION('center_axis',(1.,0.,0.));
#46909=DIRECTION('ref_axis',(0.,0.98078528040323,0.195090322016128));
#46910=DIRECTION('',(0.,-0.99144486137381,-0.130526192220052));
#46911=DIRECTION('',(0.,-0.130526192220052,0.99144486137381));
#46912=DIRECTION('',(0.,-0.99144486137381,-0.130526192220052));
#46913=DIRECTION('center_axis',(1.,0.,0.));
#46914=DIRECTION('ref_axis',(0.,0.997858923238603,0.0654031292301429));
#46915=DIRECTION('',(0.,-1.,0.));
#46916=DIRECTION('',(0.,0.,1.));
#46917=DIRECTION('',(0.,-1.,0.));
#46918=DIRECTION('center_axis',(1.,0.,0.));
#46919=DIRECTION('ref_axis',(0.,0.997858923238603,-0.0654031292301437));
#46920=DIRECTION('',(0.,0.99144486137381,-0.130526192220053));
#46921=DIRECTION('',(0.,0.130526192220053,0.99144486137381));
#46922=DIRECTION('',(0.,0.99144486137381,-0.130526192220053));
#46923=DIRECTION('center_axis',(1.,0.,0.));
#46924=DIRECTION('ref_axis',(0.,0.98078528040323,-0.19509032201613));
#46925=DIRECTION('',(0.,-0.965925826289068,0.258819045102522));
#46926=DIRECTION('',(0.,0.258819045102522,0.965925826289068));
#46927=DIRECTION('',(0.,0.965925826289068,-0.258819045102522));
#46928=DIRECTION('center_axis',(1.,0.,0.));
#46929=DIRECTION('ref_axis',(0.,0.946930129495105,-0.321439465303162));
#46930=DIRECTION('',(0.,-0.923879532511286,0.38268343236509));
#46931=DIRECTION('',(0.,0.38268343236509,0.923879532511286));
#46932=DIRECTION('',(0.,-0.923879532511286,0.38268343236509));
#46933=DIRECTION('center_axis',(1.,0.,0.));
#46934=DIRECTION('ref_axis',(0.,0.896872741532688,-0.442288690219002));
#46935=DIRECTION('',(0.,0.866025403784438,-0.5));
#46936=DIRECTION('',(0.,0.5,0.866025403784438));
#46937=DIRECTION('',(0.,-0.866025403784438,0.5));
#46938=DIRECTION('center_axis',(1.,0.,0.));
#46939=DIRECTION('ref_axis',(0.,0.831469612302545,-0.555570233019602));
#46940=DIRECTION('',(0.,0.793353340291235,-0.608761429008721));
#46941=DIRECTION('',(0.,0.608761429008721,0.793353340291235));
#46942=DIRECTION('',(0.,0.793353340291235,-0.608761429008721));
#46943=DIRECTION('center_axis',(1.,0.,0.));
#46944=DIRECTION('ref_axis',(0.,0.751839807478977,-0.65934581510007));
#46945=DIRECTION('',(0.,-0.707106781186547,0.707106781186548));
#46946=DIRECTION('',(0.,0.707106781186548,0.707106781186547));
#46947=DIRECTION('',(0.,0.60876142900872,-0.793353340291236));
#46948=DIRECTION('',(0.,0.793353340291236,0.60876142900872));
#46949=DIRECTION('',(0.,-0.60876142900872,0.793353340291236));
#46950=DIRECTION('center_axis',(1.,0.,0.));
#46951=DIRECTION('ref_axis',(0.,0.555570233019602,-0.831469612302546));
#46952=DIRECTION('',(0.,0.499999999999999,-0.866025403784439));
#46953=DIRECTION('',(0.,0.866025403784439,0.499999999999999));
#46954=DIRECTION('',(0.,0.499999999999999,-0.866025403784439));
#46955=DIRECTION('center_axis',(1.,0.,0.));
#46956=DIRECTION('ref_axis',(0.,0.442288690219,-0.896872741532689));
#46957=DIRECTION('',(0.,-0.382683432365089,0.923879532511287));
#46958=DIRECTION('',(0.,0.923879532511287,0.382683432365089));
#46959=DIRECTION('',(0.,-0.382683432365089,0.923879532511287));
#46960=DIRECTION('center_axis',(1.,0.,0.));
#46961=DIRECTION('ref_axis',(0.,0.321439465303161,-0.946930129495106));
#46962=DIRECTION('',(0.,0.25881904510252,-0.965925826289068));
#46963=DIRECTION('',(0.,0.965925826289068,0.25881904510252));
#46964=DIRECTION('',(0.,-0.25881904510252,0.965925826289068));
#46965=DIRECTION('center_axis',(1.,0.,0.));
#46966=DIRECTION('ref_axis',(0.,0.195090322016127,-0.980785280403231));
#46967=DIRECTION('',(0.,0.130526192220051,-0.991444861373811));
#46968=DIRECTION('',(0.,0.991444861373811,0.130526192220051));
#46969=DIRECTION('center_axis',(1.,0.,0.));
#46970=DIRECTION('ref_axis',(0.,0.0654031292301432,-0.997858923238603));
#46971=DIRECTION('',(0.,1.,-1.83697019872103E-16));
#46972=DIRECTION('',(0.,1.83697019872103E-16,1.));
#46973=DIRECTION('center_axis',(1.,0.,0.));
#46974=DIRECTION('ref_axis',(0.,-0.0654031292301437,-0.997858923238603));
#46975=DIRECTION('',(0.,-0.130526192220052,-0.99144486137381));
#46976=DIRECTION('',(0.,0.99144486137381,-0.130526192220052));
#46977=DIRECTION('',(0.,0.130526192220052,0.99144486137381));
#46978=DIRECTION('center_axis',(1.,0.,0.));
#46979=DIRECTION('ref_axis',(0.,-0.19509032201613,-0.98078528040323));
#46980=DIRECTION('',(0.,-0.258819045102522,-0.965925826289068));
#46981=DIRECTION('',(0.,0.965925826289068,-0.258819045102522));
#46982=DIRECTION('',(0.,-0.258819045102522,-0.965925826289068));
#46983=DIRECTION('center_axis',(1.,0.,0.));
#46984=DIRECTION('ref_axis',(0.,-0.321439465303162,-0.946930129495105));
#46985=DIRECTION('',(0.,0.38268343236509,0.923879532511286));
#46986=DIRECTION('',(0.,0.923879532511286,-0.38268343236509));
#46987=DIRECTION('',(0.,0.38268343236509,0.923879532511286));
#46988=DIRECTION('center_axis',(1.,0.,0.));
#46989=DIRECTION('ref_axis',(0.,-0.442288690219002,-0.896872741532688));
#46990=DIRECTION('',(0.,-0.5,-0.866025403784438));
#46991=DIRECTION('',(0.,0.866025403784438,-0.5));
#46992=DIRECTION('',(0.,-0.608761429008721,-0.793353340291235));
#46993=DIRECTION('',(0.,0.793353340291235,-0.608761429008721));
#46994=DIRECTION('',(0.,-0.608761429008721,-0.793353340291235));
#46995=DIRECTION('center_axis',(1.,0.,0.));
#46996=DIRECTION('ref_axis',(0.,-0.659345815100069,-0.751839807478977));
#46997=DIRECTION('',(0.,0.707106781186548,0.707106781186547));
#46998=DIRECTION('',(0.,0.707106781186547,-0.707106781186548));
#46999=DIRECTION('center_axis',(1.,0.,0.));
#47000=DIRECTION('ref_axis',(0.,-0.751839807478978,-0.659345815100068));
#47001=DIRECTION('',(0.,-0.793353340291235,-0.60876142900872));
#47002=DIRECTION('',(0.,0.60876142900872,-0.793353340291235));
#47003=DIRECTION('',(0.,0.793353340291235,0.60876142900872));
#47004=DIRECTION('center_axis',(1.,0.,0.));
#47005=DIRECTION('ref_axis',(0.,-0.831469612302545,-0.555570233019602));
#47006=DIRECTION('',(0.,-0.866025403784439,-0.5));
#47007=DIRECTION('',(0.,0.5,-0.866025403784439));
#47008=DIRECTION('',(0.,-0.866025403784439,-0.5));
#47009=DIRECTION('center_axis',(1.,0.,0.));
#47010=DIRECTION('ref_axis',(0.,-0.896872741532689,-0.442288690219));
#47011=DIRECTION('',(0.,0.923879532511287,0.382683432365089));
#47012=DIRECTION('',(0.,0.382683432365089,-0.923879532511287));
#47013=DIRECTION('',(0.,0.923879532511287,0.382683432365089));
#47014=DIRECTION('center_axis',(1.,0.,0.));
#47015=DIRECTION('ref_axis',(0.,-0.946930129495106,-0.321439465303161));
#47016=DIRECTION('',(0.,-0.965925826289068,-0.25881904510252));
#47017=DIRECTION('',(0.,0.25881904510252,-0.965925826289068));
#47018=DIRECTION('',(0.,0.965925826289068,0.25881904510252));
#47019=DIRECTION('center_axis',(1.,0.,0.));
#47020=DIRECTION('ref_axis',(0.,-0.980785280403231,-0.195090322016127));
#47021=DIRECTION('',(0.,-0.991444861373811,-0.130526192220051));
#47022=DIRECTION('',(0.,0.130526192220051,-0.991444861373811));
#47023=DIRECTION('center_axis',(1.,0.,0.));
#47024=DIRECTION('ref_axis',(0.,-0.997858923238603,-0.0654031292301433));
#47025=DIRECTION('',(0.,-1.22464679914735E-16,-1.));
#47026=DIRECTION('',(0.,1.,-1.22464679914735E-16));
#47027=DIRECTION('center_axis',(1.,0.,0.));
#47028=DIRECTION('ref_axis',(0.,-0.997858923238603,0.0654031292301436));
#47029=DIRECTION('',(0.,-0.99144486137381,0.130526192220052));
#47030=DIRECTION('',(0.,-0.130526192220052,-0.99144486137381));
#47031=DIRECTION('',(0.,0.99144486137381,-0.130526192220052));
#47032=DIRECTION('center_axis',(1.,0.,0.));
#47033=DIRECTION('ref_axis',(0.,-0.98078528040323,0.19509032201613));
#47034=DIRECTION('',(0.,-0.965925826289068,0.258819045102521));
#47035=DIRECTION('',(0.,-0.258819045102521,-0.965925826289068));
#47036=DIRECTION('',(0.,-0.965925826289068,0.258819045102521));
#47037=DIRECTION('center_axis',(1.,0.,0.));
#47038=DIRECTION('ref_axis',(0.,-0.946930129495105,0.321439465303162));
#47039=DIRECTION('',(0.,0.923879532511287,-0.38268343236509));
#47040=DIRECTION('',(0.,-0.38268343236509,-0.923879532511287));
#47041=DIRECTION('',(0.,0.923879532511287,-0.38268343236509));
#47042=DIRECTION('center_axis',(1.,0.,0.));
#47043=DIRECTION('ref_axis',(0.,-0.896872741532688,0.442288690219002));
#47044=DIRECTION('',(0.,-0.866025403784438,0.5));
#47045=DIRECTION('',(0.,-0.5,-0.866025403784438));
#47046=DIRECTION('',(0.,0.866025403784438,-0.5));
#47047=DIRECTION('center_axis',(1.,0.,0.));
#47048=DIRECTION('ref_axis',(0.,-0.831469612302545,0.555570233019602));
#47049=DIRECTION('',(0.,-0.793353340291235,0.608761429008721));
#47050=DIRECTION('',(0.,-0.608761429008721,-0.793353340291235));
#47051=DIRECTION('',(0.,-0.793353340291235,0.608761429008721));
#47052=DIRECTION('center_axis',(1.,0.,0.));
#47053=DIRECTION('ref_axis',(0.,-0.751839807478977,0.659345815100069));
#47054=DIRECTION('',(0.,0.707106781186547,-0.707106781186548));
#47055=DIRECTION('',(0.,-0.707106781186548,-0.707106781186547));
#47056=DIRECTION('',(0.,0.707106781186547,-0.707106781186548));
#47057=DIRECTION('center_axis',(1.,0.,0.));
#47058=DIRECTION('ref_axis',(0.,-0.659345815100069,0.751839807478978));
#47059=DIRECTION('',(0.,-0.60876142900872,0.793353340291235));
#47060=DIRECTION('',(0.,-0.793353340291235,-0.60876142900872));
#47061=DIRECTION('',(0.,0.60876142900872,-0.793353340291235));
#47062=DIRECTION('center_axis',(1.,0.,0.));
#47063=DIRECTION('ref_axis',(0.,-0.555570233019602,0.831469612302545));
#47064=DIRECTION('',(0.,-0.5,0.866025403784439));
#47065=DIRECTION('',(0.,-0.866025403784439,-0.5));
#47066=DIRECTION('',(0.,-0.5,0.866025403784439));
#47067=DIRECTION('center_axis',(1.,0.,0.));
#47068=DIRECTION('ref_axis',(0.,-0.442288690219001,0.896872741532688));
#47069=DIRECTION('',(0.,0.38268343236509,-0.923879532511287));
#47070=DIRECTION('',(0.,-0.923879532511287,-0.38268343236509));
#47071=DIRECTION('',(0.,0.38268343236509,-0.923879532511287));
#47072=DIRECTION('center_axis',(1.,0.,0.));
#47073=DIRECTION('ref_axis',(0.,-0.321439465303161,0.946930129495106));
#47074=DIRECTION('',(0.,-0.258819045102521,0.965925826289068));
#47075=DIRECTION('',(0.,-0.965925826289068,-0.258819045102521));
#47076=DIRECTION('',(0.,0.258819045102521,-0.965925826289068));
#47077=DIRECTION('center_axis',(1.,0.,0.));
#47078=DIRECTION('ref_axis',(0.,-0.195090322016128,0.98078528040323));
#47079=DIRECTION('',(0.,-0.130526192220051,0.991444861373811));
#47080=DIRECTION('',(0.,-0.991444861373811,-0.130526192220051));
#47081=DIRECTION('center_axis',(-1.,0.,0.));
#47082=DIRECTION('ref_axis',(0.,-1.,1.83697019872103E-16));
#47083=DIRECTION('center_axis',(1.,0.,0.));
#47084=DIRECTION('ref_axis',(0.,0.,-1.));
#47085=DIRECTION('center_axis',(-1.,0.,0.));
#47086=DIRECTION('ref_axis',(0.,-0.751839807478978,-0.659345815100068));
#47087=DIRECTION('center_axis',(0.,-0.641731962878012,0.766928997900545));
#47088=DIRECTION('ref_axis',(0.,-0.766928997900544,-0.641731962878012));
#47089=DIRECTION('center_axis',(1.,0.,0.));
#47090=DIRECTION('ref_axis',(0.,1.,0.));
#47091=DIRECTION('center_axis',(1.,-3.06322230481445E-16,3.46444446476948E-16));
#47092=DIRECTION('ref_axis',(0.,-0.749155210567656,-0.662394497621569));
#47093=DIRECTION('center_axis',(1.,0.,0.));
#47094=DIRECTION('ref_axis',(0.,0.,-1.));
#47095=DIRECTION('center_axis',(-1.,0.,0.));
#47096=DIRECTION('ref_axis',(0.,-0.749155210567656,-0.662394497621569));
#47097=DIRECTION('center_axis',(-2.68326347919584E-14,0.641456667268316,
-0.767159269002875));
#47098=DIRECTION('ref_axis',(0.,-0.767159269002875,-0.641456667268316));
#47099=DIRECTION('center_axis',(1.,0.,0.));
#47100=DIRECTION('ref_axis',(0.,1.,0.));
#47101=DIRECTION('center_axis',(1.,0.,0.));
#47102=DIRECTION('ref_axis',(0.,0.,-1.));
#47103=DIRECTION('',(1.,0.,0.));
#47104=DIRECTION('center_axis',(0.,-0.99144486137381,0.130526192220052));
#47105=DIRECTION('ref_axis',(-0.707106781186562,-0.0922959556412558,-0.701057384649964));
#47106=DIRECTION('center_axis',(1.46763321699136E-14,0.99144486137381,-0.130526192220056));
#47107=DIRECTION('ref_axis',(0.,-0.130526192220056,-0.99144486137381));
#47108=DIRECTION('center_axis',(0.,0.608761429008725,-0.793353340291232));
#47109=DIRECTION('ref_axis',(1.63551297779561E-16,-0.793353340291232,-0.608761429008725));
#47110=DIRECTION('',(0.,-0.99144486137381,0.130526192220052));
#47111=DIRECTION('center_axis',(-0.706796314701277,0.701365059961673,-0.0923364618644909));
#47112=DIRECTION('ref_axis',(0.,-0.130526192220056,-0.99144486137381));
#47113=DIRECTION('center_axis',(0.70679097001458,-0.70137035423371,0.0923371588686275));
#47114=DIRECTION('ref_axis',(-0.707106781190706,-0.696532689773595,0.12182861761868));
#47115=DIRECTION('center_axis',(0.,0.,1.));
#47116=DIRECTION('ref_axis',(1.,0.,0.));
#47117=DIRECTION('center_axis',(0.,-0.17229168332254,-0.98504597651982));
#47118=DIRECTION('ref_axis',(0.,-0.98504597651982,0.17229168332254));
#47119=DIRECTION('center_axis',(1.,0.,0.));
#47120=DIRECTION('ref_axis',(0.,-0.805930996937504,-0.592009483180228));
#47121=DIRECTION('',(-1.,0.,0.));
#47122=DIRECTION('center_axis',(1.,0.,0.));
#47123=DIRECTION('ref_axis',(0.,-0.985107749339346,0.171938134779833));
#47124=DIRECTION('',(1.,0.,0.));
#47125=DIRECTION('center_axis',(0.,0.,1.));
#47126=DIRECTION('ref_axis',(1.,0.,0.));
#47127=DIRECTION('center_axis',(0.,-0.171938134779822,-0.985107749339348));
#47128=DIRECTION('ref_axis',(0.,-0.985107749339348,0.171938134779822));
#47129=DIRECTION('center_axis',(1.,0.,0.));
#47130=DIRECTION('ref_axis',(0.,0.,-1.));
#47131=DIRECTION('center_axis',(-1.,0.,0.));
#47132=DIRECTION('ref_axis',(0.,-0.98078528040323,0.19509032201613));
#47133=DIRECTION('center_axis',(0.,0.217784015488416,0.975996989031084));
#47134=DIRECTION('ref_axis',(0.,-0.975996989031084,0.217784015488416));
#47135=DIRECTION('center_axis',(1.,0.,0.));
#47136=DIRECTION('ref_axis',(0.,1.,0.));
#47137=DIRECTION('center_axis',(1.,0.,0.));
#47138=DIRECTION('ref_axis',(0.,-0.981569683813102,0.191104567760813));
#47139=DIRECTION('center_axis',(1.,0.,0.));
#47140=DIRECTION('ref_axis',(0.,0.,-1.));
#47141=DIRECTION('center_axis',(-1.,0.,0.));
#47142=DIRECTION('ref_axis',(0.,-0.981569683813102,0.191104567760813));
#47143=DIRECTION('center_axis',(8.98680308111627E-15,-0.218134291185374,
-0.975918762504879));
#47144=DIRECTION('ref_axis',(0.,-0.975918762504879,0.218134291185374));
#47145=DIRECTION('center_axis',(1.,0.,0.));
#47146=DIRECTION('ref_axis',(0.,1.,0.));
#47147=DIRECTION('center_axis',(1.,0.,0.));
#47148=DIRECTION('ref_axis',(0.,0.,-1.));
#47149=DIRECTION('',(1.,0.,0.));
#47150=DIRECTION('center_axis',(0.,0.707106781186548,0.707106781186548));
#47151=DIRECTION('ref_axis',(-0.707106781186556,-0.499999999999994,0.499999999999994));
#47152=DIRECTION('center_axis',(0.,-0.707106781186548,-0.707106781186548));
#47153=DIRECTION('ref_axis',(0.,-0.707106781186547,0.707106781186547));
#47154=DIRECTION('center_axis',(0.,-1.,0.));
#47155=DIRECTION('ref_axis',(-4.088782444489E-17,2.89120579329464E-17,1.));
#47156=DIRECTION('',(0.,0.707106781186548,0.707106781186548));
#47157=DIRECTION('center_axis',(-0.706796314703281,-0.500219436608505,-0.500219436608505));
#47158=DIRECTION('ref_axis',(0.,-0.707106781186547,0.707106781186547));
#47159=DIRECTION('center_axis',(0.706790970016705,0.50022321252759,0.50022321252759));
#47160=DIRECTION('ref_axis',(-0.707106781188582,0.520675376310282,0.478431972699641));
#47161=DIRECTION('center_axis',(0.,0.,1.));
#47162=DIRECTION('ref_axis',(-0.892451731802692,-0.45114288911871,0.));
#47163=DIRECTION('center_axis',(0.,-0.676604984466694,0.736346178773833));
#47164=DIRECTION('ref_axis',(0.,0.736346178773833,0.676604984466694));
#47165=DIRECTION('center_axis',(1.,0.,0.));
#47166=DIRECTION('ref_axis',(0.,0.0209470044129978,0.999780587432124));
#47167=DIRECTION('',(-1.,0.,0.));
#47168=DIRECTION('center_axis',(1.,0.,0.));
#47169=DIRECTION('ref_axis',(0.,0.736103294766409,0.676869218855487));
#47170=DIRECTION('',(1.,0.,0.));
#47171=DIRECTION('center_axis',(-0.0943675359584499,-0.964005004559959,
0.24857417271407));
#47172=DIRECTION('ref_axis',(-0.342144487584426,0.265884093513226,0.90124513781337));
#47173=DIRECTION('center_axis',(0.,-0.676869218855492,0.736103294766404));
#47174=DIRECTION('ref_axis',(0.,0.736103294766404,0.676869218855492));
#47175=DIRECTION('center_axis',(1.,0.,0.));
#47176=DIRECTION('ref_axis',(0.,0.,-1.));
#47177=DIRECTION('center_axis',(-1.,0.,0.));
#47178=DIRECTION('ref_axis',(0.,0.751839807478977,0.659345815100069));
#47179=DIRECTION('center_axis',(0.,0.641731962878012,-0.766928997900544));
#47180=DIRECTION('ref_axis',(0.,0.766928997900544,0.641731962878013));
#47181=DIRECTION('center_axis',(1.,0.,0.));
#47182=DIRECTION('ref_axis',(0.,1.,0.));
#47183=DIRECTION('center_axis',(1.,0.,0.));
#47184=DIRECTION('ref_axis',(0.,0.749155210567656,0.66239449762157));
#47185=DIRECTION('center_axis',(1.,0.,0.));
#47186=DIRECTION('ref_axis',(0.,0.,-1.));
#47187=DIRECTION('center_axis',(-1.,0.,0.));
#47188=DIRECTION('ref_axis',(0.,0.749155210567656,0.662394497621569));
#47189=DIRECTION('center_axis',(-2.21475715743149E-15,-0.641456667268332,
0.767159269002861));
#47190=DIRECTION('ref_axis',(0.,0.767159269002861,0.641456667268332));
#47191=DIRECTION('center_axis',(1.,0.,0.));
#47192=DIRECTION('ref_axis',(0.,1.,0.));
#47193=DIRECTION('center_axis',(1.,0.,0.));
#47194=DIRECTION('ref_axis',(0.,0.,-1.));
#47195=DIRECTION('',(1.,0.,0.));
#47196=DIRECTION('center_axis',(0.,0.923879532511287,0.38268343236509));
#47197=DIRECTION('ref_axis',(-0.707106781186561,-0.270598050073091,0.653281482438177));
#47198=DIRECTION('center_axis',(0.,-0.923879532511289,-0.382683432365084));
#47199=DIRECTION('ref_axis',(0.,-0.382683432365084,0.923879532511289));
#47200=DIRECTION('center_axis',(0.,-0.923879532511286,0.382683432365091));
#47201=DIRECTION('ref_axis',(8.17756488897798E-17,0.382683432365091,0.923879532511286));
#47202=DIRECTION('',(0.,0.923879532511287,0.38268343236509));
#47203=DIRECTION('center_axis',(0.,0.965925826289068,0.258819045102521));
#47204=DIRECTION('ref_axis',(0.707106781186559,0.183012701892221,-0.683012701892207));
#47205=DIRECTION('center_axis',(0.,-0.965925826289067,-0.258819045102527));
#47206=DIRECTION('ref_axis',(0.,0.258819045102527,-0.965925826289067));
#47207=DIRECTION('center_axis',(0.,-0.499999999999998,-0.86602540378444));
#47208=DIRECTION('ref_axis',(0.,0.86602540378444,-0.499999999999999));
#47209=DIRECTION('',(0.,0.965925826289068,0.258819045102521));
#47210=DIRECTION('center_axis',(0.706796314702098,-0.683312457875098,-0.183093021265763));
#47211=DIRECTION('ref_axis',(0.,0.258819045102527,-0.965925826289067));
#47212=DIRECTION('center_axis',(-0.706790970015359,0.683317615876648,0.183094403348113));
#47213=DIRECTION('ref_axis',(0.707106781189927,0.674671930494452,0.211702116659494));
#47214=DIRECTION('center_axis',(0.,0.,1.));
#47215=DIRECTION('ref_axis',(1.,0.,0.));
#47216=DIRECTION('center_axis',(0.,0.29939200456439,-0.954130194262249));
#47217=DIRECTION('ref_axis',(0.,0.954130194262249,0.29939200456439));
#47218=DIRECTION('center_axis',(1.,0.,0.));
#47219=DIRECTION('ref_axis',(0.,0.,-1.));
#47220=DIRECTION('center_axis',(1.,0.,0.));
#47221=DIRECTION('ref_axis',(0.,0.948228067551138,0.317590194918285));
#47222=DIRECTION('center_axis',(3.15602894933998E-14,0.343651082071033,
-0.9390974037827));
#47223=DIRECTION('ref_axis',(-0.707106781186566,0.664042142409419,0.242998010494495));
#47224=DIRECTION('center_axis',(-1.,0.,0.));
#47225=DIRECTION('ref_axis',(0.,0.948228067551138,0.317590194918285));
#47226=DIRECTION('center_axis',(-1.,0.,0.));
#47227=DIRECTION('ref_axis',(0.,0.87630888913324,-0.481749655761234));
#47228=DIRECTION('',(1.,0.,0.));
#47229=DIRECTION('center_axis',(-1.,0.,0.));
#47230=DIRECTION('ref_axis',(0.,0.954237585951785,0.299049543649391));
#47231=DIRECTION('',(-1.,0.,0.));
#47232=DIRECTION('center_axis',(0.,0.,1.));
#47233=DIRECTION('ref_axis',(1.,0.,0.));
#47234=DIRECTION('center_axis',(0.,0.299049543649383,-0.954237585951788));
#47235=DIRECTION('ref_axis',(0.,0.954237585951788,0.299049543649383));
#47236=DIRECTION('center_axis',(-0.70679631470526,-0.653568190182148,-0.270716808309152));
#47237=DIRECTION('ref_axis',(-5.92118946466751E-14,-0.382683432365117,0.923879532511276));
#47238=DIRECTION('center_axis',(0.706790970015977,0.653573123660707,0.27071885182281));
#47239=DIRECTION('ref_axis',(-0.70710678118931,0.66412931272089,0.242759667121561));
#47240=DIRECTION('center_axis',(-0.250366849761766,-0.8070109637463,0.534836185138624));
#47241=DIRECTION('ref_axis',(-0.342144487592339,0.590536454753872,0.73089249908376));
#47242=DIRECTION('center_axis',(-1.,0.,0.));
#47243=DIRECTION('ref_axis',(0.,0.401951975455082,0.915660750184127));
#47244=DIRECTION('center_axis',(0.,0.,1.));
#47245=DIRECTION('ref_axis',(-0.917771314419815,-0.397109323018392,0.));
#47246=DIRECTION('center_axis',(0.,-0.343314013641811,0.939220681223082));
#47247=DIRECTION('ref_axis',(0.,0.939220681223082,0.343314013641811));
#47248=DIRECTION('center_axis',(1.,0.,0.));
#47249=DIRECTION('ref_axis',(0.,1.,0.));
#47250=DIRECTION('',(-1.,0.,0.));
#47251=DIRECTION('center_axis',(1.,0.,0.));
#47252=DIRECTION('ref_axis',(0.,0.948228067551138,0.317590194918285));
#47253=DIRECTION('center_axis',(1.,0.,0.));
#47254=DIRECTION('ref_axis',(0.,0.401951975455086,0.915660750184125));
#47255=DIRECTION('',(1.,0.,0.));
#47256=DIRECTION('center_axis',(1.,0.,0.));
#47257=DIRECTION('ref_axis',(0.,0.401951975455082,0.915660750184127));
#47258=DIRECTION('center_axis',(0.,0.38268343236509,-0.923879532511287));
#47259=DIRECTION('ref_axis',(-1.,0.,0.));
#47260=DIRECTION('',(-1.,0.,0.));
#47261=DIRECTION('center_axis',(0.,0.38268343236509,-0.923879532511287));
#47262=DIRECTION('ref_axis',(0.707106781186518,0.653281482438215,0.270598050073112));
#47263=DIRECTION('center_axis',(1.,0.,0.));
#47264=DIRECTION('ref_axis',(0.,0.,-1.));
#47265=DIRECTION('center_axis',(-1.,0.,0.));
#47266=DIRECTION('ref_axis',(0.,0.946930129495106,0.321439465303161));
#47267=DIRECTION('center_axis',(1.,0.,0.));
#47268=DIRECTION('ref_axis',(0.,1.,0.));
#47269=DIRECTION('',(-0.706902428155817,-0.683210034733321,-0.18306557706763));
#47270=DIRECTION('center_axis',(0.,0.5,0.866025403784439));
#47271=DIRECTION('ref_axis',(-0.707106781186556,-0.612372435695782,0.353553390593278));
#47272=DIRECTION('center_axis',(0.,-0.500000000000001,-0.866025403784438));
#47273=DIRECTION('ref_axis',(0.,-0.866025403784438,0.500000000000001));
#47274=DIRECTION('center_axis',(0.,-0.96592582628907,-0.258819045102514));
#47275=DIRECTION('ref_axis',(1.22663473334669E-16,-0.258819045102514,0.96592582628907));
#47276=DIRECTION('',(0.,0.5,0.866025403784439));
#47277=DIRECTION('center_axis',(-0.706796314703024,-0.353708555707317,-0.612641189556878));
#47278=DIRECTION('ref_axis',(0.,-0.866025403784438,0.500000000000001));
#47279=DIRECTION('center_axis',(0.706790970016425,0.35371122568532,0.612645814094433));
#47280=DIRECTION('ref_axis',(-0.707106781188862,0.379106486770073,0.596890502257808));
#47281=DIRECTION('center_axis',(0.,0.,1.));
#47282=DIRECTION('ref_axis',(-0.858053385943042,-0.51356049971905,0.));
#47283=DIRECTION('center_axis',(0.,-0.844130643547427,0.536137535175637));
#47284=DIRECTION('ref_axis',(0.,0.536137535175637,0.844130643547427));
#47285=DIRECTION('center_axis',(1.,0.,0.));
#47286=DIRECTION('ref_axis',(0.,-0.238529004405328,0.971135373703071));
#47287=DIRECTION('',(-1.,0.,0.));
#47288=DIRECTION('center_axis',(1.,0.,0.));
#47289=DIRECTION('ref_axis',(0.,0.535834538347858,0.8443230113609));
#47290=DIRECTION('',(1.,0.,0.));
#47291=DIRECTION('center_axis',(-0.00806484247964557,-0.999722309028741,
0.0221418866861002));
#47292=DIRECTION('ref_axis',(-0.34214448758315,0.0235649067522203,0.93935182162288));
#47293=DIRECTION('center_axis',(0.,-0.844323011360888,0.535834538347876));
#47294=DIRECTION('ref_axis',(0.,0.535834538347876,0.844323011360888));
#47295=DIRECTION('center_axis',(1.,0.,0.));
#47296=DIRECTION('ref_axis',(0.,0.,-1.));
#47297=DIRECTION('center_axis',(-1.,0.,0.));
#47298=DIRECTION('ref_axis',(0.,0.555570233019602,0.831469612302545));
#47299=DIRECTION('center_axis',(0.,0.818361307397102,-0.574704072158277));
#47300=DIRECTION('ref_axis',(0.,0.574704072158277,0.818361307397102));
#47301=DIRECTION('center_axis',(1.,0.,0.));
#47302=DIRECTION('ref_axis',(0.,1.,0.));
#47303=DIRECTION('center_axis',(1.,3.85550974406735E-16,-2.55357611039623E-16));
#47304=DIRECTION('ref_axis',(0.,0.552188054430745,0.833719588677145));
#47305=DIRECTION('center_axis',(1.,0.,0.));
#47306=DIRECTION('ref_axis',(0.,0.,-1.));
#47307=DIRECTION('center_axis',(-1.,0.,0.));
#47308=DIRECTION('ref_axis',(0.,0.552188054430745,0.833719588677145));
#47309=DIRECTION('center_axis',(1.41403726205245E-14,-0.818154990804665,
0.57499774870987));
#47310=DIRECTION('ref_axis',(0.,0.57499774870987,0.818154990804665));
#47311=DIRECTION('center_axis',(1.,0.,0.));
#47312=DIRECTION('ref_axis',(0.,1.,0.));
#47313=DIRECTION('center_axis',(1.,0.,0.));
#47314=DIRECTION('ref_axis',(0.,0.,-1.));
#47315=DIRECTION('',(1.,0.,0.));
#47316=DIRECTION('center_axis',(0.,0.793353340291235,0.608761429008721));
#47317=DIRECTION('ref_axis',(-0.707106781186566,-0.430459334576874,0.560985526796912));
#47318=DIRECTION('center_axis',(2.7325092008722E-15,-0.793353340291235,
-0.608761429008721));
#47319=DIRECTION('ref_axis',(0.,-0.608761429008721,0.793353340291235));
#47320=DIRECTION('center_axis',(0.,-0.991444861373811,0.130526192220051));
#47321=DIRECTION('ref_axis',(-4.088782444489E-17,0.130526192220051,0.99144486137381));
#47322=DIRECTION('',(0.,0.793353340291235,0.608761429008721));
#47323=DIRECTION('center_axis',(-0.706796314703331,-0.561231728319733,-0.430648251649807));
#47324=DIRECTION('ref_axis',(0.,-0.608761429008721,0.793353340291235));
#47325=DIRECTION('center_axis',(0.70679097001662,0.561235964791754,0.430651502409123));
#47326=DIRECTION('ref_axis',(-0.707106781188666,0.578668829919453,0.406377146597412));
#47327=DIRECTION('center_axis',(0.,0.,1.));
#47328=DIRECTION('ref_axis',(-0.903692699960971,-0.428181625057932,0.));
#47329=DIRECTION('center_axis',(0.,-0.574704072158277,0.818361307397102));
#47330=DIRECTION('ref_axis',(0.,0.818361307397102,0.574704072158277));
#47331=DIRECTION('center_axis',(1.,0.,0.));
#47332=DIRECTION('ref_axis',(0.,0.151265353019462,0.988493193186426));
#47333=DIRECTION('',(-1.,0.,0.));
#47334=DIRECTION('center_axis',(1.,0.,0.));
#47335=DIRECTION('ref_axis',(0.,0.818154990804646,0.574997748709897));
#47336=DIRECTION('',(1.,0.,0.));
#47337=DIRECTION('center_axis',(-0.14109761386294,-0.924473827538098,0.354174541094139));
#47338=DIRECTION('ref_axis',(-0.342144487584241,0.381245514330408,0.858830022425078));
#47339=DIRECTION('center_axis',(0.,-0.57499774870989,0.818154990804651));
#47340=DIRECTION('ref_axis',(0.,0.818154990804651,0.57499774870989));
#47341=DIRECTION('center_axis',(1.,0.,0.));
#47342=DIRECTION('ref_axis',(0.,0.,-1.));
#47343=DIRECTION('center_axis',(-1.,0.,0.));
#47344=DIRECTION('ref_axis',(0.,0.831469612302545,0.555570233019602));
#47345=DIRECTION('center_axis',(0.,0.536137535175637,-0.844130643547427));
#47346=DIRECTION('ref_axis',(0.,0.844130643547427,0.536137535175637));
#47347=DIRECTION('center_axis',(1.,0.,0.));
#47348=DIRECTION('ref_axis',(0.,1.,0.));
#47349=DIRECTION('center_axis',(1.,0.,0.));
#47350=DIRECTION('ref_axis',(0.,0.829205915410775,0.558943243851984));
#47351=DIRECTION('center_axis',(1.,0.,0.));
#47352=DIRECTION('ref_axis',(0.,0.,-1.));
#47353=DIRECTION('center_axis',(-1.,0.,0.));
#47354=DIRECTION('ref_axis',(0.,0.829205915410775,0.558943243851984));
#47355=DIRECTION('center_axis',(-4.05470925745193E-14,-0.535834538347868,
0.844323011360893));
#47356=DIRECTION('ref_axis',(0.,0.844323011360893,0.535834538347868));
#47357=DIRECTION('center_axis',(1.,0.,0.));
#47358=DIRECTION('ref_axis',(0.,1.,0.));
#47359=DIRECTION('center_axis',(1.,0.,0.));
#47360=DIRECTION('ref_axis',(0.,0.,-1.));
#47361=DIRECTION('',(1.,0.,0.));
#47362=DIRECTION('center_axis',(0.,0.923879532511287,0.38268343236509));
#47363=DIRECTION('ref_axis',(0.707106781186566,0.270598050073093,-0.653281482438171));
#47364=DIRECTION('center_axis',(-2.8324263850286E-15,-0.923879532511287,
-0.382683432365089));
#47365=DIRECTION('ref_axis',(0.,0.382683432365089,-0.923879532511287));
#47366=DIRECTION('center_axis',(0.,-0.382683432365094,-0.923879532511285));
#47367=DIRECTION('ref_axis',(1.63551297779561E-16,0.923879532511285,-0.382683432365094));
#47368=DIRECTION('',(0.,0.923879532511287,0.38268343236509));
#47369=DIRECTION('center_axis',(0.706796314702682,-0.653568190184553,-0.270716808310078));
#47370=DIRECTION('ref_axis',(0.,0.382683432365087,-0.923879532511288));
#47371=DIRECTION('center_axis',(-0.706790970015921,0.653573123660759,0.270718851822832));
#47372=DIRECTION('ref_axis',(0.707106781189366,0.641267347429893,0.297953333789442));
#47373=DIRECTION('center_axis',(0.,0.,1.));
#47374=DIRECTION('ref_axis',(1.,0.,0.));
#47375=DIRECTION('center_axis',(0.,0.421369645600998,-0.906888979845984));
#47376=DIRECTION('ref_axis',(0.,0.906888979845984,0.421369645600998));
#47377=DIRECTION('center_axis',(-1.,0.,0.));
#47378=DIRECTION('ref_axis',(0.,0.931692893277179,-0.363246958165926));
#47379=DIRECTION('',(1.,0.,0.));
#47380=DIRECTION('center_axis',(-1.,0.,0.));
#47381=DIRECTION('ref_axis',(0.,0.90704015290395,0.421044131914909));
#47382=DIRECTION('',(-1.,0.,0.));
#47383=DIRECTION('center_axis',(0.,0.,1.));
#47384=DIRECTION('ref_axis',(1.,0.,0.));
#47385=DIRECTION('center_axis',(0.,0.421044131914905,-0.907040152903952));
#47386=DIRECTION('ref_axis',(0.,0.907040152903951,0.421044131914905));
#47387=DIRECTION('center_axis',(1.,0.,0.));
#47388=DIRECTION('ref_axis',(0.,0.,-1.));
#47389=DIRECTION('center_axis',(1.,0.,0.));
#47390=DIRECTION('ref_axis',(0.,0.896872741532688,0.442288690219001));
#47391=DIRECTION('center_axis',(0.,-0.462969813837163,0.886374047158186));
#47392=DIRECTION('ref_axis',(0.,0.886374047158186,0.462969813837163));
#47393=DIRECTION('center_axis',(-1.,0.,0.));
#47394=DIRECTION('ref_axis',(0.,1.,0.));
#47395=DIRECTION('center_axis',(-1.,0.,0.));
#47396=DIRECTION('ref_axis',(0.,0.898662006154886,0.438641765788069));
#47397=DIRECTION('center_axis',(0.,0.965925826289068,0.258819045102521));
#47398=DIRECTION('ref_axis',(-0.707106781186559,-0.183012701892221,0.683012701892207));
#47399=DIRECTION('center_axis',(-1.91564575389552E-15,-0.965925826289067,
-0.258819045102527));
#47400=DIRECTION('ref_axis',(0.,-0.258819045102527,0.965925826289067));
#47401=DIRECTION('center_axis',(0.,-0.866025403784436,0.500000000000005));
#47402=DIRECTION('ref_axis',(0.,0.500000000000005,0.866025403784436));
#47403=DIRECTION('',(0.,0.965925826289068,0.258819045102521));
#47404=DIRECTION('center_axis',(0.,0.99144486137381,0.130526192220052));
#47405=DIRECTION('ref_axis',(0.70710678118656,0.092295955641248,-0.701057384649966));
#47406=DIRECTION('center_axis',(0.,-0.99144486137381,-0.130526192220056));
#47407=DIRECTION('ref_axis',(0.,0.130526192220056,-0.99144486137381));
#47408=DIRECTION('center_axis',(0.,-0.608761429008722,-0.793353340291234));
#47409=DIRECTION('ref_axis',(1.6355129777956E-16,0.793353340291234,-0.608761429008722));
#47410=DIRECTION('',(0.,0.99144486137381,0.130526192220052));
#47411=DIRECTION('center_axis',(0.706796314701322,-0.701365059961628,-0.0923364618644847));
#47412=DIRECTION('ref_axis',(0.,0.130526192220055,-0.99144486137381));
#47413=DIRECTION('center_axis',(-0.706790970014513,0.701370354233776,0.0923371588686358));
#47414=DIRECTION('ref_axis',(0.707106781190773,0.696532689773528,0.121828617618681));
#47415=DIRECTION('center_axis',(0.,0.,1.));
#47416=DIRECTION('ref_axis',(1.,0.,0.));
#47417=DIRECTION('center_axis',(0.,0.172291683322539,-0.98504597651982));
#47418=DIRECTION('ref_axis',(0.,0.98504597651982,0.172291683322539));
#47419=DIRECTION('center_axis',(1.,0.,0.));
#47420=DIRECTION('ref_axis',(0.,0.,-1.));
#47421=DIRECTION('center_axis',(1.,0.,0.));
#47422=DIRECTION('ref_axis',(0.,0.981569683813102,0.191104567760813));
#47423=DIRECTION('center_axis',(2.38512309261853E-15,0.218134291185378,
-0.975918762504878));
#47424=DIRECTION('ref_axis',(-0.707106781186563,0.690078774854368,0.154244236506497));
#47425=DIRECTION('center_axis',(-1.,0.,0.));
#47426=DIRECTION('ref_axis',(0.,0.981569683813102,0.191104567760813));
#47427=DIRECTION('center_axis',(-1.,0.,0.));
#47428=DIRECTION('ref_axis',(0.,0.805930996937512,-0.592009483180217));
#47429=DIRECTION('',(1.,0.,0.));
#47430=DIRECTION('center_axis',(-1.,0.,0.));
#47431=DIRECTION('ref_axis',(0.,0.985107749339347,0.171938134779827));
#47432=DIRECTION('',(-1.,0.,0.));
#47433=DIRECTION('center_axis',(0.,0.,1.));
#47434=DIRECTION('ref_axis',(1.,0.,0.));
#47435=DIRECTION('center_axis',(0.,0.171938134779822,-0.985107749339348));
#47436=DIRECTION('ref_axis',(0.,0.985107749339348,0.171938134779822));
#47437=DIRECTION('center_axis',(-0.706796314705252,-0.683312457872063,-0.183093021264917));
#47438=DIRECTION('ref_axis',(0.,-0.258819045102485,0.965925826289078));
#47439=DIRECTION('center_axis',(0.706790970015314,0.683317615876694,0.183094403348115));
#47440=DIRECTION('ref_axis',(-0.707106781189973,0.690134089358187,0.153996554185158));
#47441=DIRECTION('center_axis',(-0.939647353856836,-0.247923894858438,-0.235789297356919));
#47442=DIRECTION('ref_axis',(-0.342144487592387,0.680884948347207,0.647559137627109));
#47443=DIRECTION('center_axis',(-1.,0.,0.));
#47444=DIRECTION('ref_axis',(0.,0.518030931670901,0.85536188472025));
#47445=DIRECTION('center_axis',(0.,0.,1.));
#47446=DIRECTION('ref_axis',(-0.921538338698208,-0.388287381084355,0.));
#47447=DIRECTION('center_axis',(0.,-0.217784015488421,0.975996989031083));
#47448=DIRECTION('ref_axis',(0.,0.975996989031083,0.217784015488421));
#47449=DIRECTION('center_axis',(1.,0.,0.));
#47450=DIRECTION('ref_axis',(0.,1.,0.));
#47451=DIRECTION('',(-1.,0.,0.));
#47452=DIRECTION('center_axis',(1.,0.,0.));
#47453=DIRECTION('ref_axis',(0.,0.981569683813102,0.191104567760813));
#47454=DIRECTION('center_axis',(1.,0.,0.));
#47455=DIRECTION('ref_axis',(0.,0.518030931670901,0.85536188472025));
#47456=DIRECTION('',(1.,0.,0.));
#47457=DIRECTION('center_axis',(1.,0.,0.));
#47458=DIRECTION('ref_axis',(0.,0.518030931670901,0.85536188472025));
#47459=DIRECTION('center_axis',(0.,0.258819045102521,-0.965925826289068));
#47460=DIRECTION('ref_axis',(-1.,0.,0.));
#47461=DIRECTION('',(-1.,0.,0.));
#47462=DIRECTION('center_axis',(0.,0.258819045102521,-0.965925826289068));
#47463=DIRECTION('ref_axis',(0.707106781186523,0.683012701892242,0.183012701892228));
#47464=DIRECTION('center_axis',(1.,0.,0.));
#47465=DIRECTION('ref_axis',(0.,0.,-1.));
#47466=DIRECTION('center_axis',(-1.,0.,0.));
#47467=DIRECTION('ref_axis',(0.,0.980785280403231,0.195090322016128));
#47468=DIRECTION('center_axis',(1.,0.,0.));
#47469=DIRECTION('ref_axis',(0.,1.,0.));
#47470=DIRECTION('',(-0.706902428155816,-0.701259930876578,-0.0923226213578654));
#47471=DIRECTION('center_axis',(-0.706790970016278,0.61264581409456,0.353711225685393));
#47472=DIRECTION('ref_axis',(0.,-0.500000000000001,0.866025403784438));
#47473=DIRECTION('center_axis',(0.706796314705264,-0.612641189554924,-0.353708555706227));
#47474=DIRECTION('ref_axis',(0.707106781186549,0.626643564800585,0.3275940211512));
#47475=DIRECTION('center_axis',(1.,0.,0.));
#47476=DIRECTION('ref_axis',(0.,0.,-1.));
#47477=DIRECTION('center_axis',(1.,0.,0.));
#47478=DIRECTION('ref_axis',(0.,0.898662006154886,0.438641765788069));
#47479=DIRECTION('center_axis',(1.23515303010605E-14,0.463287907664357,
-0.886207828114818));
#47480=DIRECTION('ref_axis',(0.,0.886207828114818,0.463287907664357));
#47481=DIRECTION('center_axis',(0.192364553135132,-0.871675368857562,0.450752626197734));
#47482=DIRECTION('ref_axis',(0.342144487592246,0.490083718692063,0.80172008723943));
#47483=DIRECTION('center_axis',(1.,0.,0.));
#47484=DIRECTION('ref_axis',(0.,0.278995509497105,0.96029240634322));
#47485=DIRECTION('center_axis',(0.,-0.866025403784439,-0.5));
#47486=DIRECTION('ref_axis',(0.707106781186566,-0.353553390593262,0.61237243569578));
#47487=DIRECTION('center_axis',(0.,-0.866025403784441,-0.499999999999997));
#47488=DIRECTION('ref_axis',(1.,0.,0.));
#47489=DIRECTION('',(0.,-0.866025403784439,-0.5));
#47490=DIRECTION('center_axis',(0.,-0.965925826289065,0.258819045102532));
#47491=DIRECTION('ref_axis',(-2.04439122224448E-16,0.258819045102532,0.965925826289065));
#47492=DIRECTION('center_axis',(0.,0.,1.));
#47493=DIRECTION('ref_axis',(1.,0.,0.));
#47494=DIRECTION('center_axis',(0.,-0.38268343236509,0.923879532511287));
#47495=DIRECTION('ref_axis',(1.,0.,0.));
#47496=DIRECTION('',(1.,0.,0.));
#47497=DIRECTION('center_axis',(0.,-0.38268343236509,0.923879532511287));
#47498=DIRECTION('ref_axis',(-0.70710678118656,0.653281482438176,0.270598050073096));
#47499=DIRECTION('',(-0.706902428155816,-0.65347022547417,-0.270676229998403));
#47500=DIRECTION('center_axis',(0.706790970016286,0.61264581409455,0.353711225685393));
#47501=DIRECTION('ref_axis',(0.,0.500000000000008,-0.866025403784434));
#47502=DIRECTION('center_axis',(-0.706796314705265,-0.612641189554918,-0.353708555706235));
#47503=DIRECTION('ref_axis',(-0.70710678118655,0.597026526845132,0.37889223565974));
#47504=DIRECTION('center_axis',(0.,-0.866025403784439,-0.5));
#47505=DIRECTION('ref_axis',(-0.707106781186556,0.353553390593278,-0.612372435695782));
#47506=DIRECTION('center_axis',(0.,-0.866025403784442,-0.499999999999995));
#47507=DIRECTION('ref_axis',(-1.,0.,0.));
#47508=DIRECTION('',(0.,-0.866025403784439,-0.5));
#47509=DIRECTION('center_axis',(0.,-0.258819045102519,-0.965925826289069));
#47510=DIRECTION('ref_axis',(4.08878244448899E-17,0.965925826289069,-0.258819045102519));
#47511=DIRECTION('center_axis',(0.,0.,1.));
#47512=DIRECTION('ref_axis',(1.,0.,0.));
#47513=DIRECTION('center_axis',(0.,0.,1.));
#47514=DIRECTION('ref_axis',(1.,0.,0.));
#47515=DIRECTION('center_axis',(-1.,0.,0.));
#47516=DIRECTION('ref_axis',(0.,0.971135373703069,-0.238529004405336));
#47517=DIRECTION('center_axis',(0.,0.608761429008721,-0.793353340291235));
#47518=DIRECTION('ref_axis',(-1.,0.,0.));
#47519=DIRECTION('',(-1.,0.,0.));
#47520=DIRECTION('center_axis',(0.,0.608761429008721,-0.793353340291235));
#47521=DIRECTION('ref_axis',(0.707106781186524,0.560985526796945,0.430459334576899));
#47522=DIRECTION('',(0.706902428155818,-0.561147604116303,-0.43058370087817));
#47523=DIRECTION('center_axis',(0.,0.130526192220052,0.99144486137381));
#47524=DIRECTION('ref_axis',(-0.707106781186558,-0.701057384649966,0.0922959556412686));
#47525=DIRECTION('center_axis',(4.83043946397857E-16,-0.130526192220055,
-0.99144486137381));
#47526=DIRECTION('ref_axis',(0.,-0.99144486137381,0.130526192220055));
#47527=DIRECTION('center_axis',(0.,-0.793353340291236,-0.60876142900872));
#47528=DIRECTION('ref_axis',(8.17756488897799E-17,-0.60876142900872,0.793353340291236));
#47529=DIRECTION('',(0.,0.130526192220052,0.99144486137381));
#47530=DIRECTION('center_axis',(-0.706796314701307,-0.092336461864487,-0.701365059961643));
#47531=DIRECTION('ref_axis',(0.,-0.99144486137381,0.130526192220056));
#47532=DIRECTION('center_axis',(0.70679097001461,0.0923371588686235,0.701370354233679));
#47533=DIRECTION('ref_axis',(-0.707106781190676,0.121828617618699,0.696532689773623));
#47534=DIRECTION('center_axis',(0.,0.,1.));
#47535=DIRECTION('ref_axis',(-0.764784300456449,-0.644286406635543,0.));
#47536=DIRECTION('center_axis',(0.,-0.98504597651982,0.172291683322539));
#47537=DIRECTION('ref_axis',(0.,0.172291683322539,0.98504597651982));
#47538=DIRECTION('center_axis',(1.,0.,0.));
#47539=DIRECTION('ref_axis',(0.,-0.592009483180214,0.805930996937515));
#47540=DIRECTION('',(-1.,0.,0.));
#47541=DIRECTION('center_axis',(1.,0.,0.));
#47542=DIRECTION('ref_axis',(0.,0.171938134779829,0.985107749339347));
#47543=DIRECTION('',(1.,0.,0.));
#47544=DIRECTION('center_axis',(0.122754826313525,-0.941252632833091,-0.314602501263912));
#47545=DIRECTION('ref_axis',(-0.342144487575903,-0.337703244261558,0.876865821227308));
#47546=DIRECTION('center_axis',(0.,-0.985107749339348,0.171938134779822));
#47547=DIRECTION('ref_axis',(0.,0.171938134779822,0.985107749339348));
#47548=DIRECTION('center_axis',(1.,0.,0.));
#47549=DIRECTION('ref_axis',(0.,0.,-1.));
#47550=DIRECTION('center_axis',(-1.,0.,0.));
#47551=DIRECTION('ref_axis',(0.,0.195090322016129,0.98078528040323));
#47552=DIRECTION('center_axis',(0.,0.975996989031084,-0.217784015488416));
#47553=DIRECTION('ref_axis',(0.,0.217784015488416,0.975996989031084));
#47554=DIRECTION('center_axis',(1.,0.,0.));
#47555=DIRECTION('ref_axis',(0.,1.,0.));
#47556=DIRECTION('center_axis',(1.,0.,0.));
#47557=DIRECTION('ref_axis',(0.,0.191104567760813,0.981569683813102));
#47558=DIRECTION('center_axis',(1.,0.,0.));
#47559=DIRECTION('ref_axis',(0.,0.,-1.));
#47560=DIRECTION('center_axis',(-1.,0.,0.));
#47561=DIRECTION('ref_axis',(0.,0.191104567760813,0.981569683813102));
#47562=DIRECTION('center_axis',(3.10917831716354E-15,-0.975918762504879,
0.218134291185374));
#47563=DIRECTION('ref_axis',(0.,0.218134291185374,0.975918762504879));
#47564=DIRECTION('center_axis',(1.,0.,0.));
#47565=DIRECTION('ref_axis',(0.,1.,0.));
#47566=DIRECTION('center_axis',(1.,0.,0.));
#47567=DIRECTION('ref_axis',(0.,0.,-1.));
#47568=DIRECTION('',(1.,0.,0.));
#47569=DIRECTION('center_axis',(0.706790970016471,0.430651502409209,0.561235964791876));
#47570=DIRECTION('ref_axis',(0.,0.79335334029124,-0.608761429008714));
#47571=DIRECTION('center_axis',(-0.706796314705261,-0.430648251648628,-0.561231728318206));
#47572=DIRECTION('ref_axis',(-0.707106781186552,0.40658480727975,0.578522942059589));
#47573=DIRECTION('center_axis',(0.,-0.608761429008721,-0.793353340291235));
#47574=DIRECTION('ref_axis',(-0.707106781186562,0.560985526796919,-0.430459334576871));
#47575=DIRECTION('center_axis',(-9.01147939985612E-15,-0.608761429008721,
-0.793353340291235));
#47576=DIRECTION('ref_axis',(-1.,1.48029736616691E-14,0.));
#47577=DIRECTION('',(0.,-0.608761429008721,-0.793353340291235));
#47578=DIRECTION('center_axis',(0.,0.130526192220051,-0.991444861373811));
#47579=DIRECTION('ref_axis',(4.088782444489E-17,0.991444861373811,0.130526192220051));
#47580=DIRECTION('center_axis',(0.,0.,1.));
#47581=DIRECTION('ref_axis',(1.,0.,0.));
#47582=DIRECTION('center_axis',(0.,0.,1.));
#47583=DIRECTION('ref_axis',(1.,0.,0.));
#47584=DIRECTION('center_axis',(-1.,0.,0.));
#47585=DIRECTION('ref_axis',(0.,0.988493193186426,0.151265353019466));
#47586=DIRECTION('center_axis',(0.,0.866025403784439,-0.5));
#47587=DIRECTION('ref_axis',(-1.,0.,0.));
#47588=DIRECTION('',(-1.,0.,0.));
#47589=DIRECTION('center_axis',(0.,0.866025403784439,-0.5));
#47590=DIRECTION('ref_axis',(0.70710678118651,0.353553390593297,0.612372435695825));
#47591=DIRECTION('',(0.706902428155815,-0.353655537588269,-0.612549359480985));
#47592=DIRECTION('center_axis',(0.,0.707106781186548,0.707106781186548));
#47593=DIRECTION('ref_axis',(0.70710678118657,0.499999999999984,-0.499999999999984));
#47594=DIRECTION('center_axis',(-1.04672830578914E-14,-0.707106781186548,
-0.707106781186548));
#47595=DIRECTION('ref_axis',(0.,0.707106781186547,-0.707106781186547));
#47596=DIRECTION('center_axis',(0.,-1.0467283057892E-14,-1.));
#47597=DIRECTION('ref_axis',(-4.08878244448904E-17,1.,-1.04950770296598E-14));
#47598=DIRECTION('',(0.,0.707106781186548,0.707106781186548));
#47599=DIRECTION('center_axis',(0.706796314703387,-0.50021943660843,-0.50021943660843));
#47600=DIRECTION('ref_axis',(0.,0.707106781186547,-0.707106781186547));
#47601=DIRECTION('center_axis',(-0.706790970016736,0.500223212527568,0.500223212527568));
#47602=DIRECTION('ref_axis',(0.70710678118855,0.478431972699649,0.520675376310317));
#47603=DIRECTION('center_axis',(0.,0.,1.));
#47604=DIRECTION('ref_axis',(1.,0.,0.));
#47605=DIRECTION('center_axis',(0.,0.736346178773833,-0.676604984466694));
#47606=DIRECTION('ref_axis',(0.,0.676604984466694,0.736346178773833));
#47607=DIRECTION('center_axis',(-1.,0.,0.));
#47608=DIRECTION('ref_axis',(0.,0.999780587432124,0.0209470044129973));
#47609=DIRECTION('',(1.,0.,0.));
#47610=DIRECTION('center_axis',(-1.,0.,0.));
#47611=DIRECTION('ref_axis',(0.,0.676869218855486,0.73610329476641));
#47612=DIRECTION('',(-1.,0.,0.));
#47613=DIRECTION('center_axis',(0.,0.,1.));
#47614=DIRECTION('ref_axis',(1.,0.,0.));
#47615=DIRECTION('center_axis',(0.,0.736103294766404,-0.676869218855492));
#47616=DIRECTION('ref_axis',(0.,0.676869218855492,0.736103294766404));
#47617=DIRECTION('center_axis',(1.,0.,0.));
#47618=DIRECTION('ref_axis',(0.,0.,-1.));
#47619=DIRECTION('center_axis',(1.,0.,0.));
#47620=DIRECTION('ref_axis',(0.,0.659345815100069,0.751839807478978));
#47621=DIRECTION('center_axis',(0.,-0.766928997900546,0.64173196287801));
#47622=DIRECTION('ref_axis',(0.,0.64173196287801,0.766928997900546));
#47623=DIRECTION('center_axis',(-1.,0.,0.));
#47624=DIRECTION('ref_axis',(0.,1.,0.));
#47625=DIRECTION('center_axis',(-1.,0.,0.));
#47626=DIRECTION('ref_axis',(0.,0.662394497621569,0.749155210567656));
#47627=DIRECTION('center_axis',(0.706790970016578,0.561235964791791,0.430651502409143));
#47628=DIRECTION('ref_axis',(0.,0.608761429008714,-0.79335334029124));
#47629=DIRECTION('center_axis',(-0.706796314705263,-0.561231728318196,-0.430648251648639));
#47630=DIRECTION('ref_axis',(-0.707106781186551,0.542463521362041,0.453578359262751));
#47631=DIRECTION('center_axis',(0.,-0.793353340291235,-0.608761429008721));
#47632=DIRECTION('ref_axis',(-0.707106781186558,0.430459334576869,-0.560985526796926));
#47633=DIRECTION('center_axis',(2.7325092008722E-15,-0.793353340291235,
-0.608761429008721));
#47634=DIRECTION('ref_axis',(-1.,-1.48029736616691E-14,1.48029736616691E-14));
#47635=DIRECTION('',(0.,-0.793353340291235,-0.608761429008721));
#47636=DIRECTION('center_axis',(0.,-0.130526192220051,-0.991444861373811));
#47637=DIRECTION('ref_axis',(-8.17756488897799E-17,0.99144486137381,-0.130526192220051));
#47638=DIRECTION('center_axis',(0.,0.,1.));
#47639=DIRECTION('ref_axis',(1.,0.,0.));
#47640=DIRECTION('center_axis',(0.,0.,1.));
#47641=DIRECTION('ref_axis',(1.,0.,0.));
#47642=DIRECTION('center_axis',(-1.,0.,0.));
#47643=DIRECTION('ref_axis',(0.,0.993961458635313,-0.109729753246606));
#47644=DIRECTION('center_axis',(-1.,0.,0.));
#47645=DIRECTION('ref_axis',(0.,0.993961458635313,-0.109729753246601));
#47646=DIRECTION('',(-1.,0.,0.));
#47647=DIRECTION('center_axis',(0.,-0.608761429008721,0.793353340291235));
#47648=DIRECTION('ref_axis',(1.,0.,0.));
#47649=DIRECTION('',(-0.706902428155818,0.561147604116303,0.43058370087817));
#47650=DIRECTION('center_axis',(0.,-0.608761429008721,0.793353340291235));
#47651=DIRECTION('ref_axis',(0.707106781186524,0.560985526796945,0.430459334576899));
#47652=DIRECTION('',(1.,0.,0.));
#47653=DIRECTION('center_axis',(-0.706790970016564,0.430651502409157,0.561235964791798));
#47654=DIRECTION('ref_axis',(0.,-0.793353340291235,0.608761429008721));
#47655=DIRECTION('center_axis',(0.706796314705262,-0.430648251648606,-0.561231728318222));
#47656=DIRECTION('ref_axis',(0.707106781186551,0.453578359262751,0.542463521362041));
#47657=DIRECTION('center_axis',(1.,0.,0.));
#47658=DIRECTION('ref_axis',(0.,0.,-1.));
#47659=DIRECTION('center_axis',(1.,0.,0.));
#47660=DIRECTION('ref_axis',(0.,0.662394497621569,0.749155210567656));
#47661=DIRECTION('center_axis',(4.25914837967634E-15,0.767159269002869,
-0.641456667268323));
#47662=DIRECTION('ref_axis',(0.,0.641456667268323,0.767159269002869));
#47663=DIRECTION('center_axis',(0.0504847333736789,-0.989288526783089,0.136965333101244));
#47664=DIRECTION('ref_axis',(0.342144487592341,0.145973322135748,0.92823969901897));
#47665=DIRECTION('center_axis',(1.,0.,0.));
#47666=DIRECTION('ref_axis',(0.,-0.109729753246606,0.993961458635313));
#47667=DIRECTION('center_axis',(0.,-0.608761429008721,-0.793353340291235));
#47668=DIRECTION('ref_axis',(0.707106781186562,-0.560985526796919,0.430459334576871));
#47669=DIRECTION('center_axis',(0.,-0.608761429008721,-0.793353340291235));
#47670=DIRECTION('ref_axis',(1.,0.,0.));
#47671=DIRECTION('',(0.,-0.608761429008721,-0.793353340291235));
#47672=DIRECTION('center_axis',(0.,-0.991444861373809,-0.13052619222006));
#47673=DIRECTION('ref_axis',(-1.22663473334671E-16,-0.13052619222006,0.991444861373809));
#47674=DIRECTION('center_axis',(0.,0.,1.));
#47675=DIRECTION('ref_axis',(1.,0.,0.));
#47676=DIRECTION('center_axis',(0.,-0.707106781186548,0.707106781186548));
#47677=DIRECTION('ref_axis',(1.,0.,0.));
#47678=DIRECTION('',(1.,0.,0.));
#47679=DIRECTION('center_axis',(0.,-0.707106781186548,0.707106781186548));
#47680=DIRECTION('ref_axis',(-0.707106781186567,0.499999999999981,0.499999999999992));
#47681=DIRECTION('',(-0.706902428155815,-0.500144457665692,-0.500144457665686));
#47682=DIRECTION('center_axis',(-1.,0.,0.));
#47683=DIRECTION('ref_axis',(0.,0.988493193186426,0.151265353019465));
#47684=DIRECTION('',(-1.,0.,0.));
#47685=DIRECTION('center_axis',(0.,-0.793353340291235,0.608761429008721));
#47686=DIRECTION('ref_axis',(1.,0.,0.));
#47687=DIRECTION('',(-0.70690242815582,0.430583700878172,0.561147604116298));
#47688=DIRECTION('center_axis',(0.,-0.793353340291235,0.608761429008721));
#47689=DIRECTION('ref_axis',(0.707106781186516,0.430459334576894,0.56098552679696));
#47690=DIRECTION('',(1.,0.,0.));
#47691=DIRECTION('center_axis',(0.,0.38268343236509,0.923879532511287));
#47692=DIRECTION('ref_axis',(0.707106781186561,0.653281482438177,-0.270598050073091));
#47693=DIRECTION('center_axis',(0.,-0.382683432365087,-0.923879532511288));
#47694=DIRECTION('ref_axis',(0.,0.923879532511288,-0.382683432365087));
#47695=DIRECTION('center_axis',(0.,0.382683432365082,-0.92387953251129));
#47696=DIRECTION('ref_axis',(1.22663473334671E-16,0.92387953251129,0.382683432365082));
#47697=DIRECTION('',(0.,0.38268343236509,0.923879532511287));
#47698=DIRECTION('center_axis',(0.706796314702752,-0.270716808310053,-0.653568190184487));
#47699=DIRECTION('ref_axis',(0.,0.923879532511287,-0.382683432365089));
#47700=DIRECTION('center_axis',(-0.706790970016031,0.270718851822791,0.653573123660656));
#47701=DIRECTION('ref_axis',(0.707106781189256,0.242759667121566,0.664129312720946));
#47702=DIRECTION('center_axis',(0.,0.,1.));
#47703=DIRECTION('ref_axis',(1.,0.,0.));
#47704=DIRECTION('center_axis',(0.,0.939220681223083,-0.343314013641807));
#47705=DIRECTION('ref_axis',(0.,0.343314013641807,0.939220681223083));
#47706=DIRECTION('center_axis',(-1.,0.,0.));
#47707=DIRECTION('ref_axis',(0.,0.915660750184117,0.401951975455104));
#47708=DIRECTION('',(1.,0.,0.));
#47709=DIRECTION('center_axis',(-1.,0.,0.));
#47710=DIRECTION('ref_axis',(0.,0.34365108207103,0.939097403782702));
#47711=DIRECTION('',(-1.,0.,0.));
#47712=DIRECTION('center_axis',(0.,0.,1.));
#47713=DIRECTION('ref_axis',(1.,0.,0.));
#47714=DIRECTION('center_axis',(0.,0.9390974037827,-0.343651082071034));
#47715=DIRECTION('ref_axis',(0.,0.343651082071034,0.9390974037827));
#47716=DIRECTION('center_axis',(1.,0.,0.));
#47717=DIRECTION('ref_axis',(0.,0.,-1.));
#47718=DIRECTION('center_axis',(1.,0.,0.));
#47719=DIRECTION('ref_axis',(0.,0.321439465303162,0.946930129495105));
#47720=DIRECTION('center_axis',(0.,-0.95413019426225,0.299392004564386));
#47721=DIRECTION('ref_axis',(0.,0.299392004564386,0.95413019426225));
#47722=DIRECTION('center_axis',(-1.,0.,0.));
#47723=DIRECTION('ref_axis',(0.,1.,0.));
#47724=DIRECTION('center_axis',(-1.,0.,0.));
#47725=DIRECTION('ref_axis',(0.,0.325283431446442,0.945616565647212));
#47726=DIRECTION('center_axis',(0.,-0.258819045102521,0.965925826289068));
#47727=DIRECTION('ref_axis',(-0.70710678118656,-0.683012701892206,-0.183012701892221));
#47728=DIRECTION('center_axis',(-1.52563974426308E-14,0.258819045102528,
-0.965925826289066));
#47729=DIRECTION('ref_axis',(0.,-0.965925826289066,-0.258819045102528));
#47730=DIRECTION('center_axis',(0.,-0.500000000000007,-0.866025403784435));
#47731=DIRECTION('ref_axis',(-8.17756488897793E-17,-0.866025403784435,0.500000000000007));
#47732=DIRECTION('',(0.,-0.258819045102521,0.965925826289068));
#47733=DIRECTION('center_axis',(-0.706796314702156,0.183093021265739,-0.683312457875045));
#47734=DIRECTION('ref_axis',(0.,-0.96592582628907,-0.258819045102514));
#47735=DIRECTION('center_axis',(0.706790970015427,-0.183094403348086,0.683317615876585));
#47736=DIRECTION('ref_axis',(-0.707106781189859,-0.153996554185177,0.690134089358299));
#47737=DIRECTION('center_axis',(0.,0.,1.));
#47738=DIRECTION('ref_axis',(1.,0.,0.));
#47739=DIRECTION('center_axis',(0.,-0.975996989031084,-0.217784015488416));
#47740=DIRECTION('ref_axis',(0.,-0.217784015488416,0.975996989031084));
#47741=DIRECTION('center_axis',(1.,0.,0.));
#47742=DIRECTION('ref_axis',(0.,-0.855361884720257,0.51803093167089));
#47743=DIRECTION('',(-1.,0.,0.));
#47744=DIRECTION('center_axis',(1.,0.,0.));
#47745=DIRECTION('ref_axis',(0.,-0.218134291185384,0.975918762504877));
#47746=DIRECTION('',(1.,0.,0.));
#47747=DIRECTION('center_axis',(0.,0.,1.));
#47748=DIRECTION('ref_axis',(1.,0.,0.));
#47749=DIRECTION('center_axis',(0.,-0.975918762504877,-0.218134291185385));
#47750=DIRECTION('ref_axis',(0.,-0.218134291185385,0.975918762504877));
#47751=DIRECTION('center_axis',(1.,0.,0.));
#47752=DIRECTION('ref_axis',(0.,0.,-1.));
#47753=DIRECTION('center_axis',(-1.,0.,0.));
#47754=DIRECTION('ref_axis',(0.,-0.195090322016128,0.980785280403231));
#47755=DIRECTION('center_axis',(0.,0.98504597651982,0.172291683322539));
#47756=DIRECTION('ref_axis',(0.,-0.172291683322539,0.98504597651982));
#47757=DIRECTION('center_axis',(1.,0.,0.));
#47758=DIRECTION('ref_axis',(0.,1.,0.));
#47759=DIRECTION('center_axis',(1.,0.,0.));
#47760=DIRECTION('ref_axis',(0.,-0.199072856983482,0.979984692539855));
#47761=DIRECTION('center_axis',(1.,0.,0.));
#47762=DIRECTION('ref_axis',(0.,0.,-1.));
#47763=DIRECTION('center_axis',(-1.,0.,0.));
#47764=DIRECTION('ref_axis',(0.,-0.199072856983482,0.979984692539855));
#47765=DIRECTION('center_axis',(1.66106786807382E-14,-0.985107749339348,
-0.171938134779824));
#47766=DIRECTION('ref_axis',(0.,-0.171938134779824,0.985107749339348));
#47767=DIRECTION('center_axis',(1.,0.,0.));
#47768=DIRECTION('ref_axis',(0.,1.,0.));
#47769=DIRECTION('center_axis',(1.,0.,0.));
#47770=DIRECTION('ref_axis',(0.,0.,-1.));
#47771=DIRECTION('',(1.,0.,0.));
#47772=DIRECTION('center_axis',(0.,-0.38268343236509,0.923879532511287));
#47773=DIRECTION('ref_axis',(-0.70710678118656,-0.653281482438179,-0.270598050073091));
#47774=DIRECTION('center_axis',(-1.36761643863197E-14,0.382683432365087,
-0.923879532511288));
#47775=DIRECTION('ref_axis',(0.,-0.923879532511288,-0.382683432365087));
#47776=DIRECTION('center_axis',(0.,-0.382683432365084,-0.923879532511289));
#47777=DIRECTION('ref_axis',(4.08878244448902E-17,-0.923879532511289,0.382683432365084));
#47778=DIRECTION('',(0.,-0.38268343236509,0.923879532511287));
#47779=DIRECTION('center_axis',(-0.706796314702752,0.270716808310051,-0.653568190184488));
#47780=DIRECTION('ref_axis',(0.,-0.923879532511288,-0.382683432365087));
#47781=DIRECTION('center_axis',(0.706790970016079,-0.270718851822771,0.653573123660613));
#47782=DIRECTION('ref_axis',(-0.707106781189208,-0.242759667121587,0.66412931272099));
#47783=DIRECTION('center_axis',(0.,0.,1.));
#47784=DIRECTION('ref_axis',(1.,0.,0.));
#47785=DIRECTION('center_axis',(0.,-0.939220681223084,-0.343314013641807));
#47786=DIRECTION('ref_axis',(0.,-0.343314013641807,0.939220681223084));
#47787=DIRECTION('center_axis',(1.,0.,0.));
#47788=DIRECTION('ref_axis',(0.,-0.915660750184117,0.401951975455104));
#47789=DIRECTION('',(-1.,0.,0.));
#47790=DIRECTION('center_axis',(1.,0.,0.));
#47791=DIRECTION('ref_axis',(0.,-0.343651082071035,0.9390974037827));
#47792=DIRECTION('',(1.,0.,0.));
#47793=DIRECTION('center_axis',(0.,0.,1.));
#47794=DIRECTION('ref_axis',(1.,0.,0.));
#47795=DIRECTION('center_axis',(0.,-0.9390974037827,-0.343651082071034));
#47796=DIRECTION('ref_axis',(0.,-0.343651082071034,0.9390974037827));
#47797=DIRECTION('center_axis',(1.,0.,0.));
#47798=DIRECTION('ref_axis',(0.,0.,-1.));
#47799=DIRECTION('center_axis',(-1.,0.,0.));
#47800=DIRECTION('ref_axis',(0.,-0.321439465303161,0.946930129495106));
#47801=DIRECTION('center_axis',(0.,0.954130194262249,0.29939200456439));
#47802=DIRECTION('ref_axis',(0.,-0.29939200456439,0.954130194262249));
#47803=DIRECTION('center_axis',(1.,0.,0.));
#47804=DIRECTION('ref_axis',(0.,1.,0.));
#47805=DIRECTION('center_axis',(1.,0.,0.));
#47806=DIRECTION('ref_axis',(0.,-0.325283431446442,0.945616565647212));
#47807=DIRECTION('center_axis',(1.,0.,0.));
#47808=DIRECTION('ref_axis',(0.,0.,-1.));
#47809=DIRECTION('center_axis',(-1.,0.,0.));
#47810=DIRECTION('ref_axis',(0.,-0.325283431446442,0.945616565647212));
#47811=DIRECTION('center_axis',(5.53689289357886E-15,-0.95423758595179,
-0.299049543649378));
#47812=DIRECTION('ref_axis',(0.,-0.299049543649378,0.95423758595179));
#47813=DIRECTION('center_axis',(1.,0.,0.));
#47814=DIRECTION('ref_axis',(0.,1.,0.));
#47815=DIRECTION('center_axis',(1.,0.,0.));
#47816=DIRECTION('ref_axis',(0.,0.,-1.));
#47817=DIRECTION('',(1.,0.,0.));
#47818=DIRECTION('center_axis',(0.706790970015306,0.183094403348117,0.683317615876701));
#47819=DIRECTION('ref_axis',(0.,0.96592582628907,-0.258819045102514));
#47820=DIRECTION('center_axis',(-0.706796314705253,-0.183093021264917,-0.683312457872062));
#47821=DIRECTION('ref_axis',(-0.707106781186562,0.154244236506507,0.690078774854367));
#47822=DIRECTION('center_axis',(0.,-0.258819045102521,-0.965925826289068));
#47823=DIRECTION('ref_axis',(-0.707106781186562,0.683012701892204,-0.183012701892221));
#47824=DIRECTION('center_axis',(-9.57822876947717E-16,-0.258819045102515,
-0.96592582628907));
#47825=DIRECTION('ref_axis',(-1.,3.70074341541727E-15,0.));
#47826=DIRECTION('',(0.,-0.258819045102521,-0.965925826289068));
#47827=DIRECTION('center_axis',(0.,0.500000000000007,-0.866025403784435));
#47828=DIRECTION('ref_axis',(8.17756488897793E-17,0.866025403784435,0.500000000000007));
#47829=DIRECTION('center_axis',(0.,0.,1.));
#47830=DIRECTION('ref_axis',(1.,0.,0.));
#47831=DIRECTION('center_axis',(0.,0.,1.));
#47832=DIRECTION('ref_axis',(1.,0.,0.));
#47833=DIRECTION('center_axis',(-1.,0.,0.));
#47834=DIRECTION('ref_axis',(0.,0.855361884720257,0.518030931670889));
#47835=DIRECTION('center_axis',(0.,0.99144486137381,-0.130526192220052));
#47836=DIRECTION('ref_axis',(-1.,0.,0.));
#47837=DIRECTION('',(-1.,0.,0.));
#47838=DIRECTION('center_axis',(0.,0.99144486137381,-0.130526192220052));
#47839=DIRECTION('ref_axis',(0.707106781186521,0.0922959556412538,0.701057384650005));
#47840=DIRECTION('',(0.706902428155816,-0.0923226213578653,-0.701259930876578));
#47841=DIRECTION('center_axis',(0.,0.38268343236509,0.923879532511287));
#47842=DIRECTION('ref_axis',(-0.707106781186561,-0.653281482438177,0.270598050073091));
#47843=DIRECTION('center_axis',(0.,-0.382683432365087,-0.923879532511288));
#47844=DIRECTION('ref_axis',(0.,-0.923879532511288,0.382683432365087));
#47845=DIRECTION('center_axis',(0.,-0.923879532511289,-0.382683432365085));
#47846=DIRECTION('ref_axis',(8.17756488897795E-17,-0.382683432365085,0.923879532511289));
#47847=DIRECTION('',(0.,0.38268343236509,0.923879532511287));
#47848=DIRECTION('center_axis',(-0.706796314702627,-0.270716808310098,-0.653568190184604));
#47849=DIRECTION('ref_axis',(0.,-0.923879532511288,0.382683432365087));
#47850=DIRECTION('center_axis',(0.70679097001594,0.270718851822824,0.653573123660741));
#47851=DIRECTION('ref_axis',(-0.707106781189346,0.297953333789463,0.641267347429905));
#47852=DIRECTION('center_axis',(0.,0.,1.));
#47853=DIRECTION('ref_axis',(-0.833158187746081,-0.553034749533577,0.));
#47854=DIRECTION('center_axis',(0.,-0.906888979845984,0.421369645600998));
#47855=DIRECTION('ref_axis',(0.,0.421369645600998,0.906888979845984));
#47856=DIRECTION('center_axis',(1.,0.,0.));
#47857=DIRECTION('ref_axis',(0.,-0.363246958165936,0.931692893277176));
#47858=DIRECTION('',(-1.,0.,0.));
#47859=DIRECTION('center_axis',(1.,0.,0.));
#47860=DIRECTION('ref_axis',(0.,0.421044131914916,0.907040152903947));
#47861=DIRECTION('',(1.,0.,0.));
#47862=DIRECTION('center_axis',(0.0341251959389409,-0.995062857517424,-0.0931953893247336));
#47863=DIRECTION('ref_axis',(-0.342144487581446,-0.099246710722613,0.934391374119203));
#47864=DIRECTION('center_axis',(0.,-0.907040152903952,0.421044131914905));
#47865=DIRECTION('ref_axis',(0.,0.421044131914905,0.907040152903951));
#47866=DIRECTION('center_axis',(1.,0.,0.));
#47867=DIRECTION('ref_axis',(0.,0.,-1.));
#47868=DIRECTION('center_axis',(-1.,0.,0.));
#47869=DIRECTION('ref_axis',(0.,0.442288690219001,0.896872741532688));
#47870=DIRECTION('center_axis',(0.,0.886374047158188,-0.46296981383716));
#47871=DIRECTION('ref_axis',(0.,0.46296981383716,0.886374047158188));
#47872=DIRECTION('center_axis',(1.,0.,0.));
#47873=DIRECTION('ref_axis',(0.,1.,0.));
#47874=DIRECTION('center_axis',(1.,0.,0.));
#47875=DIRECTION('ref_axis',(0.,0.438641765788069,0.898662006154886));
#47876=DIRECTION('center_axis',(1.,0.,0.));
#47877=DIRECTION('ref_axis',(0.,0.,-1.));
#47878=DIRECTION('center_axis',(-1.,0.,0.));
#47879=DIRECTION('ref_axis',(0.,0.438641765788069,0.898662006154886));
#47880=DIRECTION('center_axis',(-1.24367132686542E-14,-0.886207828114817,
0.463287907664357));
#47881=DIRECTION('ref_axis',(0.,0.463287907664357,0.886207828114817));
#47882=DIRECTION('center_axis',(1.,0.,0.));
#47883=DIRECTION('ref_axis',(0.,1.,0.));
#47884=DIRECTION('center_axis',(1.,0.,0.));
#47885=DIRECTION('ref_axis',(0.,0.,-1.));
#47886=DIRECTION('',(1.,0.,0.));
#47887=DIRECTION('center_axis',(0.70679097001626,0.353711225685404,0.612645814094574));
#47888=DIRECTION('ref_axis',(0.,0.866025403784436,-0.500000000000005));
#47889=DIRECTION('center_axis',(-0.70679631470525,-0.353708555706216,-0.612641189554947));
#47890=DIRECTION('ref_axis',(-0.707106781186564,0.3275940211512,0.626643564800568));
#47891=DIRECTION('center_axis',(0.,-0.5,-0.866025403784439));
#47892=DIRECTION('ref_axis',(-0.707106781186556,0.612372435695782,-0.353553390593278));
#47893=DIRECTION('center_axis',(0.,-0.500000000000001,-0.866025403784438));
#47894=DIRECTION('ref_axis',(-1.,0.,0.));
#47895=DIRECTION('',(0.,-0.5,-0.866025403784439));
#47896=DIRECTION('center_axis',(0.,0.258819045102529,-0.965925826289066));
#47897=DIRECTION('ref_axis',(1.22663473334669E-16,0.965925826289066,0.258819045102529));
#47898=DIRECTION('center_axis',(0.,0.,1.));
#47899=DIRECTION('ref_axis',(1.,0.,0.));
#47900=DIRECTION('center_axis',(0.,0.,1.));
#47901=DIRECTION('ref_axis',(1.,0.,0.));
#47902=DIRECTION('center_axis',(-1.,0.,0.));
#47903=DIRECTION('ref_axis',(0.,0.96029240634322,0.278995509497105));
#47904=DIRECTION('center_axis',(0.,0.923879532511287,-0.38268343236509));
#47905=DIRECTION('ref_axis',(-1.,0.,0.));
#47906=DIRECTION('',(-1.,0.,0.));
#47907=DIRECTION('center_axis',(0.,0.923879532511287,-0.38268343236509));
#47908=DIRECTION('ref_axis',(0.707106781186519,0.270598050073107,0.653281482438216));
#47909=DIRECTION('',(0.706902428155818,-0.270676229998407,-0.653470225474167));
#47910=DIRECTION('center_axis',(-1.,0.,0.));
#47911=DIRECTION('ref_axis',(0.,0.855361884720257,0.51803093167089));
#47912=DIRECTION('',(-1.,0.,0.));
#47913=DIRECTION('center_axis',(0.,-0.965925826289068,0.258819045102521));
#47914=DIRECTION('ref_axis',(1.,0.,0.));
#47915=DIRECTION('',(-0.706902428155813,0.183065577067635,0.683210034733324));
#47916=DIRECTION('center_axis',(0.,-0.965925826289068,0.258819045102521));
#47917=DIRECTION('ref_axis',(0.707106781186512,0.18301270189223,0.683012701892253));
#47918=DIRECTION('',(1.,0.,0.));
#47919=DIRECTION('center_axis',(0.,-0.707106781186547,0.707106781186548));
#47920=DIRECTION('ref_axis',(-0.707106781186569,-0.499999999999985,-0.499999999999985));
#47921=DIRECTION('center_axis',(1.04672830578921E-14,0.707106781186548,
-0.707106781186548));
#47922=DIRECTION('ref_axis',(0.,-0.707106781186547,-0.707106781186547));
#47923=DIRECTION('center_axis',(0.,1.04672830578919E-14,-1.));
#47924=DIRECTION('ref_axis',(0.,-1.,-1.05239890875927E-14));
#47925=DIRECTION('',(0.,-0.707106781186547,0.707106781186548));
#47926=DIRECTION('center_axis',(-0.706796314703408,0.50021943660841,-0.500219436608421));
#47927=DIRECTION('ref_axis',(0.,-0.707106781186555,-0.70710678118654));
#47928=DIRECTION('center_axis',(0.706790970016716,-0.500223212527578,0.500223212527588));
#47929=DIRECTION('ref_axis',(-0.707106781188571,-0.478431972699648,0.520675376310289));
#47930=DIRECTION('center_axis',(0.,0.,1.));
#47931=DIRECTION('ref_axis',(1.,0.,0.));
#47932=DIRECTION('center_axis',(0.,-0.736346178773833,-0.676604984466694));
#47933=DIRECTION('ref_axis',(0.,-0.676604984466694,0.736346178773833));
#47934=DIRECTION('center_axis',(1.,0.,0.));
#47935=DIRECTION('ref_axis',(0.,-0.999780587432124,0.0209470044129973));
#47936=DIRECTION('',(-1.,0.,0.));
#47937=DIRECTION('center_axis',(1.,0.,0.));
#47938=DIRECTION('ref_axis',(0.,-0.676869218855487,0.736103294766409));
#47939=DIRECTION('',(1.,0.,0.));
#47940=DIRECTION('center_axis',(0.,0.,1.));
#47941=DIRECTION('ref_axis',(1.,0.,0.));
#47942=DIRECTION('center_axis',(0.,-0.736103294766404,-0.676869218855492));
#47943=DIRECTION('ref_axis',(0.,-0.676869218855492,0.736103294766404));
#47944=DIRECTION('center_axis',(1.,0.,0.));
#47945=DIRECTION('ref_axis',(0.,0.,-1.));
#47946=DIRECTION('center_axis',(-1.,0.,0.));
#47947=DIRECTION('ref_axis',(0.,-0.659345815100069,0.751839807478978));
#47948=DIRECTION('center_axis',(0.,0.766928997900544,0.641731962878012));
#47949=DIRECTION('ref_axis',(0.,-0.641731962878012,0.766928997900544));
#47950=DIRECTION('center_axis',(1.,0.,0.));
#47951=DIRECTION('ref_axis',(0.,1.,0.));
#47952=DIRECTION('center_axis',(1.,-3.46444446476948E-16,-3.06322230481445E-16));
#47953=DIRECTION('ref_axis',(0.,-0.662394497621569,0.749155210567656));
#47954=DIRECTION('center_axis',(1.,0.,0.));
#47955=DIRECTION('ref_axis',(0.,0.,-1.));
#47956=DIRECTION('center_axis',(-1.,0.,0.));
#47957=DIRECTION('ref_axis',(0.,-0.662394497621569,0.749155210567656));
#47958=DIRECTION('center_axis',(2.25734864122846E-14,-0.767159269002869,
-0.641456667268323));
#47959=DIRECTION('ref_axis',(0.,-0.641456667268323,0.767159269002869));
#47960=DIRECTION('center_axis',(1.,0.,0.));
#47961=DIRECTION('ref_axis',(0.,1.,0.));
#47962=DIRECTION('center_axis',(1.,0.,0.));
#47963=DIRECTION('ref_axis',(0.,0.,-1.));
#47964=DIRECTION('',(1.,0.,0.));
#47965=DIRECTION('center_axis',(0.,-0.866025403784438,0.5));
#47966=DIRECTION('ref_axis',(-0.707106781186555,-0.35355339059327,-0.612372435695788));
#47967=DIRECTION('center_axis',(1.28197512425574E-14,0.866025403784442,
-0.499999999999995));
#47968=DIRECTION('ref_axis',(0.,-0.499999999999995,-0.866025403784442));
#47969=DIRECTION('center_axis',(0.,0.258819045102499,-0.965925826289074));
#47970=DIRECTION('ref_axis',(8.17756488897782E-17,-0.965925826289074,-0.258819045102499));
#47971=DIRECTION('',(0.,-0.866025403784438,0.5));
#47972=DIRECTION('center_axis',(-0.706796314703091,0.612641189556821,-0.353708555707284));
#47973=DIRECTION('ref_axis',(0.,-0.500000000000001,-0.866025403784438));
#47974=DIRECTION('center_axis',(0.706790970016366,-0.612645814094484,0.353711225685349));
#47975=DIRECTION('ref_axis',(-0.707106781188921,-0.596890502257748,0.379106486770058));
#47976=DIRECTION('center_axis',(0.,0.,1.));
#47977=DIRECTION('ref_axis',(1.,0.,0.));
#47978=DIRECTION('center_axis',(0.,-0.536137535175637,-0.844130643547427));
#47979=DIRECTION('ref_axis',(0.,-0.844130643547427,0.536137535175637));
#47980=DIRECTION('center_axis',(1.,0.,0.));
#47981=DIRECTION('ref_axis',(0.,-0.971135373703073,-0.238529004405318));
#47982=DIRECTION('',(-1.,0.,0.));
#47983=DIRECTION('center_axis',(1.,0.,0.));
#47984=DIRECTION('ref_axis',(0.,-0.844323011360887,0.535834538347879));
#47985=DIRECTION('',(1.,0.,0.));
#47986=DIRECTION('center_axis',(0.,0.,1.));
#47987=DIRECTION('ref_axis',(1.,0.,0.));
#47988=DIRECTION('center_axis',(0.,-0.535834538347877,-0.844323011360888));
#47989=DIRECTION('ref_axis',(0.,-0.844323011360888,0.535834538347877));
#47990=DIRECTION('center_axis',(1.,0.,0.));
#47991=DIRECTION('ref_axis',(0.,0.,-1.));
#47992=DIRECTION('center_axis',(-1.,0.,0.));
#47993=DIRECTION('ref_axis',(0.,-0.831469612302545,0.555570233019602));
#47994=DIRECTION('center_axis',(0.,0.574704072158277,0.818361307397102));
#47995=DIRECTION('ref_axis',(0.,-0.818361307397102,0.574704072158277));
#47996=DIRECTION('center_axis',(1.,0.,0.));
#47997=DIRECTION('ref_axis',(0.,1.,0.));
#47998=DIRECTION('center_axis',(1.,6.40908585446359E-16,1.30193363367112E-16));
#47999=DIRECTION('ref_axis',(4.62446822220508E-16,-0.833719588677145,0.552188054430746));
#48000=DIRECTION('center_axis',(1.,0.,0.));
#48001=DIRECTION('ref_axis',(0.,0.,-1.));
#48002=DIRECTION('center_axis',(-1.,0.,0.));
#48003=DIRECTION('ref_axis',(0.,-0.833719588677145,0.552188054430746));
#48004=DIRECTION('center_axis',(-3.72249568383715E-14,-0.57499774870988,
-0.818154990804658));
#48005=DIRECTION('ref_axis',(0.,-0.818154990804658,0.57499774870988));
#48006=DIRECTION('center_axis',(1.,0.,0.));
#48007=DIRECTION('ref_axis',(0.,1.,0.));
#48008=DIRECTION('center_axis',(1.,0.,0.));
#48009=DIRECTION('ref_axis',(0.,0.,-1.));
#48010=DIRECTION('',(1.,0.,0.));
#48011=DIRECTION('center_axis',(0.,-0.38268343236509,0.923879532511287));
#48012=DIRECTION('ref_axis',(0.707106781186563,0.653281482438174,0.270598050073092));
#48013=DIRECTION('center_axis',(1.36761643863189E-14,0.382683432365089,
-0.923879532511287));
#48014=DIRECTION('ref_axis',(0.,0.923879532511287,0.382683432365089));
#48015=DIRECTION('center_axis',(0.,0.923879532511287,-0.382683432365089));
#48016=DIRECTION('ref_axis',(0.,0.382683432365089,0.923879532511287));
#48017=DIRECTION('',(0.,-0.38268343236509,0.923879532511287));
#48018=DIRECTION('center_axis',(0.706796314702672,0.270716808310081,-0.653568190184562));
#48019=DIRECTION('ref_axis',(0.,0.923879532511288,0.382683432365087));
#48020=DIRECTION('center_axis',(-0.706790970015944,-0.270718851822823,0.653573123660737));
#48021=DIRECTION('ref_axis',(0.707106781189343,-0.297953333789447,0.641267347429917));
#48022=DIRECTION('center_axis',(0.,0.,1.));
#48023=DIRECTION('ref_axis',(1.,0.,0.));
#48024=DIRECTION('center_axis',(0.,0.906888979845984,0.421369645600998));
#48025=DIRECTION('ref_axis',(0.,-0.421369645600998,0.906888979845984));
#48026=DIRECTION('center_axis',(-1.,0.,0.));
#48027=DIRECTION('ref_axis',(0.,0.363246958165943,0.931692893277173));
#48028=DIRECTION('',(1.,0.,0.));
#48029=DIRECTION('center_axis',(-1.,0.,0.));
#48030=DIRECTION('ref_axis',(0.,-0.421044131914909,0.90704015290395));
#48031=DIRECTION('',(-1.,0.,0.));
#48032=DIRECTION('center_axis',(0.0341251959389409,-0.995062857517424,0.0931953893247336));
#48033=DIRECTION('ref_axis',(0.342144487581495,0.0992467107226253,0.934391374119183));
#48034=DIRECTION('center_axis',(0.,0.907040152903952,0.421044131914905));
#48035=DIRECTION('ref_axis',(0.,-0.421044131914905,0.907040152903952));
#48036=DIRECTION('center_axis',(1.,0.,0.));
#48037=DIRECTION('ref_axis',(0.,0.,-1.));
#48038=DIRECTION('center_axis',(1.,0.,0.));
#48039=DIRECTION('ref_axis',(0.,-0.442288690219001,0.896872741532688));
#48040=DIRECTION('center_axis',(0.,-0.886374047158186,-0.462969813837163));
#48041=DIRECTION('ref_axis',(0.,-0.462969813837163,0.886374047158186));
#48042=DIRECTION('center_axis',(-1.,0.,0.));
#48043=DIRECTION('ref_axis',(0.,1.,0.));
#48044=DIRECTION('center_axis',(-1.,0.,0.));
#48045=DIRECTION('ref_axis',(0.,-0.438641765788069,0.898662006154886));
#48046=DIRECTION('center_axis',(0.706790970015259,-0.183094403348129,0.683317615876747));
#48047=DIRECTION('ref_axis',(0.,0.96592582628907,0.258819045102513));
#48048=DIRECTION('center_axis',(-0.706796314705246,0.183093021264868,-0.683312457872082));
#48049=DIRECTION('ref_axis',(-0.707106781186566,-0.211459960225227,0.674747867889569));
#48050=DIRECTION('center_axis',(0.,0.258819045102521,-0.965925826289068));
#48051=DIRECTION('ref_axis',(-0.707106781186564,0.683012701892201,0.183012701892222));
#48052=DIRECTION('center_axis',(-1.4298574565683E-14,0.258819045102515,
-0.96592582628907));
#48053=DIRECTION('ref_axis',(-1.,0.,1.48029736616691E-14));
#48054=DIRECTION('',(0.,0.258819045102521,-0.965925826289068));
#48055=DIRECTION('center_axis',(0.,0.866025403784435,-0.500000000000007));
#48056=DIRECTION('ref_axis',(0.,0.500000000000007,0.866025403784435));
#48057=DIRECTION('center_axis',(0.,0.,1.));
#48058=DIRECTION('ref_axis',(-0.802126387103182,0.597154300924641,0.));
#48059=DIRECTION('center_axis',(-0.077295046886547,-0.975418570101727,0.206359125864375));
#48060=DIRECTION('ref_axis',(-0.342144487592438,0.220360189464197,0.913443231136676));
#48061=DIRECTION('center_axis',(-1.,0.,0.));
#48062=DIRECTION('ref_axis',(0.,0.481749655761245,0.876308889133233));
#48063=DIRECTION('center_axis',(0.,0.923879532511287,0.38268343236509));
#48064=DIRECTION('ref_axis',(-1.,0.,0.));
#48065=DIRECTION('',(-1.,0.,0.));
#48066=DIRECTION('center_axis',(0.,0.923879532511287,0.38268343236509));
#48067=DIRECTION('ref_axis',(0.707106781186518,-0.270598050073113,0.653281482438214));
#48068=DIRECTION('',(0.706902428155814,0.270676229998409,-0.65347022547417));
#48069=DIRECTION('center_axis',(0.706790970014498,-0.0923371588686382,0.701370354233791));
#48070=DIRECTION('ref_axis',(0.,0.99144486137381,0.130526192220056));
#48071=DIRECTION('center_axis',(-0.706796314705261,0.0923364618639714,-0.701365059957726));
#48072=DIRECTION('ref_axis',(-0.707106781186553,-0.121578621047379,0.696576369757265));
#48073=DIRECTION('center_axis',(0.,0.130526192220051,-0.99144486137381));
#48074=DIRECTION('ref_axis',(-0.707106781186562,0.701057384649965,0.0922959556412482));
#48075=DIRECTION('center_axis',(0.,0.130526192220056,-0.99144486137381));
#48076=DIRECTION('ref_axis',(-1.,0.,0.));
#48077=DIRECTION('',(0.,0.130526192220051,-0.991444861373811));
#48078=DIRECTION('center_axis',(0.,0.793353340291241,-0.608761429008714));
#48079=DIRECTION('ref_axis',(0.,0.608761429008713,0.793353340291241));
#48080=DIRECTION('center_axis',(0.,0.,1.));
#48081=DIRECTION('ref_axis',(-0.764784300456388,0.644286406635615,0.));
#48082=DIRECTION('center_axis',(-0.122754826320915,-0.941252632831819,0.314602501264835));
#48083=DIRECTION('ref_axis',(-0.342144487592386,0.337703244265101,0.876865821219512));
#48084=DIRECTION('center_axis',(-1.,0.,0.));
#48085=DIRECTION('ref_axis',(0.,0.592009483180228,0.805930996937504));
#48086=DIRECTION('center_axis',(0.,0.965925826289068,0.258819045102521));
#48087=DIRECTION('ref_axis',(-1.,0.,0.));
#48088=DIRECTION('',(-1.,0.,0.));
#48089=DIRECTION('center_axis',(0.,0.965925826289068,0.258819045102521));
#48090=DIRECTION('ref_axis',(0.707106781186523,-0.183012701892228,0.683012701892242));
#48091=DIRECTION('',(0.706902428155819,0.183065577067635,-0.683210034733317));
#48092=DIRECTION('center_axis',(0.,6.12323399573677E-17,1.));
#48093=DIRECTION('ref_axis',(-0.707106781186563,-0.707106781186532,0.));
#48094=DIRECTION('center_axis',(0.,0.,-1.));
#48095=DIRECTION('ref_axis',(0.,-1.,0.));
#48096=DIRECTION('center_axis',(0.,-0.707106781186546,-0.707106781186549));
#48097=DIRECTION('ref_axis',(-4.08878244448901E-17,-0.707106781186549,0.707106781186546));
#48098=DIRECTION('',(0.,6.12323399573677E-17,1.));
#48099=DIRECTION('center_axis',(-0.706796314700322,0.,-0.707417111417333));
#48100=DIRECTION('ref_axis',(0.,-1.,0.));
#48101=DIRECTION('center_axis',(0.706790970013424,0.,0.707422451373635));
#48102=DIRECTION('ref_axis',(-0.707106781191861,0.0298705971533412,0.706475581614954));
#48103=DIRECTION('center_axis',(0.,0.,1.));
#48104=DIRECTION('ref_axis',(-0.721874560494001,-0.692023929435676,0.));
#48105=DIRECTION('center_axis',(0.,-0.999107349012797,0.0422434036107609));
#48106=DIRECTION('ref_axis',(0.,0.0422434036107609,0.999107349012797));
#48107=DIRECTION('center_axis',(1.,0.,0.));
#48108=DIRECTION('ref_axis',(0.,-0.692139864205962,0.721763401937888));
#48109=DIRECTION('',(-1.,0.,0.));
#48110=DIRECTION('center_axis',(1.,0.,0.));
#48111=DIRECTION('ref_axis',(0.,0.0418848167539273,0.999122446012244));
#48112=DIRECTION('',(1.,0.,0.));
#48113=DIRECTION('center_axis',(0.172056328312398,-0.893396984377419,-0.415016202325873));
#48114=DIRECTION('ref_axis',(-0.34214448757159,-0.449268102924446,0.825284993998464));
#48115=DIRECTION('center_axis',(0.,-0.999122446012245,0.0418848167539203));
#48116=DIRECTION('ref_axis',(0.,0.0418848167539203,0.999122446012244));
#48117=DIRECTION('center_axis',(1.,0.,0.));
#48118=DIRECTION('ref_axis',(0.,0.,-1.));
#48119=DIRECTION('center_axis',(-1.,0.,0.));
#48120=DIRECTION('ref_axis',(0.,0.0654031292301431,0.997858923238603));
#48121=DIRECTION('center_axis',(0.,0.996073717759275,-0.0885276724488819));
#48122=DIRECTION('ref_axis',(0.,0.0885276724488819,0.996073717759275));
#48123=DIRECTION('center_axis',(1.,0.,0.));
#48124=DIRECTION('ref_axis',(0.,1.,0.));
#48125=DIRECTION('center_axis',(1.,0.,0.));
#48126=DIRECTION('ref_axis',(0.,0.0613490884647571,0.998116370642493));
#48127=DIRECTION('center_axis',(1.,0.,0.));
#48128=DIRECTION('ref_axis',(0.,0.,-1.));
#48129=DIRECTION('center_axis',(-1.,0.,0.));
#48130=DIRECTION('ref_axis',(0.,0.0613490884647572,0.998116370642494));
#48131=DIRECTION('center_axis',(1.17765452698042E-14,-0.996041880624797,
0.0888851620992974));
#48132=DIRECTION('ref_axis',(0.,0.0888851620992974,0.996041880624796));
#48133=DIRECTION('center_axis',(1.,0.,0.));
#48134=DIRECTION('ref_axis',(0.,1.,0.));
#48135=DIRECTION('center_axis',(1.,0.,0.));
#48136=DIRECTION('ref_axis',(0.,0.,-1.));
#48137=DIRECTION('',(1.,0.,0.));
#48138=DIRECTION('center_axis',(0.706790970014367,0.0923371588686554,0.70137035423392));
#48139=DIRECTION('ref_axis',(0.,0.99144486137381,-0.130526192220056));
#48140=DIRECTION('center_axis',(-0.70679631470526,-0.0923364618639819,-0.701365059957726));
#48141=DIRECTION('ref_axis',(-0.707106781186553,0.0628513008672796,0.70430796813559));
#48142=DIRECTION('center_axis',(0.,-0.130526192220052,-0.99144486137381));
#48143=DIRECTION('ref_axis',(-0.707106781186562,0.701057384649962,-0.0922959556412691));
#48144=DIRECTION('center_axis',(2.41521973198931E-16,-0.130526192220056,
-0.99144486137381));
#48145=DIRECTION('ref_axis',(-1.,-1.85037170770863E-15,0.));
#48146=DIRECTION('',(0.,-0.130526192220052,-0.99144486137381));
#48147=DIRECTION('center_axis',(0.,0.608761429008712,-0.793353340291242));
#48148=DIRECTION('ref_axis',(-8.17756488897809E-17,0.793353340291242,0.608761429008712));
#48149=DIRECTION('center_axis',(0.,0.,1.));
#48150=DIRECTION('ref_axis',(1.,0.,0.));
#48151=DIRECTION('center_axis',(0.,0.,1.));
#48152=DIRECTION('ref_axis',(1.,0.,0.));
#48153=DIRECTION('center_axis',(-1.,0.,0.));
#48154=DIRECTION('ref_axis',(0.,0.780427540257714,0.625246235020487));
#48155=DIRECTION('center_axis',(0.,1.,-6.12323399573677E-17));
#48156=DIRECTION('ref_axis',(-1.,0.,0.));
#48157=DIRECTION('',(-1.,0.,0.));
#48158=DIRECTION('center_axis',(0.,1.,-6.12323399573677E-17));
#48159=DIRECTION('ref_axis',(0.707106781186527,0.,0.707106781186568));
#48160=DIRECTION('',(0.706902428155817,0.,-0.707311075176552));
#48161=DIRECTION('center_axis',(-1.,0.,0.));
#48162=DIRECTION('ref_axis',(0.,0.592009483180227,0.805930996937505));
#48163=DIRECTION('',(-1.,0.,0.));
#48164=DIRECTION('center_axis',(0.,-0.99144486137381,-0.130526192220051));
#48165=DIRECTION('ref_axis',(1.,0.,0.));
#48166=DIRECTION('',(-0.706902428155813,-0.0923226213578649,0.701259930876582));
#48167=DIRECTION('center_axis',(0.,-0.99144486137381,-0.130526192220051));
#48168=DIRECTION('ref_axis',(0.70710678118652,-0.0922959556412642,0.701057384650004));
#48169=DIRECTION('',(1.,0.,0.));
#48170=DIRECTION('center_axis',(-1.,0.,0.));
#48171=DIRECTION('ref_axis',(0.,0.481749655761243,0.876308889133235));
#48172=DIRECTION('',(-1.,0.,0.));
#48173=DIRECTION('center_axis',(0.,-0.965925826289068,-0.258819045102521));
#48174=DIRECTION('ref_axis',(1.,0.,0.));
#48175=DIRECTION('',(-0.706902428155819,-0.183065577067637,0.683210034733317));
#48176=DIRECTION('center_axis',(0.,-0.965925826289068,-0.258819045102521));
#48177=DIRECTION('ref_axis',(0.707106781186523,-0.183012701892228,0.683012701892242));
#48178=DIRECTION('',(1.,0.,0.));
#48179=DIRECTION('center_axis',(-0.706790970016278,-0.353711225685393,0.61264581409456));
#48180=DIRECTION('ref_axis',(0.,-0.866025403784438,-0.500000000000001));
#48181=DIRECTION('center_axis',(0.706796314705255,0.353708555706252,-0.61264118955492));
#48182=DIRECTION('ref_axis',(0.707106781186558,-0.327594021151197,0.626643564800577));
#48183=DIRECTION('center_axis',(1.,0.,0.));
#48184=DIRECTION('ref_axis',(0.,0.,-1.));
#48185=DIRECTION('center_axis',(1.,0.,0.));
#48186=DIRECTION('ref_axis',(0.,-0.438641765788069,0.898662006154886));
#48187=DIRECTION('center_axis',(4.06322755421133E-14,0.886207828114817,
0.463287907664357));
#48188=DIRECTION('ref_axis',(0.,-0.463287907664357,0.886207828114817));
#48189=DIRECTION('center_axis',(0.,0.,1.));
#48190=DIRECTION('ref_axis',(1.,0.,0.));
#48191=DIRECTION('center_axis',(1.,0.,0.));
#48192=DIRECTION('ref_axis',(0.,-0.960292406343216,0.278995509497118));
#48193=DIRECTION('center_axis',(0.,0.5,-0.866025403784439));
#48194=DIRECTION('ref_axis',(0.707106781186562,-0.612372435695782,-0.353553390593266));
#48195=DIRECTION('center_axis',(-2.93402459005303E-14,0.499999999999997,
-0.866025403784441));
#48196=DIRECTION('ref_axis',(1.,7.4014868308341E-15,-2.96059473233364E-14));
#48197=DIRECTION('',(0.,0.5,-0.866025403784439));
#48198=DIRECTION('center_axis',(0.,-0.258819045102534,-0.965925826289065));
#48199=DIRECTION('ref_axis',(-8.17756488897789E-17,-0.965925826289065,0.258819045102534));
#48200=DIRECTION('center_axis',(0.,0.,1.));
#48201=DIRECTION('ref_axis',(1.,0.,0.));
#48202=DIRECTION('center_axis',(0.,-0.923879532511287,-0.38268343236509));
#48203=DIRECTION('ref_axis',(1.,0.,0.));
#48204=DIRECTION('',(1.,0.,0.));
#48205=DIRECTION('center_axis',(0.,-0.923879532511287,-0.38268343236509));
#48206=DIRECTION('ref_axis',(-0.70710678118656,-0.270598050073094,0.653281482438177));
#48207=DIRECTION('',(-0.70690242815582,0.270676229998411,-0.653470225474163));
#48208=DIRECTION('center_axis',(0.706790970016497,-0.561235964791851,0.430651502409198));
#48209=DIRECTION('ref_axis',(0.,0.608761429008721,0.793353340291235));
#48210=DIRECTION('center_axis',(-0.70679631470526,0.561231728318199,-0.430648251648641));
#48211=DIRECTION('ref_axis',(-0.707106781186554,-0.578522942059575,0.406584807279766));
#48212=DIRECTION('center_axis',(0.,0.793353340291235,-0.608761429008721));
#48213=DIRECTION('ref_axis',(-0.707106781186566,0.430459334576868,0.560985526796916));
#48214=DIRECTION('center_axis',(2.07554680005844E-14,0.793353340291236,
-0.608761429008719));
#48215=DIRECTION('ref_axis',(-1.,1.48029736616691E-14,-1.48029736616691E-14));
#48216=DIRECTION('',(0.,0.793353340291235,-0.608761429008721));
#48217=DIRECTION('center_axis',(0.,0.991444861373808,0.130526192220069));
#48218=DIRECTION('ref_axis',(1.22663473334668E-16,-0.130526192220069,0.991444861373808));
#48219=DIRECTION('center_axis',(0.,0.,1.));
#48220=DIRECTION('ref_axis',(-0.903692699960903,0.428181625058075,0.));
#48221=DIRECTION('center_axis',(0.141097613864597,-0.924473827539715,-0.354174541089258));
#48222=DIRECTION('ref_axis',(-0.342144487592388,-0.381245514326488,0.858830022423572));
#48223=DIRECTION('center_axis',(-1.,0.,0.));
#48224=DIRECTION('ref_axis',(0.,-0.151265353019495,0.988493193186421));
#48225=DIRECTION('center_axis',(0.,0.5,0.866025403784438));
#48226=DIRECTION('ref_axis',(-1.,0.,0.));
#48227=DIRECTION('',(-1.,0.,0.));
#48228=DIRECTION('center_axis',(0.,0.5,0.866025403784438));
#48229=DIRECTION('ref_axis',(0.707106781186515,-0.612372435695829,0.353553390593278));
#48230=DIRECTION('',(0.706902428155818,0.612549359480981,-0.35365553758827));
#48231=DIRECTION('center_axis',(0.,-0.707106781186547,0.707106781186548));
#48232=DIRECTION('ref_axis',(0.707106781186567,0.499999999999986,0.499999999999986));
#48233=DIRECTION('center_axis',(-1.04672830578914E-14,0.707106781186548,
-0.707106781186548));
#48234=DIRECTION('ref_axis',(0.,0.707106781186547,0.707106781186547));
#48235=DIRECTION('center_axis',(0.,1.,-1.04672830578919E-14));
#48236=DIRECTION('ref_axis',(-2.04439122224452E-16,1.04950770296598E-14,
1.));
#48237=DIRECTION('',(0.,-0.707106781186547,0.707106781186548));
#48238=DIRECTION('center_axis',(0.706796314703398,0.500219436608423,-0.500219436608423));
#48239=DIRECTION('ref_axis',(0.,0.707106781186547,0.707106781186547));
#48240=DIRECTION('center_axis',(-0.706790970016721,-0.500223212527579,0.500223212527579));
#48241=DIRECTION('ref_axis',(0.707106781188566,-0.5206753763103,0.478431972699645));
#48242=DIRECTION('center_axis',(0.,0.,1.));
#48243=DIRECTION('ref_axis',(1.,0.,0.));
#48244=DIRECTION('center_axis',(0.,0.676604984466694,0.736346178773832));
#48245=DIRECTION('ref_axis',(0.,-0.736346178773832,0.676604984466694));
#48246=DIRECTION('center_axis',(-1.,0.,0.));
#48247=DIRECTION('ref_axis',(0.,-0.0209470044129973,0.999780587432124));
#48248=DIRECTION('',(1.,0.,0.));
#48249=DIRECTION('center_axis',(-1.,0.,0.));
#48250=DIRECTION('ref_axis',(0.,-0.73610329476641,0.676869218855486));
#48251=DIRECTION('',(-1.,0.,0.));
#48252=DIRECTION('center_axis',(-0.0943675359584495,-0.964005004559978,
-0.248574172713998));
#48253=DIRECTION('ref_axis',(0.342144487584567,-0.265884093513166,0.901245137813334));
#48254=DIRECTION('center_axis',(0.,0.676869218855493,0.736103294766404));
#48255=DIRECTION('ref_axis',(0.,-0.736103294766404,0.676869218855492));
#48256=DIRECTION('center_axis',(1.,0.,0.));
#48257=DIRECTION('ref_axis',(0.,0.,-1.));
#48258=DIRECTION('center_axis',(1.,0.,0.));
#48259=DIRECTION('ref_axis',(0.,-0.751839807478977,0.659345815100069));
#48260=DIRECTION('center_axis',(0.,-0.641731962878011,-0.766928997900546));
#48261=DIRECTION('ref_axis',(0.,-0.766928997900546,0.64173196287801));
#48262=DIRECTION('center_axis',(-1.,0.,0.));
#48263=DIRECTION('ref_axis',(0.,1.,0.));
#48264=DIRECTION('center_axis',(-1.,0.,0.));
#48265=DIRECTION('ref_axis',(0.,-0.749155210567656,0.662394497621569));
#48266=DIRECTION('center_axis',(0.706790970016624,-0.430651502409115,0.561235964791754));
#48267=DIRECTION('ref_axis',(0.,0.79335334029124,0.608761429008714));
#48268=DIRECTION('center_axis',(-0.706796314705265,0.430648251648656,-0.561231728318181));
#48269=DIRECTION('ref_axis',(-0.70710678118655,-0.453578359262736,0.542463521362055));
#48270=DIRECTION('center_axis',(0.,0.60876142900872,-0.793353340291235));
#48271=DIRECTION('ref_axis',(-0.707106781186568,0.560985526796914,0.430459334576867));
#48272=DIRECTION('center_axis',(-1.17439886007282E-14,0.608761429008728,
-0.793353340291229));
#48273=DIRECTION('ref_axis',(-1.,0.,1.48029736616691E-14));
#48274=DIRECTION('',(0.,0.60876142900872,-0.793353340291235));
#48275=DIRECTION('center_axis',(0.,0.991444861373812,-0.130526192220041));
#48276=DIRECTION('ref_axis',(0.,0.130526192220041,0.991444861373812));
#48277=DIRECTION('center_axis',(0.,0.,1.));
#48278=DIRECTION('ref_axis',(-0.877521329523649,0.479537606691119,0.));
#48279=DIRECTION('center_axis',(0.0504847333736789,-0.989288526783089,-0.136965333101244));
#48280=DIRECTION('ref_axis',(-0.342144487592341,-0.145973322135748,0.92823969901897));
#48281=DIRECTION('center_axis',(-1.,0.,0.));
#48282=DIRECTION('ref_axis',(0.,0.109729753246575,0.993961458635316));
#48283=DIRECTION('center_axis',(0.,0.707106781186548,0.707106781186547));
#48284=DIRECTION('ref_axis',(-1.,0.,0.));
#48285=DIRECTION('',(-1.,0.,0.));
#48286=DIRECTION('center_axis',(0.,0.707106781186548,0.707106781186547));
#48287=DIRECTION('ref_axis',(0.707106781186517,-0.500000000000016,0.500000000000026));
#48288=DIRECTION('',(0.706902428155819,0.500144457665683,-0.500144457665689));
#48289=DIRECTION('center_axis',(0.,-0.60876142900872,0.793353340291235));
#48290=DIRECTION('ref_axis',(-0.707106781186558,-0.560985526796922,-0.430459334576874));
#48291=DIRECTION('center_axis',(-1.17439886007283E-14,0.608761429008723,
-0.793353340291233));
#48292=DIRECTION('ref_axis',(0.,-0.793353340291233,-0.608761429008723));
#48293=DIRECTION('center_axis',(0.,-0.130526192220051,-0.991444861373811));
#48294=DIRECTION('ref_axis',(-1.2266347333467E-16,-0.991444861373811,0.130526192220051));
#48295=DIRECTION('',(0.,-0.60876142900872,0.793353340291235));
#48296=DIRECTION('center_axis',(-0.7067963147033,0.430648251649821,-0.561231728319761));
#48297=DIRECTION('ref_axis',(0.,-0.79335334029124,-0.608761429008714));
#48298=DIRECTION('center_axis',(0.706790970016666,-0.43065150240909,0.561235964791721));
#48299=DIRECTION('ref_axis',(-0.70710678118862,-0.406377146597434,0.578668829919494));
#48300=DIRECTION('center_axis',(0.,0.,1.));
#48301=DIRECTION('ref_axis',(1.,0.,0.));
#48302=DIRECTION('center_axis',(0.,-0.818361307397102,-0.574704072158276));
#48303=DIRECTION('ref_axis',(0.,-0.574704072158276,0.818361307397102));
#48304=DIRECTION('center_axis',(1.,0.,0.));
#48305=DIRECTION('ref_axis',(0.,-0.988493193186426,0.151265353019465));
#48306=DIRECTION('',(-1.,0.,0.));
#48307=DIRECTION('center_axis',(1.,0.,0.));
#48308=DIRECTION('ref_axis',(0.,-0.574997748709897,0.818154990804646));
#48309=DIRECTION('',(1.,0.,0.));
#48310=DIRECTION('center_axis',(0.,0.,1.));
#48311=DIRECTION('ref_axis',(1.,0.,0.));
#48312=DIRECTION('center_axis',(0.,-0.818154990804651,-0.57499774870989));
#48313=DIRECTION('ref_axis',(0.,-0.57499774870989,0.818154990804651));
#48314=DIRECTION('center_axis',(1.,0.,0.));
#48315=DIRECTION('ref_axis',(0.,0.,-1.));
#48316=DIRECTION('center_axis',(-1.,0.,0.));
#48317=DIRECTION('ref_axis',(0.,-0.555570233019602,0.831469612302545));
#48318=DIRECTION('center_axis',(0.,0.844130643547427,0.536137535175636));
#48319=DIRECTION('ref_axis',(0.,-0.536137535175636,0.844130643547427));
#48320=DIRECTION('center_axis',(1.,0.,0.));
#48321=DIRECTION('ref_axis',(0.,1.,0.));
#48322=DIRECTION('center_axis',(1.,0.,0.));
#48323=DIRECTION('ref_axis',(0.,-0.558943243851984,0.829205915410775));
#48324=DIRECTION('center_axis',(1.,0.,0.));
#48325=DIRECTION('ref_axis',(0.,0.,-1.));
#48326=DIRECTION('center_axis',(-1.,0.,0.));
#48327=DIRECTION('ref_axis',(0.,-0.558943243851984,0.829205915410775));
#48328=DIRECTION('center_axis',(4.25914837967648E-15,-0.844323011360896,
-0.535834538347864));
#48329=DIRECTION('ref_axis',(0.,-0.535834538347864,0.844323011360896));
#48330=DIRECTION('center_axis',(1.,0.,0.));
#48331=DIRECTION('ref_axis',(0.,1.,0.));
#48332=DIRECTION('center_axis',(1.,0.,0.));
#48333=DIRECTION('ref_axis',(0.,0.,-1.));
#48334=DIRECTION('',(1.,0.,0.));
#48335=DIRECTION('center_axis',(0.706790970016345,-0.35371122568536,0.612645814094502));
#48336=DIRECTION('ref_axis',(0.,0.866025403784438,0.500000000000001));
#48337=DIRECTION('center_axis',(-0.706796314705253,0.353708555706156,-0.612641189554978));
#48338=DIRECTION('ref_axis',(-0.70710678118656,-0.378892235659731,0.597026526845125));
#48339=DIRECTION('center_axis',(0.,0.5,-0.866025403784439));
#48340=DIRECTION('ref_axis',(-0.707106781186565,0.612372435695779,0.353553390593267));
#48341=DIRECTION('center_axis',(1.28197512425574E-14,0.499999999999997,
-0.866025403784441));
#48342=DIRECTION('ref_axis',(-1.,0.,-1.48029736616691E-14));
#48343=DIRECTION('',(0.,0.5,-0.866025403784439));
#48344=DIRECTION('center_axis',(0.,0.965925826289075,-0.258819045102497));
#48345=DIRECTION('ref_axis',(4.0887824444889E-17,0.258819045102497,0.965925826289075));
#48346=DIRECTION('center_axis',(0.,0.,1.));
#48347=DIRECTION('ref_axis',(-0.858053385943022,0.513560499719085,0.));
#48348=DIRECTION('center_axis',(0.00806484247865072,-0.999722309028825,
-0.022141886682713));
#48349=DIRECTION('ref_axis',(-0.342144487592434,-0.023564906748703,0.939351821619587));
#48350=DIRECTION('center_axis',(-1.,0.,0.));
#48351=DIRECTION('ref_axis',(0.,0.238529004405336,0.971135373703069));
#48352=DIRECTION('center_axis',(0.,0.793353340291235,0.60876142900872));
#48353=DIRECTION('ref_axis',(-1.,0.,0.));
#48354=DIRECTION('',(-1.,0.,0.));
#48355=DIRECTION('center_axis',(0.,0.793353340291235,0.60876142900872));
#48356=DIRECTION('ref_axis',(0.707106781186524,-0.430459334576899,0.560985526796945));
#48357=DIRECTION('',(0.706902428155818,0.430583700878177,-0.561147604116297));
#48358=DIRECTION('center_axis',(-1.,0.,0.));
#48359=DIRECTION('ref_axis',(0.,0.10972975324658,0.993961458635316));
#48360=DIRECTION('',(-1.,0.,0.));
#48361=DIRECTION('center_axis',(0.,-0.793353340291235,-0.60876142900872));
#48362=DIRECTION('ref_axis',(1.,0.,0.));
#48363=DIRECTION('',(-0.706902428155816,-0.430583700878176,0.561147604116301));
#48364=DIRECTION('center_axis',(0.,-0.793353340291235,-0.60876142900872));
#48365=DIRECTION('ref_axis',(0.707106781186524,-0.430459334576899,0.560985526796945));
#48366=DIRECTION('',(1.,0.,0.));
#48367=DIRECTION('center_axis',(-0.706790970016552,-0.561235964791808,0.430651502409164));
#48368=DIRECTION('ref_axis',(0.,-0.608761429008721,-0.793353340291235));
#48369=DIRECTION('center_axis',(0.706796314705253,0.561231728318191,-0.430648251648662));
#48370=DIRECTION('ref_axis',(0.707106781186562,-0.542463521362034,0.453578359262743));
#48371=DIRECTION('center_axis',(1.,0.,0.));
#48372=DIRECTION('ref_axis',(0.,0.,-1.));
#48373=DIRECTION('center_axis',(1.,0.,0.));
#48374=DIRECTION('ref_axis',(0.,-0.749155210567656,0.662394497621569));
#48375=DIRECTION('center_axis',(2.02735462872594E-14,0.641456667268323,
0.767159269002869));
#48376=DIRECTION('ref_axis',(0.,-0.767159269002869,0.641456667268323));
#48377=DIRECTION('center_axis',(0.,0.,1.));
#48378=DIRECTION('ref_axis',(1.,0.,0.));
#48379=DIRECTION('center_axis',(1.,0.,0.));
#48380=DIRECTION('ref_axis',(0.,-0.993961458635316,-0.109729753246575));
#48381=DIRECTION('center_axis',(0.,0.793353340291235,-0.608761429008721));
#48382=DIRECTION('ref_axis',(0.707106781186558,-0.430459334576874,-0.560985526796922));
#48383=DIRECTION('center_axis',(-2.07554680005832E-14,0.79335334029124,
-0.608761429008714));
#48384=DIRECTION('ref_axis',(1.,1.48029736616682E-14,-1.48029736616682E-14));
#48385=DIRECTION('',(0.,0.793353340291235,-0.608761429008721));
#48386=DIRECTION('center_axis',(0.,0.130526192220037,-0.991444861373812));
#48387=DIRECTION('ref_axis',(-2.45326946669336E-16,-0.991444861373812,-0.130526192220037));
#48388=DIRECTION('center_axis',(0.,0.,1.));
#48389=DIRECTION('ref_axis',(1.,0.,0.));
#48390=DIRECTION('center_axis',(0.,-0.707106781186548,-0.707106781186547));
#48391=DIRECTION('ref_axis',(1.,0.,0.));
#48392=DIRECTION('',(1.,0.,0.));
#48393=DIRECTION('center_axis',(0.,-0.707106781186548,-0.707106781186547));
#48394=DIRECTION('ref_axis',(-0.707106781186559,-0.499999999999986,0.499999999999997));
#48395=DIRECTION('',(-0.706902428155818,0.500144457665681,-0.500144457665694));
#48396=DIRECTION('center_axis',(-1.,0.,0.));
#48397=DIRECTION('ref_axis',(0.,-0.151265353019489,0.988493193186422));
#48398=DIRECTION('',(-1.,0.,0.));
#48399=DIRECTION('center_axis',(0.,-0.608761429008721,-0.793353340291235));
#48400=DIRECTION('ref_axis',(1.,0.,0.));
#48401=DIRECTION('',(-0.706902428155818,-0.561147604116303,0.43058370087817));
#48402=DIRECTION('center_axis',(0.,-0.608761429008721,-0.793353340291235));
#48403=DIRECTION('ref_axis',(0.707106781186509,-0.560985526796955,0.430459334576911));
#48404=DIRECTION('',(1.,0.,0.));
#48405=DIRECTION('center_axis',(0.,-0.965925826289068,-0.25881904510252));
#48406=DIRECTION('ref_axis',(-0.707106781186562,0.183012701892215,-0.683012701892206));
#48407=DIRECTION('center_axis',(0.,0.96592582628907,0.258819045102515));
#48408=DIRECTION('ref_axis',(0.,0.258819045102515,-0.96592582628907));
#48409=DIRECTION('center_axis',(0.,0.86602540378444,-0.499999999999997));
#48410=DIRECTION('ref_axis',(4.08878244448901E-17,-0.499999999999997,-0.86602540378444));
#48411=DIRECTION('',(0.,-0.965925826289068,-0.25881904510252));
#48412=DIRECTION('center_axis',(-0.706796314702185,0.683312457875017,0.183093021265731));
#48413=DIRECTION('ref_axis',(0.,0.258819045102514,-0.96592582628907));
#48414=DIRECTION('center_axis',(0.706790970015486,-0.683317615876528,-0.183094403348071));
#48415=DIRECTION('ref_axis',(-0.7071067811898,-0.690134089358358,-0.153996554185185));
#48416=DIRECTION('center_axis',(0.,0.,1.));
#48417=DIRECTION('ref_axis',(-0.921538338698512,0.388287381083633,0.));
#48418=DIRECTION('center_axis',(0.,0.217784015488416,-0.975996989031084));
#48419=DIRECTION('ref_axis',(0.,-0.975996989031084,-0.217784015488416));
#48420=DIRECTION('center_axis',(1.,0.,0.));
#48421=DIRECTION('ref_axis',(0.,-0.518030931670892,-0.855361884720255));
#48422=DIRECTION('',(-1.,0.,0.));
#48423=DIRECTION('center_axis',(1.,0.,0.));
#48424=DIRECTION('ref_axis',(0.,-0.975918762504877,-0.218134291185381));
#48425=DIRECTION('',(1.,0.,0.));
#48426=DIRECTION('center_axis',(-0.93964735386155,0.247923894850261,0.235789297346728));
#48427=DIRECTION('ref_axis',(-0.342144487579453,-0.680884948353929,-0.647559137626874));
#48428=DIRECTION('center_axis',(0.,0.218134291185385,-0.975918762504877));
#48429=DIRECTION('ref_axis',(0.,-0.975918762504877,-0.218134291185385));
#48430=DIRECTION('center_axis',(1.,0.,0.));
#48431=DIRECTION('ref_axis',(0.,0.,-1.));
#48432=DIRECTION('center_axis',(-1.,0.,0.));
#48433=DIRECTION('ref_axis',(0.,-0.980785280403231,-0.195090322016127));
#48434=DIRECTION('center_axis',(0.,-0.172291683322539,0.98504597651982));
#48435=DIRECTION('ref_axis',(0.,-0.98504597651982,-0.172291683322539));
#48436=DIRECTION('center_axis',(1.,0.,0.));
#48437=DIRECTION('ref_axis',(0.,1.,0.));
#48438=DIRECTION('center_axis',(1.,0.,0.));
#48439=DIRECTION('ref_axis',(0.,-0.979984692539855,-0.199072856983481));
#48440=DIRECTION('center_axis',(1.,0.,0.));
#48441=DIRECTION('ref_axis',(0.,0.,-1.));
#48442=DIRECTION('center_axis',(-1.,0.,0.));
#48443=DIRECTION('ref_axis',(0.,-0.979984692539855,-0.199072856983481));
#48444=DIRECTION('center_axis',(-2.88770260142032E-14,0.171938134779826,
-0.985107749339347));
#48445=DIRECTION('ref_axis',(0.,-0.985107749339347,-0.171938134779826));
#48446=DIRECTION('center_axis',(1.,0.,0.));
#48447=DIRECTION('ref_axis',(0.,1.,0.));
#48448=DIRECTION('center_axis',(1.,0.,0.));
#48449=DIRECTION('ref_axis',(0.,0.,-1.));
#48450=DIRECTION('',(1.,0.,0.));
#48451=DIRECTION('center_axis',(0.,-0.923879532511287,-0.382683432365089));
#48452=DIRECTION('ref_axis',(-0.707106781186561,0.270598050073094,-0.653281482438176));
#48453=DIRECTION('center_axis',(2.83242638502877E-15,0.923879532511287,
0.382683432365089));
#48454=DIRECTION('ref_axis',(0.,0.382683432365089,-0.923879532511287));
#48455=DIRECTION('center_axis',(0.,0.923879532511287,-0.382683432365089));
#48456=DIRECTION('ref_axis',(4.088782444489E-17,-0.382683432365089,-0.923879532511287));
#48457=DIRECTION('',(0.,-0.923879532511287,-0.382683432365089));
#48458=DIRECTION('center_axis',(-0.706796314702746,0.653568190184494,0.270716808310053));
#48459=DIRECTION('ref_axis',(0.,0.382683432365087,-0.923879532511288));
#48460=DIRECTION('center_axis',(0.706790970016102,-0.653573123660592,-0.270718851822762));
#48461=DIRECTION('ref_axis',(-0.707106781189185,-0.664129312721009,-0.242759667121599));
#48462=DIRECTION('center_axis',(0.,0.,1.));
#48463=DIRECTION('ref_axis',(-0.917771314419967,0.397109323018041,0.));
#48464=DIRECTION('center_axis',(0.,0.343314013641807,-0.939220681223084));
#48465=DIRECTION('ref_axis',(0.,-0.939220681223084,-0.343314013641807));
#48466=DIRECTION('center_axis',(1.,0.,0.));
#48467=DIRECTION('ref_axis',(0.,-0.401951975455108,-0.915660750184115));
#48468=DIRECTION('',(-1.,0.,0.));
#48469=DIRECTION('center_axis',(1.,0.,0.));
#48470=DIRECTION('ref_axis',(0.,-0.939097403782702,-0.343651082071028));
#48471=DIRECTION('',(1.,0.,0.));
#48472=DIRECTION('center_axis',(0.250366849757596,-0.807010963742338,0.534836185146555));
#48473=DIRECTION('ref_axis',(-0.342144487581869,-0.590536454759292,-0.730892499084282));
#48474=DIRECTION('center_axis',(0.,0.343651082071034,-0.9390974037827));
#48475=DIRECTION('ref_axis',(0.,-0.9390974037827,-0.343651082071034));
#48476=DIRECTION('center_axis',(1.,0.,0.));
#48477=DIRECTION('ref_axis',(0.,0.,-1.));
#48478=DIRECTION('center_axis',(-1.,0.,0.));
#48479=DIRECTION('ref_axis',(0.,-0.946930129495106,-0.321439465303161));
#48480=DIRECTION('center_axis',(0.,-0.299392004564389,0.954130194262249));
#48481=DIRECTION('ref_axis',(0.,-0.954130194262249,-0.299392004564389));
#48482=DIRECTION('center_axis',(1.,0.,0.));
#48483=DIRECTION('ref_axis',(0.,1.,0.));
#48484=DIRECTION('center_axis',(1.,0.,0.));
#48485=DIRECTION('ref_axis',(0.,-0.945616565647212,-0.325283431446441));
#48486=DIRECTION('center_axis',(1.,0.,0.));
#48487=DIRECTION('ref_axis',(0.,0.,-1.));
#48488=DIRECTION('center_axis',(-1.,0.,0.));
#48489=DIRECTION('ref_axis',(0.,-0.945616565647212,-0.325283431446441));
#48490=DIRECTION('center_axis',(-2.23179375095024E-14,0.299049543649391,
-0.954237585951785));
#48491=DIRECTION('ref_axis',(0.,-0.954237585951785,-0.299049543649391));
#48492=DIRECTION('center_axis',(1.,0.,0.));
#48493=DIRECTION('ref_axis',(0.,1.,0.));
#48494=DIRECTION('center_axis',(1.,0.,0.));
#48495=DIRECTION('ref_axis',(0.,0.,-1.));
#48496=DIRECTION('',(1.,0.,0.));
#48497=DIRECTION('center_axis',(0.,-0.923879532511287,0.38268343236509));
#48498=DIRECTION('ref_axis',(0.707106781186563,0.270598050073092,0.653281482438174));
#48499=DIRECTION('center_axis',(0.,0.923879532511287,-0.382683432365089));
#48500=DIRECTION('ref_axis',(0.,0.382683432365089,0.923879532511287));
#48501=DIRECTION('center_axis',(0.,0.923879532511282,0.382683432365102));
#48502=DIRECTION('ref_axis',(-1.63551297779558E-16,-0.382683432365102,0.923879532511282));
#48503=DIRECTION('',(0.,-0.923879532511287,0.38268343236509));
#48504=DIRECTION('center_axis',(0.706796314702774,0.653568190184467,-0.270716808310044));
#48505=DIRECTION('ref_axis',(0.,0.382683432365089,0.923879532511287));
#48506=DIRECTION('center_axis',(-0.706790970016032,-0.653573123660655,0.270718851822791));
#48507=DIRECTION('ref_axis',(0.707106781189254,-0.664129312720945,0.242759667121573));
#48508=DIRECTION('center_axis',(0.,0.,1.));
#48509=DIRECTION('ref_axis',(1.,0.,0.));
#48510=DIRECTION('center_axis',(0.,0.343314013641807,0.939220681223083));
#48511=DIRECTION('ref_axis',(0.,-0.939220681223083,0.343314013641807));
#48512=DIRECTION('center_axis',(-1.,0.,0.));
#48513=DIRECTION('ref_axis',(0.,-0.401951975455108,0.915660750184115));
#48514=DIRECTION('',(1.,0.,0.));
#48515=DIRECTION('center_axis',(-1.,0.,0.));
#48516=DIRECTION('ref_axis',(0.,-0.9390974037827,0.343651082071035));
#48517=DIRECTION('',(-1.,0.,0.));
#48518=DIRECTION('center_axis',(-0.250366849757643,-0.807010963742363,-0.534836185146496));
#48519=DIRECTION('ref_axis',(0.34214448758192,-0.590536454759252,0.730892499084291));
#48520=DIRECTION('center_axis',(0.,0.343651082071034,0.9390974037827));
#48521=DIRECTION('ref_axis',(0.,-0.9390974037827,0.343651082071034));
#48522=DIRECTION('center_axis',(1.,0.,0.));
#48523=DIRECTION('ref_axis',(0.,0.,-1.));
#48524=DIRECTION('center_axis',(1.,0.,0.));
#48525=DIRECTION('ref_axis',(0.,-0.946930129495106,0.321439465303162));
#48526=DIRECTION('center_axis',(0.,-0.299392004564386,-0.95413019426225));
#48527=DIRECTION('ref_axis',(0.,-0.95413019426225,0.299392004564386));
#48528=DIRECTION('center_axis',(-1.,0.,0.));
#48529=DIRECTION('ref_axis',(0.,1.,0.));
#48530=DIRECTION('center_axis',(-1.,0.,0.));
#48531=DIRECTION('ref_axis',(0.,-0.945616565647212,0.325283431446442));
#48532=DIRECTION('center_axis',(0.,-0.923879532511287,0.38268343236509));
#48533=DIRECTION('ref_axis',(-0.70710678118656,-0.270598050073094,-0.653281482438177));
#48534=DIRECTION('center_axis',(0.,0.923879532511288,-0.382683432365087));
#48535=DIRECTION('ref_axis',(0.,-0.382683432365087,-0.923879532511288));
#48536=DIRECTION('center_axis',(0.,0.38268343236508,-0.923879532511291));
#48537=DIRECTION('ref_axis',(0.,-0.923879532511291,-0.38268343236508));
#48538=DIRECTION('',(0.,-0.923879532511287,0.38268343236509));
#48539=DIRECTION('center_axis',(-0.706796314702642,0.65356819018459,-0.270716808310093));
#48540=DIRECTION('ref_axis',(0.,-0.382683432365087,-0.923879532511288));
#48541=DIRECTION('center_axis',(0.706790970015978,-0.653573123660706,0.27071885182281));
#48542=DIRECTION('ref_axis',(-0.707106781189308,-0.641267347429939,0.29795333378948));
#48543=DIRECTION('center_axis',(0.,0.,1.));
#48544=DIRECTION('ref_axis',(1.,0.,0.));
#48545=DIRECTION('center_axis',(0.,-0.421369645600998,-0.906888979845984));
#48546=DIRECTION('ref_axis',(0.,-0.906888979845984,0.421369645600998));
#48547=DIRECTION('center_axis',(1.,0.,0.));
#48548=DIRECTION('ref_axis',(0.,-0.931692893277172,-0.363246958165945));
#48549=DIRECTION('',(-1.,0.,0.));
#48550=DIRECTION('center_axis',(1.,0.,0.));
#48551=DIRECTION('ref_axis',(0.,-0.90704015290395,0.421044131914909));
#48552=DIRECTION('',(1.,0.,0.));
#48553=DIRECTION('center_axis',(0.,0.,1.));
#48554=DIRECTION('ref_axis',(1.,0.,0.));
#48555=DIRECTION('center_axis',(0.,-0.421044131914906,-0.907040152903952));
#48556=DIRECTION('ref_axis',(0.,-0.907040152903951,0.421044131914905));
#48557=DIRECTION('center_axis',(1.,0.,0.));
#48558=DIRECTION('ref_axis',(0.,0.,-1.));
#48559=DIRECTION('center_axis',(-1.,0.,0.));
#48560=DIRECTION('ref_axis',(0.,-0.896872741532688,0.442288690219002));
#48561=DIRECTION('center_axis',(0.,0.462969813837161,0.886374047158188));
#48562=DIRECTION('ref_axis',(0.,-0.886374047158188,0.462969813837161));
#48563=DIRECTION('center_axis',(1.,0.,0.));
#48564=DIRECTION('ref_axis',(0.,1.,0.));
#48565=DIRECTION('center_axis',(1.,0.,0.));
#48566=DIRECTION('ref_axis',(0.,-0.898662006154886,0.438641765788069));
#48567=DIRECTION('center_axis',(1.,0.,0.));
#48568=DIRECTION('ref_axis',(0.,0.,-1.));
#48569=DIRECTION('center_axis',(-1.,0.,0.));
#48570=DIRECTION('ref_axis',(0.,-0.898662006154886,0.438641765788069));
#48571=DIRECTION('center_axis',(1.2777445139028E-14,-0.463287907664363,
-0.886207828114815));
#48572=DIRECTION('ref_axis',(0.,-0.886207828114815,0.463287907664363));
#48573=DIRECTION('center_axis',(1.,0.,0.));
#48574=DIRECTION('ref_axis',(0.,1.,0.));
#48575=DIRECTION('center_axis',(1.,0.,0.));
#48576=DIRECTION('ref_axis',(0.,0.,-1.));
#48577=DIRECTION('',(1.,0.,0.));
#48578=DIRECTION('center_axis',(0.706790970016262,-0.612645814094573,0.353711225685403));
#48579=DIRECTION('ref_axis',(0.,0.500000000000005,0.866025403784436));
#48580=DIRECTION('center_axis',(-0.706796314705249,0.612641189554964,-0.353708555706188));
#48581=DIRECTION('ref_axis',(-0.707106781186566,-0.626643564800569,0.327594021151193));
#48582=DIRECTION('center_axis',(0.,0.866025403784438,-0.5));
#48583=DIRECTION('ref_axis',(-0.707106781186566,0.353553390593265,0.612372435695778));
#48584=DIRECTION('center_axis',(3.70074341541727E-15,0.866025403784439,
-0.5));
#48585=DIRECTION('ref_axis',(-1.,0.,-7.40148683083454E-15));
#48586=DIRECTION('',(0.,0.866025403784438,-0.5));
#48587=DIRECTION('center_axis',(0.,0.965925826289068,0.258819045102521));
#48588=DIRECTION('ref_axis',(-4.088782444489E-17,-0.258819045102521,0.965925826289068));
#48589=DIRECTION('center_axis',(0.,0.,1.));
#48590=DIRECTION('ref_axis',(-0.911951719487274,0.410297527806596,0.));
#48591=DIRECTION('center_axis',(0.192364553135179,-0.871675368857608,-0.450752626197626));
#48592=DIRECTION('ref_axis',(-0.342144487592387,-0.490083718691967,0.801720087239428));
#48593=DIRECTION('center_axis',(-1.,0.,0.));
#48594=DIRECTION('ref_axis',(0.,-0.278995509497075,0.960292406343228));
#48595=DIRECTION('center_axis',(0.,0.38268343236509,0.923879532511287));
#48596=DIRECTION('ref_axis',(-1.,0.,0.));
#48597=DIRECTION('',(-1.,0.,0.));
#48598=DIRECTION('center_axis',(0.,0.38268343236509,0.923879532511287));
#48599=DIRECTION('ref_axis',(0.707106781186519,-0.653281482438215,0.270598050073107));
#48600=DIRECTION('',(0.706902428155821,0.653470225474163,-0.270676229998408));
#48601=DIRECTION('center_axis',(-0.706790970015244,-0.683317615876759,0.183094403348142));
#48602=DIRECTION('ref_axis',(0.,-0.258819045102527,-0.965925826289067));
#48603=DIRECTION('center_axis',(0.706796314705262,0.683312457872058,-0.183093021264894));
#48604=DIRECTION('ref_axis',(0.707106781186551,-0.674747867889584,0.21145996022523));
#48605=DIRECTION('center_axis',(1.,0.,0.));
#48606=DIRECTION('ref_axis',(0.,0.,-1.));
#48607=DIRECTION('center_axis',(1.,0.,0.));
#48608=DIRECTION('ref_axis',(0.,-0.945616565647212,0.325283431446442));
#48609=DIRECTION('center_axis',(5.28134399079828E-15,0.299049543649384,
0.954237585951787));
#48610=DIRECTION('ref_axis',(0.,-0.954237585951787,0.299049543649385));
#48611=DIRECTION('center_axis',(0.,0.,1.));
#48612=DIRECTION('ref_axis',(1.,0.,0.));
#48613=DIRECTION('center_axis',(1.,0.,0.));
#48614=DIRECTION('ref_axis',(0.,-0.87630888913323,-0.481749655761251));
#48615=DIRECTION('center_axis',(0.,0.965925826289068,-0.258819045102521));
#48616=DIRECTION('ref_axis',(0.70710678118656,-0.183012701892217,-0.683012701892207));
#48617=DIRECTION('center_axis',(0.,0.96592582628907,-0.258819045102513));
#48618=DIRECTION('ref_axis',(1.,0.,0.));
#48619=DIRECTION('',(0.,0.965925826289068,-0.258819045102521));
#48620=DIRECTION('center_axis',(0.,0.499999999999995,-0.866025403784442));
#48621=DIRECTION('ref_axis',(0.,-0.866025403784442,-0.499999999999995));
#48622=DIRECTION('center_axis',(0.,0.,1.));
#48623=DIRECTION('ref_axis',(1.,0.,0.));
#48624=DIRECTION('center_axis',(0.,-0.38268343236509,-0.923879532511287));
#48625=DIRECTION('ref_axis',(1.,0.,0.));
#48626=DIRECTION('',(1.,0.,0.));
#48627=DIRECTION('center_axis',(0.,-0.38268343236509,-0.923879532511287));
#48628=DIRECTION('ref_axis',(-0.707106781186561,-0.653281482438177,0.270598050073091));
#48629=DIRECTION('',(-0.706902428155815,0.65347022547417,-0.270676229998406));
#48630=DIRECTION('center_axis',(0.,-0.793353340291235,-0.60876142900872));
#48631=DIRECTION('ref_axis',(-0.707106781186569,0.430459334576865,-0.560985526796915));
#48632=DIRECTION('center_axis',(2.34879772014565E-14,0.793353340291229,
0.608761429008728));
#48633=DIRECTION('ref_axis',(0.,0.608761429008728,-0.793353340291229));
#48634=DIRECTION('center_axis',(0.,0.991444861373812,-0.130526192220039));
#48635=DIRECTION('ref_axis',(-8.1775648889781E-17,-0.130526192220039,-0.991444861373812));
#48636=DIRECTION('',(0.,-0.793353340291235,-0.60876142900872));
#48637=DIRECTION('center_axis',(-0.706796314703326,0.561231728319736,0.43064825164981));
#48638=DIRECTION('ref_axis',(0.,0.608761429008721,-0.793353340291235));
#48639=DIRECTION('center_axis',(0.706790970016641,-0.561235964791737,-0.43065150240911));
#48640=DIRECTION('ref_axis',(-0.707106781188646,-0.578668829919466,-0.40637714659743));
#48641=DIRECTION('center_axis',(0.,0.,1.));
#48642=DIRECTION('ref_axis',(-0.903692699960975,0.428181625057922,0.));
#48643=DIRECTION('center_axis',(0.,0.574704072158276,-0.818361307397102));
#48644=DIRECTION('ref_axis',(0.,-0.818361307397102,-0.574704072158276));
#48645=DIRECTION('center_axis',(1.,0.,0.));
#48646=DIRECTION('ref_axis',(0.,-0.151265353019465,-0.988493193186426));
#48647=DIRECTION('',(-1.,0.,0.));
#48648=DIRECTION('center_axis',(1.,0.,0.));
#48649=DIRECTION('ref_axis',(0.,-0.818154990804646,-0.574997748709897));
#48650=DIRECTION('',(1.,0.,0.));
#48651=DIRECTION('center_axis',(0.14109761386294,-0.924473827538088,0.354174541094164));
#48652=DIRECTION('ref_axis',(-0.342144487584237,-0.381245514330439,-0.858830022425066));
#48653=DIRECTION('center_axis',(0.,0.57499774870989,-0.818154990804651));
#48654=DIRECTION('ref_axis',(0.,-0.818154990804651,-0.57499774870989));
#48655=DIRECTION('center_axis',(1.,0.,0.));
#48656=DIRECTION('ref_axis',(0.,0.,-1.));
#48657=DIRECTION('center_axis',(-1.,0.,0.));
#48658=DIRECTION('ref_axis',(0.,-0.831469612302545,-0.555570233019602));
#48659=DIRECTION('center_axis',(0.,-0.536137535175636,0.844130643547427));
#48660=DIRECTION('ref_axis',(0.,-0.844130643547427,-0.536137535175636));
#48661=DIRECTION('center_axis',(1.,0.,0.));
#48662=DIRECTION('ref_axis',(0.,1.,0.));
#48663=DIRECTION('center_axis',(1.,0.,0.));
#48664=DIRECTION('ref_axis',(0.,-0.829205915410775,-0.558943243851984));
#48665=DIRECTION('center_axis',(1.,0.,0.));
#48666=DIRECTION('ref_axis',(0.,0.,-1.));
#48667=DIRECTION('center_axis',(-1.,0.,0.));
#48668=DIRECTION('ref_axis',(0.,-0.829205915410775,-0.558943243851984));
#48669=DIRECTION('center_axis',(-3.26250765883222E-14,0.535834538347871,
-0.844323011360891));
#48670=DIRECTION('ref_axis',(0.,-0.844323011360891,-0.535834538347871));
#48671=DIRECTION('center_axis',(1.,0.,0.));
#48672=DIRECTION('ref_axis',(0.,1.,0.));
#48673=DIRECTION('center_axis',(1.,0.,0.));
#48674=DIRECTION('ref_axis',(0.,0.,-1.));
#48675=DIRECTION('',(1.,0.,0.));
#48676=DIRECTION('center_axis',(0.,-0.923879532511287,-0.382683432365089));
#48677=DIRECTION('ref_axis',(0.70710678118656,-0.270598050073094,0.653281482438177));
#48678=DIRECTION('center_axis',(-2.83242638502858E-15,0.923879532511288,
0.382683432365087));
#48679=DIRECTION('ref_axis',(0.,-0.382683432365087,0.923879532511288));
#48680=DIRECTION('center_axis',(0.,0.382683432365089,0.923879532511287));
#48681=DIRECTION('ref_axis',(8.17756488897798E-17,-0.923879532511287,0.382683432365089));
#48682=DIRECTION('',(0.,-0.923879532511287,-0.382683432365089));
#48683=DIRECTION('center_axis',(0.706796314702672,0.653568190184562,0.270716808310081));
#48684=DIRECTION('ref_axis',(0.,-0.382683432365087,0.923879532511288));
#48685=DIRECTION('center_axis',(-0.706790970015914,-0.653573123660765,-0.270718851822834));
#48686=DIRECTION('ref_axis',(0.707106781189373,-0.641267347429885,-0.297953333789445));
#48687=DIRECTION('center_axis',(0.,0.,1.));
#48688=DIRECTION('ref_axis',(1.,0.,0.));
#48689=DIRECTION('center_axis',(0.,-0.421369645600998,0.906888979845984));
#48690=DIRECTION('ref_axis',(0.,-0.906888979845984,-0.421369645600998));
#48691=DIRECTION('center_axis',(-1.,0.,0.));
#48692=DIRECTION('ref_axis',(0.,-0.931692893277179,0.363246958165926));
#48693=DIRECTION('',(1.,0.,0.));
#48694=DIRECTION('center_axis',(-1.,0.,0.));
#48695=DIRECTION('ref_axis',(0.,-0.90704015290395,-0.421044131914909));
#48696=DIRECTION('',(-1.,0.,0.));
#48697=DIRECTION('center_axis',(0.,0.,1.));
#48698=DIRECTION('ref_axis',(1.,0.,0.));
#48699=DIRECTION('center_axis',(0.,-0.421044131914905,0.907040152903952));
#48700=DIRECTION('ref_axis',(0.,-0.907040152903952,-0.421044131914905));
#48701=DIRECTION('center_axis',(1.,0.,0.));
#48702=DIRECTION('ref_axis',(0.,0.,-1.));
#48703=DIRECTION('center_axis',(1.,0.,0.));
#48704=DIRECTION('ref_axis',(0.,-0.896872741532689,-0.442288690219));
#48705=DIRECTION('center_axis',(0.,0.462969813837163,-0.886374047158186));
#48706=DIRECTION('ref_axis',(0.,-0.886374047158186,-0.462969813837163));
#48707=DIRECTION('center_axis',(-1.,0.,0.));
#48708=DIRECTION('ref_axis',(0.,1.,0.));
#48709=DIRECTION('center_axis',(-1.,0.,0.));
#48710=DIRECTION('ref_axis',(0.,-0.898662006154886,-0.438641765788069));
#48711=DIRECTION('center_axis',(0.706790970015214,-0.683317615876791,-0.18309440334814));
#48712=DIRECTION('ref_axis',(0.,-0.258819045102513,0.96592582628907));
#48713=DIRECTION('center_axis',(-0.706796314705262,0.683312457872044,0.183093021264946));
#48714=DIRECTION('ref_axis',(-0.707106781186552,-0.674747867889585,-0.211459960225222));
#48715=DIRECTION('center_axis',(0.,0.965925826289068,0.25881904510252));
#48716=DIRECTION('ref_axis',(-0.707106781186562,-0.183012701892215,0.683012701892206));
#48717=DIRECTION('center_axis',(0.,0.965925826289066,0.258819045102529));
#48718=DIRECTION('ref_axis',(-1.,0.,0.));
#48719=DIRECTION('',(0.,0.965925826289068,0.25881904510252));
#48720=DIRECTION('center_axis',(0.,0.500000000000003,0.866025403784437));
#48721=DIRECTION('ref_axis',(1.2266347333467E-16,-0.866025403784437,0.500000000000003));
#48722=DIRECTION('center_axis',(0.,0.,1.));
#48723=DIRECTION('ref_axis',(1.,0.,0.));
#48724=DIRECTION('center_axis',(0.,0.,1.));
#48725=DIRECTION('ref_axis',(1.,0.,0.));
#48726=DIRECTION('center_axis',(-1.,0.,0.));
#48727=DIRECTION('ref_axis',(0.,-0.87630888913324,0.481749655761233));
#48728=DIRECTION('center_axis',(0.,-0.382683432365089,0.923879532511287));
#48729=DIRECTION('ref_axis',(-1.,0.,0.));
#48730=DIRECTION('',(-1.,0.,0.));
#48731=DIRECTION('center_axis',(0.,-0.382683432365089,0.923879532511287));
#48732=DIRECTION('ref_axis',(0.707106781186519,-0.653281482438215,-0.270598050073107));
#48733=DIRECTION('',(0.706902428155816,0.653470225474171,0.2706762299984));
#48734=DIRECTION('center_axis',(0.706790970014439,-0.70137035423385,-0.0923371588686459));
#48735=DIRECTION('ref_axis',(0.,-0.130526192220056,0.99144486137381));
#48736=DIRECTION('center_axis',(-0.706796314705254,0.701365059957731,0.0923364618639829));
#48737=DIRECTION('ref_axis',(-0.70710678118656,-0.696576369757257,-0.121578621047388));
#48738=DIRECTION('center_axis',(0.,0.99144486137381,0.130526192220051));
#48739=DIRECTION('ref_axis',(-0.707106781186561,-0.0922959556412554,0.701057384649965));
#48740=DIRECTION('center_axis',(1.46763321699136E-14,0.99144486137381,0.130526192220056));
#48741=DIRECTION('ref_axis',(-1.,1.48029736616691E-14,0.));
#48742=DIRECTION('',(0.,0.991444861373811,0.130526192220051));
#48743=DIRECTION('center_axis',(0.,0.608761429008727,0.793353340291231));
#48744=DIRECTION('ref_axis',(-2.04439122224451E-16,-0.79335334029123,0.608761429008727));
#48745=DIRECTION('center_axis',(0.,0.,1.));
#48746=DIRECTION('ref_axis',(1.,0.,0.));
#48747=DIRECTION('center_axis',(0.,0.,1.));
#48748=DIRECTION('ref_axis',(1.,0.,0.));
#48749=DIRECTION('center_axis',(-1.,0.,0.));
#48750=DIRECTION('ref_axis',(0.,-0.805930996937513,0.592009483180216));
#48751=DIRECTION('center_axis',(0.,-0.25881904510252,0.965925826289068));
#48752=DIRECTION('ref_axis',(-1.,0.,0.));
#48753=DIRECTION('',(-1.,0.,0.));
#48754=DIRECTION('center_axis',(0.,-0.25881904510252,0.965925826289068));
#48755=DIRECTION('ref_axis',(0.707106781186522,-0.683012701892242,-0.183012701892233));
#48756=DIRECTION('',(0.70690242815582,0.683210034733317,0.183065577067634));
#48757=DIRECTION('center_axis',(0.,-1.,1.22464679914735E-16));
#48758=DIRECTION('ref_axis',(-0.707106781186561,-8.17756488897784E-17,-0.707106781186534));
#48759=DIRECTION('center_axis',(0.,1.,0.));
#48760=DIRECTION('ref_axis',(0.,0.,-1.));
#48761=DIRECTION('center_axis',(0.,0.70710678118655,-0.707106781186545));
#48762=DIRECTION('ref_axis',(-4.08878244448901E-17,-0.707106781186545,-0.70710678118655));
#48763=DIRECTION('',(0.,-1.,1.22464679914735E-16));
#48764=DIRECTION('center_axis',(-0.706796314700322,0.707417111417333,0.));
#48765=DIRECTION('ref_axis',(0.,0.,-1.));
#48766=DIRECTION('center_axis',(0.706790970013417,-0.707422451373643,0.));
#48767=DIRECTION('ref_axis',(-0.707106781191869,-0.706475581614947,0.0298705971533368));
#48768=DIRECTION('center_axis',(0.429570054990523,0.177774910040184,-0.885361874724479));
#48769=DIRECTION('ref_axis',(-0.818074617559303,-0.338555120062959,-0.464902517507009));
#48770=DIRECTION('center_axis',(0.,-0.042243403610761,-0.999107349012797));
#48771=DIRECTION('ref_axis',(0.,-0.999107349012797,0.042243403610761));
#48772=DIRECTION('center_axis',(1.,0.,0.));
#48773=DIRECTION('ref_axis',(0.,-0.721763401937878,-0.692139864205972));
#48774=DIRECTION('',(-1.,0.,0.));
#48775=DIRECTION('center_axis',(1.,0.,0.));
#48776=DIRECTION('ref_axis',(0.,-0.999122446012244,0.0418848167539264));
#48777=DIRECTION('',(1.,0.,0.));
#48778=DIRECTION('center_axis',(-0.939647353864348,0.30050285376847,0.163587546141918));
#48779=DIRECTION('ref_axis',(-0.342144487571735,-0.825284993998399,-0.449268102924454));
#48780=DIRECTION('center_axis',(0.,-0.0418848167539204,-0.999122446012245));
#48781=DIRECTION('ref_axis',(0.,-0.999122446012244,0.0418848167539204));
#48782=DIRECTION('center_axis',(1.,0.,0.));
#48783=DIRECTION('ref_axis',(0.,0.,-1.));
#48784=DIRECTION('center_axis',(-1.,0.,0.));
#48785=DIRECTION('ref_axis',(0.,-0.997858923238603,0.0654031292301436));
#48786=DIRECTION('center_axis',(0.,0.0885276724488821,0.996073717759275));
#48787=DIRECTION('ref_axis',(0.,-0.996073717759275,0.0885276724488821));
#48788=DIRECTION('center_axis',(1.,0.,0.));
#48789=DIRECTION('ref_axis',(0.,1.,0.));
#48790=DIRECTION('center_axis',(1.,0.,0.));
#48791=DIRECTION('ref_axis',(0.,-0.998116370642493,0.0613490884647576));
#48792=DIRECTION('center_axis',(1.,0.,0.));
#48793=DIRECTION('ref_axis',(0.,0.,-1.));
#48794=DIRECTION('center_axis',(-1.,0.,0.));
#48795=DIRECTION('ref_axis',(0.,-0.998116370642493,0.0613490884647577));
#48796=DIRECTION('center_axis',(1.12335038513957E-14,-0.0888851620992988,
-0.996041880624797));
#48797=DIRECTION('ref_axis',(0.,-0.996041880624796,0.0888851620992988));
#48798=DIRECTION('center_axis',(1.,0.,0.));
#48799=DIRECTION('ref_axis',(0.,1.,0.));
#48800=DIRECTION('center_axis',(1.,0.,0.));
#48801=DIRECTION('ref_axis',(0.,0.,-1.));
#48802=DIRECTION('',(1.,0.,0.));
#48803=DIRECTION('center_axis',(0.706790970015359,-0.683317615876648,0.183094403348113));
#48804=DIRECTION('ref_axis',(0.,0.258819045102527,0.965925826289067));
#48805=DIRECTION('center_axis',(-0.706796314705253,0.683312457872062,-0.183093021264916));
#48806=DIRECTION('ref_axis',(-0.707106781186562,-0.690078774854367,0.154244236506507));
#48807=DIRECTION('center_axis',(0.,0.965925826289068,-0.258819045102521));
#48808=DIRECTION('ref_axis',(-0.707106781186561,0.183012701892216,0.683012701892207));
#48809=DIRECTION('center_axis',(0.,0.965925826289066,-0.258819045102528));
#48810=DIRECTION('ref_axis',(-1.,0.,0.));
#48811=DIRECTION('',(0.,0.965925826289068,-0.258819045102521));
#48812=DIRECTION('center_axis',(0.,0.866025403784436,0.500000000000005));
#48813=DIRECTION('ref_axis',(-1.63551297779559E-16,-0.500000000000005,0.866025403784436));
#48814=DIRECTION('center_axis',(0.,0.,1.));
#48815=DIRECTION('ref_axis',(-0.921538338698281,0.388287381084181,0.));
#48816=DIRECTION('center_axis',(-0.939647353856842,0.247923894858416,-0.235789297356914));
#48817=DIRECTION('ref_axis',(-0.342144487592343,-0.680884948347189,0.64755913762715));
#48818=DIRECTION('center_axis',(-1.,0.,0.));
#48819=DIRECTION('ref_axis',(0.,-0.518030931670889,0.855361884720257));
#48820=DIRECTION('center_axis',(-1.,0.,0.));
#48821=DIRECTION('ref_axis',(0.,-0.518030931670894,0.855361884720254));
#48822=DIRECTION('',(-1.,0.,0.));
#48823=DIRECTION('center_axis',(0.,-0.258819045102521,-0.965925826289068));
#48824=DIRECTION('ref_axis',(1.,0.,0.));
#48825=DIRECTION('',(-0.706902428155817,-0.683210034733321,0.183065577067633));
#48826=DIRECTION('center_axis',(0.,-0.258819045102521,-0.965925826289068));
#48827=DIRECTION('ref_axis',(0.707106781186512,-0.683012701892253,0.18301270189223));
#48828=DIRECTION('',(1.,0.,0.));
#48829=DIRECTION('center_axis',(0.706790970014404,-0.701370354233883,0.0923371588686503));
#48830=DIRECTION('ref_axis',(0.,0.130526192220056,0.99144486137381));
#48831=DIRECTION('center_axis',(-0.706796314705254,0.701365059957736,-0.0923364618639514));
#48832=DIRECTION('ref_axis',(-0.707106781186561,-0.704307968135582,0.0628513008672784));
#48833=DIRECTION('center_axis',(0.,0.99144486137381,-0.130526192220052));
#48834=DIRECTION('ref_axis',(-0.70710678118656,0.0922959556412559,0.701057384649965));
#48835=DIRECTION('center_axis',(1.49178541431126E-14,0.99144486137381,-0.130526192220056));
#48836=DIRECTION('ref_axis',(-1.,1.48029736616691E-14,-1.85037170770863E-15));
#48837=DIRECTION('',(0.,0.99144486137381,-0.130526192220052));
#48838=DIRECTION('center_axis',(0.,0.793353340291238,0.608761429008717));
#48839=DIRECTION('ref_axis',(1.63551297779561E-16,-0.608761429008717,0.793353340291238));
#48840=DIRECTION('center_axis',(0.,0.,1.));
#48841=DIRECTION('ref_axis',(-0.923502716555982,0.383591882752648,0.));
#48842=DIRECTION('center_axis',(-0.939647353856839,0.276579550719403,-0.201411525275229));
#48843=DIRECTION('ref_axis',(-0.342144487592345,-0.759583311697356,0.553145859788401));
#48844=DIRECTION('center_axis',(-1.,0.,0.));
#48845=DIRECTION('ref_axis',(0.,-0.625246235020483,0.780427540257717));
#48846=DIRECTION('center_axis',(0.,1.22464679914735E-16,1.));
#48847=DIRECTION('ref_axis',(-1.,0.,0.));
#48848=DIRECTION('',(-1.,0.,0.));
#48849=DIRECTION('center_axis',(0.,1.22464679914735E-16,1.));
#48850=DIRECTION('ref_axis',(0.707106781186527,-0.707106781186568,8.65956056235553E-17));
#48851=DIRECTION('',(0.706902428155817,0.707311075176552,0.));
#48852=DIRECTION('center_axis',(-1.,0.,0.));
#48853=DIRECTION('ref_axis',(0.,-0.805930996937512,0.592009483180217));
#48854=DIRECTION('',(-1.,0.,0.));
#48855=DIRECTION('center_axis',(0.,0.130526192220051,-0.99144486137381));
#48856=DIRECTION('ref_axis',(1.,0.,0.));
#48857=DIRECTION('',(-0.706902428155813,-0.701259930876582,-0.0923226213578649));
#48858=DIRECTION('center_axis',(0.,0.130526192220051,-0.99144486137381));
#48859=DIRECTION('ref_axis',(0.70710678118652,-0.701057384650004,-0.0922959556412642));
#48860=DIRECTION('',(1.,0.,0.));
#48861=DIRECTION('center_axis',(-1.,0.,0.));
#48862=DIRECTION('ref_axis',(0.,-0.87630888913324,0.481749655761234));
#48863=DIRECTION('',(-1.,0.,0.));
#48864=DIRECTION('center_axis',(0.,0.25881904510252,-0.965925826289068));
#48865=DIRECTION('ref_axis',(1.,0.,0.));
#48866=DIRECTION('',(-0.706902428155817,-0.683210034733321,-0.183065577067633));
#48867=DIRECTION('center_axis',(0.,0.25881904510252,-0.965925826289068));
#48868=DIRECTION('ref_axis',(0.707106781186522,-0.683012701892242,-0.183012701892233));
#48869=DIRECTION('',(1.,0.,0.));
#48870=DIRECTION('center_axis',(-0.706790970016285,-0.612645814094553,-0.353711225685392));
#48871=DIRECTION('ref_axis',(0.,0.500000000000005,-0.866025403784436));
#48872=DIRECTION('center_axis',(0.706796314705255,0.612641189554909,0.353708555706272));
#48873=DIRECTION('ref_axis',(0.707106781186558,-0.626643564800577,-0.327594021151197));
#48874=DIRECTION('center_axis',(1.,0.,0.));
#48875=DIRECTION('ref_axis',(0.,0.,-1.));
#48876=DIRECTION('center_axis',(1.,0.,0.));
#48877=DIRECTION('ref_axis',(0.,-0.898662006154886,-0.438641765788069));
#48878=DIRECTION('center_axis',(-5.8776247639534E-15,-0.463287907664357,
0.886207828114818));
#48879=DIRECTION('ref_axis',(0.,-0.886207828114818,-0.463287907664357));
#48880=DIRECTION('center_axis',(-0.192364553135179,-0.871675368857559,0.45075262619772));
#48881=DIRECTION('ref_axis',(0.342144487592291,-0.49008371869206,-0.801720087239412));
#48882=DIRECTION('center_axis',(1.,0.,0.));
#48883=DIRECTION('ref_axis',(0.,-0.278995509497148,-0.960292406343207));
#48884=DIRECTION('center_axis',(0.,0.866025403784439,0.5));
#48885=DIRECTION('ref_axis',(0.707106781186558,0.353553390593268,-0.612372435695786));
#48886=DIRECTION('center_axis',(0.,0.866025403784438,0.500000000000001));
#48887=DIRECTION('ref_axis',(1.,0.,0.));
#48888=DIRECTION('',(0.,0.866025403784439,0.5));
#48889=DIRECTION('center_axis',(0.,0.965925826289068,-0.258819045102521));
#48890=DIRECTION('ref_axis',(1.2266347333467E-16,-0.258819045102521,-0.965925826289068));
#48891=DIRECTION('center_axis',(0.,0.,1.));
#48892=DIRECTION('ref_axis',(1.,0.,0.));
#48893=DIRECTION('center_axis',(0.,0.382683432365089,-0.923879532511287));
#48894=DIRECTION('ref_axis',(1.,0.,0.));
#48895=DIRECTION('',(1.,0.,0.));
#48896=DIRECTION('center_axis',(0.,0.382683432365089,-0.923879532511287));
#48897=DIRECTION('ref_axis',(-0.707106781186561,-0.653281482438177,-0.270598050073091));
#48898=DIRECTION('',(-0.706902428155816,0.65347022547417,0.270676229998403));
#48899=DIRECTION('center_axis',(0.706790970016273,-0.612645814094562,-0.3537112256854));
#48900=DIRECTION('ref_axis',(0.,-0.500000000000008,0.866025403784434));
#48901=DIRECTION('center_axis',(-0.706796314705252,0.612641189554944,0.353708555706217));
#48902=DIRECTION('ref_axis',(-0.707106781186562,-0.597026526845112,-0.378892235659747));
#48903=DIRECTION('center_axis',(0.,0.866025403784439,0.5));
#48904=DIRECTION('ref_axis',(-0.707106781186561,-0.353553390593267,0.612372435695783));
#48905=DIRECTION('center_axis',(7.40148683083455E-15,0.866025403784438,
0.500000000000001));
#48906=DIRECTION('ref_axis',(-1.,0.,1.48029736616691E-14));
#48907=DIRECTION('',(0.,0.866025403784439,0.5));
#48908=DIRECTION('center_axis',(0.,0.258819045102524,0.965925826289067));
#48909=DIRECTION('ref_axis',(-8.17756488897802E-17,-0.965925826289067,0.258819045102524));
#48910=DIRECTION('center_axis',(0.,0.,1.));
#48911=DIRECTION('ref_axis',(1.,0.,0.));
#48912=DIRECTION('center_axis',(0.,0.,1.));
#48913=DIRECTION('ref_axis',(1.,0.,0.));
#48914=DIRECTION('center_axis',(-1.,0.,0.));
#48915=DIRECTION('ref_axis',(0.,-0.971135373703069,0.238529004405336));
#48916=DIRECTION('center_axis',(0.,-0.60876142900872,0.793353340291235));
#48917=DIRECTION('ref_axis',(-1.,0.,0.));
#48918=DIRECTION('',(-1.,0.,0.));
#48919=DIRECTION('center_axis',(0.,-0.60876142900872,0.793353340291235));
#48920=DIRECTION('ref_axis',(0.707106781186524,-0.560985526796945,-0.430459334576899));
#48921=DIRECTION('',(0.706902428155818,0.561147604116297,0.430583700878177));
#48922=DIRECTION('center_axis',(0.,-0.130526192220052,-0.99144486137381));
#48923=DIRECTION('ref_axis',(-0.70710678118656,0.701057384649966,-0.0922959556412584));
#48924=DIRECTION('center_axis',(4.83043946397912E-16,0.13052619222007,0.991444861373808));
#48925=DIRECTION('ref_axis',(0.,0.991444861373808,-0.13052619222007));
#48926=DIRECTION('center_axis',(0.,0.793353340291228,0.60876142900873));
#48927=DIRECTION('ref_axis',(8.1775648889781E-17,0.60876142900873,-0.793353340291228));
#48928=DIRECTION('',(0.,-0.130526192220052,-0.99144486137381));
#48929=DIRECTION('center_axis',(-0.706796314701344,0.0923364618644818,0.701365059961606));
#48930=DIRECTION('ref_axis',(0.,0.99144486137381,-0.130526192220055));
#48931=DIRECTION('center_axis',(0.70679097001452,-0.0923371588686349,-0.701370354233768));
#48932=DIRECTION('ref_axis',(-0.707106781190766,-0.121828617618676,-0.696532689773536));
#48933=DIRECTION('center_axis',(0.,0.,1.));
#48934=DIRECTION('ref_axis',(-0.764784300456407,0.644286406635592,0.));
#48935=DIRECTION('center_axis',(0.,0.98504597651982,-0.17229168332254));
#48936=DIRECTION('ref_axis',(0.,-0.17229168332254,-0.98504597651982));
#48937=DIRECTION('center_axis',(1.,0.,0.));
#48938=DIRECTION('ref_axis',(0.,0.59200948318021,-0.805930996937517));
#48939=DIRECTION('',(-1.,0.,0.));
#48940=DIRECTION('center_axis',(1.,0.,0.));
#48941=DIRECTION('ref_axis',(0.,-0.171938134779829,-0.985107749339347));
#48942=DIRECTION('',(1.,0.,0.));
#48943=DIRECTION('center_axis',(-0.122754826313525,-0.941252632833084,-0.314602501263934));
#48944=DIRECTION('ref_axis',(-0.342144487575902,0.337703244261566,-0.876865821227305));
#48945=DIRECTION('center_axis',(0.,0.985107749339348,-0.171938134779822));
#48946=DIRECTION('ref_axis',(0.,-0.171938134779822,-0.985107749339348));
#48947=DIRECTION('center_axis',(1.,0.,0.));
#48948=DIRECTION('ref_axis',(0.,0.,-1.));
#48949=DIRECTION('center_axis',(-1.,0.,0.));
#48950=DIRECTION('ref_axis',(0.,-0.19509032201613,-0.98078528040323));
#48951=DIRECTION('center_axis',(0.,-0.975996989031084,0.217784015488417));
#48952=DIRECTION('ref_axis',(0.,-0.217784015488417,-0.975996989031083));
#48953=DIRECTION('center_axis',(1.,0.,0.));
#48954=DIRECTION('ref_axis',(0.,1.,0.));
#48955=DIRECTION('center_axis',(1.,0.,0.));
#48956=DIRECTION('ref_axis',(0.,-0.191104567760814,-0.981569683813102));
#48957=DIRECTION('center_axis',(1.,0.,0.));
#48958=DIRECTION('ref_axis',(0.,0.,-1.));
#48959=DIRECTION('center_axis',(-1.,0.,0.));
#48960=DIRECTION('ref_axis',(0.,-0.191104567760814,-0.981569683813102));
#48961=DIRECTION('center_axis',(1.72921424214846E-14,0.975918762504878,
-0.218134291185378));
#48962=DIRECTION('ref_axis',(0.,-0.218134291185377,-0.975918762504878));
#48963=DIRECTION('center_axis',(1.,0.,0.));
#48964=DIRECTION('ref_axis',(0.,1.,0.));
#48965=DIRECTION('center_axis',(1.,0.,0.));
#48966=DIRECTION('ref_axis',(0.,0.,-1.));
#48967=DIRECTION('',(1.,0.,0.));
#48968=DIRECTION('center_axis',(0.706790970016575,-0.561235964791789,-0.43065150240915));
#48969=DIRECTION('ref_axis',(0.,-0.608761429008721,0.793353340291235));
#48970=DIRECTION('center_axis',(-0.706796314705255,0.561231728318206,0.430648251648638));
#48971=DIRECTION('ref_axis',(-0.70710678118656,-0.542463521362063,-0.453578359262712));
#48972=DIRECTION('center_axis',(0.,0.793353340291235,0.60876142900872));
#48973=DIRECTION('ref_axis',(-0.707106781186563,-0.430459334576869,0.56098552679692));
#48974=DIRECTION('center_axis',(2.34879772014569E-14,0.793353340291242,
0.608761429008712));
#48975=DIRECTION('ref_axis',(-1.,2.96059473233381E-14,0.));
#48976=DIRECTION('',(0.,0.793353340291235,0.60876142900872));
#48977=DIRECTION('center_axis',(0.,0.13052619222005,0.991444861373811));
#48978=DIRECTION('ref_axis',(-1.2266347333467E-16,-0.991444861373811,0.13052619222005));
#48979=DIRECTION('center_axis',(0.,0.,1.));
#48980=DIRECTION('ref_axis',(1.,0.,0.));
#48981=DIRECTION('center_axis',(0.,0.,1.));
#48982=DIRECTION('ref_axis',(1.,0.,0.));
#48983=DIRECTION('center_axis',(-1.,0.,0.));
#48984=DIRECTION('ref_axis',(0.,-0.993961458635313,0.109729753246606));
#48985=DIRECTION('center_axis',(-1.,0.,0.));
#48986=DIRECTION('ref_axis',(0.,-0.993961458635313,0.109729753246601));
#48987=DIRECTION('',(-1.,0.,0.));
#48988=DIRECTION('center_axis',(0.,0.60876142900872,-0.793353340291235));
#48989=DIRECTION('ref_axis',(1.,0.,0.));
#48990=DIRECTION('',(-0.706902428155814,-0.5611476041163,-0.430583700878181));
#48991=DIRECTION('center_axis',(0.,0.60876142900872,-0.793353340291235));
#48992=DIRECTION('ref_axis',(0.707106781186524,-0.560985526796945,-0.430459334576899));
#48993=DIRECTION('',(1.,0.,0.));
#48994=DIRECTION('center_axis',(0.,0.25881904510252,-0.965925826289068));
#48995=DIRECTION('ref_axis',(-0.707106781186564,0.683012701892207,0.183012701892201));
#48996=DIRECTION('center_axis',(0.,-0.258819045102515,0.96592582628907));
#48997=DIRECTION('ref_axis',(0.,0.96592582628907,0.258819045102515));
#48998=DIRECTION('center_axis',(0.,0.500000000000006,0.866025403784435));
#48999=DIRECTION('ref_axis',(-1.22663473334669E-16,0.866025403784435,-0.500000000000006));
#49000=DIRECTION('',(0.,0.25881904510252,-0.965925826289068));
#49001=DIRECTION('center_axis',(-0.706796314702179,-0.183093021265733,0.683312457875023));
#49002=DIRECTION('ref_axis',(0.,0.96592582628907,0.258819045102515));
#49003=DIRECTION('center_axis',(0.706790970015427,0.183094403348087,-0.683317615876585));
#49004=DIRECTION('ref_axis',(-0.70710678118986,0.153996554185174,-0.690134089358299));
#49005=DIRECTION('center_axis',(0.,0.,1.));
#49006=DIRECTION('ref_axis',(1.,0.,0.));
#49007=DIRECTION('center_axis',(0.,0.975996989031084,0.217784015488416));
#49008=DIRECTION('ref_axis',(0.,0.217784015488416,-0.975996989031084));
#49009=DIRECTION('center_axis',(1.,0.,0.));
#49010=DIRECTION('ref_axis',(0.,0.855361884720247,-0.518030931670906));
#49011=DIRECTION('',(-1.,0.,0.));
#49012=DIRECTION('center_axis',(1.,0.,0.));
#49013=DIRECTION('ref_axis',(0.,0.218134291185381,-0.975918762504877));
#49014=DIRECTION('',(1.,0.,0.));
#49015=DIRECTION('center_axis',(0.,0.,1.));
#49016=DIRECTION('ref_axis',(1.,0.,0.));
#49017=DIRECTION('center_axis',(0.,0.975918762504877,0.218134291185385));
#49018=DIRECTION('ref_axis',(0.,0.218134291185385,-0.975918762504877));
#49019=DIRECTION('center_axis',(1.,0.,0.));
#49020=DIRECTION('ref_axis',(0.,0.,-1.));
#49021=DIRECTION('center_axis',(-1.,0.,0.));
#49022=DIRECTION('ref_axis',(0.,0.195090322016127,-0.980785280403231));
#49023=DIRECTION('center_axis',(0.,-0.98504597651982,-0.172291683322539));
#49024=DIRECTION('ref_axis',(0.,0.172291683322539,-0.98504597651982));
#49025=DIRECTION('center_axis',(1.,0.,0.));
#49026=DIRECTION('ref_axis',(0.,1.,0.));
#49027=DIRECTION('center_axis',(1.,0.,0.));
#49028=DIRECTION('ref_axis',(0.,0.199072856983481,-0.979984692539855));
#49029=DIRECTION('center_axis',(1.,0.,0.));
#49030=DIRECTION('ref_axis',(0.,0.,-1.));
#49031=DIRECTION('center_axis',(-1.,0.,0.));
#49032=DIRECTION('ref_axis',(0.,0.199072856983481,-0.979984692539855));
#49033=DIRECTION('center_axis',(1.70365935187056E-14,0.985107749339347,
0.171938134779828));
#49034=DIRECTION('ref_axis',(0.,0.171938134779828,-0.985107749339347));
#49035=DIRECTION('center_axis',(1.,0.,0.));
#49036=DIRECTION('ref_axis',(0.,1.,0.));
#49037=DIRECTION('center_axis',(1.,0.,0.));
#49038=DIRECTION('ref_axis',(0.,0.,-1.));
#49039=DIRECTION('',(1.,0.,0.));
#49040=DIRECTION('center_axis',(0.,0.382683432365089,-0.923879532511287));
#49041=DIRECTION('ref_axis',(-0.707106781186563,0.653281482438174,0.270598050073092));
#49042=DIRECTION('center_axis',(-2.83242638502877E-15,-0.382683432365089,
0.923879532511287));
#49043=DIRECTION('ref_axis',(0.,0.923879532511287,0.382683432365089));
#49044=DIRECTION('center_axis',(0.,0.382683432365095,0.923879532511285));
#49045=DIRECTION('ref_axis',(-1.63551297779559E-16,0.923879532511285,-0.382683432365095));
#49046=DIRECTION('',(0.,0.382683432365089,-0.923879532511287));
#49047=DIRECTION('center_axis',(-0.706796314702699,-0.270716808310071,0.653568190184537));
#49048=DIRECTION('ref_axis',(0.,0.923879532511288,0.382683432365087));
#49049=DIRECTION('center_axis',(0.706790970016103,0.270718851822762,-0.65357312366059));
#49050=DIRECTION('ref_axis',(-0.707106781189184,0.242759667121606,-0.664129312721008));
#49051=DIRECTION('center_axis',(0.,0.,1.));
#49052=DIRECTION('ref_axis',(1.,0.,0.));
#49053=DIRECTION('center_axis',(0.,0.939220681223084,0.343314013641807));
#49054=DIRECTION('ref_axis',(0.,0.343314013641807,-0.939220681223084));
#49055=DIRECTION('center_axis',(1.,0.,0.));
#49056=DIRECTION('ref_axis',(0.,0.915660750184117,-0.401951975455104));
#49057=DIRECTION('',(-1.,0.,0.));
#49058=DIRECTION('center_axis',(1.,0.,0.));
#49059=DIRECTION('ref_axis',(0.,0.343651082071023,-0.939097403782704));
#49060=DIRECTION('',(1.,0.,0.));
#49061=DIRECTION('center_axis',(0.,0.,1.));
#49062=DIRECTION('ref_axis',(1.,0.,0.));
#49063=DIRECTION('center_axis',(0.,0.9390974037827,0.343651082071034));
#49064=DIRECTION('ref_axis',(0.,0.343651082071034,-0.9390974037827));
#49065=DIRECTION('center_axis',(1.,0.,0.));
#49066=DIRECTION('ref_axis',(0.,0.,-1.));
#49067=DIRECTION('center_axis',(-1.,0.,0.));
#49068=DIRECTION('ref_axis',(0.,0.321439465303161,-0.946930129495106));
#49069=DIRECTION('center_axis',(0.,-0.954130194262249,-0.299392004564389));
#49070=DIRECTION('ref_axis',(0.,0.299392004564389,-0.954130194262249));
#49071=DIRECTION('center_axis',(1.,0.,0.));
#49072=DIRECTION('ref_axis',(0.,1.,0.));
#49073=DIRECTION('center_axis',(1.,0.,0.));
#49074=DIRECTION('ref_axis',(0.,0.325283431446441,-0.945616565647212));
#49075=DIRECTION('center_axis',(1.,0.,0.));
#49076=DIRECTION('ref_axis',(0.,0.,-1.));
#49077=DIRECTION('center_axis',(-1.,0.,0.));
#49078=DIRECTION('ref_axis',(0.,0.325283431446441,-0.945616565647212));
#49079=DIRECTION('center_axis',(-1.52477511992402E-14,0.954237585951787,
0.299049543649384));
#49080=DIRECTION('ref_axis',(0.,0.299049543649385,-0.954237585951787));
#49081=DIRECTION('center_axis',(1.,0.,0.));
#49082=DIRECTION('ref_axis',(0.,1.,0.));
#49083=DIRECTION('center_axis',(1.,0.,0.));
#49084=DIRECTION('ref_axis',(0.,0.,-1.));
#49085=DIRECTION('',(1.,0.,0.));
#49086=DIRECTION('center_axis',(0.706790970015321,-0.183094403348123,-0.683317615876684));
#49087=DIRECTION('ref_axis',(0.,-0.965925826289066,0.258819045102528));
#49088=DIRECTION('center_axis',(-0.706796314705245,0.183093021264929,0.683312457872067));
#49089=DIRECTION('ref_axis',(-0.707106781186569,-0.154244236506505,-0.69007877485436));
#49090=DIRECTION('center_axis',(0.,0.258819045102522,0.965925826289068));
#49091=DIRECTION('ref_axis',(-0.707106781186562,-0.683012701892203,0.183012701892221));
#49092=DIRECTION('center_axis',(-9.57822876947717E-16,0.258819045102515,
0.96592582628907));
#49093=DIRECTION('ref_axis',(-1.,-3.70074341541727E-15,0.));
#49094=DIRECTION('',(0.,0.258819045102522,0.965925826289068));
#49095=DIRECTION('center_axis',(0.,-0.500000000000001,0.866025403784438));
#49096=DIRECTION('ref_axis',(8.17756488897798E-17,-0.866025403784438,-0.500000000000001));
#49097=DIRECTION('center_axis',(0.,0.,1.));
#49098=DIRECTION('ref_axis',(1.,0.,0.));
#49099=DIRECTION('center_axis',(0.,0.,1.));
#49100=DIRECTION('ref_axis',(1.,0.,0.));
#49101=DIRECTION('center_axis',(-1.,0.,0.));
#49102=DIRECTION('ref_axis',(0.,-0.855361884720259,-0.518030931670887));
#49103=DIRECTION('center_axis',(0.,-0.99144486137381,0.130526192220052));
#49104=DIRECTION('ref_axis',(-1.,0.,0.));
#49105=DIRECTION('',(-1.,0.,0.));
#49106=DIRECTION('center_axis',(0.,-0.99144486137381,0.130526192220052));
#49107=DIRECTION('ref_axis',(0.70710678118651,-0.0922959556412628,-0.701057384650015));
#49108=DIRECTION('',(0.706902428155816,0.0923226213578668,0.701259930876578));
#49109=DIRECTION('center_axis',(0.,-0.38268343236509,-0.923879532511287));
#49110=DIRECTION('ref_axis',(0.707106781186563,-0.653281482438174,0.270598050073092));
#49111=DIRECTION('center_axis',(0.,0.382683432365087,0.923879532511288));
#49112=DIRECTION('ref_axis',(0.,-0.923879532511288,0.382683432365087));
#49113=DIRECTION('center_axis',(0.,-0.382683432365086,0.923879532511288));
#49114=DIRECTION('ref_axis',(-1.6355129777956E-16,-0.923879532511288,-0.382683432365086));
#49115=DIRECTION('',(0.,-0.38268343236509,-0.923879532511286));
#49116=DIRECTION('center_axis',(0.706796314702752,0.270716808310051,0.653568190184488));
#49117=DIRECTION('ref_axis',(0.,-0.923879532511288,0.382683432365087));
#49118=DIRECTION('center_axis',(-0.706790970016056,-0.27071885182278,-0.653573123660634));
#49119=DIRECTION('ref_axis',(0.707106781189231,-0.24275966712158,-0.664129312720968));
#49120=DIRECTION('center_axis',(0.,0.,1.));
#49121=DIRECTION('ref_axis',(1.,0.,0.));
#49122=DIRECTION('center_axis',(0.,-0.939220681223083,0.343314013641808));
#49123=DIRECTION('ref_axis',(0.,-0.343314013641808,-0.939220681223083));
#49124=DIRECTION('center_axis',(-1.,0.,0.));
#49125=DIRECTION('ref_axis',(0.,-0.915660750184125,-0.401951975455086));
#49126=DIRECTION('',(1.,0.,0.));
#49127=DIRECTION('center_axis',(-1.,0.,0.));
#49128=DIRECTION('ref_axis',(0.,-0.343651082071028,-0.939097403782702));
#49129=DIRECTION('',(-1.,0.,0.));
#49130=DIRECTION('center_axis',(0.,0.,1.));
#49131=DIRECTION('ref_axis',(1.,0.,0.));
#49132=DIRECTION('center_axis',(0.,-0.9390974037827,0.343651082071035));
#49133=DIRECTION('ref_axis',(0.,-0.343651082071035,-0.9390974037827));
#49134=DIRECTION('center_axis',(1.,0.,0.));
#49135=DIRECTION('ref_axis',(0.,0.,-1.));
#49136=DIRECTION('center_axis',(1.,0.,0.));
#49137=DIRECTION('ref_axis',(0.,-0.321439465303162,-0.946930129495106));
#49138=DIRECTION('center_axis',(0.,0.95413019426225,-0.299392004564386));
#49139=DIRECTION('ref_axis',(0.,-0.299392004564386,-0.95413019426225));
#49140=DIRECTION('center_axis',(-1.,0.,0.));
#49141=DIRECTION('ref_axis',(0.,1.,0.));
#49142=DIRECTION('center_axis',(-1.,0.,0.));
#49143=DIRECTION('ref_axis',(0.,-0.325283431446442,-0.945616565647212));
#49144=DIRECTION('center_axis',(0.,-0.38268343236509,-0.923879532511287));
#49145=DIRECTION('ref_axis',(-0.707106781186566,0.653281482438171,-0.270598050073093));
#49146=DIRECTION('center_axis',(-1.36761643863197E-14,0.382683432365092,
0.923879532511286));
#49147=DIRECTION('ref_axis',(0.,0.923879532511286,-0.382683432365092));
#49148=DIRECTION('center_axis',(0.,0.923879532511289,0.382683432365084));
#49149=DIRECTION('ref_axis',(-1.22663473334669E-16,0.382683432365084,-0.923879532511289));
#49150=DIRECTION('',(0.,-0.38268343236509,-0.923879532511286));
#49151=DIRECTION('center_axis',(-0.706796314702669,0.270716808310082,0.653568190184565));
#49152=DIRECTION('ref_axis',(0.,0.923879532511288,-0.382683432365087));
#49153=DIRECTION('center_axis',(0.706790970015992,-0.270718851822805,-0.653573123660694));
#49154=DIRECTION('ref_axis',(-0.707106781189295,-0.297953333789474,-0.641267347429957));
#49155=DIRECTION('center_axis',(0.,0.,1.));
#49156=DIRECTION('ref_axis',(-0.833158187746095,0.553034749533556,0.));
#49157=DIRECTION('center_axis',(0.,0.906888979845984,-0.421369645600999));
#49158=DIRECTION('ref_axis',(0.,-0.421369645600999,-0.906888979845984));
#49159=DIRECTION('center_axis',(1.,0.,0.));
#49160=DIRECTION('ref_axis',(0.,0.363246958165936,-0.931692893277176));
#49161=DIRECTION('',(-1.,0.,0.));
#49162=DIRECTION('center_axis',(1.,0.,0.));
#49163=DIRECTION('ref_axis',(0.,-0.421044131914909,-0.90704015290395));
#49164=DIRECTION('',(1.,0.,0.));
#49165=DIRECTION('center_axis',(-0.0341251959389409,-0.995062857517424,
-0.0931953893247336));
#49166=DIRECTION('ref_axis',(-0.342144487581495,0.0992467107226253,-0.934391374119183));
#49167=DIRECTION('center_axis',(0.,0.907040152903951,-0.421044131914906));
#49168=DIRECTION('ref_axis',(0.,-0.421044131914906,-0.907040152903951));
#49169=DIRECTION('center_axis',(1.,0.,0.));
#49170=DIRECTION('ref_axis',(0.,0.,-1.));
#49171=DIRECTION('center_axis',(-1.,0.,0.));
#49172=DIRECTION('ref_axis',(0.,-0.442288690219002,-0.896872741532688));
#49173=DIRECTION('center_axis',(0.,-0.886374047158188,0.462969813837161));
#49174=DIRECTION('ref_axis',(0.,-0.462969813837161,-0.886374047158187));
#49175=DIRECTION('center_axis',(1.,0.,0.));
#49176=DIRECTION('ref_axis',(0.,1.,0.));
#49177=DIRECTION('center_axis',(1.,0.,0.));
#49178=DIRECTION('ref_axis',(0.,-0.43864176578807,-0.898662006154886));
#49179=DIRECTION('center_axis',(1.,0.,0.));
#49180=DIRECTION('ref_axis',(0.,0.,-1.));
#49181=DIRECTION('center_axis',(-1.,0.,0.));
#49182=DIRECTION('ref_axis',(0.,-0.43864176578807,-0.898662006154886));
#49183=DIRECTION('center_axis',(-4.33581305051025E-14,0.886207828114814,
-0.463287907664363));
#49184=DIRECTION('ref_axis',(0.,-0.463287907664363,-0.886207828114814));
#49185=DIRECTION('center_axis',(1.,0.,0.));
#49186=DIRECTION('ref_axis',(0.,1.,0.));
#49187=DIRECTION('center_axis',(1.,0.,0.));
#49188=DIRECTION('ref_axis',(0.,0.,-1.));
#49189=DIRECTION('',(1.,0.,0.));
#49190=DIRECTION('center_axis',(0.706790970016481,-0.430651502409207,-0.561235964791864));
#49191=DIRECTION('ref_axis',(0.,-0.793353340291235,0.608761429008721));
#49192=DIRECTION('center_axis',(-0.70679631470526,0.430648251648679,0.561231728318169));
#49193=DIRECTION('ref_axis',(-0.707106781186552,-0.40658480727975,-0.578522942059589));
#49194=DIRECTION('center_axis',(0.,0.608761429008721,0.793353340291235));
#49195=DIRECTION('ref_axis',(-0.707106781186563,-0.560985526796918,0.430459334576872));
#49196=DIRECTION('center_axis',(0.,0.608761429008712,0.793353340291242));
#49197=DIRECTION('ref_axis',(-1.,0.,0.));
#49198=DIRECTION('center_axis',(0.,-0.130526192220042,0.991444861373812));
#49199=DIRECTION('ref_axis',(-1.22663473334671E-16,-0.991444861373812,-0.130526192220042));
#49200=DIRECTION('center_axis',(0.,0.,1.));
#49201=DIRECTION('ref_axis',(1.,0.,0.));
#49202=DIRECTION('center_axis',(0.,0.,1.));
#49203=DIRECTION('ref_axis',(1.,0.,0.));
#49204=DIRECTION('center_axis',(0.,-0.707106781186548,-0.707106781186547));
#49205=DIRECTION('ref_axis',(0.707106781186559,-0.499999999999992,0.499999999999992));
#49206=DIRECTION('center_axis',(-1.04672830578914E-14,0.707106781186548,
0.707106781186548));
#49207=DIRECTION('ref_axis',(0.,-0.707106781186548,0.707106781186548));
#49208=DIRECTION('center_axis',(0.,0.,1.));
#49209=DIRECTION('ref_axis',(-1.6355129777956E-16,-1.,-2.89120579329473E-17));
#49210=DIRECTION('',(0.,-0.707106781186548,-0.707106781186547));
#49211=DIRECTION('center_axis',(0.706796314703398,0.500219436608423,0.500219436608423));
#49212=DIRECTION('ref_axis',(0.,-0.707106781186547,0.707106781186547));
#49213=DIRECTION('center_axis',(-0.706790970016695,-0.500223212527598,-0.500223212527598));
#49214=DIRECTION('ref_axis',(0.707106781188592,-0.478431972699633,-0.520675376310275));
#49215=DIRECTION('center_axis',(0.,0.,1.));
#49216=DIRECTION('ref_axis',(1.,0.,0.));
#49217=DIRECTION('center_axis',(0.,-0.736346178773832,0.676604984466694));
#49218=DIRECTION('ref_axis',(0.,-0.676604984466694,-0.736346178773832));
#49219=DIRECTION('center_axis',(-1.,0.,0.));
#49220=DIRECTION('ref_axis',(0.,-0.999780587432124,-0.0209470044129764));
#49221=DIRECTION('',(1.,0.,0.));
#49222=DIRECTION('center_axis',(-1.,0.,0.));
#49223=DIRECTION('ref_axis',(0.,-0.676869218855494,-0.736103294766403));
#49224=DIRECTION('',(-1.,0.,0.));
#49225=DIRECTION('center_axis',(0.,0.,1.));
#49226=DIRECTION('ref_axis',(1.,0.,0.));
#49227=DIRECTION('center_axis',(0.,-0.736103294766404,0.676869218855493));
#49228=DIRECTION('ref_axis',(0.,-0.676869218855493,-0.736103294766404));
#49229=DIRECTION('center_axis',(1.,0.,0.));
#49230=DIRECTION('ref_axis',(0.,0.,-1.));
#49231=DIRECTION('center_axis',(1.,0.,0.));
#49232=DIRECTION('ref_axis',(0.,-0.659345815100069,-0.751839807478977));
#49233=DIRECTION('center_axis',(0.,0.766928997900546,-0.641731962878011));
#49234=DIRECTION('ref_axis',(0.,-0.641731962878011,-0.766928997900546));
#49235=DIRECTION('center_axis',(-1.,0.,0.));
#49236=DIRECTION('ref_axis',(0.,1.,0.));
#49237=DIRECTION('center_axis',(-1.,0.,0.));
#49238=DIRECTION('ref_axis',(0.,-0.66239449762157,-0.749155210567655));
#49239=DIRECTION('center_axis',(-0.706790970016593,-0.430651502409139,-0.561235964791775));
#49240=DIRECTION('ref_axis',(0.,0.793353340291235,-0.608761429008721));
#49241=DIRECTION('center_axis',(0.706796314705252,0.430648251648626,0.56123172831822));
#49242=DIRECTION('ref_axis',(0.707106781186562,-0.453578359262743,-0.542463521362034));
#49243=DIRECTION('center_axis',(1.,0.,0.));
#49244=DIRECTION('ref_axis',(0.,0.,-1.));
#49245=DIRECTION('center_axis',(1.,0.,0.));
#49246=DIRECTION('ref_axis',(0.,-0.66239449762157,-0.749155210567655));
#49247=DIRECTION('center_axis',(-2.52993413752754E-14,-0.767159269002869,
0.641456667268323));
#49248=DIRECTION('ref_axis',(0.,-0.641456667268323,-0.767159269002869));
#49249=DIRECTION('center_axis',(-0.0504847333736788,-0.989288526783087,
0.136965333101256));
#49250=DIRECTION('ref_axis',(0.342144487592337,-0.145973322135758,-0.92823969901897));
#49251=DIRECTION('center_axis',(1.,0.,0.));
#49252=DIRECTION('ref_axis',(0.,0.10972975324662,-0.993961458635311));
#49253=DIRECTION('center_axis',(0.,0.608761429008721,0.793353340291235));
#49254=DIRECTION('ref_axis',(0.707106781186562,0.560985526796919,-0.430459334576871));
#49255=DIRECTION('center_axis',(0.,0.608761429008721,0.793353340291235));
#49256=DIRECTION('ref_axis',(1.,0.,0.));
#49257=DIRECTION('',(0.,0.608761429008721,0.793353340291235));
#49258=DIRECTION('center_axis',(0.,0.991444861373809,0.13052619222006));
#49259=DIRECTION('ref_axis',(-1.22663473334671E-16,0.13052619222006,-0.991444861373809));
#49260=DIRECTION('center_axis',(0.,0.,1.));
#49261=DIRECTION('ref_axis',(1.,0.,0.));
#49262=DIRECTION('center_axis',(0.,0.707106781186547,-0.707106781186548));
#49263=DIRECTION('ref_axis',(1.,0.,0.));
#49264=DIRECTION('',(1.,0.,0.));
#49265=DIRECTION('center_axis',(0.,0.707106781186547,-0.707106781186548));
#49266=DIRECTION('ref_axis',(-0.707106781186559,-0.499999999999986,-0.499999999999997));
#49267=DIRECTION('',(-0.706902428155818,0.500144457665694,0.500144457665681));
#49268=DIRECTION('center_axis',(0.706790970016296,-0.353711225685386,-0.612645814094543));
#49269=DIRECTION('ref_axis',(0.,-0.866025403784436,0.500000000000005));
#49270=DIRECTION('center_axis',(-0.706796314705255,0.353708555706203,0.612641189554949));
#49271=DIRECTION('ref_axis',(-0.707106781186559,-0.32759402115119,-0.626643564800579));
#49272=DIRECTION('center_axis',(0.,0.5,0.866025403784438));
#49273=DIRECTION('ref_axis',(-0.70710678118656,-0.612372435695783,0.35355339059327));
#49274=DIRECTION('center_axis',(-3.7007434154173E-15,0.500000000000005,
0.866025403784436));
#49275=DIRECTION('ref_axis',(-1.,-7.40148683083454E-15,0.));
#49276=DIRECTION('',(0.,0.5,0.866025403784438));
#49277=DIRECTION('center_axis',(0.,-0.258819045102521,0.965925826289068));
#49278=DIRECTION('ref_axis',(-8.17756488897799E-17,-0.965925826289068,-0.258819045102521));
#49279=DIRECTION('center_axis',(0.,0.,1.));
#49280=DIRECTION('ref_axis',(1.,0.,0.));
#49281=DIRECTION('center_axis',(0.,0.,1.));
#49282=DIRECTION('ref_axis',(1.,0.,0.));
#49283=DIRECTION('center_axis',(-1.,0.,0.));
#49284=DIRECTION('ref_axis',(0.,-0.96029240634322,-0.278995509497105));
#49285=DIRECTION('center_axis',(0.,-0.923879532511287,0.38268343236509));
#49286=DIRECTION('ref_axis',(-1.,0.,0.));
#49287=DIRECTION('',(-1.,0.,0.));
#49288=DIRECTION('center_axis',(0.,-0.923879532511287,0.38268343236509));
#49289=DIRECTION('ref_axis',(0.707106781186517,-0.270598050073114,-0.653281482438214));
#49290=DIRECTION('',(0.706902428155814,0.270676229998409,0.65347022547417));
#49291=DIRECTION('center_axis',(-0.706790970015228,-0.183094403348147,-0.683317615876775));
#49292=DIRECTION('ref_axis',(0.,0.965925826289067,-0.258819045102527));
#49293=DIRECTION('center_axis',(0.706796314705254,0.183093021264956,0.683312457872049));
#49294=DIRECTION('ref_axis',(0.70710678118656,-0.211459960225217,-0.674747867889578));
#49295=DIRECTION('center_axis',(1.,0.,0.));
#49296=DIRECTION('ref_axis',(0.,0.,-1.));
#49297=DIRECTION('center_axis',(1.,0.,0.));
#49298=DIRECTION('ref_axis',(0.,-0.325283431446442,-0.945616565647212));
#49299=DIRECTION('center_axis',(2.23179375095024E-14,-0.954237585951785,
0.299049543649391));
#49300=DIRECTION('ref_axis',(0.,-0.299049543649391,-0.954237585951785));
#49301=DIRECTION('center_axis',(0.0772950468865004,-0.975418570101725,-0.206359125864401));
#49302=DIRECTION('ref_axis',(0.342144487592387,0.220360189464224,-0.913443231136689));
#49303=DIRECTION('center_axis',(1.,0.,0.));
#49304=DIRECTION('ref_axis',(0.,0.481749655761233,-0.87630888913324));
#49305=DIRECTION('center_axis',(0.,0.258819045102522,0.965925826289068));
#49306=DIRECTION('ref_axis',(0.707106781186561,0.683012701892208,-0.18301270189221));
#49307=DIRECTION('center_axis',(0.,0.258819045102527,0.965925826289067));
#49308=DIRECTION('ref_axis',(1.,0.,0.));
#49309=DIRECTION('',(0.,0.258819045102522,0.965925826289068));
#49310=DIRECTION('center_axis',(0.,0.866025403784442,0.499999999999995));
#49311=DIRECTION('ref_axis',(2.45326946669339E-16,0.499999999999995,-0.866025403784442));
#49312=DIRECTION('center_axis',(0.,0.,1.));
#49313=DIRECTION('ref_axis',(1.,0.,0.));
#49314=DIRECTION('center_axis',(0.,0.923879532511287,-0.38268343236509));
#49315=DIRECTION('ref_axis',(1.,0.,0.));
#49316=DIRECTION('',(1.,0.,0.));
#49317=DIRECTION('center_axis',(0.,0.923879532511287,-0.38268343236509));
#49318=DIRECTION('ref_axis',(-0.70710678118656,-0.270598050073094,-0.653281482438177));
#49319=DIRECTION('',(-0.706902428155812,0.270676229998407,0.653470225474173));
#49320=DIRECTION('center_axis',(-1.,0.,0.));
#49321=DIRECTION('ref_axis',(0.,-0.855361884720258,-0.518030931670888));
#49322=DIRECTION('',(-1.,0.,0.));
#49323=DIRECTION('center_axis',(0.,0.965925826289068,-0.258819045102522));
#49324=DIRECTION('ref_axis',(1.,0.,0.));
#49325=DIRECTION('',(-0.706902428155817,-0.183065577067631,-0.683210034733321));
#49326=DIRECTION('center_axis',(0.,0.965925826289068,-0.258819045102522));
#49327=DIRECTION('ref_axis',(0.707106781186523,-0.183012701892228,-0.683012701892242));
#49328=DIRECTION('',(1.,0.,0.));
#49329=DIRECTION('center_axis',(0.706790970015237,0.183094403348135,-0.683317615876769));
#49330=DIRECTION('ref_axis',(0.,-0.96592582628907,-0.258819045102513));
#49331=DIRECTION('center_axis',(-0.706796314705248,-0.183093021264939,0.683312457872061));
#49332=DIRECTION('ref_axis',(-0.707106781186566,0.211459960225227,-0.674747867889569));
#49333=DIRECTION('center_axis',(0.,-0.25881904510252,0.965925826289068));
#49334=DIRECTION('ref_axis',(-0.707106781186562,-0.68301270189221,-0.1830127018922));
#49335=DIRECTION('center_axis',(0.,-0.258819045102513,0.96592582628907));
#49336=DIRECTION('ref_axis',(-1.,0.,0.));
#49337=DIRECTION('',(0.,-0.25881904510252,0.965925826289068));
#49338=DIRECTION('center_axis',(0.,-0.866025403784435,0.500000000000007));
#49339=DIRECTION('ref_axis',(-8.17756488897806E-17,-0.500000000000007,-0.866025403784435));
#49340=DIRECTION('center_axis',(0.,0.,1.));
#49341=DIRECTION('ref_axis',(-0.802126387103182,-0.597154300924641,0.));
#49342=DIRECTION('center_axis',(0.0772950468865003,-0.97541857010173,0.206359125864377));
#49343=DIRECTION('ref_axis',(-0.342144487592388,-0.220360189464213,-0.913443231136691));
#49344=DIRECTION('center_axis',(-1.,0.,0.));
#49345=DIRECTION('ref_axis',(0.,-0.481749655761233,-0.87630888913324));
#49346=DIRECTION('center_axis',(0.,-0.923879532511287,-0.382683432365089));
#49347=DIRECTION('ref_axis',(-1.,0.,0.));
#49348=DIRECTION('',(-1.,0.,0.));
#49349=DIRECTION('center_axis',(0.,-0.923879532511287,-0.382683432365089));
#49350=DIRECTION('ref_axis',(0.707106781186519,0.270598050073107,-0.653281482438216));
#49351=DIRECTION('',(0.706902428155815,-0.270676229998406,0.65347022547417));
#49352=DIRECTION('center_axis',(0.706790970014446,0.092337158868645,-0.701370354233842));
#49353=DIRECTION('ref_axis',(0.,-0.99144486137381,-0.130526192220056));
#49354=DIRECTION('center_axis',(-0.706796314705254,-0.0923364618639724,
0.701365059957734));
#49355=DIRECTION('ref_axis',(-0.70710678118656,0.121578621047381,-0.696576369757257));
#49356=DIRECTION('center_axis',(0.,-0.130526192220051,0.99144486137381));
#49357=DIRECTION('ref_axis',(-0.70710678118656,-0.701057384649966,-0.092295955641248));
#49358=DIRECTION('center_axis',(-4.83043946397914E-16,-0.13052619222007,
0.991444861373808));
#49359=DIRECTION('ref_axis',(-1.,3.70074341541727E-15,0.));
#49360=DIRECTION('',(0.,-0.130526192220051,0.991444861373811));
#49361=DIRECTION('center_axis',(0.,-0.793353340291231,0.608761429008727));
#49362=DIRECTION('ref_axis',(1.63551297779561E-16,-0.608761429008727,-0.793353340291231));
#49363=DIRECTION('center_axis',(0.,0.,1.));
#49364=DIRECTION('ref_axis',(-0.764784300456357,-0.644286406635652,0.));
#49365=DIRECTION('center_axis',(0.122754826320915,-0.941252632831819,0.314602501264835));
#49366=DIRECTION('ref_axis',(-0.342144487592387,-0.337703244265098,-0.876865821219513));
#49367=DIRECTION('center_axis',(-1.,0.,0.));
#49368=DIRECTION('ref_axis',(0.,-0.592009483180216,-0.805930996937513));
#49369=DIRECTION('center_axis',(0.,-0.965925826289068,-0.25881904510252));
#49370=DIRECTION('ref_axis',(-1.,0.,0.));
#49371=DIRECTION('',(-1.,0.,0.));
#49372=DIRECTION('center_axis',(0.,-0.965925826289068,-0.25881904510252));
#49373=DIRECTION('ref_axis',(0.707106781186512,0.18301270189223,-0.683012701892253));
#49374=DIRECTION('',(0.70690242815582,-0.183065577067634,0.683210034733317));
#49375=DIRECTION('center_axis',(0.,-1.83697019872103E-16,-1.));
#49376=DIRECTION('ref_axis',(-0.707106781186561,0.707106781186534,0.));
#49377=DIRECTION('center_axis',(0.,0.,1.));
#49378=DIRECTION('ref_axis',(0.,1.,0.));
#49379=DIRECTION('center_axis',(0.,0.707106781186543,0.707106781186552));
#49380=DIRECTION('ref_axis',(4.08878244448902E-17,0.707106781186552,-0.707106781186543));
#49381=DIRECTION('',(0.,-1.83697019872103E-16,-1.));
#49382=DIRECTION('center_axis',(-0.706796314700263,0.,0.707417111417392));
#49383=DIRECTION('ref_axis',(0.,1.,0.));
#49384=DIRECTION('center_axis',(0.706790970013424,0.,-0.707422451373635));
#49385=DIRECTION('ref_axis',(-0.707106781191861,-0.0298705971533384,-0.706475581614954));
#49386=DIRECTION('center_axis',(0.,0.,1.));
#49387=DIRECTION('ref_axis',(-0.721874560494001,0.692023929435676,0.));
#49388=DIRECTION('center_axis',(0.,0.999107349012797,-0.0422434036107611));
#49389=DIRECTION('ref_axis',(0.,-0.0422434036107611,-0.999107349012797));
#49390=DIRECTION('center_axis',(1.,0.,0.));
#49391=DIRECTION('ref_axis',(0.,0.692139864205961,-0.721763401937888));
#49392=DIRECTION('',(-1.,0.,0.));
#49393=DIRECTION('center_axis',(1.,0.,0.));
#49394=DIRECTION('ref_axis',(0.,-0.0418848167539264,-0.999122446012244));
#49395=DIRECTION('',(1.,0.,0.));
#49396=DIRECTION('center_axis',(-0.172056328312398,-0.89339698437742,-0.415016202325872));
#49397=DIRECTION('ref_axis',(-0.342144487571549,0.449268102924446,-0.82528499399848));
#49398=DIRECTION('center_axis',(0.,0.999122446012245,-0.0418848167539204));
#49399=DIRECTION('ref_axis',(0.,-0.0418848167539204,-0.999122446012244));
#49400=DIRECTION('center_axis',(1.,0.,0.));
#49401=DIRECTION('ref_axis',(0.,0.,-1.));
#49402=DIRECTION('center_axis',(-1.,0.,0.));
#49403=DIRECTION('ref_axis',(0.,-0.0654031292301436,-0.997858923238603));
#49404=DIRECTION('center_axis',(0.,-0.996073717759275,0.0885276724488825));
#49405=DIRECTION('ref_axis',(0.,-0.0885276724488825,-0.996073717759275));
#49406=DIRECTION('center_axis',(1.,0.,0.));
#49407=DIRECTION('ref_axis',(0.,1.,0.));
#49408=DIRECTION('center_axis',(1.,0.,0.));
#49409=DIRECTION('ref_axis',(0.,-0.0613490884647577,-0.998116370642493));
#49410=DIRECTION('center_axis',(1.,0.,0.));
#49411=DIRECTION('ref_axis',(0.,0.,-1.));
#49412=DIRECTION('center_axis',(-1.,0.,0.));
#49413=DIRECTION('ref_axis',(0.,-0.0613490884647577,-0.998116370642493));
#49414=DIRECTION('center_axis',(1.56523702953091E-14,0.996041880624797,
-0.088885162099298));
#49415=DIRECTION('ref_axis',(0.,-0.088885162099298,-0.996041880624797));
#49416=DIRECTION('center_axis',(1.,0.,0.));
#49417=DIRECTION('ref_axis',(0.,1.,0.));
#49418=DIRECTION('center_axis',(1.,0.,0.));
#49419=DIRECTION('ref_axis',(0.,0.,-1.));
#49420=DIRECTION('',(1.,0.,0.));
#49421=DIRECTION('center_axis',(0.70679097001436,-0.0923371588686562,-0.701370354233927));
#49422=DIRECTION('ref_axis',(0.,-0.99144486137381,0.130526192220056));
#49423=DIRECTION('center_axis',(-0.706796314705253,0.0923364618639724,0.701365059957734));
#49424=DIRECTION('ref_axis',(-0.707106781186561,-0.0628513008672803,-0.704307968135582));
#49425=DIRECTION('center_axis',(0.,0.130526192220052,0.99144486137381));
#49426=DIRECTION('ref_axis',(-0.707106781186557,-0.701057384649968,0.092295955641258));
#49427=DIRECTION('center_axis',(-2.41521973198928E-16,0.130526192220055,
0.99144486137381));
#49428=DIRECTION('ref_axis',(-1.,-1.85037170770863E-15,0.));
#49429=DIRECTION('',(0.,0.130526192220052,0.99144486137381));
#49430=DIRECTION('center_axis',(0.,-0.608761429008706,0.793353340291247));
#49431=DIRECTION('ref_axis',(-1.22663473334672E-16,-0.793353340291247,-0.608761429008706));
#49432=DIRECTION('center_axis',(0.,0.,1.));
#49433=DIRECTION('ref_axis',(1.,0.,0.));
#49434=DIRECTION('center_axis',(0.,0.,1.));
#49435=DIRECTION('ref_axis',(1.,0.,0.));
#49436=DIRECTION('center_axis',(-1.,0.,0.));
#49437=DIRECTION('ref_axis',(0.,-0.780427540257703,-0.625246235020501));
#49438=DIRECTION('center_axis',(0.,-1.,1.83697019872103E-16));
#49439=DIRECTION('ref_axis',(-1.,0.,0.));
#49440=DIRECTION('',(-1.,0.,0.));
#49441=DIRECTION('center_axis',(0.,-1.,1.83697019872103E-16));
#49442=DIRECTION('ref_axis',(0.707106781186516,0.,-0.707106781186579));
#49443=DIRECTION('',(0.706902428155817,0.,0.707311075176552));
#49444=DIRECTION('center_axis',(-1.,0.,0.));
#49445=DIRECTION('ref_axis',(0.,-0.592009483180217,-0.805930996937512));
#49446=DIRECTION('',(-1.,0.,0.));
#49447=DIRECTION('center_axis',(0.,0.99144486137381,0.130526192220051));
#49448=DIRECTION('ref_axis',(1.,0.,0.));
#49449=DIRECTION('',(-0.706902428155813,0.0923226213578633,-0.701259930876582));
#49450=DIRECTION('center_axis',(0.,0.99144486137381,0.130526192220051));
#49451=DIRECTION('ref_axis',(0.707106781186521,0.0922959556412538,-0.701057384650005));
#49452=DIRECTION('',(1.,0.,0.));
#49453=DIRECTION('center_axis',(-1.,0.,0.));
#49454=DIRECTION('ref_axis',(0.,-0.481749655761234,-0.87630888913324));
#49455=DIRECTION('',(-1.,0.,0.));
#49456=DIRECTION('center_axis',(0.,0.965925826289068,0.25881904510252));
#49457=DIRECTION('ref_axis',(1.,0.,0.));
#49458=DIRECTION('',(-0.706902428155816,0.183065577067636,-0.68321003473332));
#49459=DIRECTION('center_axis',(0.,0.965925826289068,0.25881904510252));
#49460=DIRECTION('ref_axis',(0.707106781186512,0.18301270189223,-0.683012701892253));
#49461=DIRECTION('',(1.,0.,0.));
#49462=DIRECTION('center_axis',(0.,0.866025403784438,-0.5));
#49463=DIRECTION('ref_axis',(-0.707106781186561,0.35355339059326,0.612372435695786));
#49464=DIRECTION('center_axis',(0.,-0.866025403784442,0.499999999999995));
#49465=DIRECTION('ref_axis',(0.,0.499999999999995,0.866025403784442));
#49466=DIRECTION('center_axis',(0.,-0.25881904510251,0.965925826289071));
#49467=DIRECTION('ref_axis',(0.,0.965925826289071,0.25881904510251));
#49468=DIRECTION('',(0.,0.866025403784438,-0.5));
#49469=DIRECTION('center_axis',(-0.706796314703074,-0.612641189556835,0.353708555707293));
#49470=DIRECTION('ref_axis',(0.,0.500000000000001,0.866025403784438));
#49471=DIRECTION('center_axis',(0.706790970016345,0.612645814094502,-0.353711225685359));
#49472=DIRECTION('ref_axis',(-0.707106781188942,0.596890502257736,-0.37910648677004));
#49473=DIRECTION('center_axis',(0.,0.,1.));
#49474=DIRECTION('ref_axis',(1.,0.,0.));
#49475=DIRECTION('center_axis',(0.,0.536137535175637,0.844130643547427));
#49476=DIRECTION('ref_axis',(0.,0.844130643547427,-0.536137535175637));
#49477=DIRECTION('center_axis',(1.,0.,0.));
#49478=DIRECTION('ref_axis',(0.,0.971135373703069,0.238529004405333));
#49479=DIRECTION('',(-1.,0.,0.));
#49480=DIRECTION('center_axis',(1.,0.,0.));
#49481=DIRECTION('ref_axis',(0.,0.844323011360887,-0.535834538347879));
#49482=DIRECTION('',(1.,0.,0.));
#49483=DIRECTION('center_axis',(0.,0.,1.));
#49484=DIRECTION('ref_axis',(1.,0.,0.));
#49485=DIRECTION('center_axis',(0.,0.535834538347877,0.844323011360888));
#49486=DIRECTION('ref_axis',(0.,0.844323011360888,-0.535834538347877));
#49487=DIRECTION('center_axis',(1.,0.,0.));
#49488=DIRECTION('ref_axis',(0.,0.,-1.));
#49489=DIRECTION('center_axis',(-1.,0.,0.));
#49490=DIRECTION('ref_axis',(0.,0.831469612302545,-0.555570233019602));
#49491=DIRECTION('center_axis',(0.,-0.574704072158277,-0.818361307397102));
#49492=DIRECTION('ref_axis',(0.,0.818361307397102,-0.574704072158277));
#49493=DIRECTION('center_axis',(1.,0.,0.));
#49494=DIRECTION('ref_axis',(0.,1.,0.));
#49495=DIRECTION('center_axis',(1.,-2.55357611039623E-16,-3.85550974406735E-16));
#49496=DIRECTION('ref_axis',(0.,0.833719588677145,-0.552188054430745));
#49497=DIRECTION('center_axis',(1.,0.,0.));
#49498=DIRECTION('ref_axis',(0.,0.,-1.));
#49499=DIRECTION('center_axis',(-1.,0.,0.));
#49500=DIRECTION('ref_axis',(0.,0.833719588677145,-0.552188054430745));
#49501=DIRECTION('center_axis',(-1.15848835927189E-14,0.574997748709887,
0.818154990804653));
#49502=DIRECTION('ref_axis',(0.,0.818154990804653,-0.574997748709887));
#49503=DIRECTION('center_axis',(1.,0.,0.));
#49504=DIRECTION('ref_axis',(0.,1.,0.));
#49505=DIRECTION('center_axis',(1.,0.,0.));
#49506=DIRECTION('ref_axis',(0.,0.,-1.));
#49507=DIRECTION('',(1.,0.,0.));
#49508=DIRECTION('center_axis',(0.,0.923879532511287,-0.38268343236509));
#49509=DIRECTION('ref_axis',(0.707106781186561,-0.270598050073091,-0.653281482438177));
#49510=DIRECTION('center_axis',(-2.8324263850286E-15,-0.923879532511287,
0.382683432365089));
#49511=DIRECTION('ref_axis',(0.,-0.382683432365089,-0.923879532511287));
#49512=DIRECTION('center_axis',(0.,-0.923879532511286,-0.382683432365091));
#49513=DIRECTION('ref_axis',(8.17756488897798E-17,0.382683432365091,-0.923879532511286));
#49514=DIRECTION('',(0.,0.923879532511286,-0.38268343236509));
#49515=DIRECTION('center_axis',(0.706796314702699,-0.653568190184537,0.270716808310071));
#49516=DIRECTION('ref_axis',(0.,-0.382683432365087,-0.923879532511288));
#49517=DIRECTION('center_axis',(-0.706790970016047,0.653573123660642,-0.270718851822783));
#49518=DIRECTION('ref_axis',(0.707106781189239,0.66412931272096,-0.242759667121575));
#49519=DIRECTION('center_axis',(0.,0.,1.));
#49520=DIRECTION('ref_axis',(1.,0.,0.));
#49521=DIRECTION('center_axis',(0.,-0.343314013641808,-0.939220681223083));
#49522=DIRECTION('ref_axis',(0.,0.939220681223083,-0.343314013641808));
#49523=DIRECTION('center_axis',(-1.,0.,0.));
#49524=DIRECTION('ref_axis',(0.,0.401951975455096,-0.91566075018412));
#49525=DIRECTION('',(1.,0.,0.));
#49526=DIRECTION('center_axis',(-1.,0.,0.));
#49527=DIRECTION('ref_axis',(0.,0.9390974037827,-0.343651082071033));
#49528=DIRECTION('',(-1.,0.,0.));
#49529=DIRECTION('center_axis',(0.250366849757598,-0.807010963742299,-0.534836185146613));
#49530=DIRECTION('ref_axis',(0.342144487581777,0.590536454759322,-0.730892499084301));
#49531=DIRECTION('center_axis',(0.,-0.343651082071035,-0.9390974037827));
#49532=DIRECTION('ref_axis',(0.,0.9390974037827,-0.343651082071035));
#49533=DIRECTION('center_axis',(1.,0.,0.));
#49534=DIRECTION('ref_axis',(0.,0.,-1.));
#49535=DIRECTION('center_axis',(1.,0.,0.));
#49536=DIRECTION('ref_axis',(0.,0.946930129495106,-0.321439465303162));
#49537=DIRECTION('center_axis',(0.,0.299392004564386,0.95413019426225));
#49538=DIRECTION('ref_axis',(0.,0.95413019426225,-0.299392004564386));
#49539=DIRECTION('center_axis',(-1.,0.,0.));
#49540=DIRECTION('ref_axis',(0.,1.,0.));
#49541=DIRECTION('center_axis',(-1.,1.5042628919339E-16,4.37297375822624E-16));
#49542=DIRECTION('ref_axis',(0.,0.945616565647212,-0.325283431446443));
#49543=DIRECTION('center_axis',(0.,0.923879532511287,-0.38268343236509));
#49544=DIRECTION('ref_axis',(-0.707106781186561,0.270598050073091,0.653281482438177));
#49545=DIRECTION('center_axis',(0.,-0.923879532511288,0.382683432365087));
#49546=DIRECTION('ref_axis',(0.,0.382683432365087,0.923879532511288));
#49547=DIRECTION('center_axis',(0.,-0.382683432365089,0.923879532511287));
#49548=DIRECTION('ref_axis',(1.6355129777956E-16,0.923879532511287,0.382683432365089));
#49549=DIRECTION('',(0.,0.923879532511286,-0.38268343236509));
#49550=DIRECTION('center_axis',(-0.706796314702688,-0.653568190184547,0.270716808310075));
#49551=DIRECTION('ref_axis',(0.,0.382683432365087,0.923879532511288));
#49552=DIRECTION('center_axis',(0.706790970015985,0.6535731236607,-0.270718851822807));
#49553=DIRECTION('ref_axis',(-0.707106781189301,0.641267347429948,-0.297953333789477));
#49554=DIRECTION('center_axis',(0.,0.,1.));
#49555=DIRECTION('ref_axis',(1.,0.,0.));
#49556=DIRECTION('center_axis',(0.,0.421369645600999,0.906888979845984));
#49557=DIRECTION('ref_axis',(0.,0.906888979845984,-0.421369645600999));
#49558=DIRECTION('center_axis',(1.,0.,0.));
#49559=DIRECTION('ref_axis',(0.,0.931692893277172,0.363246958165945));
#49560=DIRECTION('',(-1.,0.,0.));
#49561=DIRECTION('center_axis',(1.,0.,0.));
#49562=DIRECTION('ref_axis',(0.,0.907040152903953,-0.421044131914903));
#49563=DIRECTION('',(1.,0.,0.));
#49564=DIRECTION('center_axis',(0.,0.,1.));
#49565=DIRECTION('ref_axis',(1.,0.,0.));
#49566=DIRECTION('center_axis',(0.,0.421044131914906,0.907040152903951));
#49567=DIRECTION('ref_axis',(0.,0.907040152903951,-0.421044131914906));
#49568=DIRECTION('center_axis',(1.,0.,0.));
#49569=DIRECTION('ref_axis',(0.,0.,-1.));
#49570=DIRECTION('center_axis',(-1.,0.,0.));
#49571=DIRECTION('ref_axis',(0.,0.896872741532688,-0.442288690219002));
#49572=DIRECTION('center_axis',(0.,-0.462969813837161,-0.886374047158187));
#49573=DIRECTION('ref_axis',(0.,0.886374047158187,-0.462969813837161));
#49574=DIRECTION('center_axis',(1.,0.,0.));
#49575=DIRECTION('ref_axis',(0.,1.,0.));
#49576=DIRECTION('center_axis',(1.,0.,0.));
#49577=DIRECTION('ref_axis',(0.,0.898662006154886,-0.43864176578807));
#49578=DIRECTION('center_axis',(1.,0.,0.));
#49579=DIRECTION('ref_axis',(0.,0.,-1.));
#49580=DIRECTION('center_axis',(-1.,0.,0.));
#49581=DIRECTION('ref_axis',(0.,0.898662006154886,-0.43864176578807));
#49582=DIRECTION('center_axis',(-1.58440319723961E-14,0.463287907664363,
0.886207828114815));
#49583=DIRECTION('ref_axis',(0.,0.886207828114815,-0.463287907664363));
#49584=DIRECTION('center_axis',(1.,0.,0.));
#49585=DIRECTION('ref_axis',(0.,1.,0.));
#49586=DIRECTION('center_axis',(1.,0.,0.));
#49587=DIRECTION('ref_axis',(0.,0.,-1.));
#49588=DIRECTION('',(1.,0.,0.));
#49589=DIRECTION('center_axis',(0.,0.60876142900872,-0.793353340291236));
#49590=DIRECTION('ref_axis',(-0.707106781186558,0.560985526796926,0.430459334576869));
#49591=DIRECTION('center_axis',(0.,-0.608761429008714,0.79335334029124));
#49592=DIRECTION('ref_axis',(0.,0.79335334029124,0.608761429008714));
#49593=DIRECTION('center_axis',(0.,0.130526192220061,0.991444861373809));
#49594=DIRECTION('ref_axis',(-1.22663473334669E-16,0.991444861373809,-0.130526192220061));
#49595=DIRECTION('',(0.,0.60876142900872,-0.793353340291236));
#49596=DIRECTION('center_axis',(-0.706796314703292,-0.430648251649831,0.561231728319763));
#49597=DIRECTION('ref_axis',(0.,0.793353340291235,0.608761429008721));
#49598=DIRECTION('center_axis',(0.706790970016666,0.430651502409095,-0.561235964791717));
#49599=DIRECTION('ref_axis',(-0.70710678118862,0.406377146597434,-0.578668829919494));
#49600=DIRECTION('center_axis',(0.,0.,1.));
#49601=DIRECTION('ref_axis',(1.,0.,0.));
#49602=DIRECTION('center_axis',(0.,0.818361307397103,0.574704072158276));
#49603=DIRECTION('ref_axis',(0.,0.574704072158276,-0.818361307397103));
#49604=DIRECTION('center_axis',(1.,0.,0.));
#49605=DIRECTION('ref_axis',(0.,0.988493193186423,-0.151265353019486));
#49606=DIRECTION('',(-1.,0.,0.));
#49607=DIRECTION('center_axis',(1.,0.,0.));
#49608=DIRECTION('ref_axis',(0.,0.57499774870989,-0.818154990804651));
#49609=DIRECTION('',(1.,0.,0.));
#49610=DIRECTION('center_axis',(0.,0.,1.));
#49611=DIRECTION('ref_axis',(1.,0.,0.));
#49612=DIRECTION('center_axis',(0.,0.818154990804651,0.574997748709889));
#49613=DIRECTION('ref_axis',(0.,0.574997748709889,-0.818154990804651));
#49614=DIRECTION('center_axis',(1.,0.,0.));
#49615=DIRECTION('ref_axis',(0.,0.,-1.));
#49616=DIRECTION('center_axis',(-1.,0.,0.));
#49617=DIRECTION('ref_axis',(0.,0.555570233019602,-0.831469612302546));
#49618=DIRECTION('center_axis',(0.,-0.844130643547427,-0.536137535175636));
#49619=DIRECTION('ref_axis',(0.,0.536137535175636,-0.844130643547427));
#49620=DIRECTION('center_axis',(1.,0.,0.));
#49621=DIRECTION('ref_axis',(0.,1.,0.));
#49622=DIRECTION('center_axis',(1.,-2.58481526920973E-16,3.83463640548161E-16));
#49623=DIRECTION('ref_axis',(4.62446822220508E-16,0.558943243851984,-0.829205915410775));
#49624=DIRECTION('center_axis',(1.,0.,0.));
#49625=DIRECTION('ref_axis',(0.,0.,-1.));
#49626=DIRECTION('center_axis',(-1.,0.,0.));
#49627=DIRECTION('ref_axis',(0.,0.558943243851984,-0.829205915410775));
#49628=DIRECTION('center_axis',(-3.40731870374111E-16,0.844323011360893,
0.535834538347868));
#49629=DIRECTION('ref_axis',(0.,0.535834538347868,-0.844323011360893));
#49630=DIRECTION('center_axis',(1.,0.,0.));
#49631=DIRECTION('ref_axis',(0.,1.,0.));
#49632=DIRECTION('center_axis',(1.,0.,0.));
#49633=DIRECTION('ref_axis',(0.,0.,-1.));
#49634=DIRECTION('',(1.,0.,0.));
#49635=DIRECTION('center_axis',(0.,0.382683432365089,-0.923879532511287));
#49636=DIRECTION('ref_axis',(0.707106781186561,-0.653281482438177,-0.270598050073091));
#49637=DIRECTION('center_axis',(0.,-0.382683432365087,0.923879532511288));
#49638=DIRECTION('ref_axis',(0.,-0.923879532511288,-0.382683432365087));
#49639=DIRECTION('center_axis',(0.,-0.923879532511287,0.382683432365089));
#49640=DIRECTION('ref_axis',(-8.17756488897799E-17,-0.382683432365089,-0.923879532511287));
#49641=DIRECTION('',(0.,0.382683432365089,-0.923879532511287));
#49642=DIRECTION('center_axis',(0.706796314702667,-0.270716808310085,0.653568190184566));
#49643=DIRECTION('ref_axis',(0.,-0.923879532511287,-0.382683432365089));
#49644=DIRECTION('center_axis',(-0.706790970015948,0.270718851822823,-0.653573123660733));
#49645=DIRECTION('ref_axis',(0.707106781189338,0.297953333789467,-0.641267347429913));
#49646=DIRECTION('center_axis',(0.,0.,1.));
#49647=DIRECTION('ref_axis',(1.,0.,0.));
#49648=DIRECTION('center_axis',(0.,-0.906888979845984,-0.421369645600998));
#49649=DIRECTION('ref_axis',(0.,0.421369645600998,-0.906888979845984));
#49650=DIRECTION('center_axis',(-1.,0.,0.));
#49651=DIRECTION('ref_axis',(0.,-0.363246958165926,-0.931692893277179));
#49652=DIRECTION('',(1.,0.,0.));
#49653=DIRECTION('center_axis',(-1.,0.,0.));
#49654=DIRECTION('ref_axis',(0.,0.421044131914909,-0.90704015290395));
#49655=DIRECTION('',(-1.,0.,0.));
#49656=DIRECTION('center_axis',(-0.0341251959389409,-0.995062857517424,
0.0931953893247336));
#49657=DIRECTION('ref_axis',(0.342144487581495,-0.0992467107226136,-0.934391374119185));
#49658=DIRECTION('center_axis',(0.,-0.907040152903952,-0.421044131914905));
#49659=DIRECTION('ref_axis',(0.,0.421044131914905,-0.907040152903952));
#49660=DIRECTION('center_axis',(1.,0.,0.));
#49661=DIRECTION('ref_axis',(0.,0.,-1.));
#49662=DIRECTION('center_axis',(1.,0.,0.));
#49663=DIRECTION('ref_axis',(0.,0.442288690219,-0.896872741532689));
#49664=DIRECTION('center_axis',(0.,0.886374047158187,0.462969813837162));
#49665=DIRECTION('ref_axis',(0.,0.462969813837162,-0.886374047158187));
#49666=DIRECTION('center_axis',(-1.,0.,0.));
#49667=DIRECTION('ref_axis',(0.,1.,0.));
#49668=DIRECTION('center_axis',(-1.,0.,0.));
#49669=DIRECTION('ref_axis',(0.,0.438641765788068,-0.898662006154887));
#49670=DIRECTION('center_axis',(-0.706790970016282,0.353711225685391,-0.612645814094556));
#49671=DIRECTION('ref_axis',(0.,0.866025403784438,0.500000000000001));
#49672=DIRECTION('center_axis',(0.706796314705248,-0.353708555706286,0.612641189554909));
#49673=DIRECTION('ref_axis',(0.707106781186564,0.3275940211512,-0.626643564800568));
#49674=DIRECTION('center_axis',(1.,0.,0.));
#49675=DIRECTION('ref_axis',(0.,0.,-1.));
#49676=DIRECTION('center_axis',(1.,0.,0.));
#49677=DIRECTION('ref_axis',(0.,0.438641765788068,-0.898662006154887));
#49678=DIRECTION('center_axis',(2.4958609504901E-14,-0.886207828114815,
-0.463287907664363));
#49679=DIRECTION('ref_axis',(0.,0.463287907664363,-0.886207828114815));
#49680=DIRECTION('center_axis',(0.,0.,1.));
#49681=DIRECTION('ref_axis',(1.,0.,0.));
#49682=DIRECTION('center_axis',(1.,0.,0.));
#49683=DIRECTION('ref_axis',(0.,0.960292406343207,-0.278995509497148));
#49684=DIRECTION('center_axis',(0.,-0.499999999999999,0.866025403784439));
#49685=DIRECTION('ref_axis',(0.707106781186556,0.612372435695782,0.353553390593278));
#49686=DIRECTION('center_axis',(3.70074341541706E-15,-0.500000000000001,
0.866025403784438));
#49687=DIRECTION('ref_axis',(1.,7.4014868308341E-15,0.));
#49688=DIRECTION('',(0.,-0.499999999999999,0.866025403784439));
#49689=DIRECTION('center_axis',(0.,0.258819045102529,0.965925826289066));
#49690=DIRECTION('ref_axis',(-4.08878244448897E-17,0.965925826289066,-0.258819045102529));
#49691=DIRECTION('center_axis',(0.,0.,1.));
#49692=DIRECTION('ref_axis',(1.,0.,0.));
#49693=DIRECTION('center_axis',(0.,0.923879532511287,0.382683432365089));
#49694=DIRECTION('ref_axis',(1.,0.,0.));
#49695=DIRECTION('',(1.,0.,0.));
#49696=DIRECTION('center_axis',(0.,0.923879532511287,0.382683432365089));
#49697=DIRECTION('ref_axis',(-0.707106781186561,0.270598050073091,-0.653281482438177));
#49698=DIRECTION('',(-0.706902428155816,-0.270676229998406,0.653470225474169));
#49699=DIRECTION('center_axis',(0.706790970016302,0.353711225685381,-0.612645814094539));
#49700=DIRECTION('ref_axis',(0.,-0.866025403784438,-0.500000000000001));
#49701=DIRECTION('center_axis',(-0.706796314705254,-0.353708555706211,0.612641189554944));
#49702=DIRECTION('ref_axis',(-0.70710678118656,0.378892235659731,-0.597026526845125));
#49703=DIRECTION('center_axis',(0.,-0.499999999999999,0.866025403784439));
#49704=DIRECTION('ref_axis',(-0.707106781186556,-0.612372435695782,-0.353553390593278));
#49705=DIRECTION('center_axis',(0.,-0.500000000000001,0.866025403784438));
#49706=DIRECTION('ref_axis',(-1.,0.,0.));
#49707=DIRECTION('',(0.,-0.499999999999999,0.866025403784439));
#49708=DIRECTION('center_axis',(0.,-0.96592582628907,0.258819045102514));
#49709=DIRECTION('ref_axis',(-8.17756488897793E-17,-0.258819045102514,-0.96592582628907));
#49710=DIRECTION('center_axis',(0.,0.,1.));
#49711=DIRECTION('ref_axis',(-0.858053385943022,-0.513560499719085,0.));
#49712=DIRECTION('center_axis',(-0.00806484247865072,-0.999722309028825,
-0.0221418866826893));
#49713=DIRECTION('ref_axis',(-0.342144487592342,0.0235649067486914,-0.93935182161962));
#49714=DIRECTION('center_axis',(-1.,0.,0.));
#49715=DIRECTION('ref_axis',(0.,-0.238529004405322,-0.971135373703072));
#49716=DIRECTION('center_axis',(0.,-0.793353340291236,-0.60876142900872));
#49717=DIRECTION('ref_axis',(-1.,0.,0.));
#49718=DIRECTION('',(-1.,0.,0.));
#49719=DIRECTION('center_axis',(0.,-0.793353340291236,-0.60876142900872));
#49720=DIRECTION('ref_axis',(0.707106781186516,0.430459334576894,-0.56098552679696));
#49721=DIRECTION('',(0.706902428155818,-0.430583700878177,0.561147604116297));
#49722=DIRECTION('center_axis',(0.706790970016333,0.612645814094511,-0.353711225685368));
#49723=DIRECTION('ref_axis',(0.,-0.500000000000005,-0.866025403784436));
#49724=DIRECTION('center_axis',(-0.706796314705255,-0.612641189554953,0.353708555706195));
#49725=DIRECTION('ref_axis',(-0.707106781186559,0.626643564800579,-0.32759402115119));
#49726=DIRECTION('center_axis',(0.,-0.866025403784438,0.5));
#49727=DIRECTION('ref_axis',(-0.707106781186566,-0.353553390593262,-0.61237243569578));
#49728=DIRECTION('center_axis',(0.,-0.866025403784436,0.500000000000005));
#49729=DIRECTION('ref_axis',(-1.,0.,0.));
#49730=DIRECTION('',(0.,-0.866025403784438,0.5));
#49731=DIRECTION('center_axis',(0.,-0.965925826289068,-0.258819045102521));
#49732=DIRECTION('ref_axis',(0.,0.258819045102521,-0.965925826289068));
#49733=DIRECTION('center_axis',(0.,0.,1.));
#49734=DIRECTION('ref_axis',(-0.911951719487308,-0.410297527806519,0.));
#49735=DIRECTION('center_axis',(-0.192364553135181,-0.871675368857593,-0.450752626197654));
#49736=DIRECTION('ref_axis',(-0.34214448759239,0.490083718691995,-0.80172008723941));
#49737=DIRECTION('center_axis',(-1.,0.,0.));
#49738=DIRECTION('ref_axis',(0.,0.278995509497118,-0.960292406343216));
#49739=DIRECTION('center_axis',(0.,-0.38268343236509,-0.923879532511287));
#49740=DIRECTION('ref_axis',(-1.,0.,0.));
#49741=DIRECTION('',(-1.,0.,0.));
#49742=DIRECTION('center_axis',(0.,-0.38268343236509,-0.923879532511287));
#49743=DIRECTION('ref_axis',(0.707106781186519,0.653281482438215,-0.270598050073107));
#49744=DIRECTION('',(0.706902428155817,-0.653470225474166,0.27067622999841));
#49745=DIRECTION('center_axis',(-0.706790970015287,0.683317615876718,-0.183094403348131));
#49746=DIRECTION('ref_axis',(0.,0.258819045102527,0.965925826289067));
#49747=DIRECTION('center_axis',(0.706796314705261,-0.683312457872046,0.183093021264943));
#49748=DIRECTION('ref_axis',(0.707106781186553,0.674747867889586,-0.211459960225215));
#49749=DIRECTION('center_axis',(1.,0.,0.));
#49750=DIRECTION('ref_axis',(0.,0.,-1.));
#49751=DIRECTION('center_axis',(1.,0.,0.));
#49752=DIRECTION('ref_axis',(0.,0.945616565647212,-0.325283431446443));
#49753=DIRECTION('center_axis',(-7.36832669684028E-15,-0.299049543649382,
-0.954237585951788));
#49754=DIRECTION('ref_axis',(0.,0.954237585951788,-0.299049543649382));
#49755=DIRECTION('center_axis',(0.,0.,1.));
#49756=DIRECTION('ref_axis',(1.,0.,0.));
#49757=DIRECTION('center_axis',(1.,0.,0.));
#49758=DIRECTION('ref_axis',(0.,0.87630888913324,0.481749655761233));
#49759=DIRECTION('center_axis',(0.,-0.965925826289068,0.258819045102522));
#49760=DIRECTION('ref_axis',(0.707106781186554,0.183012701892219,0.683012701892212));
#49761=DIRECTION('center_axis',(0.,-0.965925826289067,0.258819045102525));
#49762=DIRECTION('ref_axis',(1.,0.,0.));
#49763=DIRECTION('',(0.,-0.965925826289068,0.258819045102522));
#49764=DIRECTION('center_axis',(0.,-0.500000000000002,0.866025403784437));
#49765=DIRECTION('ref_axis',(-1.2266347333467E-16,0.866025403784437,0.500000000000002));
#49766=DIRECTION('center_axis',(0.,0.,1.));
#49767=DIRECTION('ref_axis',(1.,0.,0.));
#49768=DIRECTION('center_axis',(0.,0.38268343236509,0.923879532511287));
#49769=DIRECTION('ref_axis',(1.,0.,0.));
#49770=DIRECTION('',(1.,0.,0.));
#49771=DIRECTION('center_axis',(0.,0.38268343236509,0.923879532511287));
#49772=DIRECTION('ref_axis',(-0.70710678118656,0.653281482438176,-0.270598050073096));
#49773=DIRECTION('',(-0.706902428155812,-0.653470225474173,0.270676229998407));
#49774=DIRECTION('center_axis',(-1.,0.,0.));
#49775=DIRECTION('ref_axis',(0.,0.518030931670888,-0.855361884720258));
#49776=DIRECTION('',(1.,0.,0.));
#49777=DIRECTION('',(-1.,0.,0.));
#49778=DIRECTION('center_axis',(1.,0.,0.));
#49779=DIRECTION('ref_axis',(0.,1.,0.));
#49780=DIRECTION('',(-0.706902428155817,-0.68321003473332,0.183065577067633));
#49781=DIRECTION('center_axis',(-1.,0.,0.));
#49782=DIRECTION('ref_axis',(0.,0.98078528040323,-0.19509032201613));
#49783=DIRECTION('',(0.706902428155816,0.701259930876578,-0.0923226213578685));
#49784=DIRECTION('center_axis',(1.,0.,0.));
#49785=DIRECTION('ref_axis',(0.,0.,-1.));
#49786=DIRECTION('center_axis',(0.,0.258819045102522,0.965925826289068));
#49787=DIRECTION('ref_axis',(1.,0.,0.));
#49788=DIRECTION('',(-0.706902428155817,0.683210034733321,-0.183065577067633));
#49789=DIRECTION('center_axis',(0.,0.258819045102522,0.965925826289068));
#49790=DIRECTION('ref_axis',(0.707106781186513,0.683012701892254,-0.183012701892225));
#49791=DIRECTION('',(1.,0.,0.));
#49792=DIRECTION('center_axis',(0.,0.258819045102522,0.965925826289068));
#49793=DIRECTION('ref_axis',(-0.707106781186565,0.683012701892202,-0.183012701892217));
#49794=DIRECTION('center_axis',(0.706790970016542,0.561235964791816,-0.43065150240917));
#49795=DIRECTION('ref_axis',(0.,-0.608761429008721,-0.793353340291235));
#49796=DIRECTION('center_axis',(-0.706796314705254,-0.561231728318169,0.430648251648689));
#49797=DIRECTION('ref_axis',(-0.707106781186558,0.578522942059579,-0.406584807279753));
#49798=DIRECTION('center_axis',(0.,-0.793353340291235,0.608761429008721));
#49799=DIRECTION('ref_axis',(-0.707106781186562,-0.430459334576871,-0.560985526796919));
#49800=DIRECTION('center_axis',(0.,-0.793353340291235,0.608761429008721));
#49801=DIRECTION('ref_axis',(-1.,0.,0.));
#49802=DIRECTION('',(0.,-0.793353340291235,0.608761429008721));
#49803=DIRECTION('center_axis',(0.,-0.99144486137381,-0.130526192220052));
#49804=DIRECTION('ref_axis',(4.08878244448899E-17,0.130526192220052,-0.99144486137381));
#49805=DIRECTION('center_axis',(0.,0.,1.));
#49806=DIRECTION('ref_axis',(-0.903692699960925,-0.428181625058027,0.));
#49807=DIRECTION('center_axis',(-0.141097613864597,-0.924473827539728,-0.354174541089223));
#49808=DIRECTION('ref_axis',(-0.342144487592437,0.381245514326465,-0.858830022423563));
#49809=DIRECTION('center_axis',(-1.,0.,0.));
#49810=DIRECTION('ref_axis',(0.,0.151265353019466,-0.988493193186426));
#49811=DIRECTION('center_axis',(0.,-0.5,-0.866025403784438));
#49812=DIRECTION('ref_axis',(-1.,0.,0.));
#49813=DIRECTION('',(-1.,0.,0.));
#49814=DIRECTION('center_axis',(0.,-0.5,-0.866025403784438));
#49815=DIRECTION('ref_axis',(0.707106781186512,0.612372435695827,-0.353553390593288));
#49816=DIRECTION('',(0.706902428155815,-0.612549359480985,0.353655537588269));
#49817=DIRECTION('center_axis',(0.,0.707106781186547,-0.707106781186548));
#49818=DIRECTION('ref_axis',(0.707106781186563,-0.499999999999978,-0.499999999999999));
#49819=DIRECTION('center_axis',(0.,-0.707106781186548,0.707106781186548));
#49820=DIRECTION('ref_axis',(0.,-0.707106781186547,-0.707106781186547));
#49821=DIRECTION('center_axis',(0.,-1.,0.));
#49822=DIRECTION('ref_axis',(0.,0.,-1.));
#49823=DIRECTION('',(0.,0.707106781186547,-0.707106781186548));
#49824=DIRECTION('center_axis',(0.706796314703336,-0.500219436608466,0.500219436608466));
#49825=DIRECTION('ref_axis',(0.,-0.707106781186547,-0.707106781186547));
#49826=DIRECTION('center_axis',(-0.70679097001671,0.500223212527587,-0.500223212527587));
#49827=DIRECTION('ref_axis',(0.707106781188576,0.520675376310293,-0.478431972699637));
#49828=DIRECTION('center_axis',(0.,0.,1.));
#49829=DIRECTION('ref_axis',(1.,0.,0.));
#49830=DIRECTION('center_axis',(0.,-0.676604984466694,-0.736346178773832));
#49831=DIRECTION('ref_axis',(0.,0.736346178773832,-0.676604984466694));
#49832=DIRECTION('center_axis',(-1.,0.,0.));
#49833=DIRECTION('ref_axis',(0.,0.0209470044129978,-0.999780587432124));
#49834=DIRECTION('',(1.,0.,0.));
#49835=DIRECTION('center_axis',(-1.,0.,0.));
#49836=DIRECTION('ref_axis',(0.,0.736103294766417,-0.676869218855478));
#49837=DIRECTION('',(-1.,0.,0.));
#49838=DIRECTION('center_axis',(0.0943675359584502,-0.964005004559962,-0.248574172714059));
#49839=DIRECTION('ref_axis',(0.342144487584433,0.265884093513232,-0.901245137813366));
#49840=DIRECTION('center_axis',(0.,-0.676869218855493,-0.736103294766404));
#49841=DIRECTION('ref_axis',(0.,0.736103294766404,-0.676869218855493));
#49842=DIRECTION('center_axis',(1.,0.,0.));
#49843=DIRECTION('ref_axis',(0.,0.,-1.));
#49844=DIRECTION('center_axis',(1.,0.,0.));
#49845=DIRECTION('ref_axis',(0.,0.751839807478977,-0.65934581510007));
#49846=DIRECTION('center_axis',(0.,0.641731962878011,0.766928997900546));
#49847=DIRECTION('ref_axis',(0.,0.766928997900546,-0.641731962878011));
#49848=DIRECTION('center_axis',(-1.,0.,0.));
#49849=DIRECTION('ref_axis',(0.,1.,0.));
#49850=DIRECTION('center_axis',(-1.,0.,0.));
#49851=DIRECTION('ref_axis',(0.,0.749155210567655,-0.66239449762157));
#49852=DIRECTION('center_axis',(0.706790970016547,0.430651502409167,-0.561235964791811));
#49853=DIRECTION('ref_axis',(0.,-0.793353340291235,-0.608761429008721));
#49854=DIRECTION('center_axis',(-0.706796314705247,-0.430648251648649,0.561231728318209));
#49855=DIRECTION('ref_axis',(-0.707106781186567,0.453578359262747,-0.542463521362024));
#49856=DIRECTION('center_axis',(0.,-0.60876142900872,0.793353340291236));
#49857=DIRECTION('ref_axis',(-0.707106781186562,-0.560985526796919,-0.430459334576871));
#49858=DIRECTION('center_axis',(0.,-0.608761429008714,0.79335334029124));
#49859=DIRECTION('ref_axis',(-1.,0.,0.));
#49860=DIRECTION('center_axis',(0.,-0.991444861373811,0.130526192220051));
#49861=DIRECTION('ref_axis',(4.08878244448899E-17,-0.130526192220051,-0.991444861373811));
#49862=DIRECTION('center_axis',(0.,0.,1.));
#49863=DIRECTION('ref_axis',(-0.877521329523614,-0.479537606691185,0.));
#49864=DIRECTION('center_axis',(-0.050484733373679,-0.98928852678309,-0.136965333101232));
#49865=DIRECTION('ref_axis',(-0.342144487592388,0.145973322135736,-0.928239699018955));
#49866=DIRECTION('center_axis',(-0.706790970016564,0.561235964791798,-0.430651502409157));
#49867=DIRECTION('ref_axis',(0.,0.608761429008721,0.793353340291235));
#49868=DIRECTION('center_axis',(0.706796314705259,-0.561231728318196,0.430648251648647));
#49869=DIRECTION('ref_axis',(0.707106781186556,0.542463521362045,-0.453578359262739));
#49870=DIRECTION('center_axis',(1.,0.,0.));
#49871=DIRECTION('ref_axis',(0.,0.,-1.));
#49872=DIRECTION('center_axis',(1.,0.,0.));
#49873=DIRECTION('ref_axis',(0.,0.749155210567655,-0.66239449762157));
#49874=DIRECTION('center_axis',(-9.19976050010013E-15,-0.641456667268323,
-0.767159269002869));
#49875=DIRECTION('ref_axis',(0.,0.767159269002869,-0.641456667268323));
#49876=DIRECTION('center_axis',(0.,0.,1.));
#49877=DIRECTION('ref_axis',(1.,0.,0.));
#49878=DIRECTION('center_axis',(1.,0.,0.));
#49879=DIRECTION('ref_axis',(0.,0.993961458635311,0.10972975324662));
#49880=DIRECTION('center_axis',(0.,-0.793353340291235,0.608761429008721));
#49881=DIRECTION('ref_axis',(0.707106781186566,0.430459334576874,0.560985526796912));
#49882=DIRECTION('center_axis',(0.,-0.793353340291235,0.608761429008721));
#49883=DIRECTION('ref_axis',(1.,0.,0.));
#49884=DIRECTION('',(0.,-0.793353340291235,0.608761429008721));
#49885=DIRECTION('center_axis',(0.,-0.13052619222005,0.991444861373811));
#49886=DIRECTION('ref_axis',(4.08878244448899E-17,0.991444861373811,0.13052619222005));
#49887=DIRECTION('center_axis',(0.,0.,1.));
#49888=DIRECTION('ref_axis',(1.,0.,0.));
#49889=DIRECTION('center_axis',(0.,0.707106781186548,0.707106781186547));
#49890=DIRECTION('ref_axis',(1.,0.,0.));
#49891=DIRECTION('',(1.,0.,0.));
#49892=DIRECTION('center_axis',(0.,0.707106781186548,0.707106781186547));
#49893=DIRECTION('ref_axis',(-0.707106781186567,0.499999999999981,-0.499999999999992));
#49894=DIRECTION('',(-0.706902428155818,-0.500144457665681,0.500144457665694));
#49895=DIRECTION('center_axis',(-1.,0.,0.));
#49896=DIRECTION('ref_axis',(0.,0.151265353019465,-0.988493193186426));
#49897=DIRECTION('',(-1.,0.,0.));
#49898=DIRECTION('center_axis',(0.,0.608761429008721,0.793353340291235));
#49899=DIRECTION('ref_axis',(1.,0.,0.));
#49900=DIRECTION('',(-0.706902428155816,0.561147604116301,-0.430583700878176));
#49901=DIRECTION('center_axis',(0.,0.608761429008721,0.793353340291235));
#49902=DIRECTION('ref_axis',(0.707106781186516,0.56098552679696,-0.430459334576894));
#49903=DIRECTION('',(1.,0.,0.));
#49904=DIRECTION('center_axis',(1.,0.,0.));
#49905=DIRECTION('ref_axis',(0.,0.,-1.));
#49906=DIRECTION('center_axis',(0.,0.0885276724488783,0.996073717759275));
#49907=DIRECTION('ref_axis',(1.,0.,0.));
#49908=DIRECTION('center_axis',(1.,0.,0.));
#49909=DIRECTION('ref_axis',(0.,0.998116759314604,-0.061342764653323));
#49910=DIRECTION('center_axis',(0.,0.99144486137381,-0.130526192220053));
#49911=DIRECTION('ref_axis',(0.707106781186562,-0.0922959556412482,-0.701057384649965));
#49912=DIRECTION('center_axis',(0.,-0.99144486137381,0.130526192220056));
#49913=DIRECTION('ref_axis',(-2.72374715374705E-11,-0.130526192220056,-0.99144486137381));
#49914=DIRECTION('center_axis',(0.,-0.793353340291239,-0.608761429008716));
#49915=DIRECTION('ref_axis',(4.08878244448902E-17,0.608761429008716,-0.793353340291238));
#49916=DIRECTION('',(0.,0.99144486137381,-0.130526192220053));
#49917=DIRECTION('center_axis',(0.,0.,1.));
#49918=DIRECTION('ref_axis',(1.,0.,0.));
#49919=DIRECTION('center_axis',(0.706790970018731,-0.701370354229598,0.0923371588680839));
#49920=DIRECTION('ref_axis',(0.,-0.130526192220056,-0.99144486137381));
#49921=DIRECTION('center_axis',(0.706796314705259,-0.701365059957719,0.0923364618640445));
#49922=DIRECTION('ref_axis',(5.9211894646675E-14,-0.1305261922201,-0.991444861373804));
#49923=DIRECTION('center_axis',(0.,0.130526192220053,0.99144486137381));
#49924=DIRECTION('ref_axis',(1.,0.,0.));
#49925=DIRECTION('',(1.,0.,0.));
#49926=DIRECTION('',(0.,-0.99144486137381,0.130526192220053));
#49927=DIRECTION('',(-1.,0.,0.));
#49928=DIRECTION('center_axis',(1.,0.,0.));
#49929=DIRECTION('ref_axis',(0.,0.,-1.));
#49930=DIRECTION('center_axis',(1.,0.,0.));
#49931=DIRECTION('ref_axis',(0.,0.98078528040323,-0.195090322016129));
#49932=DIRECTION('center_axis',(0.,0.258819045102522,0.965925826289068));
#49933=DIRECTION('ref_axis',(0.707106781186513,0.683012701892254,-0.183012701892225));
#49934=DIRECTION('',(0.,0.258819045102522,0.965925826289068));
#49935=DIRECTION('center_axis',(0.,-0.965925826289068,0.258819045102522));
#49936=DIRECTION('ref_axis',(1.,0.,0.));
#49937=DIRECTION('',(-1.,0.,0.));
#49938=DIRECTION('',(0.,-0.258819045102522,-0.965925826289068));
#49939=DIRECTION('center_axis',(0.,-0.258819045102522,-0.965925826289068));
#49940=DIRECTION('ref_axis',(-1.,0.,0.));
#49941=DIRECTION('',(1.,0.,0.));
#49942=DIRECTION('',(0.706902428155814,0.683210034733323,-0.183065577067632));
#49943=DIRECTION('center_axis',(0.,-0.258819045102522,-0.965925826289068));
#49944=DIRECTION('ref_axis',(-0.707106781186565,0.683012701892202,-0.183012701892217));
#49945=DIRECTION('center_axis',(-1.,0.,0.));
#49946=DIRECTION('ref_axis',(0.,0.27899550949712,-0.960292406343215));
#49947=DIRECTION('',(-1.,0.,0.));
#49948=DIRECTION('center_axis',(0.,0.5,0.866025403784438));
#49949=DIRECTION('ref_axis',(1.,0.,0.));
#49950=DIRECTION('',(-0.706902428155818,0.612549359480975,-0.35365553758828));
#49951=DIRECTION('center_axis',(0.,0.5,0.866025403784438));
#49952=DIRECTION('ref_axis',(0.707106781186512,0.612372435695827,-0.353553390593288));
#49953=DIRECTION('',(1.,0.,0.));
#49954=DIRECTION('center_axis',(1.,0.,0.));
#49955=DIRECTION('ref_axis',(0.,0.,-1.));
#49956=DIRECTION('center_axis',(1.,0.,0.));
#49957=DIRECTION('ref_axis',(0.,0.896872741532688,-0.442288690219002));
#49958=DIRECTION('center_axis',(0.,0.5,0.866025403784438));
#49959=DIRECTION('ref_axis',(0.707106781186512,0.612372435695827,-0.353553390593288));
#49960=DIRECTION('',(0.,0.5,0.866025403784438));
#49961=DIRECTION('center_axis',(0.,-0.866025403784438,0.5));
#49962=DIRECTION('ref_axis',(1.,0.,0.));
#49963=DIRECTION('',(0.,-0.5,-0.866025403784438));
#49964=DIRECTION('center_axis',(1.,0.,0.));
#49965=DIRECTION('ref_axis',(0.,0.,-1.));
#49966=DIRECTION('center_axis',(1.,0.,0.));
#49967=DIRECTION('ref_axis',(0.,0.831469612302545,-0.555570233019602));
#49968=DIRECTION('center_axis',(0.,0.608761429008721,0.793353340291235));
#49969=DIRECTION('ref_axis',(0.707106781186516,0.56098552679696,-0.430459334576894));
#49970=DIRECTION('',(0.,0.608761429008721,0.793353340291235));
#49971=DIRECTION('center_axis',(0.,-0.793353340291235,0.608761429008721));
#49972=DIRECTION('ref_axis',(1.,0.,0.));
#49973=DIRECTION('',(-1.,0.,0.));
#49974=DIRECTION('',(0.,-0.608761429008721,-0.793353340291235));
#49975=DIRECTION('center_axis',(0.,-0.608761429008721,-0.793353340291235));
#49976=DIRECTION('ref_axis',(-1.,0.,0.));
#49977=DIRECTION('',(1.,0.,0.));
#49978=DIRECTION('',(0.706902428155819,0.561147604116299,-0.430583700878174));
#49979=DIRECTION('center_axis',(0.,-0.608761429008721,-0.793353340291235));
#49980=DIRECTION('ref_axis',(-0.707106781186558,0.560985526796926,-0.430459334576869));
#49981=DIRECTION('center_axis',(1.,0.,0.));
#49982=DIRECTION('ref_axis',(0.,0.,-1.));
#49983=DIRECTION('center_axis',(1.,0.,0.));
#49984=DIRECTION('ref_axis',(0.,0.659345815100068,-0.751839807478978));
#49985=DIRECTION('center_axis',(0.,0.793353340291236,0.60876142900872));
#49986=DIRECTION('ref_axis',(0.707106781186516,0.430459334576894,-0.56098552679696));
#49987=DIRECTION('',(0.,0.793353340291236,0.60876142900872));
#49988=DIRECTION('center_axis',(0.,-0.60876142900872,0.793353340291236));
#49989=DIRECTION('ref_axis',(1.,0.,0.));
#49990=DIRECTION('',(0.,-0.793353340291236,-0.60876142900872));
#49991=DIRECTION('center_axis',(-1.,0.,0.));
#49992=DIRECTION('ref_axis',(0.,-0.238529004405328,-0.971135373703071));
#49993=DIRECTION('',(-1.,0.,0.));
#49994=DIRECTION('center_axis',(0.,0.866025403784439,0.499999999999999));
#49995=DIRECTION('ref_axis',(1.,0.,0.));
#49996=DIRECTION('',(-0.706902428155815,0.353655537588269,-0.612549359480985));
#49997=DIRECTION('center_axis',(0.,0.866025403784439,0.499999999999999));
#49998=DIRECTION('ref_axis',(0.70710678118651,0.353553390593297,-0.612372435695825));
#49999=DIRECTION('',(1.,0.,0.));
#50000=DIRECTION('center_axis',(1.,0.,0.));
#50001=DIRECTION('ref_axis',(0.,0.,-1.));
#50002=DIRECTION('center_axis',(1.,0.,0.));
#50003=DIRECTION('ref_axis',(0.,0.555570233019602,-0.831469612302545));
#50004=DIRECTION('center_axis',(0.,0.866025403784439,0.499999999999999));
#50005=DIRECTION('ref_axis',(0.70710678118651,0.353553390593297,-0.612372435695825));
#50006=DIRECTION('',(0.,0.866025403784439,0.499999999999999));
#50007=DIRECTION('center_axis',(0.,-0.499999999999999,0.866025403784439));
#50008=DIRECTION('ref_axis',(1.,0.,0.));
#50009=DIRECTION('',(-1.,0.,0.));
#50010=DIRECTION('',(0.,-0.866025403784439,-0.499999999999999));
#50011=DIRECTION('center_axis',(0.,-0.866025403784439,-0.499999999999999));
#50012=DIRECTION('ref_axis',(-1.,0.,0.));
#50013=DIRECTION('',(1.,0.,0.));
#50014=DIRECTION('',(0.706902428155817,0.353655537588279,-0.612549359480977));
#50015=DIRECTION('center_axis',(0.,-0.866025403784439,-0.499999999999999));
#50016=DIRECTION('ref_axis',(-0.707106781186557,0.353553390593258,-0.612372435695793));
#50017=DIRECTION('center_axis',(1.,0.,0.));
#50018=DIRECTION('ref_axis',(0.,0.,-1.));
#50019=DIRECTION('center_axis',(1.,0.,0.));
#50020=DIRECTION('ref_axis',(0.,0.321439465303161,-0.946930129495106));
#50021=DIRECTION('center_axis',(0.,0.965925826289068,0.25881904510252));
#50022=DIRECTION('ref_axis',(0.707106781186512,0.18301270189223,-0.683012701892253));
#50023=DIRECTION('',(0.,0.965925826289068,0.25881904510252));
#50024=DIRECTION('center_axis',(0.,-0.25881904510252,0.965925826289068));
#50025=DIRECTION('ref_axis',(1.,0.,0.));
#50026=DIRECTION('',(0.,-0.965925826289068,-0.25881904510252));
#50027=DIRECTION('center_axis',(1.,0.,0.));
#50028=DIRECTION('ref_axis',(0.,0.,-1.));
#50029=DIRECTION('center_axis',(1.,0.,0.));
#50030=DIRECTION('ref_axis',(0.,0.195090322016127,-0.980785280403231));
#50031=DIRECTION('center_axis',(-1.,0.,0.));
#50032=DIRECTION('ref_axis',(0.,-0.780427540257703,-0.625246235020501));
#50033=DIRECTION('',(-1.,0.,0.));
#50034=DIRECTION('center_axis',(0.,0.99144486137381,-0.130526192220052));
#50035=DIRECTION('ref_axis',(1.,0.,0.));
#50036=DIRECTION('',(-0.706902428155816,-0.0923226213578668,-0.701259930876578));
#50037=DIRECTION('center_axis',(0.,0.99144486137381,-0.130526192220052));
#50038=DIRECTION('ref_axis',(0.70710678118651,-0.0922959556412628,-0.701057384650015));
#50039=DIRECTION('',(1.,0.,0.));
#50040=DIRECTION('center_axis',(-0.706790970014404,0.0923371588686503,-0.701370354233883));
#50041=DIRECTION('ref_axis',(0.,0.99144486137381,0.130526192220056));
#50042=DIRECTION('center_axis',(0.706796314705253,-0.0923364618639829,0.701365059957733));
#50043=DIRECTION('ref_axis',(0.70710678118656,0.0628513008672821,-0.704307968135582));
#50044=DIRECTION('center_axis',(0.,0.,1.));
#50045=DIRECTION('ref_axis',(1.,0.,0.));
#50046=DIRECTION('center_axis',(1.,0.,0.));
#50047=DIRECTION('ref_axis',(0.,0.780427540257703,-0.625246235020501));
#50048=DIRECTION('center_axis',(0.,-0.130526192220051,0.99144486137381));
#50049=DIRECTION('ref_axis',(0.707106781186561,0.701057384649966,0.0922959556412481));
#50050=DIRECTION('center_axis',(0.,-0.130526192220056,0.99144486137381));
#50051=DIRECTION('ref_axis',(1.,0.,0.));
#50052=DIRECTION('',(0.,-0.130526192220051,0.991444861373811));
#50053=DIRECTION('center_axis',(0.,0.60876142900871,0.793353340291243));
#50054=DIRECTION('ref_axis',(8.1775648889781E-17,0.793353340291243,-0.60876142900871));
#50055=DIRECTION('center_axis',(0.,0.,1.));
#50056=DIRECTION('ref_axis',(1.,0.,0.));
#50057=DIRECTION('center_axis',(0.,0.99144486137381,0.130526192220051));
#50058=DIRECTION('ref_axis',(0.707106781186521,0.0922959556412538,-0.701057384650005));
#50059=DIRECTION('',(0.,0.991444861373811,0.130526192220051));
#50060=DIRECTION('center_axis',(0.,-0.130526192220051,0.99144486137381));
#50061=DIRECTION('ref_axis',(1.,0.,0.));
#50062=DIRECTION('',(-1.,0.,0.));
#50063=DIRECTION('',(0.,-0.991444861373811,-0.130526192220051));
#50064=DIRECTION('center_axis',(0.,-0.99144486137381,-0.130526192220051));
#50065=DIRECTION('ref_axis',(-1.,0.,0.));
#50066=DIRECTION('',(1.,0.,0.));
#50067=DIRECTION('center_axis',(1.,0.,0.));
#50068=DIRECTION('ref_axis',(0.,0.,-1.));
#50069=DIRECTION('center_axis',(1.,0.,0.));
#50070=DIRECTION('ref_axis',(0.,-0.0654031292301436,-0.997858923238603));
#50071=DIRECTION('center_axis',(0.,0.99144486137381,-0.130526192220052));
#50072=DIRECTION('ref_axis',(0.70710678118651,-0.0922959556412628,-0.701057384650015));
#50073=DIRECTION('',(0.,0.99144486137381,-0.130526192220052));
#50074=DIRECTION('center_axis',(0.,0.130526192220052,0.99144486137381));
#50075=DIRECTION('ref_axis',(1.,0.,0.));
#50076=DIRECTION('',(0.,-0.99144486137381,0.130526192220052));
#50077=DIRECTION('center_axis',(1.,0.,0.));
#50078=DIRECTION('ref_axis',(0.,0.,-1.));
#50079=DIRECTION('center_axis',(1.,0.,0.));
#50080=DIRECTION('ref_axis',(0.,-0.19509032201613,-0.98078528040323));
#50081=DIRECTION('center_axis',(0.,0.965925826289068,-0.258819045102522));
#50082=DIRECTION('ref_axis',(0.707106781186523,-0.183012701892228,-0.683012701892242));
#50083=DIRECTION('',(0.,0.965925826289068,-0.258819045102522));
#50084=DIRECTION('center_axis',(0.,0.258819045102522,0.965925826289068));
#50085=DIRECTION('ref_axis',(1.,0.,0.));
#50086=DIRECTION('',(-1.,0.,0.));
#50087=DIRECTION('',(0.,-0.965925826289068,0.258819045102522));
#50088=DIRECTION('center_axis',(0.,-0.965925826289068,0.258819045102522));
#50089=DIRECTION('ref_axis',(-1.,0.,0.));
#50090=DIRECTION('',(1.,0.,0.));
#50091=DIRECTION('',(0.706902428155814,-0.183065577067632,-0.683210034733323));
#50092=DIRECTION('center_axis',(0.,-0.965925826289068,0.258819045102522));
#50093=DIRECTION('ref_axis',(-0.707106781186555,-0.183012701892214,-0.683012701892213));
#50094=DIRECTION('center_axis',(-1.,0.,0.));
#50095=DIRECTION('ref_axis',(0.,-0.96029240634322,-0.278995509497103));
#50096=DIRECTION('',(-1.,0.,0.));
#50097=DIRECTION('center_axis',(0.,0.866025403784438,-0.5));
#50098=DIRECTION('ref_axis',(1.,0.,0.));
#50099=DIRECTION('',(-0.706902428155818,-0.35365553758828,-0.612549359480975));
#50100=DIRECTION('center_axis',(0.,0.866025403784438,-0.5));
#50101=DIRECTION('ref_axis',(0.707106781186512,-0.353553390593288,-0.612372435695827));
#50102=DIRECTION('',(1.,0.,0.));
#50103=DIRECTION('center_axis',(1.,0.,0.));
#50104=DIRECTION('ref_axis',(0.,0.,-1.));
#50105=DIRECTION('center_axis',(1.,0.,0.));
#50106=DIRECTION('ref_axis',(0.,-0.442288690219002,-0.896872741532688));
#50107=DIRECTION('center_axis',(0.,0.866025403784438,-0.5));
#50108=DIRECTION('ref_axis',(0.707106781186512,-0.353553390593288,-0.612372435695827));
#50109=DIRECTION('center_axis',(0.,-0.866025403784438,0.5));
#50110=DIRECTION('ref_axis',(0.707106781186512,-0.353553390593288,-0.612372435695827));
#50111=DIRECTION('',(0.,0.866025403784438,-0.5));
#50112=DIRECTION('center_axis',(0.,0.5,0.866025403784438));
#50113=DIRECTION('ref_axis',(1.,0.,0.));
#50114=DIRECTION('',(-1.,0.,0.));
#50115=DIRECTION('',(0.,-0.866025403784438,0.5));
#50116=DIRECTION('center_axis',(1.,0.,0.));
#50117=DIRECTION('ref_axis',(0.,0.,-1.));
#50118=DIRECTION('center_axis',(1.,0.,0.));
#50119=DIRECTION('ref_axis',(0.,-0.555570233019602,-0.831469612302545));
#50120=DIRECTION('center_axis',(0.,0.793353340291235,-0.608761429008721));
#50121=DIRECTION('ref_axis',(0.707106781186527,-0.430459334576891,-0.560985526796948));
#50122=DIRECTION('',(0.,0.793353340291235,-0.608761429008721));
#50123=DIRECTION('center_axis',(0.,0.608761429008721,0.793353340291235));
#50124=DIRECTION('ref_axis',(1.,0.,0.));
#50125=DIRECTION('',(-1.,0.,0.));
#50126=DIRECTION('',(0.,-0.793353340291235,0.608761429008721));
#50127=DIRECTION('center_axis',(0.,-0.793353340291235,0.608761429008721));
#50128=DIRECTION('ref_axis',(-1.,0.,0.));
#50129=DIRECTION('',(1.,0.,0.));
#50130=DIRECTION('',(0.706902428155818,-0.430583700878177,-0.561147604116297));
#50131=DIRECTION('center_axis',(0.,-0.793353340291235,0.608761429008721));
#50132=DIRECTION('ref_axis',(-0.707106781186558,-0.430459334576869,-0.560985526796926));
#50133=DIRECTION('center_axis',(1.,0.,0.));
#50134=DIRECTION('ref_axis',(0.,0.,-1.));
#50135=DIRECTION('center_axis',(1.,0.,0.));
#50136=DIRECTION('ref_axis',(0.,-0.751839807478979,-0.659345815100068));
#50137=DIRECTION('center_axis',(0.,0.60876142900872,-0.793353340291235));
#50138=DIRECTION('ref_axis',(0.707106781186524,-0.560985526796945,-0.430459334576899));
#50139=DIRECTION('',(0.,0.60876142900872,-0.793353340291235));
#50140=DIRECTION('center_axis',(0.,0.793353340291235,0.60876142900872));
#50141=DIRECTION('ref_axis',(1.,0.,0.));
#50142=DIRECTION('',(0.,-0.60876142900872,0.793353340291235));
#50143=DIRECTION('center_axis',(-1.,0.,0.));
#50144=DIRECTION('ref_axis',(0.,-0.971135373703068,0.238529004405338));
#50145=DIRECTION('',(-1.,0.,0.));
#50146=DIRECTION('center_axis',(0.,0.5,-0.866025403784439));
#50147=DIRECTION('ref_axis',(1.,0.,0.));
#50148=DIRECTION('',(-0.706902428155816,-0.61254935948098,-0.353655537588276));
#50149=DIRECTION('center_axis',(0.,0.5,-0.866025403784439));
#50150=DIRECTION('ref_axis',(0.707106781186524,-0.612372435695816,-0.353553390593283));
#50151=DIRECTION('',(1.,0.,0.));
#50152=DIRECTION('center_axis',(1.,0.,0.));
#50153=DIRECTION('ref_axis',(0.,0.,-1.));
#50154=DIRECTION('center_axis',(1.,0.,0.));
#50155=DIRECTION('ref_axis',(0.,-0.831469612302546,-0.555570233019602));
#50156=DIRECTION('center_axis',(0.,0.5,-0.866025403784439));
#50157=DIRECTION('ref_axis',(0.707106781186524,-0.612372435695816,-0.353553390593283));
#50158=DIRECTION('',(0.,0.5,-0.866025403784439));
#50159=DIRECTION('center_axis',(0.,0.866025403784439,0.5));
#50160=DIRECTION('ref_axis',(1.,0.,0.));
#50161=DIRECTION('',(-1.,0.,0.));
#50162=DIRECTION('',(0.,-0.5,0.866025403784439));
#50163=DIRECTION('center_axis',(0.,-0.5,0.866025403784439));
#50164=DIRECTION('ref_axis',(-1.,0.,0.));
#50165=DIRECTION('',(1.,0.,0.));
#50166=DIRECTION('',(0.706902428155815,-0.612549359480982,-0.353655537588275));
#50167=DIRECTION('center_axis',(0.,-0.5,0.866025403784439));
#50168=DIRECTION('ref_axis',(-0.707106781186566,-0.61237243569578,-0.353553390593262));
#50169=DIRECTION('center_axis',(1.,0.,0.));
#50170=DIRECTION('ref_axis',(0.,0.,-1.));
#50171=DIRECTION('center_axis',(1.,0.,0.));
#50172=DIRECTION('ref_axis',(0.,-0.946930129495106,-0.321439465303161));
#50173=DIRECTION('center_axis',(0.,0.25881904510252,-0.965925826289068));
#50174=DIRECTION('ref_axis',(0.707106781186522,-0.683012701892242,-0.183012701892233));
#50175=DIRECTION('',(0.,0.25881904510252,-0.965925826289068));
#50176=DIRECTION('center_axis',(0.,0.965925826289068,0.25881904510252));
#50177=DIRECTION('ref_axis',(1.,0.,0.));
#50178=DIRECTION('',(0.,-0.25881904510252,0.965925826289068));
#50179=DIRECTION('center_axis',(1.,0.,0.));
#50180=DIRECTION('ref_axis',(0.,0.,-1.));
#50181=DIRECTION('center_axis',(1.,0.,0.));
#50182=DIRECTION('ref_axis',(0.,-0.980785280403231,-0.195090322016127));
#50183=DIRECTION('center_axis',(-1.,0.,0.));
#50184=DIRECTION('ref_axis',(0.,-0.625246235020479,0.780427540257721));
#50185=DIRECTION('',(-1.,0.,0.));
#50186=DIRECTION('center_axis',(0.,-0.130526192220052,-0.99144486137381));
#50187=DIRECTION('ref_axis',(1.,0.,0.));
#50188=DIRECTION('',(-0.706902428155813,-0.701259930876582,0.0923226213578656));
#50189=DIRECTION('center_axis',(0.,-0.130526192220052,-0.99144486137381));
#50190=DIRECTION('ref_axis',(0.707106781186531,-0.701057384649994,0.0922959556412603));
#50191=DIRECTION('',(1.,0.,0.));
#50192=DIRECTION('center_axis',(-0.706790970014441,-0.701370354233847,-0.0923371588686456));
#50193=DIRECTION('ref_axis',(0.,0.130526192220056,-0.99144486137381));
#50194=DIRECTION('center_axis',(0.706796314705258,0.701365059957718,0.0923364618640549));
#50195=DIRECTION('ref_axis',(0.707106781186554,-0.70430796813559,-0.0628513008672723));
#50196=DIRECTION('center_axis',(-0.939647353856869,-0.276579550719351,-0.201411525275157));
#50197=DIRECTION('ref_axis',(0.342144487592294,-0.759583311697419,-0.553145859788346));
#50198=DIRECTION('center_axis',(1.,0.,0.));
#50199=DIRECTION('ref_axis',(0.,-0.625246235020487,-0.780427540257714));
#50200=DIRECTION('center_axis',(0.,0.99144486137381,0.130526192220051));
#50201=DIRECTION('ref_axis',(0.70710678118656,0.0922959556412558,-0.701057384649966));
#50202=DIRECTION('center_axis',(-1.49178541431117E-14,0.99144486137381,
0.130526192220056));
#50203=DIRECTION('ref_axis',(1.,1.48029736616682E-14,1.85037170770852E-15));
#50204=DIRECTION('',(0.,0.991444861373811,0.130526192220051));
#50205=DIRECTION('center_axis',(0.,0.793353340291233,-0.608761429008724));
#50206=DIRECTION('ref_axis',(-4.08878244448898E-17,-0.608761429008724,-0.793353340291233));
#50207=DIRECTION('center_axis',(0.,0.,1.));
#50208=DIRECTION('ref_axis',(1.,0.,0.));
#50209=DIRECTION('center_axis',(0.,0.130526192220051,-0.99144486137381));
#50210=DIRECTION('ref_axis',(0.70710678118652,-0.701057384650004,-0.0922959556412642));
#50211=DIRECTION('',(0.,0.130526192220051,-0.991444861373811));
#50212=DIRECTION('center_axis',(0.,0.99144486137381,0.130526192220051));
#50213=DIRECTION('ref_axis',(1.,0.,0.));
#50214=DIRECTION('',(-1.,0.,0.));
#50215=DIRECTION('',(0.,-0.130526192220051,0.991444861373811));
#50216=DIRECTION('center_axis',(0.,-0.130526192220051,0.99144486137381));
#50217=DIRECTION('ref_axis',(-1.,0.,0.));
#50218=DIRECTION('',(1.,0.,0.));
#50219=DIRECTION('center_axis',(1.,0.,0.));
#50220=DIRECTION('ref_axis',(0.,0.,-1.));
#50221=DIRECTION('center_axis',(1.,0.,0.));
#50222=DIRECTION('ref_axis',(0.,-0.997858923238603,0.0654031292301436));
#50223=DIRECTION('center_axis',(0.,-0.130526192220052,-0.99144486137381));
#50224=DIRECTION('ref_axis',(0.707106781186531,-0.701057384649994,0.0922959556412603));
#50225=DIRECTION('center_axis',(0.,0.130526192220052,0.99144486137381));
#50226=DIRECTION('ref_axis',(0.707106781186531,-0.701057384649994,0.0922959556412603));
#50227=DIRECTION('',(0.,-0.130526192220052,-0.99144486137381));
#50228=DIRECTION('center_axis',(0.,0.99144486137381,-0.130526192220052));
#50229=DIRECTION('ref_axis',(1.,0.,0.));
#50230=DIRECTION('',(-1.,0.,0.));
#50231=DIRECTION('',(0.,0.130526192220052,0.99144486137381));
#50232=DIRECTION('center_axis',(1.,0.,0.));
#50233=DIRECTION('ref_axis',(0.,0.,-1.));
#50234=DIRECTION('center_axis',(1.,0.,0.));
#50235=DIRECTION('ref_axis',(0.,-0.98078528040323,0.195090322016129));
#50236=DIRECTION('center_axis',(0.,-0.258819045102521,-0.965925826289068));
#50237=DIRECTION('ref_axis',(0.707106781186512,-0.683012701892253,0.18301270189223));
#50238=DIRECTION('',(0.,-0.258819045102521,-0.965925826289068));
#50239=DIRECTION('center_axis',(0.,0.965925826289068,-0.258819045102521));
#50240=DIRECTION('ref_axis',(1.,0.,0.));
#50241=DIRECTION('',(-1.,0.,0.));
#50242=DIRECTION('',(0.,0.258819045102521,0.965925826289068));
#50243=DIRECTION('center_axis',(0.,0.258819045102521,0.965925826289068));
#50244=DIRECTION('ref_axis',(-1.,0.,0.));
#50245=DIRECTION('',(1.,0.,0.));
#50246=DIRECTION('',(0.706902428155814,-0.683210034733323,0.183065577067632));
#50247=DIRECTION('center_axis',(0.,0.258819045102521,0.965925826289068));
#50248=DIRECTION('ref_axis',(-0.707106781186564,-0.683012701892201,0.183012701892222));
#50249=DIRECTION('center_axis',(-1.,0.,0.));
#50250=DIRECTION('ref_axis',(0.,-0.27899550949708,0.960292406343227));
#50251=DIRECTION('',(-1.,0.,0.));
#50252=DIRECTION('center_axis',(0.,-0.5,-0.866025403784438));
#50253=DIRECTION('ref_axis',(1.,0.,0.));
#50254=DIRECTION('',(-0.706902428155822,-0.612549359480972,0.353655537588279));
#50255=DIRECTION('center_axis',(0.,-0.5,-0.866025403784438));
#50256=DIRECTION('ref_axis',(0.707106781186515,-0.612372435695829,0.353553390593278));
#50257=DIRECTION('',(1.,0.,0.));
#50258=DIRECTION('center_axis',(1.,0.,0.));
#50259=DIRECTION('ref_axis',(0.,0.,-1.));
#50260=DIRECTION('center_axis',(1.,0.,0.));
#50261=DIRECTION('ref_axis',(0.,-0.896872741532688,0.442288690219002));
#50262=DIRECTION('center_axis',(0.,-0.5,-0.866025403784438));
#50263=DIRECTION('ref_axis',(0.707106781186515,-0.612372435695829,0.353553390593278));
#50264=DIRECTION('',(0.,-0.5,-0.866025403784438));
#50265=DIRECTION('center_axis',(0.,0.866025403784438,-0.5));
#50266=DIRECTION('ref_axis',(1.,0.,0.));
#50267=DIRECTION('',(0.,0.5,0.866025403784438));
#50268=DIRECTION('center_axis',(1.,0.,0.));
#50269=DIRECTION('ref_axis',(0.,0.,-1.));
#50270=DIRECTION('center_axis',(1.,0.,0.));
#50271=DIRECTION('ref_axis',(0.,-0.831469612302545,0.555570233019602));
#50272=DIRECTION('center_axis',(0.,-0.608761429008721,-0.793353340291235));
#50273=DIRECTION('ref_axis',(0.707106781186509,-0.560985526796955,0.430459334576911));
#50274=DIRECTION('',(0.,-0.608761429008721,-0.793353340291235));
#50275=DIRECTION('center_axis',(0.,0.793353340291235,-0.608761429008721));
#50276=DIRECTION('ref_axis',(1.,0.,0.));
#50277=DIRECTION('',(-1.,0.,0.));
#50278=DIRECTION('',(0.,0.608761429008721,0.793353340291235));
#50279=DIRECTION('center_axis',(0.,0.608761429008721,0.793353340291235));
#50280=DIRECTION('ref_axis',(-1.,0.,0.));
#50281=DIRECTION('',(1.,0.,0.));
#50282=DIRECTION('',(0.706902428155816,-0.561147604116301,0.430583700878176));
#50283=DIRECTION('center_axis',(0.,0.608761429008721,0.793353340291235));
#50284=DIRECTION('ref_axis',(-0.707106781186551,-0.560985526796921,0.430459334576886));
#50285=DIRECTION('center_axis',(1.,0.,0.));
#50286=DIRECTION('ref_axis',(0.,0.,-1.));
#50287=DIRECTION('center_axis',(1.,0.,0.));
#50288=DIRECTION('ref_axis',(0.,-0.659345815100069,0.751839807478978));
#50289=DIRECTION('center_axis',(0.,-0.793353340291235,-0.60876142900872));
#50290=DIRECTION('ref_axis',(0.707106781186524,-0.430459334576899,0.560985526796945));
#50291=DIRECTION('',(0.,-0.793353340291235,-0.60876142900872));
#50292=DIRECTION('center_axis',(0.,0.60876142900872,-0.793353340291235));
#50293=DIRECTION('ref_axis',(1.,0.,0.));
#50294=DIRECTION('',(0.,0.793353340291235,0.60876142900872));
#50295=DIRECTION('center_axis',(-1.,0.,0.));
#50296=DIRECTION('ref_axis',(0.,0.238529004405333,0.971135373703069));
#50297=DIRECTION('',(-1.,0.,0.));
#50298=DIRECTION('center_axis',(0.,-0.866025403784439,-0.5));
#50299=DIRECTION('ref_axis',(1.,0.,0.));
#50300=DIRECTION('',(-0.706902428155816,-0.353655537588276,0.61254935948098));
#50301=DIRECTION('center_axis',(0.,-0.866025403784439,-0.5));
#50302=DIRECTION('ref_axis',(0.707106781186511,-0.353553390593292,0.612372435695826));
#50303=DIRECTION('',(1.,0.,0.));
#50304=DIRECTION('center_axis',(1.,0.,0.));
#50305=DIRECTION('ref_axis',(0.,0.,-1.));
#50306=DIRECTION('center_axis',(1.,0.,0.));
#50307=DIRECTION('ref_axis',(0.,-0.555570233019602,0.831469612302545));
#50308=DIRECTION('center_axis',(0.,-0.866025403784439,-0.5));
#50309=DIRECTION('ref_axis',(0.707106781186511,-0.353553390593292,0.612372435695826));
#50310=DIRECTION('',(0.,-0.866025403784439,-0.5));
#50311=DIRECTION('center_axis',(0.,0.5,-0.866025403784439));
#50312=DIRECTION('ref_axis',(1.,0.,0.));
#50313=DIRECTION('',(-1.,0.,0.));
#50314=DIRECTION('',(0.,0.866025403784439,0.5));
#50315=DIRECTION('center_axis',(0.,0.866025403784439,0.5));
#50316=DIRECTION('ref_axis',(-1.,0.,0.));
#50317=DIRECTION('',(1.,0.,0.));
#50318=DIRECTION('',(0.706902428155815,-0.353655537588275,0.612549359480982));
#50319=DIRECTION('center_axis',(0.,0.866025403784439,0.5));
#50320=DIRECTION('ref_axis',(-0.707106781186554,-0.353553390593267,0.612372435695791));
#50321=DIRECTION('center_axis',(1.,0.,0.));
#50322=DIRECTION('ref_axis',(0.,0.,-1.));
#50323=DIRECTION('center_axis',(1.,0.,0.));
#50324=DIRECTION('ref_axis',(0.,-0.321439465303161,0.946930129495106));
#50325=DIRECTION('center_axis',(0.,-0.965925826289068,-0.258819045102521));
#50326=DIRECTION('ref_axis',(0.707106781186523,-0.183012701892228,0.683012701892242));
#50327=DIRECTION('',(0.,-0.965925826289068,-0.258819045102521));
#50328=DIRECTION('center_axis',(0.,0.258819045102521,-0.965925826289068));
#50329=DIRECTION('ref_axis',(1.,0.,0.));
#50330=DIRECTION('',(0.,0.965925826289068,0.258819045102521));
#50331=DIRECTION('center_axis',(1.,0.,0.));
#50332=DIRECTION('ref_axis',(0.,0.,-1.));
#50333=DIRECTION('center_axis',(1.,0.,0.));
#50334=DIRECTION('ref_axis',(0.,-0.195090322016128,0.980785280403231));
#50335=DIRECTION('center_axis',(-1.,0.,0.));
#50336=DIRECTION('ref_axis',(0.,0.780427540257713,0.625246235020488));
#50337=DIRECTION('',(-1.,0.,0.));
#50338=DIRECTION('center_axis',(0.,-0.99144486137381,0.130526192220052));
#50339=DIRECTION('ref_axis',(1.,0.,0.));
#50340=DIRECTION('',(-0.706902428155813,0.0923226213578656,0.701259930876582));
#50341=DIRECTION('center_axis',(0.,-0.99144486137381,0.130526192220052));
#50342=DIRECTION('ref_axis',(0.707106781186521,0.0922959556412538,0.701057384650005));
#50343=DIRECTION('',(1.,0.,0.));
#50344=DIRECTION('center_axis',(-0.706790970014375,-0.0923371588686543,
0.701370354233913));
#50345=DIRECTION('ref_axis',(0.,-0.99144486137381,-0.130526192220056));
#50346=DIRECTION('center_axis',(0.70679631470526,0.0923364618639818,-0.701365059957726));
#50347=DIRECTION('ref_axis',(0.707106781186553,-0.0628513008672796,0.70430796813559));
#50348=DIRECTION('center_axis',(0.,0.,1.));
#50349=DIRECTION('ref_axis',(1.,0.,0.));
#50350=DIRECTION('center_axis',(1.,0.,0.));
#50351=DIRECTION('ref_axis',(0.,-0.780427540257714,0.625246235020487));
#50352=DIRECTION('center_axis',(0.,0.130526192220051,-0.99144486137381));
#50353=DIRECTION('ref_axis',(0.707106781186557,-0.701057384649968,-0.092295955641258));
#50354=DIRECTION('center_axis',(-1.46763321699128E-14,0.130526192220054,
-0.99144486137381));
#50355=DIRECTION('ref_axis',(1.,0.,-1.48029736616682E-14));
#50356=DIRECTION('',(0.,0.130526192220051,-0.991444861373811));
#50357=DIRECTION('center_axis',(0.,-0.60876142900873,-0.793353340291228));
#50358=DIRECTION('ref_axis',(-1.63551297779558E-16,-0.793353340291228,0.60876142900873));
#50359=DIRECTION('center_axis',(0.,0.,1.));
#50360=DIRECTION('ref_axis',(1.,0.,0.));
#50361=DIRECTION('center_axis',(0.,-0.99144486137381,-0.130526192220051));
#50362=DIRECTION('ref_axis',(0.70710678118652,-0.0922959556412642,0.701057384650004));
#50363=DIRECTION('',(0.,-0.991444861373811,-0.130526192220051));
#50364=DIRECTION('center_axis',(0.,0.130526192220051,-0.99144486137381));
#50365=DIRECTION('ref_axis',(1.,0.,0.));
#50366=DIRECTION('',(-1.,0.,0.));
#50367=DIRECTION('',(0.,0.991444861373811,0.130526192220051));
#50368=DIRECTION('center_axis',(0.,0.99144486137381,0.130526192220051));
#50369=DIRECTION('ref_axis',(-1.,0.,0.));
#50370=DIRECTION('',(1.,0.,0.));
#50371=DIRECTION('center_axis',(1.,0.,0.));
#50372=DIRECTION('ref_axis',(0.,0.,-1.));
#50373=DIRECTION('center_axis',(1.,0.,0.));
#50374=DIRECTION('ref_axis',(0.,0.0654031292301431,0.997858923238603));
#50375=DIRECTION('center_axis',(0.,-0.99144486137381,0.130526192220052));
#50376=DIRECTION('ref_axis',(0.707106781186521,0.0922959556412538,0.701057384650005));
#50377=DIRECTION('',(0.,-0.99144486137381,0.130526192220052));
#50378=DIRECTION('center_axis',(0.,-0.130526192220052,-0.99144486137381));
#50379=DIRECTION('ref_axis',(1.,0.,0.));
#50380=DIRECTION('',(0.,0.99144486137381,-0.130526192220052));
#50381=DIRECTION('center_axis',(1.,0.,0.));
#50382=DIRECTION('ref_axis',(0.,0.,-1.));
#50383=DIRECTION('center_axis',(1.,0.,0.));
#50384=DIRECTION('ref_axis',(0.,0.195090322016129,0.98078528040323));
#50385=DIRECTION('center_axis',(-1.,0.,0.));
#50386=DIRECTION('ref_axis',(0.,0.96029240634322,0.278995509497103));
#50387=DIRECTION('',(-1.,0.,0.));
#50388=DIRECTION('center_axis',(0.,-0.866025403784439,0.5));
#50389=DIRECTION('ref_axis',(1.,0.,0.));
#50390=DIRECTION('',(-0.706902428155818,0.35365553758828,0.612549359480975));
#50391=DIRECTION('center_axis',(0.,-0.866025403784439,0.5));
#50392=DIRECTION('ref_axis',(0.70710678118651,0.353553390593297,0.612372435695825));
#50393=DIRECTION('',(1.,0.,0.));
#50394=DIRECTION('center_axis',(-0.706790970015311,0.183094403348125,0.683317615876694));
#50395=DIRECTION('ref_axis',(0.,-0.965925826289067,0.258819045102527));
#50396=DIRECTION('center_axis',(0.706796314705268,-0.183093021264932,-0.683312457872042));
#50397=DIRECTION('ref_axis',(0.707106781186546,0.211459960225213,0.674747867889595));
#50398=DIRECTION('center_axis',(1.,0.,0.));
#50399=DIRECTION('ref_axis',(0.,0.,-1.));
#50400=DIRECTION('center_axis',(1.,0.,0.));
#50401=DIRECTION('ref_axis',(0.,0.325283431446442,0.945616565647212));
#50402=DIRECTION('center_axis',(2.44475116993405E-14,0.95423758595179,-0.299049543649378));
#50403=DIRECTION('ref_axis',(0.,0.299049543649378,0.95423758595179));
#50404=DIRECTION('center_axis',(-0.0772950468865003,-0.97541857010173,-0.206359125864377));
#50405=DIRECTION('ref_axis',(0.342144487592297,-0.220360189464209,0.913443231136726));
#50406=DIRECTION('center_axis',(1.,0.,0.));
#50407=DIRECTION('ref_axis',(0.,-0.481749655761245,0.876308889133233));
#50408=DIRECTION('center_axis',(0.,-0.258819045102521,-0.965925826289068));
#50409=DIRECTION('ref_axis',(0.707106781186557,-0.68301270189221,0.18301270189222));
#50410=DIRECTION('center_axis',(1.42985745656822E-14,-0.258819045102523,
-0.965925826289068));
#50411=DIRECTION('ref_axis',(1.,0.,1.48029736616682E-14));
#50412=DIRECTION('',(0.,-0.258819045102521,-0.965925826289068));
#50413=DIRECTION('center_axis',(0.,0.86602540378444,0.499999999999998));
#50414=DIRECTION('ref_axis',(0.,-0.499999999999998,0.86602540378444));
#50415=DIRECTION('center_axis',(0.,-0.965925826289068,0.258819045102521));
#50416=DIRECTION('ref_axis',(0.707106781186512,0.18301270189223,0.683012701892253));
#50417=DIRECTION('',(0.,-0.965925826289068,0.258819045102521));
#50418=DIRECTION('center_axis',(0.,0.,1.));
#50419=DIRECTION('ref_axis',(1.,0.,0.));
#50420=DIRECTION('center_axis',(0.,-0.923879532511287,0.38268343236509));
#50421=DIRECTION('ref_axis',(1.,0.,0.));
#50422=DIRECTION('',(1.,0.,0.));
#50423=DIRECTION('center_axis',(0.,-0.923879532511287,0.38268343236509));
#50424=DIRECTION('ref_axis',(-0.707106781186561,0.270598050073091,0.653281482438177));
#50425=DIRECTION('',(-0.706902428155818,-0.270676229998407,-0.653470225474167));
#50426=DIRECTION('center_axis',(0.,0.965925826289068,-0.258819045102521));
#50427=DIRECTION('ref_axis',(-1.,0.,0.));
#50428=DIRECTION('',(1.,0.,0.));
#50429=DIRECTION('',(0.706902428155814,0.183065577067632,0.683210034733323));
#50430=DIRECTION('center_axis',(0.,0.965925826289068,-0.258819045102521));
#50431=DIRECTION('ref_axis',(-0.707106781186554,0.183012701892219,0.683012701892212));
#50432=DIRECTION('',(-1.,0.,0.));
#50433=DIRECTION('center_axis',(1.,0.,0.));
#50434=DIRECTION('ref_axis',(0.,0.,-1.));
#50435=DIRECTION('center_axis',(1.,0.,0.));
#50436=DIRECTION('ref_axis',(0.,0.442288690219001,0.896872741532688));
#50437=DIRECTION('center_axis',(0.,-0.866025403784439,0.5));
#50438=DIRECTION('ref_axis',(0.70710678118651,0.353553390593297,0.612372435695825));
#50439=DIRECTION('',(0.,-0.866025403784439,0.5));
#50440=DIRECTION('center_axis',(0.,-0.5,-0.866025403784439));
#50441=DIRECTION('ref_axis',(1.,0.,0.));
#50442=DIRECTION('',(0.,0.866025403784439,-0.5));
#50443=DIRECTION('center_axis',(1.,0.,0.));
#50444=DIRECTION('ref_axis',(0.,0.,-1.));
#50445=DIRECTION('center_axis',(1.,0.,0.));
#50446=DIRECTION('ref_axis',(0.,0.555570233019602,0.831469612302545));
#50447=DIRECTION('center_axis',(0.,-0.793353340291235,0.608761429008721));
#50448=DIRECTION('ref_axis',(0.707106781186516,0.430459334576894,0.56098552679696));
#50449=DIRECTION('',(0.,-0.793353340291235,0.608761429008721));
#50450=DIRECTION('center_axis',(0.,-0.608761429008721,-0.793353340291235));
#50451=DIRECTION('ref_axis',(1.,0.,0.));
#50452=DIRECTION('',(-1.,0.,0.));
#50453=DIRECTION('',(0.,0.793353340291235,-0.608761429008721));
#50454=DIRECTION('center_axis',(0.,0.793353340291235,-0.608761429008721));
#50455=DIRECTION('ref_axis',(-1.,0.,0.));
#50456=DIRECTION('',(1.,0.,0.));
#50457=DIRECTION('',(0.706902428155819,0.430583700878174,0.561147604116299));
#50458=DIRECTION('center_axis',(0.,0.793353340291235,-0.608761429008721));
#50459=DIRECTION('ref_axis',(-0.707106781186558,0.430459334576869,0.560985526796926));
#50460=DIRECTION('center_axis',(1.,0.,0.));
#50461=DIRECTION('ref_axis',(0.,0.,-1.));
#50462=DIRECTION('center_axis',(1.,0.,0.));
#50463=DIRECTION('ref_axis',(0.,0.751839807478977,0.659345815100069));
#50464=DIRECTION('center_axis',(-1.,0.,0.));
#50465=DIRECTION('ref_axis',(0.,0.971135373703069,-0.238529004405333));
#50466=DIRECTION('',(-1.,0.,0.));
#50467=DIRECTION('center_axis',(0.,-0.5,0.866025403784439));
#50468=DIRECTION('ref_axis',(1.,0.,0.));
#50469=DIRECTION('',(-0.706902428155818,0.612549359480981,0.35365553758827));
#50470=DIRECTION('center_axis',(0.,-0.5,0.866025403784439));
#50471=DIRECTION('ref_axis',(0.707106781186512,0.612372435695827,0.353553390593288));
#50472=DIRECTION('',(1.,0.,0.));
#50473=DIRECTION('center_axis',(0.,-0.608761429008721,0.793353340291235));
#50474=DIRECTION('ref_axis',(0.707106781186524,0.560985526796945,0.430459334576899));
#50475=DIRECTION('',(0.,-0.608761429008721,0.793353340291235));
#50476=DIRECTION('center_axis',(0.,-0.793353340291235,-0.608761429008721));
#50477=DIRECTION('ref_axis',(1.,0.,0.));
#50478=DIRECTION('',(0.,0.608761429008721,-0.793353340291235));
#50479=DIRECTION('center_axis',(1.,0.,0.));
#50480=DIRECTION('ref_axis',(0.,0.,-1.));
#50481=DIRECTION('center_axis',(1.,0.,0.));
#50482=DIRECTION('ref_axis',(0.,0.831469612302545,0.555570233019602));
#50483=DIRECTION('center_axis',(0.,-0.5,0.866025403784439));
#50484=DIRECTION('ref_axis',(0.707106781186512,0.612372435695827,0.353553390593288));
#50485=DIRECTION('',(0.,-0.5,0.866025403784439));
#50486=DIRECTION('center_axis',(0.,-0.866025403784439,-0.5));
#50487=DIRECTION('ref_axis',(1.,0.,0.));
#50488=DIRECTION('',(-1.,0.,0.));
#50489=DIRECTION('',(0.,0.5,-0.866025403784439));
#50490=DIRECTION('center_axis',(0.,0.5,-0.866025403784439));
#50491=DIRECTION('ref_axis',(-1.,0.,0.));
#50492=DIRECTION('',(1.,0.,0.));
#50493=DIRECTION('',(0.706902428155815,0.612549359480982,0.353655537588275));
#50494=DIRECTION('center_axis',(0.,0.5,-0.866025403784439));
#50495=DIRECTION('ref_axis',(-0.707106781186565,0.612372435695779,0.353553390593267));
#50496=DIRECTION('center_axis',(0.,1.,0.));
#50497=DIRECTION('ref_axis',(-0.707106781186561,0.,0.707106781186534));
#50498=DIRECTION('center_axis',(0.,-1.,0.));
#50499=DIRECTION('ref_axis',(0.,0.,1.));
#50500=DIRECTION('center_axis',(0.,-0.70710678118655,0.707106781186545));
#50501=DIRECTION('ref_axis',(4.08878244448901E-17,0.707106781186545,0.70710678118655));
#50502=DIRECTION('',(0.,1.,0.));
#50503=DIRECTION('center_axis',(-0.706796314700315,-0.70741711141734,0.));
#50504=DIRECTION('ref_axis',(0.,0.,1.));
#50505=DIRECTION('center_axis',(0.706790970013439,0.70742245137362,0.));
#50506=DIRECTION('ref_axis',(-0.707106781191846,0.706475581614969,-0.0298705971533396));
#50507=DIRECTION('center_axis',(-0.429570054990523,0.17777491004016,-0.885361874724484));
#50508=DIRECTION('ref_axis',(-0.81807461755933,0.338555120062927,0.464902517506986));
#50509=DIRECTION('center_axis',(0.,0.0422434036107609,0.999107349012797));
#50510=DIRECTION('ref_axis',(0.,0.999107349012797,-0.0422434036107609));
#50511=DIRECTION('center_axis',(1.,0.,0.));
#50512=DIRECTION('ref_axis',(0.,0.721763401937886,0.692139864205963));
#50513=DIRECTION('',(-1.,0.,0.));
#50514=DIRECTION('center_axis',(1.,0.,0.));
#50515=DIRECTION('ref_axis',(0.,0.999122446012244,-0.0418848167539264));
#50516=DIRECTION('',(1.,0.,0.));
#50517=DIRECTION('center_axis',(1.,0.,0.));
#50518=DIRECTION('ref_axis',(0.,0.,-1.));
#50519=DIRECTION('center_axis',(-1.,0.,0.));
#50520=DIRECTION('ref_axis',(0.,0.998116370642493,-0.0613490884647577));
#50521=DIRECTION('center_axis',(-1.06478709491899E-17,0.088885162099298,
0.996041880624797));
#50522=DIRECTION('ref_axis',(0.707106781186568,0.704307968135575,-0.0628513008672772));
#50523=DIRECTION('center_axis',(1.,0.,0.));
#50524=DIRECTION('ref_axis',(0.,0.998116370642493,-0.0613490884647578));
#50525=DIRECTION('center_axis',(-0.939647353864408,-0.300502853768332,-0.163587546141829));
#50526=DIRECTION('ref_axis',(-0.342144487571591,0.825284993998467,0.449268102924437));
#50527=DIRECTION('center_axis',(0.,0.0418848167539202,0.999122446012245));
#50528=DIRECTION('ref_axis',(0.,0.999122446012244,-0.0418848167539202));
#50529=DIRECTION('center_axis',(-0.939647353856791,0.276579550719521,-0.201411525275291));
#50530=DIRECTION('ref_axis',(0.342144487592485,0.75958331169735,-0.553145859788322));
#50531=DIRECTION('center_axis',(1.,0.,0.));
#50532=DIRECTION('ref_axis',(0.,0.625246235020501,-0.780427540257703));
#50533=DIRECTION('center_axis',(1.,0.,0.));
#50534=DIRECTION('ref_axis',(0.,0.,-1.));
#50535=DIRECTION('center_axis',(-1.,0.,0.));
#50536=DIRECTION('ref_axis',(0.,0.997858923238603,-0.0654031292301437));
#50537=DIRECTION('center_axis',(0.,-0.0885276724488827,-0.996073717759275));
#50538=DIRECTION('ref_axis',(0.,0.996073717759275,-0.0885276724488827));
#50539=DIRECTION('center_axis',(1.,0.,0.));
#50540=DIRECTION('ref_axis',(0.,1.,0.));
#50541=DIRECTION('center_axis',(1.,0.,0.));
#50542=DIRECTION('ref_axis',(0.,0.998116370642493,-0.0613490884647577));
#50543=DIRECTION('center_axis',(1.,0.,0.));
#50544=DIRECTION('ref_axis',(0.,0.,-1.));
#50545=DIRECTION('center_axis',(-1.,0.,0.));
#50546=DIRECTION('ref_axis',(0.,0.998116370642493,-0.0613490884647578));
#50547=DIRECTION('center_axis',(1.06478709491899E-17,0.088885162099298,
0.996041880624797));
#50548=DIRECTION('ref_axis',(0.,0.996041880624797,-0.088885162099298));
#50549=DIRECTION('center_axis',(1.,0.,0.));
#50550=DIRECTION('ref_axis',(0.,1.,0.));
#50551=DIRECTION('',(1.,0.,0.));
#50552=DIRECTION('center_axis',(-1.,0.,0.));
#50553=DIRECTION('ref_axis',(0.,0.6252462350205,-0.780427540257704));
#50554=DIRECTION('center_axis',(-1.,0.,0.));
#50555=DIRECTION('ref_axis',(0.,0.625246235020501,-0.780427540257703));
#50556=DIRECTION('center_axis',(0.,0.99144486137381,0.130526192220052));
#50557=DIRECTION('ref_axis',(-0.707106781186562,-0.0922959556412482,0.701057384649965));
#50558=DIRECTION('center_axis',(0.,-0.99144486137381,-0.130526192220056));
#50559=DIRECTION('ref_axis',(0.,-0.130526192220056,0.99144486137381));
#50560=DIRECTION('center_axis',(0.,-0.793353340291238,0.608761429008717));
#50561=DIRECTION('ref_axis',(4.08878244448902E-17,0.608761429008717,0.793353340291238));
#50562=DIRECTION('',(0.,0.99144486137381,0.130526192220052));
#50563=DIRECTION('center_axis',(0.,1.,0.));
#50564=DIRECTION('ref_axis',(0.707106781186561,0.,-0.707106781186534));
#50565=DIRECTION('center_axis',(0.,-1.,0.));
#50566=DIRECTION('ref_axis',(0.,0.,-1.));
#50567=DIRECTION('center_axis',(0.,-0.70710678118655,-0.707106781186545));
#50568=DIRECTION('ref_axis',(-4.08878244448901E-17,0.707106781186545,-0.70710678118655));
#50569=DIRECTION('',(0.,1.,0.));
#50570=DIRECTION('center_axis',(0.706796314700315,-0.70741711141734,0.));
#50571=DIRECTION('ref_axis',(0.,0.,-1.));
#50572=DIRECTION('center_axis',(-0.706790970013424,0.707422451373635,0.));
#50573=DIRECTION('ref_axis',(0.707106781191861,0.706475581614954,0.0298705971533402));
#50574=DIRECTION('center_axis',(-0.429570054990522,-0.177774910040183,-0.885361874724479));
#50575=DIRECTION('ref_axis',(0.818074617559305,0.33855512006296,-0.464902517507005));
#50576=DIRECTION('center_axis',(0.,0.0422434036107609,-0.999107349012797));
#50577=DIRECTION('ref_axis',(0.,0.999107349012797,0.0422434036107609));
#50578=DIRECTION('center_axis',(1.,0.,0.));
#50579=DIRECTION('ref_axis',(0.,0.,-1.));
#50580=DIRECTION('center_axis',(1.,0.,0.));
#50581=DIRECTION('ref_axis',(0.,0.998116370642493,0.0613490884647571));
#50582=DIRECTION('center_axis',(-1.25644877200442E-15,0.0888851620992974,
-0.996041880624797));
#50583=DIRECTION('ref_axis',(-0.707106781186561,0.704307968135582,0.0628513008672784));
#50584=DIRECTION('center_axis',(-1.,0.,0.));
#50585=DIRECTION('ref_axis',(0.,0.998116370642494,0.061349088464757));
#50586=DIRECTION('center_axis',(-1.,0.,0.));
#50587=DIRECTION('ref_axis',(0.,0.721763401937886,-0.692139864205963));
#50588=DIRECTION('',(1.,0.,0.));
#50589=DIRECTION('center_axis',(-1.,0.,0.));
#50590=DIRECTION('ref_axis',(0.,0.999122446012244,0.0418848167539264));
#50591=DIRECTION('',(-1.,0.,0.));
#50592=DIRECTION('center_axis',(-0.939647353864401,0.300502853768353,-0.163587546141832));
#50593=DIRECTION('ref_axis',(0.34214448757159,0.825284993998465,-0.449268102924442));
#50594=DIRECTION('center_axis',(0.,0.0418848167539202,-0.999122446012245));
#50595=DIRECTION('ref_axis',(0.,0.999122446012244,0.0418848167539202));
#50596=DIRECTION('center_axis',(-0.706796314705253,-0.701365059957732,-0.0923364618639934));
#50597=DIRECTION('ref_axis',(0.,-0.130526192220085,0.991444861373806));
#50598=DIRECTION('center_axis',(0.706790970014375,0.701370354233913,0.0923371588686543));
#50599=DIRECTION('ref_axis',(-0.707106781190911,0.704330480384932,0.0625985175108835));
#50600=DIRECTION('center_axis',(-0.939647353856844,-0.276579550719404,-0.201411525275205));
#50601=DIRECTION('ref_axis',(-0.34214448759234,0.759583311697393,0.553145859788353));
#50602=DIRECTION('center_axis',(-1.,0.,0.));
#50603=DIRECTION('ref_axis',(0.,0.625246235020486,0.780427540257715));
#50604=DIRECTION('center_axis',(0.,0.,1.));
#50605=DIRECTION('ref_axis',(-0.923502716555982,-0.383591882752648,0.));
#50606=DIRECTION('center_axis',(0.,-0.0885276724488875,0.996073717759274));
#50607=DIRECTION('ref_axis',(0.,0.996073717759274,0.0885276724488875));
#50608=DIRECTION('center_axis',(1.,0.,0.));
#50609=DIRECTION('ref_axis',(0.,1.,0.));
#50610=DIRECTION('',(-1.,0.,0.));
#50611=DIRECTION('center_axis',(1.,0.,0.));
#50612=DIRECTION('ref_axis',(0.,0.998116370642494,0.061349088464757));
#50613=DIRECTION('center_axis',(1.,0.,0.));
#50614=DIRECTION('ref_axis',(0.,0.625246235020487,0.780427540257714));
#50615=DIRECTION('',(1.,0.,0.));
#50616=DIRECTION('center_axis',(1.,0.,0.));
#50617=DIRECTION('ref_axis',(0.,0.625246235020486,0.780427540257715));
#50618=DIRECTION('center_axis',(0.,0.130526192220052,-0.99144486137381));
#50619=DIRECTION('ref_axis',(-1.,0.,0.));
#50620=DIRECTION('',(-1.,0.,0.));
#50621=DIRECTION('center_axis',(0.,0.130526192220052,-0.99144486137381));
#50622=DIRECTION('ref_axis',(0.707106781186521,0.701057384650005,0.092295955641259));
#50623=DIRECTION('center_axis',(1.,0.,0.));
#50624=DIRECTION('ref_axis',(0.,0.,-1.));
#50625=DIRECTION('center_axis',(-1.,0.,0.));
#50626=DIRECTION('ref_axis',(0.,0.997858923238603,0.065403129230143));
#50627=DIRECTION('center_axis',(1.,0.,0.));
#50628=DIRECTION('ref_axis',(0.,1.,0.));
#50629=DIRECTION('',(-0.706902428155817,-0.707311075176552,0.));
#50630=DIRECTION('center_axis',(1.,0.,0.));
#50631=DIRECTION('ref_axis',(0.,0.,-1.));
#50632=DIRECTION('center_axis',(1.,0.,0.));
#50633=DIRECTION('ref_axis',(0.,0.997858923238603,0.065403129230143));
#50634=DIRECTION('center_axis',(0.706796314705259,-0.70136505995772,-0.092336461864034));
#50635=DIRECTION('ref_axis',(0.707106781186553,0.70430796813559,0.0628513008672796));
#50636=DIRECTION('center_axis',(1.,0.,0.));
#50637=DIRECTION('ref_axis',(0.,0.,-1.));
#50638=DIRECTION('center_axis',(1.25644877200442E-15,0.0888851620992974,
-0.996041880624797));
#50639=DIRECTION('ref_axis',(0.,0.996041880624796,0.0888851620992974));
#50640=DIRECTION('center_axis',(-1.,0.,0.));
#50641=DIRECTION('ref_axis',(0.,0.998116370642493,0.0613490884647571));
#50642=DIRECTION('center_axis',(-0.939647353856868,0.27657955071935,0.201411525275163));
#50643=DIRECTION('ref_axis',(0.342144487592292,0.759583311697414,0.553145859788354));
#50644=DIRECTION('center_axis',(-1.,0.,0.));
#50645=DIRECTION('ref_axis',(0.,1.,0.));
#50646=DIRECTION('center_axis',(0.,0.,1.));
#50647=DIRECTION('ref_axis',(1.,0.,0.));
#50648=DIRECTION('',(1.,0.,0.));
#50649=DIRECTION('center_axis',(0.,0.,1.));
#50650=DIRECTION('ref_axis',(-0.707106781186568,0.707106781186527,0.));
#50651=DIRECTION('center_axis',(0.70679097001436,0.701370354233927,-0.0923371588686562));
#50652=DIRECTION('ref_axis',(0.,-0.130526192220056,-0.99144486137381));
#50653=DIRECTION('center_axis',(-0.706796314705254,-0.701365059957736,0.0923364618639516));
#50654=DIRECTION('ref_axis',(-0.707106781186561,0.704307968135582,-0.0628513008672803));
#50655=DIRECTION('center_axis',(0.,-0.99144486137381,0.130526192220053));
#50656=DIRECTION('ref_axis',(-0.707106781186559,-0.0922959556412688,-0.701057384649965));
#50657=DIRECTION('center_axis',(2.4152197319893E-16,-0.99144486137381,0.130526192220056));
#50658=DIRECTION('ref_axis',(-1.,0.,1.85037170770863E-15));
#50659=DIRECTION('center_axis',(0.,-0.793353340291234,-0.608761429008722));
#50660=DIRECTION('ref_axis',(4.08878244448899E-17,0.608761429008722,-0.793353340291234));
#50661=DIRECTION('center_axis',(0.,0.,1.));
#50662=DIRECTION('ref_axis',(-0.923502716555893,-0.383591882752863,0.));
#50663=DIRECTION('center_axis',(-0.939647353856834,-0.276579550719425,0.201411525275222));
#50664=DIRECTION('ref_axis',(-0.342144487592389,0.759583311697371,-0.553145859788353));
#50665=DIRECTION('center_axis',(1.,0.,0.));
#50666=DIRECTION('ref_axis',(0.,0.,-1.));
#50667=DIRECTION('center_axis',(-1.,0.,0.));
#50668=DIRECTION('ref_axis',(0.,-1.,1.83697019872103E-16));
#50669=DIRECTION('center_axis',(-1.,0.,0.));
#50670=DIRECTION('ref_axis',(0.,-1.,1.83697019872103E-16));
#50671=DIRECTION('center_axis',(0.,-1.,-1.22464679914735E-16));
#50672=DIRECTION('ref_axis',(0.,-1.22464679914735E-16,1.));
#50673=DIRECTION('center_axis',(1.,0.,0.));
#50674=DIRECTION('ref_axis',(0.,1.,0.));
#50675=DIRECTION('',(-1.,0.,0.));
#50676=DIRECTION('center_axis',(1.,0.,0.));
#50677=DIRECTION('ref_axis',(0.,-1.,1.83697019872103E-16));
#50678=DIRECTION('center_axis',(1.,0.,0.));
#50679=DIRECTION('ref_axis',(0.,-1.,1.83697019872103E-16));
#50680=DIRECTION('center_axis',(1.,0.,0.));
#50681=DIRECTION('ref_axis',(0.,0.,-1.));
#50682=DIRECTION('center_axis',(1.,0.,0.));
#50683=DIRECTION('ref_axis',(0.,0.980785280403231,0.195090322016128));
#50684=DIRECTION('center_axis',(0.706796314705266,-0.683312457872038,-0.183093021264955));
#50685=DIRECTION('ref_axis',(0.707106781186548,0.690078774854383,0.154244236506501));
#50686=DIRECTION('center_axis',(1.,0.,0.));
#50687=DIRECTION('ref_axis',(0.,0.,-1.));
#50688=DIRECTION('center_axis',(-2.38512309261853E-15,0.218134291185378,
-0.975918762504878));
#50689=DIRECTION('ref_axis',(0.,0.975918762504878,0.218134291185378));
#50690=DIRECTION('center_axis',(-1.,0.,0.));
#50691=DIRECTION('ref_axis',(0.,0.981569683813102,0.191104567760813));
#50692=DIRECTION('center_axis',(-0.939647353856857,0.247923894858407,0.235789297356865));
#50693=DIRECTION('ref_axis',(0.342144487592296,0.680884948347239,0.647559137627123));
#50694=DIRECTION('center_axis',(1.,0.,0.));
#50695=DIRECTION('ref_axis',(0.,0.,-1.));
#50696=DIRECTION('center_axis',(1.,0.,0.));
#50697=DIRECTION('ref_axis',(0.,0.946930129495106,0.321439465303162));
#50698=DIRECTION('center_axis',(0.70679631470526,-0.653568190182165,-0.270716808309112));
#50699=DIRECTION('ref_axis',(0.707106781186554,0.664042142409423,0.24299801049452));
#50700=DIRECTION('center_axis',(1.,0.,0.));
#50701=DIRECTION('ref_axis',(0.,0.,-1.));
#50702=DIRECTION('center_axis',(-3.15602894933998E-14,0.343651082071033,
-0.9390974037827));
#50703=DIRECTION('ref_axis',(0.,0.9390974037827,0.343651082071033));
#50704=DIRECTION('center_axis',(-1.,0.,0.));
#50705=DIRECTION('ref_axis',(0.,0.948228067551138,0.317590194918285));
#50706=DIRECTION('center_axis',(0.250366849761719,-0.8070109637463,0.534836185138648));
#50707=DIRECTION('ref_axis',(0.342144487592296,0.590536454753879,0.730892499083774));
#50708=DIRECTION('center_axis',(-1.,0.,0.));
#50709=DIRECTION('ref_axis',(0.,1.,0.));
#50710=DIRECTION('center_axis',(0.,-0.258819045102521,0.965925826289068));
#50711=DIRECTION('ref_axis',(0.707106781186523,0.683012701892242,0.183012701892228));
#50712=DIRECTION('',(0.,-0.258819045102521,0.965925826289068));
#50713=DIRECTION('center_axis',(0.,-0.965925826289068,-0.258819045102521));
#50714=DIRECTION('ref_axis',(1.,0.,0.));
#50715=DIRECTION('',(0.,0.258819045102521,-0.965925826289068));
#50716=DIRECTION('',(1.,0.,0.));
#50717=DIRECTION('center_axis',(-1.,0.,0.));
#50718=DIRECTION('ref_axis',(0.,1.,0.));
#50719=DIRECTION('center_axis',(0.,-0.130526192220052,0.99144486137381));
#50720=DIRECTION('ref_axis',(0.707106781186521,0.701057384650005,0.092295955641259));
#50721=DIRECTION('',(0.,-0.130526192220052,0.99144486137381));
#50722=DIRECTION('center_axis',(0.,-0.99144486137381,-0.130526192220052));
#50723=DIRECTION('ref_axis',(1.,0.,0.));
#50724=DIRECTION('',(0.,0.130526192220052,-0.99144486137381));
#50725=DIRECTION('',(1.,0.,0.));
#50726=DIRECTION('center_axis',(1.,0.,0.));
#50727=DIRECTION('ref_axis',(0.,0.,-1.));
#50728=DIRECTION('center_axis',(0.,-1.,-1.22464679914735E-16));
#50729=DIRECTION('ref_axis',(0.,-1.22464679914735E-16,1.));
#50730=DIRECTION('center_axis',(0.,0.,1.));
#50731=DIRECTION('ref_axis',(0.707106781186527,0.707106781186568,0.));
#50732=DIRECTION('center_axis',(0.,0.,-1.));
#50733=DIRECTION('ref_axis',(0.707106781186527,0.707106781186568,0.));
#50734=DIRECTION('',(0.,0.,1.));
#50735=DIRECTION('center_axis',(0.,-1.,0.));
#50736=DIRECTION('ref_axis',(1.,0.,0.));
#50737=DIRECTION('',(-1.,0.,0.));
#50738=DIRECTION('',(0.,0.,-1.));
#50739=DIRECTION('center_axis',(0.,0.,-1.));
#50740=DIRECTION('ref_axis',(-0.707106781186568,0.707106781186527,0.));
#50741=DIRECTION('center_axis',(0.,0.130526192220052,-0.99144486137381));
#50742=DIRECTION('ref_axis',(-0.707106781186562,0.701057384649963,0.0922959556412548));
#50743=DIRECTION('center_axis',(0.,-0.130526192220052,0.99144486137381));
#50744=DIRECTION('ref_axis',(-0.707106781186562,0.701057384649963,0.0922959556412548));
#50745=DIRECTION('center_axis',(0.,0.258819045102521,-0.965925826289068));
#50746=DIRECTION('ref_axis',(-0.707106781186555,0.683012701892213,0.183012701892214));
#50747=DIRECTION('center_axis',(0.,-0.258819045102521,0.965925826289068));
#50748=DIRECTION('ref_axis',(-0.707106781186555,0.683012701892213,0.183012701892214));
#50749=DIRECTION('center_axis',(1.,0.,0.));
#50750=DIRECTION('ref_axis',(0.,0.278995509497106,0.960292406343219));
#50751=DIRECTION('',(-1.,0.,0.));
#50752=DIRECTION('center_axis',(0.,-0.38268343236509,0.923879532511287));
#50753=DIRECTION('ref_axis',(0.707106781186518,0.653281482438215,0.270598050073112));
#50754=DIRECTION('',(0.,-0.38268343236509,0.923879532511287));
#50755=DIRECTION('center_axis',(0.,-0.923879532511287,-0.38268343236509));
#50756=DIRECTION('ref_axis',(1.,0.,0.));
#50757=DIRECTION('',(0.,0.38268343236509,-0.923879532511287));
#50758=DIRECTION('center_axis',(0.,0.38268343236509,-0.923879532511287));
#50759=DIRECTION('ref_axis',(-0.70710678118656,0.653281482438176,0.270598050073096));
#50760=DIRECTION('center_axis',(1.,0.,0.));
#50761=DIRECTION('ref_axis',(0.,0.,-1.));
#50762=DIRECTION('center_axis',(-1.,0.,0.));
#50763=DIRECTION('ref_axis',(0.,0.896872741532688,0.442288690219001));
#50764=DIRECTION('center_axis',(0.,0.5,-0.866025403784439));
#50765=DIRECTION('ref_axis',(-0.707106781186565,0.612372435695779,0.353553390593267));
#50766=DIRECTION('center_axis',(0.,0.608761429008721,-0.793353340291235));
#50767=DIRECTION('ref_axis',(-0.707106781186566,0.560985526796912,0.430459334576874));
#50768=DIRECTION('center_axis',(0.,0.707106781186548,-0.707106781186548));
#50769=DIRECTION('ref_axis',(-1.,0.,0.));
#50770=DIRECTION('',(-1.,0.,0.));
#50771=DIRECTION('center_axis',(0.,0.707106781186548,-0.707106781186548));
#50772=DIRECTION('ref_axis',(0.707106781186514,0.500000000000024,0.500000000000024));
#50773=DIRECTION('',(0.706902428155817,-0.500144457665688,-0.500144457665688));
#50774=DIRECTION('center_axis',(1.,0.,0.));
#50775=DIRECTION('ref_axis',(0.,-0.109729753246601,0.993961458635313));
#50776=DIRECTION('',(-1.,0.,0.));
#50777=DIRECTION('center_axis',(0.,-0.707106781186548,0.707106781186548));
#50778=DIRECTION('ref_axis',(0.707106781186514,0.500000000000024,0.500000000000024));
#50779=DIRECTION('',(0.,-0.707106781186548,0.707106781186548));
#50780=DIRECTION('center_axis',(0.,-0.707106781186548,-0.707106781186548));
#50781=DIRECTION('ref_axis',(1.,0.,0.));
#50782=DIRECTION('',(0.,0.707106781186548,-0.707106781186548));
#50783=DIRECTION('center_axis',(0.,0.707106781186548,-0.707106781186548));
#50784=DIRECTION('ref_axis',(-0.707106781186567,0.499999999999981,0.499999999999992));
#50785=DIRECTION('center_axis',(1.,0.,0.));
#50786=DIRECTION('ref_axis',(0.,0.,-1.));
#50787=DIRECTION('center_axis',(-1.,0.,0.));
#50788=DIRECTION('ref_axis',(0.,0.659345815100069,0.751839807478978));
#50789=DIRECTION('center_axis',(0.,0.793353340291235,-0.608761429008721));
#50790=DIRECTION('ref_axis',(-0.707106781186558,0.430459334576869,0.560985526796926));
#50791=DIRECTION('center_axis',(0.,0.866025403784439,-0.5));
#50792=DIRECTION('ref_axis',(-0.707106781186561,0.35355339059328,0.612372435695775));
#50793=DIRECTION('center_axis',(1.,0.,0.));
#50794=DIRECTION('ref_axis',(0.,-0.481749655761243,0.876308889133235));
#50795=DIRECTION('',(-1.,0.,0.));
#50796=DIRECTION('center_axis',(0.,-0.923879532511287,0.38268343236509));
#50797=DIRECTION('ref_axis',(0.707106781186519,0.270598050073107,0.653281482438216));
#50798=DIRECTION('',(0.,-0.923879532511287,0.38268343236509));
#50799=DIRECTION('center_axis',(0.,-0.38268343236509,-0.923879532511287));
#50800=DIRECTION('ref_axis',(1.,0.,0.));
#50801=DIRECTION('',(0.,0.923879532511287,-0.38268343236509));
#50802=DIRECTION('center_axis',(0.,0.923879532511287,-0.38268343236509));
#50803=DIRECTION('ref_axis',(-0.707106781186561,0.270598050073091,0.653281482438177));
#50804=DIRECTION('center_axis',(1.,0.,0.));
#50805=DIRECTION('ref_axis',(0.,0.,-1.));
#50806=DIRECTION('center_axis',(-1.,0.,0.));
#50807=DIRECTION('ref_axis',(0.,0.321439465303162,0.946930129495105));
#50808=DIRECTION('center_axis',(0.,0.965925826289068,-0.258819045102521));
#50809=DIRECTION('ref_axis',(-0.707106781186554,0.183012701892219,0.683012701892212));
#50810=DIRECTION('',(0.,0.965925826289068,-0.258819045102521));
#50811=DIRECTION('center_axis',(0.,-0.258819045102521,-0.965925826289068));
#50812=DIRECTION('ref_axis',(1.,0.,0.));
#50813=DIRECTION('center_axis',(0.,0.99144486137381,-0.130526192220052));
#50814=DIRECTION('ref_axis',(-0.707106781186563,0.0922959556412483,0.701057384649964));
#50815=DIRECTION('center_axis',(1.,0.,0.));
#50816=DIRECTION('ref_axis',(0.,-0.780427540257712,0.625246235020489));
#50817=DIRECTION('center_axis',(0.,-1.,6.12323399573677E-17));
#50818=DIRECTION('ref_axis',(0.707106781186527,0.,0.707106781186568));
#50819=DIRECTION('',(0.,-1.,6.12323399573677E-17));
#50820=DIRECTION('center_axis',(0.,-6.12323399573677E-17,-1.));
#50821=DIRECTION('ref_axis',(1.,0.,0.));
#50822=DIRECTION('',(0.,1.,-6.12323399573677E-17));
#50823=DIRECTION('center_axis',(0.,1.,-6.12323399573677E-17));
#50824=DIRECTION('ref_axis',(-0.707106781186568,0.,0.707106781186527));
#50825=DIRECTION('center_axis',(1.,0.,0.));
#50826=DIRECTION('ref_axis',(0.,0.,-1.));
#50827=DIRECTION('center_axis',(-1.,0.,0.));
#50828=DIRECTION('ref_axis',(0.,-0.0654031292301429,0.997858923238603));
#50829=DIRECTION('center_axis',(0.,0.99144486137381,0.130526192220051));
#50830=DIRECTION('ref_axis',(-0.707106781186552,-0.0922959556412574,0.701057384649974));
#50831=DIRECTION('center_axis',(0.,0.965925826289068,0.258819045102521));
#50832=DIRECTION('ref_axis',(-0.707106781186565,-0.183012701892217,0.683012701892202));
#50833=DIRECTION('center_axis',(1.,0.,0.));
#50834=DIRECTION('ref_axis',(0.,-0.960292406343215,0.27899550949712));
#50835=DIRECTION('',(-1.,0.,0.));
#50836=DIRECTION('center_axis',(0.,-0.923879532511287,-0.38268343236509));
#50837=DIRECTION('ref_axis',(0.707106781186518,-0.270598050073113,0.653281482438214));
#50838=DIRECTION('',(0.,-0.923879532511287,-0.38268343236509));
#50839=DIRECTION('center_axis',(0.,0.38268343236509,-0.923879532511287));
#50840=DIRECTION('ref_axis',(1.,0.,0.));
#50841=DIRECTION('',(0.,0.923879532511287,0.38268343236509));
#50842=DIRECTION('center_axis',(0.,0.923879532511287,0.38268343236509));
#50843=DIRECTION('ref_axis',(-0.70710678118656,-0.270598050073094,0.653281482438177));
#50844=DIRECTION('center_axis',(1.,0.,0.));
#50845=DIRECTION('ref_axis',(0.,0.,-1.));
#50846=DIRECTION('center_axis',(-1.,0.,0.));
#50847=DIRECTION('ref_axis',(0.,-0.442288690219001,0.896872741532688));
#50848=DIRECTION('center_axis',(0.,0.866025403784439,0.5));
#50849=DIRECTION('ref_axis',(-0.707106781186554,-0.353553390593267,0.612372435695791));
#50850=DIRECTION('center_axis',(0.,0.793353340291235,0.60876142900872));
#50851=DIRECTION('ref_axis',(-0.707106781186558,-0.430459334576869,0.560985526796926));
#50852=DIRECTION('center_axis',(1.,0.,0.));
#50853=DIRECTION('ref_axis',(0.,-0.993961458635316,-0.109729753246582));
#50854=DIRECTION('',(-1.,0.,0.));
#50855=DIRECTION('center_axis',(0.,-0.707106781186548,-0.707106781186547));
#50856=DIRECTION('ref_axis',(0.707106781186517,-0.500000000000016,0.500000000000026));
#50857=DIRECTION('',(0.,-0.707106781186548,-0.707106781186547));
#50858=DIRECTION('center_axis',(0.,0.707106781186547,-0.707106781186548));
#50859=DIRECTION('ref_axis',(1.,0.,0.));
#50860=DIRECTION('',(0.,0.707106781186548,0.707106781186547));
#50861=DIRECTION('center_axis',(0.,0.707106781186548,0.707106781186547));
#50862=DIRECTION('ref_axis',(-0.707106781186559,-0.499999999999986,0.499999999999997));
#50863=DIRECTION('center_axis',(1.,0.,0.));
#50864=DIRECTION('ref_axis',(0.,0.,-1.));
#50865=DIRECTION('center_axis',(-1.,0.,0.));
#50866=DIRECTION('ref_axis',(0.,-0.751839807478977,0.659345815100069));
#50867=DIRECTION('center_axis',(0.,0.608761429008721,0.793353340291235));
#50868=DIRECTION('ref_axis',(-0.707106781186551,-0.560985526796921,0.430459334576886));
#50869=DIRECTION('center_axis',(0.,0.5,0.866025403784438));
#50870=DIRECTION('ref_axis',(-0.707106781186552,-0.612372435695789,0.353553390593276));
#50871=DIRECTION('center_axis',(1.,0.,0.));
#50872=DIRECTION('ref_axis',(0.,-0.87630888913323,-0.481749655761251));
#50873=DIRECTION('',(-1.,0.,0.));
#50874=DIRECTION('center_axis',(0.,-0.38268343236509,-0.923879532511287));
#50875=DIRECTION('ref_axis',(0.707106781186519,-0.653281482438215,0.270598050073107));
#50876=DIRECTION('',(0.,-0.38268343236509,-0.923879532511287));
#50877=DIRECTION('center_axis',(0.,0.923879532511287,-0.38268343236509));
#50878=DIRECTION('ref_axis',(1.,0.,0.));
#50879=DIRECTION('',(0.,0.38268343236509,0.923879532511287));
#50880=DIRECTION('center_axis',(0.,0.38268343236509,0.923879532511287));
#50881=DIRECTION('ref_axis',(-0.707106781186561,-0.653281482438177,0.270598050073091));
#50882=DIRECTION('center_axis',(1.,0.,0.));
#50883=DIRECTION('ref_axis',(0.,0.,-1.));
#50884=DIRECTION('center_axis',(-1.,0.,0.));
#50885=DIRECTION('ref_axis',(0.,-0.946930129495105,0.321439465303162));
#50886=DIRECTION('center_axis',(0.,0.258819045102521,0.965925826289068));
#50887=DIRECTION('ref_axis',(-0.707106781186564,-0.683012701892201,0.183012701892222));
#50888=DIRECTION('center_axis',(0.,0.130526192220052,0.99144486137381));
#50889=DIRECTION('ref_axis',(-1.,0.,0.));
#50890=DIRECTION('',(0.706902428155816,0.701259930876578,-0.0923226213578653));
#50891=DIRECTION('center_axis',(0.,0.130526192220052,0.99144486137381));
#50892=DIRECTION('ref_axis',(-0.707106781186562,-0.701057384649963,0.0922959556412587));
#50893=DIRECTION('center_axis',(1.,0.,0.));
#50894=DIRECTION('ref_axis',(0.,-0.625246235020489,-0.780427540257712));
#50895=DIRECTION('center_axis',(0.,-1.22464679914735E-16,-1.));
#50896=DIRECTION('ref_axis',(0.707106781186527,-0.707106781186568,8.65956056235553E-17));
#50897=DIRECTION('',(0.,-1.22464679914735E-16,-1.));
#50898=DIRECTION('center_axis',(0.,1.,-1.22464679914735E-16));
#50899=DIRECTION('ref_axis',(1.,0.,0.));
#50900=DIRECTION('',(0.,1.22464679914735E-16,1.));
#50901=DIRECTION('center_axis',(0.,1.22464679914735E-16,1.));
#50902=DIRECTION('ref_axis',(-0.707106781186568,-0.707106781186527,8.65956056235502E-17));
#50903=DIRECTION('center_axis',(1.,0.,0.));
#50904=DIRECTION('ref_axis',(0.,0.,-1.));
#50905=DIRECTION('center_axis',(-1.,0.,0.));
#50906=DIRECTION('ref_axis',(0.,-0.997858923238603,-0.0654031292301432));
#50907=DIRECTION('center_axis',(0.,-0.130526192220051,0.99144486137381));
#50908=DIRECTION('ref_axis',(-0.707106781186573,-0.701057384649953,-0.0922959556412549));
#50909=DIRECTION('center_axis',(0.,-0.25881904510252,0.965925826289068));
#50910=DIRECTION('ref_axis',(-0.707106781186564,-0.683012701892201,-0.183012701892222));
#50911=DIRECTION('center_axis',(1.,0.,0.));
#50912=DIRECTION('ref_axis',(0.,-0.278995509497142,-0.960292406343209));
#50913=DIRECTION('',(-1.,0.,0.));
#50914=DIRECTION('center_axis',(0.,0.382683432365089,-0.923879532511287));
#50915=DIRECTION('ref_axis',(0.707106781186519,-0.653281482438215,-0.270598050073107));
#50916=DIRECTION('',(0.,0.382683432365089,-0.923879532511287));
#50917=DIRECTION('center_axis',(0.,0.923879532511287,0.382683432365089));
#50918=DIRECTION('ref_axis',(1.,0.,0.));
#50919=DIRECTION('',(0.,-0.382683432365089,0.923879532511287));
#50920=DIRECTION('center_axis',(0.,-0.382683432365089,0.923879532511287));
#50921=DIRECTION('ref_axis',(-0.707106781186561,-0.653281482438177,-0.270598050073091));
#50922=DIRECTION('center_axis',(1.,0.,0.));
#50923=DIRECTION('ref_axis',(0.,0.,-1.));
#50924=DIRECTION('center_axis',(-1.,0.,0.));
#50925=DIRECTION('ref_axis',(0.,-0.896872741532689,-0.442288690219));
#50926=DIRECTION('center_axis',(0.,-0.5,0.866025403784439));
#50927=DIRECTION('ref_axis',(-0.707106781186566,-0.61237243569578,-0.353553390593262));
#50928=DIRECTION('center_axis',(0.,-0.60876142900872,0.793353340291235));
#50929=DIRECTION('ref_axis',(-0.707106781186558,-0.560985526796926,-0.430459334576869));
#50930=DIRECTION('center_axis',(0.,-0.707106781186547,0.707106781186548));
#50931=DIRECTION('ref_axis',(-1.,0.,0.));
#50932=DIRECTION('',(-1.,0.,0.));
#50933=DIRECTION('center_axis',(0.,-0.707106781186547,0.707106781186548));
#50934=DIRECTION('ref_axis',(0.707106781186517,-0.500000000000016,-0.500000000000026));
#50935=DIRECTION('',(0.706902428155819,0.500144457665689,0.500144457665683));
#50936=DIRECTION('center_axis',(1.,0.,0.));
#50937=DIRECTION('ref_axis',(0.,0.109729753246624,-0.993961458635311));
#50938=DIRECTION('',(-1.,0.,0.));
#50939=DIRECTION('center_axis',(0.,0.707106781186547,-0.707106781186548));
#50940=DIRECTION('ref_axis',(0.707106781186517,-0.500000000000016,-0.500000000000026));
#50941=DIRECTION('',(0.,0.707106781186547,-0.707106781186548));
#50942=DIRECTION('center_axis',(0.,0.707106781186548,0.707106781186547));
#50943=DIRECTION('ref_axis',(1.,0.,0.));
#50944=DIRECTION('',(0.,-0.707106781186547,0.707106781186548));
#50945=DIRECTION('center_axis',(0.,-0.707106781186547,0.707106781186548));
#50946=DIRECTION('ref_axis',(-0.707106781186559,-0.499999999999986,-0.499999999999997));
#50947=DIRECTION('center_axis',(1.,0.,0.));
#50948=DIRECTION('ref_axis',(0.,0.,-1.));
#50949=DIRECTION('center_axis',(-1.,0.,0.));
#50950=DIRECTION('ref_axis',(0.,-0.65934581510007,-0.751839807478977));
#50951=DIRECTION('center_axis',(0.,-0.793353340291235,0.608761429008721));
#50952=DIRECTION('ref_axis',(-0.707106781186558,-0.430459334576869,-0.560985526796926));
#50953=DIRECTION('center_axis',(0.,-0.866025403784438,0.5));
#50954=DIRECTION('ref_axis',(-1.,0.,0.));
#50955=DIRECTION('',(0.706902428155815,0.353655537588269,0.612549359480985));
#50956=DIRECTION('center_axis',(0.,-0.866025403784438,0.5));
#50957=DIRECTION('ref_axis',(-0.707106781186554,-0.353553390593267,-0.612372435695791));
#50958=DIRECTION('center_axis',(1.,0.,0.));
#50959=DIRECTION('ref_axis',(0.,0.481749655761234,-0.876308889133239));
#50960=DIRECTION('',(-1.,0.,0.));
#50961=DIRECTION('center_axis',(0.,0.923879532511287,-0.38268343236509));
#50962=DIRECTION('ref_axis',(0.707106781186517,-0.270598050073114,-0.653281482438214));
#50963=DIRECTION('',(0.,0.923879532511286,-0.38268343236509));
#50964=DIRECTION('center_axis',(0.,0.38268343236509,0.923879532511287));
#50965=DIRECTION('ref_axis',(1.,0.,0.));
#50966=DIRECTION('',(0.,-0.923879532511286,0.38268343236509));
#50967=DIRECTION('center_axis',(0.,-0.923879532511287,0.38268343236509));
#50968=DIRECTION('ref_axis',(-0.70710678118656,-0.270598050073094,-0.653281482438177));
#50969=DIRECTION('center_axis',(1.,0.,0.));
#50970=DIRECTION('ref_axis',(0.,0.,-1.));
#50971=DIRECTION('center_axis',(-1.,0.,0.));
#50972=DIRECTION('ref_axis',(0.,-0.321439465303162,-0.946930129495105));
#50973=DIRECTION('center_axis',(0.,-0.965925826289068,0.258819045102522));
#50974=DIRECTION('ref_axis',(-0.707106781186555,-0.183012701892214,-0.683012701892213));
#50975=DIRECTION('center_axis',(0.,-0.99144486137381,0.130526192220052));
#50976=DIRECTION('ref_axis',(-0.707106781186563,-0.0922959556412483,-0.701057384649964));
#50977=DIRECTION('center_axis',(1.,0.,0.));
#50978=DIRECTION('ref_axis',(0.,0.780427540257703,-0.625246235020501));
#50979=DIRECTION('center_axis',(0.,1.,-1.83697019872103E-16));
#50980=DIRECTION('ref_axis',(0.707106781186516,0.,-0.707106781186579));
#50981=DIRECTION('',(0.,1.,-1.83697019872103E-16));
#50982=DIRECTION('center_axis',(0.,1.83697019872103E-16,1.));
#50983=DIRECTION('ref_axis',(1.,0.,0.));
#50984=DIRECTION('',(0.,-1.,1.83697019872103E-16));
#50985=DIRECTION('center_axis',(0.,-1.,1.83697019872103E-16));
#50986=DIRECTION('ref_axis',(-0.707106781186558,0.,-0.707106781186537));
#50987=DIRECTION('center_axis',(1.,0.,0.));
#50988=DIRECTION('ref_axis',(0.,0.,-1.));
#50989=DIRECTION('center_axis',(-1.,0.,0.));
#50990=DIRECTION('ref_axis',(0.,0.0654031292301432,-0.997858923238603));
#50991=DIRECTION('center_axis',(0.,-0.99144486137381,-0.130526192220051));
#50992=DIRECTION('ref_axis',(-0.707106781186563,0.0922959556412483,-0.701057384649964));
#50993=DIRECTION('center_axis',(0.,-0.965925826289068,-0.25881904510252));
#50994=DIRECTION('ref_axis',(-0.707106781186567,0.183012701892202,-0.683012701892204));
#50995=DIRECTION('center_axis',(1.,0.,0.));
#50996=DIRECTION('ref_axis',(0.,0.960292406343209,-0.278995509497142));
#50997=DIRECTION('',(-1.,0.,0.));
#50998=DIRECTION('center_axis',(0.,0.923879532511287,0.382683432365089));
#50999=DIRECTION('ref_axis',(0.707106781186519,0.270598050073107,-0.653281482438216));
#51000=DIRECTION('',(0.,0.923879532511287,0.382683432365089));
#51001=DIRECTION('center_axis',(0.,-0.382683432365089,0.923879532511287));
#51002=DIRECTION('ref_axis',(1.,0.,0.));
#51003=DIRECTION('',(0.,-0.923879532511287,-0.382683432365089));
#51004=DIRECTION('center_axis',(0.,-0.923879532511287,-0.382683432365089));
#51005=DIRECTION('ref_axis',(-0.707106781186561,0.270598050073091,-0.653281482438177));
#51006=DIRECTION('center_axis',(1.,0.,0.));
#51007=DIRECTION('ref_axis',(0.,0.,-1.));
#51008=DIRECTION('center_axis',(-1.,0.,0.));
#51009=DIRECTION('ref_axis',(0.,0.442288690219,-0.896872741532689));
#51010=DIRECTION('center_axis',(0.,-0.866025403784439,-0.499999999999999));
#51011=DIRECTION('ref_axis',(-0.707106781186557,0.353553390593258,-0.612372435695793));
#51012=DIRECTION('center_axis',(0.,-0.793353340291236,-0.60876142900872));
#51013=DIRECTION('ref_axis',(-0.707106781186562,0.430459334576871,-0.560985526796919));
#51014=DIRECTION('center_axis',(0.,-0.707106781186548,-0.707106781186547));
#51015=DIRECTION('ref_axis',(-1.,0.,0.));
#51016=DIRECTION('',(-1.,0.,0.));
#51017=DIRECTION('center_axis',(0.,-0.707106781186548,-0.707106781186547));
#51018=DIRECTION('ref_axis',(0.707106781186525,0.500000000000011,-0.500000000000021));
#51019=DIRECTION('',(0.706902428155819,-0.500144457665683,0.500144457665689));
#51020=DIRECTION('center_axis',(1.,0.,0.));
#51021=DIRECTION('ref_axis',(0.,0.993961458635311,0.109729753246624));
#51022=DIRECTION('',(-1.,0.,0.));
#51023=DIRECTION('center_axis',(0.,0.707106781186548,0.707106781186547));
#51024=DIRECTION('ref_axis',(0.707106781186525,0.500000000000011,-0.500000000000021));
#51025=DIRECTION('',(0.,0.707106781186548,0.707106781186547));
#51026=DIRECTION('center_axis',(0.,-0.707106781186547,0.707106781186548));
#51027=DIRECTION('ref_axis',(1.,0.,0.));
#51028=DIRECTION('',(0.,-0.707106781186548,-0.707106781186547));
#51029=DIRECTION('center_axis',(0.,-0.707106781186548,-0.707106781186547));
#51030=DIRECTION('ref_axis',(-0.707106781186567,0.499999999999981,-0.499999999999992));
#51031=DIRECTION('center_axis',(1.,0.,0.));
#51032=DIRECTION('ref_axis',(0.,0.,-1.));
#51033=DIRECTION('center_axis',(-1.,0.,0.));
#51034=DIRECTION('ref_axis',(0.,0.751839807478977,-0.659345815100069));
#51035=DIRECTION('center_axis',(0.,-0.608761429008721,-0.793353340291235));
#51036=DIRECTION('ref_axis',(-0.707106781186558,0.560985526796926,-0.430459334576869));
#51037=DIRECTION('center_axis',(0.,-0.5,-0.866025403784438));
#51038=DIRECTION('ref_axis',(-0.707106781186556,0.612372435695792,-0.353553390593262));
#51039=DIRECTION('center_axis',(1.,0.,0.));
#51040=DIRECTION('ref_axis',(0.,0.87630888913324,0.481749655761234));
#51041=DIRECTION('',(-1.,0.,0.));
#51042=DIRECTION('center_axis',(0.,0.38268343236509,0.923879532511287));
#51043=DIRECTION('ref_axis',(0.707106781186519,0.653281482438215,-0.270598050073107));
#51044=DIRECTION('',(0.,0.38268343236509,0.923879532511286));
#51045=DIRECTION('center_axis',(0.,-0.923879532511287,0.38268343236509));
#51046=DIRECTION('ref_axis',(1.,0.,0.));
#51047=DIRECTION('',(0.,-0.38268343236509,-0.923879532511286));
#51048=DIRECTION('center_axis',(0.,-0.38268343236509,-0.923879532511287));
#51049=DIRECTION('ref_axis',(-0.70710678118656,0.653281482438176,-0.270598050073096));
#51050=DIRECTION('center_axis',(1.,0.,0.));
#51051=DIRECTION('ref_axis',(0.,0.,-1.));
#51052=DIRECTION('center_axis',(-1.,0.,0.));
#51053=DIRECTION('ref_axis',(0.,0.946930129495105,-0.321439465303162));
#51054=DIRECTION('center_axis',(0.,-0.258819045102522,-0.965925826289068));
#51055=DIRECTION('ref_axis',(-0.707106781186565,0.683012701892202,-0.183012701892217));
#51056=DIRECTION('center_axis',(1.,0.,0.));
#51057=DIRECTION('ref_axis',(0.,0.,-1.));
#51058=DIRECTION('center_axis',(0.,-0.130526192220053,-0.99144486137381));
#51059=DIRECTION('ref_axis',(-1.,0.,0.));
#51060=DIRECTION('',(0.706902428155816,-0.701259930876578,0.0923226213578653));
#51061=DIRECTION('',(1.,0.,0.));
#51062=DIRECTION('center_axis',(0.,-0.130526192220053,-0.99144486137381));
#51063=DIRECTION('ref_axis',(-0.707106781186562,0.701057384649963,-0.0922959556412561));
#51064=DIRECTION('',(-1.,0.,0.));
#51065=DIRECTION('center_axis',(0.,-0.130526192220053,-0.99144486137381));
#51066=DIRECTION('ref_axis',(0.70710678118652,0.701057384650004,-0.0922959556412616));
#51067=DIRECTION('center_axis',(0.,0.130526192220053,0.99144486137381));
#51068=DIRECTION('ref_axis',(0.70710678118652,0.701057384650004,-0.0922959556412616));
#51069=DIRECTION('',(0.,0.130526192220053,0.99144486137381));
#51070=DIRECTION('center_axis',(0.,-0.99144486137381,0.130526192220053));
#51071=DIRECTION('ref_axis',(1.,0.,0.));
#51072=DIRECTION('',(0.,-0.130526192220053,-0.99144486137381));
#51073=DIRECTION('center_axis',(0.,-0.130526192220053,-0.99144486137381));
#51074=DIRECTION('ref_axis',(-0.707106781186562,0.701057384649963,-0.0922959556412561));
#51075=DIRECTION('center_axis',(1.,0.,0.));
#51076=DIRECTION('ref_axis',(0.,0.805930996937515,0.592009483180214));
#51077=DIRECTION('',(-1.,0.,0.));
#51078=DIRECTION('center_axis',(-1.,0.,0.));
#51079=DIRECTION('ref_axis',(0.,1.,0.));
#51080=DIRECTION('center_axis',(1.,0.,0.));
#51081=DIRECTION('ref_axis',(0.,0.,-1.));
#51082=DIRECTION('center_axis',(1.,0.,0.));
#51083=DIRECTION('ref_axis',(0.,1.,0.));
#51084=DIRECTION('center_axis',(1.,0.,0.));
#51085=DIRECTION('ref_axis',(0.,1.,0.));
#51086=DIRECTION('center_axis',(1.,0.,0.));
#51087=DIRECTION('ref_axis',(0.,0.,-1.));
#51088=DIRECTION('center_axis',(1.,0.,0.));
#51089=DIRECTION('ref_axis',(0.,1.,0.));
#51090=DIRECTION('center_axis',(-1.,0.,0.));
#51091=DIRECTION('ref_axis',(0.,1.,0.));
#51092=DIRECTION('center_axis',(-1.,0.,0.));
#51093=DIRECTION('ref_axis',(0.,1.,0.));
#51094=DIRECTION('center_axis',(1.,0.,0.));
#51095=DIRECTION('ref_axis',(0.,1.,0.));
#51096=DIRECTION('center_axis',(1.,0.,0.));
#51097=DIRECTION('ref_axis',(0.,0.,-1.));
#51098=DIRECTION('center_axis',(1.,0.,0.));
#51099=DIRECTION('ref_axis',(0.,1.,0.));
#51100=DIRECTION('center_axis',(-1.,0.,0.));
#51101=DIRECTION('ref_axis',(0.,1.,0.));
#51102=DIRECTION('center_axis',(-1.,0.,0.));
#51103=DIRECTION('ref_axis',(0.,1.,0.));
#51104=DIRECTION('center_axis',(1.,0.,0.));
#51105=DIRECTION('ref_axis',(0.,1.,0.));
#51106=DIRECTION('center_axis',(1.,0.,0.));
#51107=DIRECTION('ref_axis',(0.,0.,-1.));
#51108=DIRECTION('center_axis',(1.,0.,0.));
#51109=DIRECTION('ref_axis',(0.,1.,0.));
#51110=DIRECTION('center_axis',(-1.,0.,0.));
#51111=DIRECTION('ref_axis',(0.,1.,0.));
#51112=DIRECTION('center_axis',(-1.,0.,0.));
#51113=DIRECTION('ref_axis',(0.,1.,0.));
#51114=DIRECTION('center_axis',(1.,0.,0.));
#51115=DIRECTION('ref_axis',(0.,1.,0.));
#51116=DIRECTION('center_axis',(-1.,0.,0.));
#51117=DIRECTION('ref_axis',(0.,1.,0.));
#51118=DIRECTION('center_axis',(-1.,0.,0.));
#51119=DIRECTION('ref_axis',(0.,1.,0.));
#51120=DIRECTION('center_axis',(1.,0.,0.));
#51121=DIRECTION('ref_axis',(0.,1.,0.));
#51122=DIRECTION('center_axis',(1.,0.,0.));
#51123=DIRECTION('ref_axis',(0.,0.,-1.));
#51124=DIRECTION('center_axis',(1.,0.,0.));
#51125=DIRECTION('ref_axis',(0.,1.,0.));
#51126=DIRECTION('center_axis',(-1.,0.,0.));
#51127=DIRECTION('ref_axis',(0.,1.,0.));
#51128=DIRECTION('center_axis',(-1.,0.,0.));
#51129=DIRECTION('ref_axis',(0.,1.,0.));
#51130=DIRECTION('center_axis',(1.,0.,0.));
#51131=DIRECTION('ref_axis',(0.,1.,0.));
#51132=DIRECTION('center_axis',(1.,0.,0.));
#51133=DIRECTION('ref_axis',(0.,0.,-1.));
#51134=DIRECTION('center_axis',(1.,0.,0.));
#51135=DIRECTION('ref_axis',(0.,1.,0.));
#51136=DIRECTION('center_axis',(-1.,0.,0.));
#51137=DIRECTION('ref_axis',(0.,1.,0.));
#51138=DIRECTION('center_axis',(-1.,0.,0.));
#51139=DIRECTION('ref_axis',(0.,1.,0.));
#51140=DIRECTION('center_axis',(1.,0.,0.));
#51141=DIRECTION('ref_axis',(0.,1.,0.));
#51142=DIRECTION('center_axis',(1.,0.,0.));
#51143=DIRECTION('ref_axis',(0.,0.,-1.));
#51144=DIRECTION('center_axis',(1.,0.,0.));
#51145=DIRECTION('ref_axis',(0.,1.,0.));
#51146=DIRECTION('center_axis',(-1.,0.,0.));
#51147=DIRECTION('ref_axis',(0.,1.,0.));
#51148=DIRECTION('center_axis',(-1.,0.,0.));
#51149=DIRECTION('ref_axis',(0.,1.,0.));
#51150=DIRECTION('center_axis',(1.,0.,0.));
#51151=DIRECTION('ref_axis',(0.,1.,0.));
#51152=DIRECTION('center_axis',(-1.,0.,0.));
#51153=DIRECTION('ref_axis',(0.,1.,0.));
#51154=DIRECTION('center_axis',(-1.,0.,0.));
#51155=DIRECTION('ref_axis',(0.,1.,0.));
#51156=DIRECTION('center_axis',(1.,0.,0.));
#51157=DIRECTION('ref_axis',(0.,1.,0.));
#51158=DIRECTION('center_axis',(1.,0.,0.));
#51159=DIRECTION('ref_axis',(0.,0.,-1.));
#51160=DIRECTION('center_axis',(1.,0.,0.));
#51161=DIRECTION('ref_axis',(0.,1.,0.));
#51162=DIRECTION('center_axis',(-1.,0.,0.));
#51163=DIRECTION('ref_axis',(0.,1.,0.));
#51164=DIRECTION('center_axis',(-1.,0.,0.));
#51165=DIRECTION('ref_axis',(0.,1.,0.));
#51166=DIRECTION('center_axis',(1.,0.,0.));
#51167=DIRECTION('ref_axis',(0.,1.,0.));
#51168=DIRECTION('center_axis',(1.,0.,0.));
#51169=DIRECTION('ref_axis',(0.,0.,-1.));
#51170=DIRECTION('center_axis',(1.,0.,0.));
#51171=DIRECTION('ref_axis',(0.,1.,0.));
#51172=DIRECTION('center_axis',(-1.,0.,0.));
#51173=DIRECTION('ref_axis',(0.,1.,0.));
#51174=DIRECTION('center_axis',(-1.,0.,0.));
#51175=DIRECTION('ref_axis',(0.,1.,0.));
#51176=DIRECTION('center_axis',(1.,0.,0.));
#51177=DIRECTION('ref_axis',(0.,1.,0.));
#51178=DIRECTION('center_axis',(1.,0.,0.));
#51179=DIRECTION('ref_axis',(0.,0.,-1.));
#51180=DIRECTION('center_axis',(1.,0.,0.));
#51181=DIRECTION('ref_axis',(0.,1.,0.));
#51182=DIRECTION('center_axis',(-1.,0.,0.));
#51183=DIRECTION('ref_axis',(0.,1.,0.));
#51184=DIRECTION('center_axis',(-1.,0.,0.));
#51185=DIRECTION('ref_axis',(0.,1.,0.));
#51186=DIRECTION('center_axis',(1.,0.,0.));
#51187=DIRECTION('ref_axis',(0.,1.,0.));
#51188=DIRECTION('center_axis',(-1.,0.,0.));
#51189=DIRECTION('ref_axis',(0.,1.,0.));
#51190=DIRECTION('center_axis',(-1.,0.,0.));
#51191=DIRECTION('ref_axis',(0.,1.,0.));
#51192=DIRECTION('center_axis',(1.,0.,0.));
#51193=DIRECTION('ref_axis',(0.,1.,0.));
#51194=DIRECTION('center_axis',(1.,0.,0.));
#51195=DIRECTION('ref_axis',(0.,0.,-1.));
#51196=DIRECTION('center_axis',(1.,0.,0.));
#51197=DIRECTION('ref_axis',(0.,1.,0.));
#51198=DIRECTION('center_axis',(-1.,0.,0.));
#51199=DIRECTION('ref_axis',(0.,1.,0.));
#51200=DIRECTION('center_axis',(-1.,0.,0.));
#51201=DIRECTION('ref_axis',(0.,1.,0.));
#51202=DIRECTION('center_axis',(1.,0.,0.));
#51203=DIRECTION('ref_axis',(0.,1.,0.));
#51204=DIRECTION('center_axis',(1.,0.,0.));
#51205=DIRECTION('ref_axis',(0.,0.,-1.));
#51206=DIRECTION('center_axis',(1.,0.,0.));
#51207=DIRECTION('ref_axis',(0.,1.,0.));
#51208=DIRECTION('center_axis',(-1.,0.,0.));
#51209=DIRECTION('ref_axis',(0.,1.,0.));
#51210=DIRECTION('center_axis',(-1.,0.,0.));
#51211=DIRECTION('ref_axis',(0.,1.,0.));
#51212=DIRECTION('center_axis',(1.,0.,0.));
#51213=DIRECTION('ref_axis',(0.,1.,0.));
#51214=DIRECTION('center_axis',(1.,0.,0.));
#51215=DIRECTION('ref_axis',(0.,0.,-1.));
#51216=DIRECTION('center_axis',(1.,0.,0.));
#51217=DIRECTION('ref_axis',(0.,1.,0.));
#51218=DIRECTION('center_axis',(0.,-0.258819045102521,0.965925826289068));
#51219=DIRECTION('ref_axis',(1.,0.,0.));
#51220=DIRECTION('center_axis',(0.,-0.130526192220052,0.99144486137381));
#51221=DIRECTION('ref_axis',(1.,0.,0.));
#51222=DIRECTION('center_axis',(-1.,0.,0.));
#51223=DIRECTION('ref_axis',(0.,1.,0.));
#51224=DIRECTION('',(0.706902428155817,-0.707311075176552,3.92409675951017E-16));
#51225=DIRECTION('center_axis',(0.,0.,-1.));
#51226=DIRECTION('ref_axis',(-1.,0.,0.));
#68016=CARTESIAN_POINT('',(0.,0.,0.));
#68017=CARTESIAN_POINT('Origin',(121.7,-1.6,18.875));
#68018=CARTESIAN_POINT('',(121.7,-1.3,37.841926118218));
#68019=CARTESIAN_POINT('',(122.,-1.6,37.841926118218));
#68020=CARTESIAN_POINT('Origin',(121.7,-1.6,37.841926118218));
#68021=CARTESIAN_POINT('',(122.,-1.6,36.2));
#68022=CARTESIAN_POINT('',(122.,-1.6,18.875));
#68023=CARTESIAN_POINT('',(121.7,-1.3,36.5));
#68024=CARTESIAN_POINT('Origin',(121.7,-1.6,36.2));
#68025=CARTESIAN_POINT('',(121.7,-1.3,18.875));
#68026=CARTESIAN_POINT('Ctrl Pts',(121.699999999994,-1.3,37.8419261182243));
#68027=CARTESIAN_POINT('Ctrl Pts',(121.591912387508,-1.3,37.950110301428));
#68028=CARTESIAN_POINT('Ctrl Pts',(121.483824361116,-1.3,38.0582940710949));
#68029=CARTESIAN_POINT('Ctrl Pts',(121.375735931282,-1.3,38.1664774376736));
#68030=CARTESIAN_POINT('Ctrl Pts',(121.756617543134,-1.3,37.8984931216591));
#68031=CARTESIAN_POINT('Ctrl Pts',(121.648526737394,-1.30000014726686,38.0066744036192));
#68032=CARTESIAN_POINT('Ctrl Pts',(121.540435642302,-1.29999985529285,38.1148553910149));
#68033=CARTESIAN_POINT('Ctrl Pts',(121.432344074471,-1.3,38.223035904161));
#68034=CARTESIAN_POINT('Ctrl Pts',(121.869289488093,-1.36773987413571,38.0110644898949));
#68035=CARTESIAN_POINT('Ctrl Pts',(121.761192595294,-1.36773221916774,38.1192402630671));
#68036=CARTESIAN_POINT('Ctrl Pts',(121.653095242547,-1.36772474312819,38.2274155681001));
#68037=CARTESIAN_POINT('Ctrl Pts',(121.54499769289,-1.36771721901169,38.3355906629474));
#68038=CARTESIAN_POINT('Ctrl Pts',(121.913823234173,-1.5289633238052,38.0555584828822));
#68039=CARTESIAN_POINT('Ctrl Pts',(121.805730586264,-1.52894179178494,38.1637387275019));
#68040=CARTESIAN_POINT('Ctrl Pts',(121.697637909653,-1.52892049658419,38.2719189220196));
#68041=CARTESIAN_POINT('Ctrl Pts',(121.589544531164,-1.52889933018762,38.3800984089656));
#68042=CARTESIAN_POINT('Ctrl Pts',(121.91213203435,-1.60896117914607,38.0538687927104));
#68043=CARTESIAN_POINT('Ctrl Pts',(121.804044421864,-1.60893560624471,38.1620540571656));
#68044=CARTESIAN_POINT('Ctrl Pts',(121.695956395472,-1.60891025216513,38.2702388941964));
#68045=CARTESIAN_POINT('Ctrl Pts',(121.587867965638,-1.60888511138663,38.3784233147169));
#68046=CARTESIAN_POINT('',(121.375735931282,-1.3,38.1664774376736));
#68047=CARTESIAN_POINT('',(121.587867965638,-1.60888511138651,38.378423314714));
#68048=CARTESIAN_POINT('Origin',(121.375735931282,-1.6,38.1664774376736));
#68049=CARTESIAN_POINT('',(121.91213203435,-1.60896117914593,38.0538687927072));
#68050=CARTESIAN_POINT('Ctrl Pts',(121.587867965638,-1.60888511138663,38.3784233147169));
#68051=CARTESIAN_POINT('Ctrl Pts',(121.695956395472,-1.60891025216513,38.2702388941964));
#68052=CARTESIAN_POINT('Ctrl Pts',(121.804044421864,-1.60893560624471,38.1620540571656));
#68053=CARTESIAN_POINT('Ctrl Pts',(121.91213203435,-1.60896117914607,38.0538687927104));
#68054=CARTESIAN_POINT('Origin',(121.699999999994,-1.6,37.8419261182243));
#68055=CARTESIAN_POINT('Ctrl Pts',(121.699999999994,-1.3,37.8419261182243));
#68056=CARTESIAN_POINT('Ctrl Pts',(121.591912387508,-1.3,37.950110301428));
#68057=CARTESIAN_POINT('Ctrl Pts',(121.483824361116,-1.3,38.0582940710949));
#68058=CARTESIAN_POINT('Ctrl Pts',(121.375735931282,-1.3,38.1664774376736));
#68059=CARTESIAN_POINT('Origin',(121.7,-1.6,37.841926118218));
#68060=CARTESIAN_POINT('Origin',(121.7,-1.6,37.841926118218));
#68061=CARTESIAN_POINT('Origin',(104.3,-0.553665449701519,16.4635827375088));
#68062=CARTESIAN_POINT('',(104.3,-3.65048420269754,37.6878672442806));
#68063=CARTESIAN_POINT('',(104.,-3.3530507442854,37.7270251019467));
#68064=CARTESIAN_POINT('Origin',(104.3,-3.3530507442854,37.7270251019467));
#68065=CARTESIAN_POINT('',(104.,-3.13873638016776,36.099145889284));
#68066=CARTESIAN_POINT('',(104.,-0.553665449701519,16.4635827375088));
#68067=CARTESIAN_POINT('',(104.3,-3.47532769624592,36.3574214900301));
#68068=CARTESIAN_POINT('Origin',(104.3,-3.13873638016776,36.099145889284));
#68069=CARTESIAN_POINT('',(104.3,-0.851098908113666,16.4244248798428));
#68070=CARTESIAN_POINT('Origin',(104.624264068712,0.,0.));
#68071=CARTESIAN_POINT('',(104.412132034356,-1.39632770509236,38.386744539812));
#68072=CARTESIAN_POINT('',(104.412132034356,-3.41426858245336,38.2600922303079));
#68073=CARTESIAN_POINT('Origin',(104.412132034356,-1.94289029309402E-15,
0.));
#68074=CARTESIAN_POINT('',(104.624264068712,-3.42207874082297,38.3476124040547));
#68075=CARTESIAN_POINT('Origin',(104.624264068712,-3.39541319219318,38.0487998398672));
#68076=CARTESIAN_POINT('',(104.624264068712,-1.61256544502617,38.4662141714714));
#68077=CARTESIAN_POINT('Origin',(104.624264068712,0.,0.));
#68078=CARTESIAN_POINT('Ctrl Pts',(104.624264068712,-1.61256544502617,38.4662141714714));
#68079=CARTESIAN_POINT('Ctrl Pts',(104.623447602755,-1.61174649862236,38.4662485030193));
#68080=CARTESIAN_POINT('Ctrl Pts',(104.622631133476,-1.61092740818292,38.4662794783954));
#68081=CARTESIAN_POINT('Ctrl Pts',(104.585817132852,-1.5739888912899,38.4675247911796));
#68082=CARTESIAN_POINT('Ctrl Pts',(104.54955560756,-1.53733192330198,38.4622264673224));
#68083=CARTESIAN_POINT('Ctrl Pts',(104.476315456228,-1.46272037966997,38.4364482549859));
#68084=CARTESIAN_POINT('Ctrl Pts',(104.441383090818,-1.42678484563727,38.4149070554611));
#68085=CARTESIAN_POINT('Ctrl Pts',(104.412132034356,-1.39632770509233,38.386744539812));
#68086=CARTESIAN_POINT('Origin',(113.,-1.6,38.1664774376677));
#68087=CARTESIAN_POINT('',(121.375735931288,-1.61256544502617,38.4662141714714));
#68088=CARTESIAN_POINT('',(113.,-1.61256544502617,38.4662141714714));
#68089=CARTESIAN_POINT('Origin',(121.375735931288,-1.6,38.1664774376677));
#68090=CARTESIAN_POINT('',(104.188611756946,-1.3,38.1664774376677));
#68091=CARTESIAN_POINT('',(113.,-1.3,38.1664774376677));
#68092=CARTESIAN_POINT('Ctrl Pts',(104.188611312035,-1.30000000000033,38.1664778823209));
#68093=CARTESIAN_POINT('Ctrl Pts',(104.192037383128,-1.30000000508132,38.1699059400815));
#68094=CARTESIAN_POINT('Ctrl Pts',(104.195442206093,-1.30005879098899,38.1733107348444));
#68095=CARTESIAN_POINT('Ctrl Pts',(104.234593964868,-1.30139139994017,38.2124398080324));
#68096=CARTESIAN_POINT('Ctrl Pts',(104.273440501065,-1.30939267959732,38.2510389834921));
#68097=CARTESIAN_POINT('Ctrl Pts',(104.347490784093,-1.34162007078634,38.3240173010395));
#68098=CARTESIAN_POINT('Ctrl Pts',(104.382711610234,-1.36576189057206,38.3584163096784));
#68099=CARTESIAN_POINT('Ctrl Pts',(104.411969203877,-1.39615825493878,38.3865877651743));
#68100=CARTESIAN_POINT('Ctrl Pts',(104.412050624034,-1.39624293804697,38.3866661590711));
#68101=CARTESIAN_POINT('Ctrl Pts',(104.412132034356,-1.39632770509232,38.386744539812));
#68102=CARTESIAN_POINT('Ctrl Pts',(104.300000000005,-3.65048420269823,37.6878672442858));
#68103=CARTESIAN_POINT('Ctrl Pts',(104.408087612489,-3.66460507219003,37.7951258968034));
#68104=CARTESIAN_POINT('Ctrl Pts',(104.51617563888,-3.67872588770446,37.9023841393222));
#68105=CARTESIAN_POINT('Ctrl Pts',(104.624264068712,-3.69284665060532,38.0096419822012));
#68106=CARTESIAN_POINT('Ctrl Pts',(104.243382456865,-3.65786767826186,37.7439503091645));
#68107=CARTESIAN_POINT('Ctrl Pts',(104.351473262604,-3.67198802305842,37.8512061044813));
#68108=CARTESIAN_POINT('Ctrl Pts',(104.459564357694,-3.68610876488972,37.9584615504213));
#68109=CARTESIAN_POINT('Ctrl Pts',(104.567655925523,-3.70022901187372,38.0657165831673));
#68110=CARTESIAN_POINT('Ctrl Pts',(104.13070824621,-3.60540421753157,37.8644022801433));
#68111=CARTESIAN_POINT('Ctrl Pts',(104.238805139007,-3.61953157877265,37.9716515954047));
#68112=CARTESIAN_POINT('Ctrl Pts',(104.346902493405,-3.63365869985868,38.078900468474));
#68113=CARTESIAN_POINT('Ctrl Pts',(104.45500004306,-3.64778584282857,38.1861491282932));
#68114=CARTESIAN_POINT('Ctrl Pts',(104.086176765826,-3.45136431096225,37.9295576652633));
#68115=CARTESIAN_POINT('Ctrl Pts',(104.194269413733,-3.46550601417653,38.0368096023995));
#68116=CARTESIAN_POINT('Ctrl Pts',(104.302362090343,-3.4796474760577,38.1440615207735));
#68117=CARTESIAN_POINT('Ctrl Pts',(104.410455468831,-3.49378871787998,38.2513127544414));
#68118=CARTESIAN_POINT('Ctrl Pts',(104.087867965649,-3.37183029953947,37.9383242460686));
#68119=CARTESIAN_POINT('Ctrl Pts',(104.195955578133,-3.38597666428456,38.0455806326541));
#68120=CARTESIAN_POINT('Ctrl Pts',(104.304043604524,-3.40012275628983,38.1528366240338));
#68121=CARTESIAN_POINT('Ctrl Pts',(104.412132034356,-3.41426858245336,38.2600922303079));
#68122=CARTESIAN_POINT('',(104.624264068712,-3.69284665060532,38.0096419822012));
#68123=CARTESIAN_POINT('Origin',(104.624264068712,-3.39541319219318,38.0487998398672));
#68124=CARTESIAN_POINT('',(104.087867965649,-3.37183029953923,37.938324246066));
#68125=CARTESIAN_POINT('Ctrl Pts',(104.412132034356,-3.41426858245336,38.2600922303079));
#68126=CARTESIAN_POINT('Ctrl Pts',(104.304043604524,-3.40012275628983,38.1528366240338));
#68127=CARTESIAN_POINT('Ctrl Pts',(104.195955578133,-3.38597666428456,38.0455806326541));
#68128=CARTESIAN_POINT('Ctrl Pts',(104.087867965649,-3.37183029953947,37.9383242460686));
#68129=CARTESIAN_POINT('Origin',(104.300000000005,-3.35305074428609,37.7270251019518));
#68130=CARTESIAN_POINT('Ctrl Pts',(104.300000000005,-3.65048420269823,37.6878672442858));
#68131=CARTESIAN_POINT('Ctrl Pts',(104.408087612489,-3.66460507219003,37.7951258968034));
#68132=CARTESIAN_POINT('Ctrl Pts',(104.51617563888,-3.67872588770446,37.9023841393222));
#68133=CARTESIAN_POINT('Ctrl Pts',(104.624264068712,-3.69284665060532,38.0096419822012));
#68134=CARTESIAN_POINT('Origin',(104.624264068712,-3.39541319219318,38.0487998398672));
#68135=CARTESIAN_POINT('Origin',(104.624264068712,-3.39541319219318,38.0487998398672));
#68136=CARTESIAN_POINT('Origin',(104.3,-3.35305074428562,37.7270251019466));
#68137=CARTESIAN_POINT('Origin',(104.3,-3.35305074428562,37.7270251019466));
#68138=CARTESIAN_POINT('Origin',(121.375735931288,-1.59999999999975,38.1664774376677));
#68139=CARTESIAN_POINT('Origin',(121.375735931288,-1.59999999999975,38.1664774376677));
#68140=CARTESIAN_POINT('Origin',(113.,-1.3,37.75));
#68141=CARTESIAN_POINT('',(104.3,-1.3,36.5));
#68142=CARTESIAN_POINT('',(103.5,-1.3,36.5));
#68143=CARTESIAN_POINT('',(104.,-1.3,36.2));
#68144=CARTESIAN_POINT('Origin',(104.3,-1.3,36.2));
#68145=CARTESIAN_POINT('',(104.,-1.3,37.8534195593564));
#68146=CARTESIAN_POINT('',(104.,-1.3,18.875));
#68147=CARTESIAN_POINT('',(104.087868515434,-1.3,38.0656759583793));
#68148=CARTESIAN_POINT('Ctrl Pts',(104.087868240379,-1.3,38.0656762332744));
#68149=CARTESIAN_POINT('Ctrl Pts',(104.061688713442,-1.3,38.0394815117177));
#68150=CARTESIAN_POINT('Ctrl Pts',(104.037012788768,-1.3,38.0025291999168));
#68151=CARTESIAN_POINT('Ctrl Pts',(104.008670719845,-1.3,37.9340820569223));
#68152=CARTESIAN_POINT('Ctrl Pts',(104.,-1.3,37.8904723424532));
#68153=CARTESIAN_POINT('Ctrl Pts',(104.,-1.3,37.8534195593564));
#68154=CARTESIAN_POINT('',(104.25,-1.3,38.2279011681123));
#68155=CARTESIAN_POINT('Origin',(122.,33.,0.));
#68156=CARTESIAN_POINT('',(122.,1.3,36.2));
#68157=CARTESIAN_POINT('',(122.,16.5,36.2));
#68158=CARTESIAN_POINT('',(122.,-3.3530507442854,37.7270251019467));
#68159=CARTESIAN_POINT('Origin',(122.,0.,0.));
#68160=CARTESIAN_POINT('',(122.,-3.13873638016776,36.099145889284));
#68161=CARTESIAN_POINT('',(122.,-0.596258166840185,16.787106543887));
#68162=CARTESIAN_POINT('',(122.,-6.01392647815181,35.7206199318459));
#68163=CARTESIAN_POINT('',(122.,11.493839908519,38.0255611038277));
#68164=CARTESIAN_POINT('',(122.,-6.22974103737677,37.3598942576647));
#68165=CARTESIAN_POINT('',(122.,-3.47144826482424,16.4085805864488));
#68166=CARTESIAN_POINT('',(122.,-8.54148233004192,36.9000603243714));
#68167=CARTESIAN_POINT('Origin',(122.,0.,0.));
#68168=CARTESIAN_POINT('',(122.,-8.11354585853546,35.3029796702975));
#68169=CARTESIAN_POINT('',(122.,-2.52421548335591,14.4433147298394));
#68170=CARTESIAN_POINT('',(122.,-10.624953006887,34.630050153031));
#68171=CARTESIAN_POINT('',(122.,6.02546014851037,39.0915149116643));
#68172=CARTESIAN_POINT('',(122.,-11.0528894783935,36.2271308071048));
#68173=CARTESIAN_POINT('',(122.,-5.03562263170748,13.7703852125729));
#68174=CARTESIAN_POINT('',(122.,-13.2848331314657,35.4694880285264));
#68175=CARTESIAN_POINT('Origin',(122.,0.,0.));
#68176=CARTESIAN_POINT('',(122.,-12.6520968593516,33.9419275389832));
#68177=CARTESIAN_POINT('',(122.,-3.60573733841541,12.1020836934361));
#68178=CARTESIAN_POINT('',(122.,-15.3313475036343,32.8321455851244));
#68179=CARTESIAN_POINT('',(122.,0.23049069317278,39.2780700216976));
#68180=CARTESIAN_POINT('',(122.,-15.9596854262438,34.3490875196417));
#68181=CARTESIAN_POINT('',(122.,-6.28498798269814,10.9923017395774));
#68182=CARTESIAN_POINT('',(122.,-17.5353224130539,33.5720693465106));
#68183=CARTESIAN_POINT('Origin',(122.,0.,0.));
#68184=CARTESIAN_POINT('',(122.,-16.7143593539449,32.1501196169967));
#68185=CARTESIAN_POINT('',(122.,-3.9268593539449,10.0015199152097));
#68186=CARTESIAN_POINT('',(122.,-19.2258330249198,30.7001196169967));
#68187=CARTESIAN_POINT('',(122.,-5.72499999999999,38.4948291982183));
#68188=CARTESIAN_POINT('',(122.,-20.052542804598,32.1320229585134));
#68189=CARTESIAN_POINT('',(122.,-6.43833302491977,8.55151991520966));
#68190=CARTESIAN_POINT('',(122.,-22.0123424414419,30.8225267065723));
#68191=CARTESIAN_POINT('Origin',(122.,0.,0.));
#68192=CARTESIAN_POINT('',(122.,-21.0058043877371,29.5107807762541));
#68193=CARTESIAN_POINT('',(122.,-4.34426975225679,7.79704608882359));
#68194=CARTESIAN_POINT('',(122.,-23.0685230724943,27.9280010608314));
#68195=CARTESIAN_POINT('',(122.,-11.6519066080199,36.6882789854275));
#68196=CARTESIAN_POINT('',(122.,-24.0750611261991,29.2397469911497));
#68197=CARTESIAN_POINT('',(122.,-6.40698843701401,6.21426637340092));
#68198=CARTESIAN_POINT('',(122.,-25.8471708459779,27.6856484770629));
#68199=CARTESIAN_POINT('Origin',(122.,0.,0.));
#68200=CARTESIAN_POINT('',(122.,-24.6780266634105,26.5165042944955));
#68201=CARTESIAN_POINT('',(122.,-4.17740167935357,6.0158793104386));
#68202=CARTESIAN_POINT('',(122.,-26.7286363288515,24.4658946290545));
#68203=CARTESIAN_POINT('',(122.,-17.347265478953,33.847265478953));
#68204=CARTESIAN_POINT('',(122.,-27.8896534212507,25.6269117214538));
#68205=CARTESIAN_POINT('',(122.,-6.22801134479456,3.96526964499761));
#68206=CARTESIAN_POINT('',(122.,-29.0480002025284,24.3060703646348));
#68207=CARTESIAN_POINT('Origin',(122.,0.,0.));
#68208=CARTESIAN_POINT('',(122.,-27.7453726321288,23.3065290745817));
#68209=CARTESIAN_POINT('',(122.,-3.61526888948732,4.79084925012077));
#68210=CARTESIAN_POINT('',(122.,-29.510780776254,21.0058043877371));
#68211=CARTESIAN_POINT('',(122.,-22.6046480406385,30.0060517970005));
#68212=CARTESIAN_POINT('',(122.,-30.8225267065723,22.0123424414419));
#68213=CARTESIAN_POINT('',(122.,-5.38067703361261,2.49012456327619));
#68214=CARTESIAN_POINT('',(122.,-32.1320229585134,20.052542804598));
#68215=CARTESIAN_POINT('Origin',(122.,0.,0.));
#68216=CARTESIAN_POINT('',(122.,-30.7001196169967,19.2258330249198));
#68217=CARTESIAN_POINT('',(122.,-3.32122949643128,3.41862344369815));
#68218=CARTESIAN_POINT('',(122.,-32.0001196169967,16.9741669750802));
#68219=CARTESIAN_POINT('',(122.,-27.2251196169967,25.2447095812216));
#68220=CARTESIAN_POINT('',(122.,-33.4320229585134,17.8008767547585));
#68221=CARTESIAN_POINT('',(122.,-4.62122949643128,1.16695739385862));
#68222=CARTESIAN_POINT('',(122.,-34.4745111043772,15.686919915995));
#68223=CARTESIAN_POINT('Origin',(122.,0.,0.));
#68224=CARTESIAN_POINT('',(122.,-32.946950614834,15.0541836438809));
#68225=CARTESIAN_POINT('',(122.,-2.85710676928691,2.59056223336673));
#68226=CARTESIAN_POINT('',(122.,-34.0567325686927,12.3749329995982));
#68227=CARTESIAN_POINT('',(122.,-31.0280700216976,19.6867711964053));
#68228=CARTESIAN_POINT('',(122.,-35.57367450321,13.0032709222077));
#68229=CARTESIAN_POINT('',(122.,-3.96688872314567,-0.0886884109160058));
#68230=CARTESIAN_POINT('',(122.,-36.1383832819455,11.3396925048198));
#68231=CARTESIAN_POINT('Origin',(122.,0.,0.));
#68232=CARTESIAN_POINT('',(122.,-34.5524044395002,10.9147307547738));
#68233=CARTESIAN_POINT('',(122.,-2.42302991782051,2.30569079837259));
#68234=CARTESIAN_POINT('',(122.,-35.3029796702975,8.11354585853547));
#68235=CARTESIAN_POINT('',(122.,-33.8612244928859,13.4942494327113));
#68236=CARTESIAN_POINT('',(122.,-36.9000603243714,8.54148233004193));
#68237=CARTESIAN_POINT('',(122.,-3.17360514861782,-0.495494097865709));
#68238=CARTESIAN_POINT('',(122.,-37.3598942576647,6.22974103737679));
#68239=CARTESIAN_POINT('Origin',(122.,0.,0.));
#68240=CARTESIAN_POINT('',(122.,-35.7206199318459,6.01392647815184));
#68241=CARTESIAN_POINT('',(122.,-2.32494964165979,1.61730307584363));
#68242=CARTESIAN_POINT('',(122.,-36.059988031618,3.43616983857993));
#68243=CARTESIAN_POINT('',(122.,-35.6091920486168,6.86030528046169));
#68244=CARTESIAN_POINT('',(122.,-37.6992623574369,3.65198439780488));
#68245=CARTESIAN_POINT('',(122.,-2.66431774143193,-0.960453563728275));
#68246=CARTESIAN_POINT('',(122.,-37.8534195593564,1.30000000000001));
#68247=CARTESIAN_POINT('Origin',(122.,0.,0.));
#68248=CARTESIAN_POINT('',(122.,-36.2,1.3));
#68249=CARTESIAN_POINT('',(122.,-2.375,1.3));
#68250=CARTESIAN_POINT('',(122.,-36.2,-1.6));
#68251=CARTESIAN_POINT('',(122.,-36.2,6.45388863150655E-15));
#68252=CARTESIAN_POINT('',(122.,-37.841926118218,-1.6));
#68253=CARTESIAN_POINT('',(122.,-2.375,-1.6));
#68254=CARTESIAN_POINT('',(122.,-37.7270251019467,-3.3530507442854));
#68255=CARTESIAN_POINT('Origin',(122.,0.,0.));
#68256=CARTESIAN_POINT('',(122.,-36.099145889284,-3.13873638016776));
#68257=CARTESIAN_POINT('',(122.,-2.70347559909794,1.25788702214042));
#68258=CARTESIAN_POINT('',(122.,-35.7206199318459,-6.01392647815181));
#68259=CARTESIAN_POINT('',(122.,-35.6091920486168,-6.86030528046165));
#68260=CARTESIAN_POINT('',(122.,-37.3598942576647,-6.22974103737676));
#68261=CARTESIAN_POINT('',(122.,-2.32494964165979,-1.61730307584363));
#68262=CARTESIAN_POINT('',(122.,-36.9000603243714,-8.54148233004191));
#68263=CARTESIAN_POINT('Origin',(122.,0.,0.));
#68264=CARTESIAN_POINT('',(122.,-35.3029796702975,-8.11354585853545));
#68265=CARTESIAN_POINT('',(122.,-3.17360514861782,0.495494097865712));
#68266=CARTESIAN_POINT('',(122.,-34.630050153031,-10.624953006887));
#68267=CARTESIAN_POINT('',(122.,-33.8612244928859,-13.4942494327112));
#68268=CARTESIAN_POINT('',(122.,-36.2271308071049,-11.0528894783935));
#68269=CARTESIAN_POINT('',(122.,-2.50067563135127,-2.01591305048587));
#68270=CARTESIAN_POINT('',(122.,-35.4694880285264,-13.2848331314656));
#68271=CARTESIAN_POINT('Origin',(122.,0.,0.));
#68272=CARTESIAN_POINT('',(122.,-33.9419275389832,-12.6520968593516));
#68273=CARTESIAN_POINT('',(122.,-3.85208369343613,-0.188475448837376));
#68274=CARTESIAN_POINT('',(122.,-32.8321455851244,-15.3313475036343));
#68275=CARTESIAN_POINT('',(122.,-31.0280700216976,-19.6867711964052));
#68276=CARTESIAN_POINT('',(122.,-34.3490875196417,-15.9596854262438));
#68277=CARTESIAN_POINT('',(122.,-2.74230173957738,-2.86772609312011));
#68278=CARTESIAN_POINT('',(122.,-33.5720693465106,-17.5353224130539));
#68279=CARTESIAN_POINT('Origin',(122.,0.,0.));
#68280=CARTESIAN_POINT('',(122.,-32.1501196169967,-16.7143593539449));
#68281=CARTESIAN_POINT('',(122.,-4.77122949643128,-0.907149772723275));
#68282=CARTESIAN_POINT('',(122.,-30.7001196169967,-19.2258330249198));
#68283=CARTESIAN_POINT('',(122.,-27.2251196169967,-25.2447095812216));
#68284=CARTESIAN_POINT('',(122.,-32.1320229585134,-20.052542804598));
#68285=CARTESIAN_POINT('',(122.,-3.32122949643128,-3.41862344369815));
#68286=CARTESIAN_POINT('',(122.,-30.8225267065723,-22.0123424414419));
#68287=CARTESIAN_POINT('Origin',(122.,0.,0.));
#68288=CARTESIAN_POINT('',(122.,-29.5107807762541,-21.0058043877371));
#68289=CARTESIAN_POINT('',(122.,-5.3806770336126,-2.49012456327617));
#68290=CARTESIAN_POINT('',(122.,-27.9280010608314,-23.0685230724943));
#68291=CARTESIAN_POINT('',(122.,-22.6046480406385,-30.0060517970005));
#68292=CARTESIAN_POINT('',(122.,-29.2397469911497,-24.0750611261991));
#68293=CARTESIAN_POINT('',(122.,-3.79789731818993,-4.55284324803339));
#68294=CARTESIAN_POINT('',(122.,-27.6856484770629,-25.8471708459779));
#68295=CARTESIAN_POINT('Origin',(122.,0.,0.));
#68296=CARTESIAN_POINT('',(122.,-26.5165042944955,-24.6780266634105));
#68297=CARTESIAN_POINT('',(122.,-6.01587931043859,-4.17740167935356));
#68298=CARTESIAN_POINT('',(122.,-24.4658946290546,-26.7286363288515));
#68299=CARTESIAN_POINT('',(122.,-17.347265478953,-33.847265478953));
#68300=CARTESIAN_POINT('',(122.,-25.6269117214538,-27.8896534212507));
#68301=CARTESIAN_POINT('',(122.,-3.96526964499761,-6.22801134479455));
#68302=CARTESIAN_POINT('',(122.,-24.3060703646348,-29.0480002025284));
#68303=CARTESIAN_POINT('Origin',(122.,0.,0.));
#68304=CARTESIAN_POINT('',(122.,-23.3065290745817,-27.7453726321287));
#68305=CARTESIAN_POINT('',(122.,-6.64499443910137,-6.03163794469829));
#68306=CARTESIAN_POINT('',(122.,-20.7677983856497,-29.6934092049567));
#68307=CARTESIAN_POINT('',(122.,-11.6519066080199,-36.6882789854275));
#68308=CARTESIAN_POINT('',(122.,-21.7673396757028,-30.9960367753563));
#68309=CARTESIAN_POINT('',(122.,-4.10626375016942,-7.9796745175262));
#68310=CARTESIAN_POINT('',(122.,-20.052542804598,-32.1320229585134));
#68311=CARTESIAN_POINT('Origin',(122.,0.,0.));
#68312=CARTESIAN_POINT('',(122.,-19.2258330249198,-30.7001196169967));
#68313=CARTESIAN_POINT('',(122.,-6.43833302491977,-8.55151991520965));
#68314=CARTESIAN_POINT('',(122.,-16.9741669750802,-32.0001196169967));
#68315=CARTESIAN_POINT('',(122.,-5.72500000000002,-38.4948291982183));
#68316=CARTESIAN_POINT('',(122.,-17.8008767547585,-33.4320229585134));
#68317=CARTESIAN_POINT('',(122.,-4.18666697508023,-9.85151991520965));
#68318=CARTESIAN_POINT('',(122.,-15.686919915995,-34.4745111043772));
#68319=CARTESIAN_POINT('Origin',(122.,0.,0.));
#68320=CARTESIAN_POINT('',(122.,-15.0541836438809,-32.946950614834));
#68321=CARTESIAN_POINT('',(122.,-6.00782412294476,-11.1071067692869));
#68322=CARTESIAN_POINT('',(122.,-12.3749329995982,-34.0567325686927));
#68323=CARTESIAN_POINT('',(122.,0.230490693172739,-39.2780700216976));
#68324=CARTESIAN_POINT('',(122.,-13.0032709222078,-35.57367450321));
#68325=CARTESIAN_POINT('',(122.,-3.32857347866203,-12.2168887231457));
#68326=CARTESIAN_POINT('',(122.,-11.3396925048199,-36.1383832819455));
#68327=CARTESIAN_POINT('Origin',(122.,0.,0.));
#68328=CARTESIAN_POINT('',(122.,-10.9147307547738,-34.5524044395002));
#68329=CARTESIAN_POINT('',(122.,-5.32540037959422,-13.6927394990421));
#68330=CARTESIAN_POINT('',(122.,-8.11354585853549,-35.3029796702975));
#68331=CARTESIAN_POINT('',(122.,6.02546014851033,-39.0915149116643));
#68332=CARTESIAN_POINT('',(122.,-8.54148233004195,-36.9000603243714));
#68333=CARTESIAN_POINT('',(122.,-2.52421548335592,-14.4433147298394));
#68334=CARTESIAN_POINT('',(122.,-6.2297410373768,-37.3598942576647));
#68335=CARTESIAN_POINT('Origin',(122.,0.,0.));
#68336=CARTESIAN_POINT('',(122.,-6.01392647815185,-35.7206199318459));
#68337=CARTESIAN_POINT('',(122.,-3.47144826482425,-16.4085805864488));
#68338=CARTESIAN_POINT('',(122.,-3.43616983857994,-36.059988031618));
#68339=CARTESIAN_POINT('',(122.,11.4938399085189,-38.0255611038277));
#68340=CARTESIAN_POINT('',(122.,-3.6519843978049,-37.6992623574369));
#68341=CARTESIAN_POINT('',(122.,-0.893691625252346,-16.7479486862209));
#68342=CARTESIAN_POINT('',(122.,-1.30000000000001,-37.8534195593564));
#68343=CARTESIAN_POINT('Origin',(122.,0.,0.));
#68344=CARTESIAN_POINT('',(122.,-1.30000000000001,-36.2));
#68345=CARTESIAN_POINT('',(122.,-1.3,-18.875));
#68346=CARTESIAN_POINT('',(122.,1.59999999999999,-36.2));
#68347=CARTESIAN_POINT('',(122.,16.5,-36.2));
#68348=CARTESIAN_POINT('',(122.,1.59999999999999,-37.841926118218));
#68349=CARTESIAN_POINT('',(122.,1.6,-18.875));
#68350=CARTESIAN_POINT('',(122.,3.3530507442854,-37.7270251019467));
#68351=CARTESIAN_POINT('Origin',(122.,0.,0.));
#68352=CARTESIAN_POINT('',(122.,3.13873638016776,-36.099145889284));
#68353=CARTESIAN_POINT('',(122.,1.15848203307056,-21.0576207880785));
#68354=CARTESIAN_POINT('',(122.,6.0139264781518,-35.7206199318459));
#68355=CARTESIAN_POINT('',(122.,20.9439362252507,-33.7550468596362));
#68356=CARTESIAN_POINT('',(122.,6.22974103737675,-37.3598942576647));
#68357=CARTESIAN_POINT('',(122.,4.0336721310546,-20.6790948306404));
#68358=CARTESIAN_POINT('',(122.,8.54148233004191,-36.9000603243714));
#68359=CARTESIAN_POINT('Origin',(122.,0.,0.));
#68360=CARTESIAN_POINT('',(122.,8.11354585853545,-35.3029796702976));
#68361=CARTESIAN_POINT('',(122.,4.73479632091266,-22.6933147298394));
#68362=CARTESIAN_POINT('',(122.,10.624953006887,-34.630050153031));
#68363=CARTESIAN_POINT('',(122.,24.7639590139329,-30.8415149116643));
#68364=CARTESIAN_POINT('',(122.,11.0528894783935,-36.2271308071049));
#68365=CARTESIAN_POINT('',(122.,7.24620346926423,-22.0203852125729));
#68366=CARTESIAN_POINT('',(122.,13.2848331314656,-35.4694880285264));
#68367=CARTESIAN_POINT('Origin',(122.,0.,0.));
#68368=CARTESIAN_POINT('',(122.,12.6520968593516,-33.9419275389832));
#68369=CARTESIAN_POINT('',(122.,8.43847544883736,-23.7693455830142));
#68370=CARTESIAN_POINT('',(122.,15.3313475036343,-32.8321455851244));
#68371=CARTESIAN_POINT('',(122.,27.9367711964053,-27.6108081321196));
#68372=CARTESIAN_POINT('',(122.,15.9596854262438,-34.3490875196417));
#68373=CARTESIAN_POINT('',(122.,11.1177260931201,-22.6595636291554));
#68374=CARTESIAN_POINT('',(122.,17.5353224130539,-33.5720693465106));
#68375=CARTESIAN_POINT('Origin',(122.,0.,0.));
#68376=CARTESIAN_POINT('',(122.,16.7143593539449,-32.1501196169967));
#68377=CARTESIAN_POINT('',(122.,12.1768593539449,-24.2909390776529));
#68378=CARTESIAN_POINT('',(122.,19.2258330249197,-30.7001196169967));
#68379=CARTESIAN_POINT('',(122.,30.475,-24.2054100357751));
#68380=CARTESIAN_POINT('',(122.,20.052542804598,-32.1320229585134));
#68381=CARTESIAN_POINT('',(122.,14.6883330249197,-22.8409390776529));
#68382=CARTESIAN_POINT('',(122.,22.0123424414418,-30.8225267065723));
#68383=CARTESIAN_POINT('Origin',(122.,0.,0.));
#68384=CARTESIAN_POINT('',(122.,21.0058043877371,-29.5107807762541));
#68385=CARTESIAN_POINT('',(122.,16.5737555080652,-23.7348222225932));
#68386=CARTESIAN_POINT('',(122.,23.3065290745816,-27.7453726321288));
#68387=CARTESIAN_POINT('',(122.,32.4224208522115,-20.7505028516579));
#68388=CARTESIAN_POINT('',(122.,24.3060703646347,-29.0480002025284));
#68389=CARTESIAN_POINT('',(122.,18.8744801949098,-21.9694140784679));
#68390=CARTESIAN_POINT('',(122.,25.8471708459779,-27.6856484770629));
#68391=CARTESIAN_POINT('Origin',(122.,0.,0.));
#68392=CARTESIAN_POINT('',(122.,24.6780266634105,-26.5165042944955));
#68393=CARTESIAN_POINT('',(122.,20.6774016793536,-22.5158793104386));
#68394=CARTESIAN_POINT('',(122.,26.7286363288515,-24.4658946290546));
#68395=CARTESIAN_POINT('',(122.,33.847265478953,-17.347265478953));
#68396=CARTESIAN_POINT('',(122.,27.8896534212507,-25.6269117214538));
#68397=CARTESIAN_POINT('',(122.,22.7280113447945,-20.4652696449976));
#68398=CARTESIAN_POINT('',(122.,29.0480002025284,-24.3060703646348));
#68399=CARTESIAN_POINT('Origin',(122.,0.,0.));
#68400=CARTESIAN_POINT('',(122.,27.7453726321287,-23.3065290745817));
#68401=CARTESIAN_POINT('',(122.,24.3857831336789,-20.7286253838904));
#68402=CARTESIAN_POINT('',(122.,29.510780776254,-21.0058043877371));
#68403=CARTESIAN_POINT('',(122.,34.8341337964469,-14.0682756632309));
#68404=CARTESIAN_POINT('',(122.,30.8225267065723,-22.0123424414419));
#68405=CARTESIAN_POINT('',(122.,26.1511912778042,-18.4279006970458));
#68406=CARTESIAN_POINT('',(122.,32.1320229585134,-20.052542804598));
#68407=CARTESIAN_POINT('Origin',(122.,0.,0.));
#68408=CARTESIAN_POINT('',(122.,30.7001196169967,-19.2258330249198));
#68409=CARTESIAN_POINT('',(122.,28.0712294964313,-17.7080426061414));
#68410=CARTESIAN_POINT('',(122.,32.0001196169967,-16.9741669750802));
#68411=CARTESIAN_POINT('',(122.,35.4751196169967,-10.9552904187784));
#68412=CARTESIAN_POINT('',(122.,33.4320229585134,-17.8008767547585));
#68413=CARTESIAN_POINT('',(122.,29.3712294964313,-15.4563765563019));
#68414=CARTESIAN_POINT('',(122.,34.4745111043772,-15.686919915995));
#68415=CARTESIAN_POINT('Origin',(122.,0.,0.));
#68416=CARTESIAN_POINT('',(122.,32.946950614834,-15.0541836438809));
#68417=CARTESIAN_POINT('',(122.,31.0243686588649,-14.2578241229448));
#68418=CARTESIAN_POINT('',(122.,34.0567325686927,-12.3749329995982));
#68419=CARTESIAN_POINT('',(122.,35.8608081321196,-8.01950930682725));
#68420=CARTESIAN_POINT('',(122.,35.57367450321,-13.0032709222078));
#68421=CARTESIAN_POINT('',(122.,32.1341506127237,-11.578573478662));
#68422=CARTESIAN_POINT('',(122.,36.1383832819455,-11.3396925048199));
#68423=CARTESIAN_POINT('Origin',(122.,0.,0.));
#68424=CARTESIAN_POINT('',(122.,34.5524044395002,-10.9147307547738));
#68425=CARTESIAN_POINT('',(122.,33.2124490802637,-10.5556907983726));
#68426=CARTESIAN_POINT('',(122.,35.3029796702975,-8.11354585853549));
#68427=CARTESIAN_POINT('',(122.,36.0718053304427,-5.24424943271127));
#68428=CARTESIAN_POINT('',(122.,36.9000603243714,-8.54148233004195));
#68429=CARTESIAN_POINT('',(122.,33.963024311061,-7.75450590213432));
#68430=CARTESIAN_POINT('',(122.,37.3598942576647,-6.22974103737681));
#68431=CARTESIAN_POINT('Origin',(122.,0.,0.));
#68432=CARTESIAN_POINT('',(122.,35.7206199318459,-6.01392647815186));
#68433=CARTESIAN_POINT('',(122.,34.7627257754294,-5.88781732003526));
#68434=CARTESIAN_POINT('',(122.,36.099145889284,-3.13873638016781));
#68435=CARTESIAN_POINT('',(122.,36.1714159148471,-2.58979103627009));
#68436=CARTESIAN_POINT('',(122.,37.7270251019467,-3.35305074428517));
#68437=CARTESIAN_POINT('',(122.,35.1412517328676,-3.01262722205121));
#68438=CARTESIAN_POINT('',(122.,37.8534195593564,-1.3));
#68439=CARTESIAN_POINT('Origin',(122.,0.,0.));
#68440=CARTESIAN_POINT('',(122.,36.2,-1.3));
#68441=CARTESIAN_POINT('',(122.,35.375,-1.3));
#68442=CARTESIAN_POINT('',(122.,36.2,1.6));
#68443=CARTESIAN_POINT('',(122.,36.2,0.));
#68444=CARTESIAN_POINT('',(122.,37.841926118218,1.6));
#68445=CARTESIAN_POINT('',(122.,35.375,1.6));
#68446=CARTESIAN_POINT('',(122.,37.7082051239441,3.55846015394631));
#68447=CARTESIAN_POINT('Origin',(122.,0.,0.));
#68448=CARTESIAN_POINT('',(121.99999999999,37.3901659198826,3.61129107980547));
#68449=CARTESIAN_POINT('Ctrl Pts',(121.999999999985,37.3901659198775,3.6112910798048));
#68450=CARTESIAN_POINT('Ctrl Pts',(121.999999999986,37.4147644713433,3.61452954054231));
#68451=CARTESIAN_POINT('Ctrl Pts',(121.999987724128,37.439413439332,3.61613920013212));
#68452=CARTESIAN_POINT('Ctrl Pts',(121.999974368396,37.4638391859231,3.61622518432456));
#68453=CARTESIAN_POINT('Ctrl Pts',(121.99996064796,37.4889319253132,3.6163135164836));
#68454=CARTESIAN_POINT('Ctrl Pts',(121.99994679397,37.51379013716,3.61479353886272));
#68455=CARTESIAN_POINT('Ctrl Pts',(121.999942939738,37.5381223118721,3.61172465010631));
#68456=CARTESIAN_POINT('Ctrl Pts',(121.999939088435,37.5624359899569,3.60865809423188));
#68457=CARTESIAN_POINT('Ctrl Pts',(121.999946268812,37.586225548992,3.6040444993169));
#68458=CARTESIAN_POINT('Ctrl Pts',(121.999957114286,37.6091887957611,3.5978955377201));
#68459=CARTESIAN_POINT('Ctrl Pts',(121.999967383637,37.6309322104034,3.59207321551265));
#68460=CARTESIAN_POINT('Ctrl Pts',(121.999981474336,37.6516622887486,3.58494729598929));
#68461=CARTESIAN_POINT('Ctrl Pts',(121.999982177192,37.6711880810454,3.57657789114267));
#68462=CARTESIAN_POINT('Ctrl Pts',(121.999982586305,37.6825534694728,3.57170630716071));
#68463=CARTESIAN_POINT('Ctrl Pts',(121.999978259513,37.69351076305,3.56641246421013));
#68464=CARTESIAN_POINT('Ctrl Pts',(121.999962779518,37.7040202161395,3.56070093829109));
#68465=CARTESIAN_POINT('Ctrl Pts',(121.999960731871,37.7054103750205,3.55994543480174));
#68466=CARTESIAN_POINT('Ctrl Pts',(121.999958484763,37.7067926945339,3.55918261593986));
#68467=CARTESIAN_POINT('Ctrl Pts',(121.999956061457,37.7081671136506,3.5584125488769));
#68468=CARTESIAN_POINT('',(122.,36.059988031618,3.43616983857991));
#68469=CARTESIAN_POINT('',(122.,35.1020938752016,3.31006068046332));
#68470=CARTESIAN_POINT('',(122.,35.6814620741799,6.31135993656396));
#68471=CARTESIAN_POINT('',(122.,36.1714159148471,2.58979103627007));
#68472=CARTESIAN_POINT('',(122.,37.3093412868425,6.5256743006816));
#68473=CARTESIAN_POINT('',(122.,34.7235679177634,6.18525077844737));
#68474=CARTESIAN_POINT('',(122.,36.9211339477026,8.44992546431459));
#68475=CARTESIAN_POINT('Origin',(122.,0.,0.));
#68476=CARTESIAN_POINT('',(121.99999999999,36.5989197935365,8.46079196799643));
#68477=CARTESIAN_POINT('Ctrl Pts',(121.999999999985,36.5989197935316,8.46079196799511));
#68478=CARTESIAN_POINT('Ctrl Pts',(121.999999999986,36.6228851263621,8.46721345957338));
#68479=CARTESIAN_POINT('Ctrl Pts',(121.999987711225,36.64711303615,8.47202665421094));
#68480=CARTESIAN_POINT('Ctrl Pts',(121.999974335413,36.6713185103745,8.47530007007943));
#68481=CARTESIAN_POINT('Ctrl Pts',(121.999960594297,36.6961850586286,8.47866288598191));
#68482=CARTESIAN_POINT('Ctrl Pts',(121.999946712013,36.7210290085033,8.48040052432379));
#68483=CARTESIAN_POINT('Ctrl Pts',(121.999942827852,36.7455535940209,8.48053383551588));
#68484=CARTESIAN_POINT('Ctrl Pts',(121.999938946639,36.7700595619423,8.4806670455061));
#68485=CARTESIAN_POINT('Ctrl Pts',(121.999946095472,36.7942478221578,8.47919803143947));
#68486=CARTESIAN_POINT('Ctrl Pts',(121.999956913762,36.8178172451242,8.47609893109096));
#68487=CARTESIAN_POINT('Ctrl Pts',(121.999967157364,36.8401346160559,8.47316446077613));
#68488=CARTESIAN_POINT('Ctrl Pts',(121.999981226569,36.8616174742831,8.46880528228881));
#68489=CARTESIAN_POINT('Ctrl Pts',(121.999981917037,36.882068659817,8.46305607728145));
#68490=CARTESIAN_POINT('Ctrl Pts',(121.999982318937,36.893972657035,8.45970964436685));
#68491=CARTESIAN_POINT('Ctrl Pts',(121.999977988042,36.9055271696955,8.4558913045846));
#68492=CARTESIAN_POINT('Ctrl Pts',(121.99996250808,36.9166921957328,8.45160040851319));
#68493=CARTESIAN_POINT('Ctrl Pts',(121.999960460433,36.9181690746058,8.45103282060672));
#68494=CARTESIAN_POINT('Ctrl Pts',(121.999958213397,36.9196391360696,8.45045695678252));
#68495=CARTESIAN_POINT('Ctrl Pts',(121.999955790232,36.9211023108481,8.44987287566783));
#68496=CARTESIAN_POINT('',(122.,35.3029796702975,8.11354585853546));
#68497=CARTESIAN_POINT('',(122.,33.9630243110611,7.75450590213429));
#68498=CARTESIAN_POINT('',(122.,34.5524044395002,10.9147307547738));
#68499=CARTESIAN_POINT('',(122.,36.0718053304427,5.24424943271125));
#68500=CARTESIAN_POINT('',(122.,36.1383832819455,11.3396925048198));
#68501=CARTESIAN_POINT('',(122.,33.2124490802637,10.5556907983726));
#68502=CARTESIAN_POINT('',(122.,35.5023319331436,13.1968102072265));
#68503=CARTESIAN_POINT('Origin',(122.,0.,0.));
#68504=CARTESIAN_POINT('',(121.99999999999,35.1814560023854,13.1655263598403));
#68505=CARTESIAN_POINT('Ctrl Pts',(121.999999999985,35.1814560023807,13.1655263598383));
#68506=CARTESIAN_POINT('Ctrl Pts',(121.999999999986,35.2043780829081,13.1750209964706));
#68507=CARTESIAN_POINT('Ctrl Pts',(121.999987701162,35.2277704127031,13.1829553589989));
#68508=CARTESIAN_POINT('Ctrl Pts',(121.999974309691,35.2513414779448,13.1893601851582));
#68509=CARTESIAN_POINT('Ctrl Pts',(121.999960552446,35.275556363974,13.1959399529326));
#68510=CARTESIAN_POINT('Ctrl Pts',(121.999946648096,35.2999609717918,13.2009054850175));
#68511=CARTESIAN_POINT('Ctrl Pts',(121.999942740594,35.3242583539513,13.2042387253936));
#68512=CARTESIAN_POINT('Ctrl Pts',(121.999938836055,35.3485373105397,13.2075694380547));
#68513=CARTESIAN_POINT('Ctrl Pts',(121.999945960287,35.3727104092644,13.2092701576887));
#68514=CARTESIAN_POINT('Ctrl Pts',(121.999956757376,35.3964827340622,13.2092739626102));
#68515=CARTESIAN_POINT('Ctrl Pts',(121.999966980897,35.4189922132096,13.2092775654047));
#68516=CARTESIAN_POINT('Ctrl Pts',(121.999981033339,35.4408602809818,13.2077597257109));
#68517=CARTESIAN_POINT('Ctrl Pts',(121.999981714146,35.461886938273,13.2047291002568));
#68518=CARTESIAN_POINT('Ctrl Pts',(121.999982110422,35.4741258713076,13.2029650717918));
#68519=CARTESIAN_POINT('Ctrl Pts',(121.999977776326,35.4860799076194,13.2006875622858));
#68520=CARTESIAN_POINT('Ctrl Pts',(121.999962296389,35.4977094726143,13.197890707857));
#68521=CARTESIAN_POINT('Ctrl Pts',(121.999960248743,35.4992478016722,13.1975207471198));
#68522=CARTESIAN_POINT('Ctrl Pts',(121.999958001763,35.500780451891,13.1971416915083));
#68523=CARTESIAN_POINT('Ctrl Pts',(121.999955578709,35.5023073469343,13.1967535901029));
#68524=CARTESIAN_POINT('',(122.,33.9419275389832,12.6520968593516));
#68525=CARTESIAN_POINT('',(122.,32.0193455830142,11.8557373384154));
#68526=CARTESIAN_POINT('',(122.,32.8321455851244,15.3313475036343));
#68527=CARTESIAN_POINT('',(122.,35.8608081321196,8.01950930682723));
#68528=CARTESIAN_POINT('',(122.,34.3490875196417,15.9596854262438));
#68529=CARTESIAN_POINT('',(122.,30.9095636291554,14.5349879826981));
#68530=CARTESIAN_POINT('',(122.,33.5720693465106,17.5353224130539));
#68531=CARTESIAN_POINT('Origin',(122.,0.,0.));
#68532=CARTESIAN_POINT('',(122.,32.1501196169967,16.7143593539449));
#68533=CARTESIAN_POINT('',(122.,29.5212294964313,15.1965689351665));
#68534=CARTESIAN_POINT('',(122.,30.7001196169967,19.2258330249198));
#68535=CARTESIAN_POINT('',(122.,35.4751196169967,10.9552904187784));
#68536=CARTESIAN_POINT('',(122.,32.1320229585134,20.052542804598));
#68537=CARTESIAN_POINT('',(122.,28.0712294964313,17.7080426061414));
#68538=CARTESIAN_POINT('',(122.,30.8225267065723,22.0123424414419));
#68539=CARTESIAN_POINT('Origin',(122.,0.,0.));
#68540=CARTESIAN_POINT('',(122.,29.5107807762541,21.0058043877371));
#68541=CARTESIAN_POINT('',(122.,26.1511912778042,18.4279006970458));
#68542=CARTESIAN_POINT('',(122.,27.9280010608314,23.0685230724943));
#68543=CARTESIAN_POINT('',(122.,34.8341337964469,14.0682756632309));
#68544=CARTESIAN_POINT('',(122.,29.2397469911497,24.0750611261991));
#68545=CARTESIAN_POINT('',(122.,24.5684115623815,20.490619381803));
#68546=CARTESIAN_POINT('',(122.,27.6856484770629,25.8471708459779));
#68547=CARTESIAN_POINT('Origin',(122.,0.,0.));
#68548=CARTESIAN_POINT('',(122.,26.5165042944955,24.6780266634105));
#68549=CARTESIAN_POINT('',(122.,22.5158793104386,20.6774016793536));
#68550=CARTESIAN_POINT('',(122.,24.4658946290545,26.7286363288515));
#68551=CARTESIAN_POINT('',(122.,33.847265478953,17.347265478953));
#68552=CARTESIAN_POINT('',(122.,25.6269117214538,27.8896534212507));
#68553=CARTESIAN_POINT('',(122.,20.4652696449976,22.7280113447946));
#68554=CARTESIAN_POINT('',(122.,24.3060703646348,29.0480002025284));
#68555=CARTESIAN_POINT('Origin',(122.,0.,0.));
#68556=CARTESIAN_POINT('',(122.,23.3065290745817,27.7453726321288));
#68557=CARTESIAN_POINT('',(122.,18.8744801949098,21.9694140784679));
#68558=CARTESIAN_POINT('',(122.,21.0058043877371,29.510780776254));
#68559=CARTESIAN_POINT('',(122.,32.4224208522115,20.7505028516579));
#68560=CARTESIAN_POINT('',(122.,22.0123424414419,30.8225267065723));
#68561=CARTESIAN_POINT('',(122.,16.5737555080652,23.7348222225932));
#68562=CARTESIAN_POINT('',(122.,20.052542804598,32.1320229585134));
#68563=CARTESIAN_POINT('Origin',(122.,0.,0.));
#68564=CARTESIAN_POINT('',(122.,19.2258330249198,30.7001196169967));
#68565=CARTESIAN_POINT('',(122.,14.6883330249198,22.8409390776529));
#68566=CARTESIAN_POINT('',(122.,16.9741669750802,32.0001196169967));
#68567=CARTESIAN_POINT('',(122.,30.475,24.2054100357751));
#68568=CARTESIAN_POINT('',(122.,17.8008767547584,33.4320229585134));
#68569=CARTESIAN_POINT('',(122.,12.4366669750802,24.1409390776529));
#68570=CARTESIAN_POINT('',(122.,15.686919915995,34.4745111043772));
#68571=CARTESIAN_POINT('Origin',(122.,0.,0.));
#68572=CARTESIAN_POINT('',(122.,15.0541836438809,32.946950614834));
#68573=CARTESIAN_POINT('',(122.,10.8405622333667,22.7743686588649));
#68574=CARTESIAN_POINT('',(122.,12.3749329995982,34.0567325686927));
#68575=CARTESIAN_POINT('',(122.,27.9367711964053,27.6108081321196));
#68576=CARTESIAN_POINT('',(122.,13.0032709222077,35.57367450321));
#68577=CARTESIAN_POINT('',(122.,8.161311589084,23.8841506127237));
#68578=CARTESIAN_POINT('',(122.,11.3396925048198,36.1383832819455));
#68579=CARTESIAN_POINT('Origin',(122.,0.,0.));
#68580=CARTESIAN_POINT('',(122.,10.9147307547738,34.5524044395002));
#68581=CARTESIAN_POINT('',(122.,7.53598121715098,21.9427394990421));
#68582=CARTESIAN_POINT('',(122.,8.11354585853547,35.3029796702975));
#68583=CARTESIAN_POINT('',(122.,24.7639590139329,30.8415149116643));
#68584=CARTESIAN_POINT('',(122.,8.54148233004193,36.9000603243714));
#68585=CARTESIAN_POINT('',(122.,4.73479632091268,22.6933147298394));
#68586=CARTESIAN_POINT('',(122.,6.22974103737678,37.3598942576647));
#68587=CARTESIAN_POINT('Origin',(122.,0.,0.));
#68588=CARTESIAN_POINT('',(122.,6.01392647815183,35.7206199318459));
#68589=CARTESIAN_POINT('',(122.,4.03367213105462,20.6790948306404));
#68590=CARTESIAN_POINT('',(122.,3.43616983857992,36.059988031618));
#68591=CARTESIAN_POINT('',(122.,20.9439362252507,33.7550468596361));
#68592=CARTESIAN_POINT('',(122.,3.65198439780487,37.6992623574369));
#68593=CARTESIAN_POINT('',(122.,1.45591549148271,21.0184629304125));
#68594=CARTESIAN_POINT('',(122.,1.3,37.8534195593564));
#68595=CARTESIAN_POINT('Origin',(122.,0.,0.));
#68596=CARTESIAN_POINT('',(122.,1.3,18.875));
#68597=CARTESIAN_POINT('',(122.,-4.07807384116069E-15,33.3));
#68598=CARTESIAN_POINT('Origin',(122.,0.,0.));
#68599=CARTESIAN_POINT('Origin',(121.7,0.,0.));
#68600=CARTESIAN_POINT('',(121.912132034351,-3.37183029953924,37.938324246066));
#68601=CARTESIAN_POINT('Origin',(121.912132034356,-1.94289029309402E-15,
0.));
#68602=CARTESIAN_POINT('Origin',(121.7,-3.35305074428562,37.7270251019467));
#68603=CARTESIAN_POINT('Origin',(121.75,0.,0.));
#68604=CARTESIAN_POINT('',(121.587867965644,-3.41426858245336,38.2600922303079));
#68605=CARTESIAN_POINT('Origin',(121.587867965644,-1.94289029309402E-15,
0.));
#68606=CARTESIAN_POINT('Ctrl Pts',(121.912132034351,-3.37183029953947,37.9383242460686));
#68607=CARTESIAN_POINT('Ctrl Pts',(121.804044421867,-3.38597666428456,38.0455806326541));
#68608=CARTESIAN_POINT('Ctrl Pts',(121.695956395476,-3.40012275628983,38.1528366240338));
#68609=CARTESIAN_POINT('Ctrl Pts',(121.587867965644,-3.41426858245336,38.2600922303079));
#68610=CARTESIAN_POINT('Origin',(121.375735931288,0.,0.));
#68611=CARTESIAN_POINT('',(121.375735931288,-3.42207874082297,38.3476124040547));
#68612=CARTESIAN_POINT('Origin',(121.375735931288,0.,0.));
#68613=CARTESIAN_POINT('Origin',(121.375735931288,-3.39541319219318,38.0487998398672));
#68614=CARTESIAN_POINT('Origin',(113.,0.,0.));
#68615=CARTESIAN_POINT('',(113.,-3.42207874082297,38.3476124040547));
#68616=CARTESIAN_POINT('Origin',(121.7,-2.375,-1.6));
#68617=CARTESIAN_POINT('',(121.7,-37.841926118218,-1.3));
#68618=CARTESIAN_POINT('Origin',(121.7,-37.841926118218,-1.6));
#68619=CARTESIAN_POINT('',(121.7,-36.5,-1.3));
#68620=CARTESIAN_POINT('Origin',(121.7,-36.2,-1.6));
#68621=CARTESIAN_POINT('',(121.7,-2.375,-1.3));
#68622=CARTESIAN_POINT('Ctrl Pts',(121.699999999994,-37.8419261182244,-1.3));
#68623=CARTESIAN_POINT('Ctrl Pts',(121.591912387508,-37.950110301428,-1.3));
#68624=CARTESIAN_POINT('Ctrl Pts',(121.483824361116,-38.058294071095,-1.3));
#68625=CARTESIAN_POINT('Ctrl Pts',(121.375735931282,-38.1664774376737,-1.3));
#68626=CARTESIAN_POINT('Ctrl Pts',(121.756617543134,-37.8984931216592,-1.3));
#68627=CARTESIAN_POINT('Ctrl Pts',(121.648526737394,-38.0066744036193,-1.30000014726686));
#68628=CARTESIAN_POINT('Ctrl Pts',(121.540435642302,-38.114855391015,-1.29999985529284));
#68629=CARTESIAN_POINT('Ctrl Pts',(121.432344074471,-38.223035904161,-1.3));
#68630=CARTESIAN_POINT('Ctrl Pts',(121.869289488093,-38.011064489895,-1.3677398741357));
#68631=CARTESIAN_POINT('Ctrl Pts',(121.761192595294,-38.1192402630672,-1.36773221916773));
#68632=CARTESIAN_POINT('Ctrl Pts',(121.653095242547,-38.2274155681001,-1.36772474312819));
#68633=CARTESIAN_POINT('Ctrl Pts',(121.54499769289,-38.3355906629475,-1.36771721901169));
#68634=CARTESIAN_POINT('Ctrl Pts',(121.913823234172,-38.0555584828823,-1.52896332380519));
#68635=CARTESIAN_POINT('Ctrl Pts',(121.805730586264,-38.163738727502,-1.52894179178493));
#68636=CARTESIAN_POINT('Ctrl Pts',(121.697637909653,-38.2719189220197,-1.52892049658418));
#68637=CARTESIAN_POINT('Ctrl Pts',(121.589544531163,-38.3800984089656,-1.52889933018762));
#68638=CARTESIAN_POINT('Ctrl Pts',(121.91213203435,-38.0538687927105,-1.60896117914606));
#68639=CARTESIAN_POINT('Ctrl Pts',(121.804044421864,-38.1620540571657,-1.6089356062447));
#68640=CARTESIAN_POINT('Ctrl Pts',(121.695956395472,-38.2702388941965,-1.60891025216513));
#68641=CARTESIAN_POINT('Ctrl Pts',(121.587867965638,-38.378423314717,-1.60888511138663));
#68642=CARTESIAN_POINT('',(121.375735931282,-38.1664774376737,-1.3));
#68643=CARTESIAN_POINT('',(121.587867965638,-38.378423314714,-1.6088851113865));
#68644=CARTESIAN_POINT('Origin',(121.375735931282,-38.1664774376737,-1.6));
#68645=CARTESIAN_POINT('',(121.91213203435,-38.0538687927073,-1.60896117914593));
#68646=CARTESIAN_POINT('Ctrl Pts',(121.587867965638,-38.378423314717,-1.60888511138663));
#68647=CARTESIAN_POINT('Ctrl Pts',(121.695956395472,-38.2702388941965,-1.60891025216513));
#68648=CARTESIAN_POINT('Ctrl Pts',(121.804044421864,-38.1620540571657,-1.6089356062447));
#68649=CARTESIAN_POINT('Ctrl Pts',(121.91213203435,-38.0538687927105,-1.60896117914606));
#68650=CARTESIAN_POINT('Origin',(121.699999999994,-37.8419261182244,-1.6));
#68651=CARTESIAN_POINT('Ctrl Pts',(121.699999999994,-37.8419261182244,-1.3));
#68652=CARTESIAN_POINT('Ctrl Pts',(121.591912387508,-37.950110301428,-1.3));
#68653=CARTESIAN_POINT('Ctrl Pts',(121.483824361116,-38.058294071095,-1.3));
#68654=CARTESIAN_POINT('Ctrl Pts',(121.375735931282,-38.1664774376737,-1.3));
#68655=CARTESIAN_POINT('Origin',(121.7,-37.841926118218,-1.59999999999999));
#68656=CARTESIAN_POINT('Origin',(121.7,-37.841926118218,-1.59999999999999));
#68657=CARTESIAN_POINT('Origin',(104.3,-0.246068316236606,1.58141082851857));
#68658=CARTESIAN_POINT('',(104.3,-37.6878672442806,-3.65048420269754));
#68659=CARTESIAN_POINT('',(104.,-37.7270251019467,-3.3530507442854));
#68660=CARTESIAN_POINT('Origin',(104.3,-37.7270251019467,-3.3530507442854));
#68661=CARTESIAN_POINT('',(104.,-36.099145889284,-3.13873638016776));
#68662=CARTESIAN_POINT('',(104.,-0.246068316236606,1.58141082851857));
#68663=CARTESIAN_POINT('',(104.3,-36.3574214900301,-3.47532769624592));
#68664=CARTESIAN_POINT('Origin',(104.3,-36.099145889284,-3.13873638016776));
#68665=CARTESIAN_POINT('',(104.3,-0.206910458570591,1.28397737010643));
#68666=CARTESIAN_POINT('Origin',(104.624264068712,0.,0.));
#68667=CARTESIAN_POINT('',(104.412132034356,-38.386744539812,-1.39632770509236));
#68668=CARTESIAN_POINT('',(104.412132034356,-38.2600922303079,-3.41426858245335));
#68669=CARTESIAN_POINT('Origin',(104.412132034356,0.,2.77555756156289E-15));
#68670=CARTESIAN_POINT('',(104.624264068712,-38.3476124040547,-3.42207874082296));
#68671=CARTESIAN_POINT('Origin',(104.624264068712,-38.0487998398672,-3.39541319219318));
#68672=CARTESIAN_POINT('',(104.624264068712,-38.4662141714714,-1.61256544502617));
#68673=CARTESIAN_POINT('Origin',(104.624264068712,0.,0.));
#68674=CARTESIAN_POINT('Ctrl Pts',(104.624264068712,-38.4662141714714,-1.61256544502617));
#68675=CARTESIAN_POINT('Ctrl Pts',(104.623447602755,-38.4662485030193,-1.61174649862237));
#68676=CARTESIAN_POINT('Ctrl Pts',(104.622631133476,-38.4662794783954,-1.61092740818289));
#68677=CARTESIAN_POINT('Ctrl Pts',(104.585817132852,-38.4675247911796,-1.57398889129001));
#68678=CARTESIAN_POINT('Ctrl Pts',(104.54955560756,-38.4622264673224,-1.53733192330197));
#68679=CARTESIAN_POINT('Ctrl Pts',(104.476315456227,-38.4364482549859,-1.46272037966975));
#68680=CARTESIAN_POINT('Ctrl Pts',(104.441383090818,-38.414907055461,-1.42678484563711));
#68681=CARTESIAN_POINT('Ctrl Pts',(104.412132034356,-38.386744539812,-1.39632770509232));
#68682=CARTESIAN_POINT('Origin',(113.,-38.1664774376677,-1.6));
#68683=CARTESIAN_POINT('',(121.375735931288,-38.4662141714714,-1.61256544502617));
#68684=CARTESIAN_POINT('',(113.,-38.4662141714714,-1.61256544502617));
#68685=CARTESIAN_POINT('Origin',(121.375735931288,-38.1664774376677,-1.6));
#68686=CARTESIAN_POINT('',(104.188611756946,-38.1664774376677,-1.3));
#68687=CARTESIAN_POINT('',(113.,-38.1664774376677,-1.3));
#68688=CARTESIAN_POINT('Ctrl Pts',(104.188611312035,-38.1664778823209,-1.30000000000032));
#68689=CARTESIAN_POINT('Ctrl Pts',(104.192037383128,-38.1699059400815,-1.30000000508131));
#68690=CARTESIAN_POINT('Ctrl Pts',(104.195442206093,-38.1733107348444,-1.30005879098899));
#68691=CARTESIAN_POINT('Ctrl Pts',(104.234593964868,-38.2124398080324,-1.30139139994017));
#68692=CARTESIAN_POINT('Ctrl Pts',(104.273440501065,-38.2510389834921,-1.30939267959732));
#68693=CARTESIAN_POINT('Ctrl Pts',(104.347490784093,-38.3240173010395,-1.34162007078635));
#68694=CARTESIAN_POINT('Ctrl Pts',(104.382711610234,-38.3584163096784,-1.36576189057206));
#68695=CARTESIAN_POINT('Ctrl Pts',(104.411969203877,-38.3865877651743,-1.39615825493878));
#68696=CARTESIAN_POINT('Ctrl Pts',(104.412050624034,-38.3866661590711,-1.39624293804698));
#68697=CARTESIAN_POINT('Ctrl Pts',(104.412132034356,-38.386744539812,-1.39632770509232));
#68698=CARTESIAN_POINT('Ctrl Pts',(104.300000000005,-37.6878672442858,-3.65048420269822));
#68699=CARTESIAN_POINT('Ctrl Pts',(104.408087612489,-37.7951258968034,-3.66460507219002));
#68700=CARTESIAN_POINT('Ctrl Pts',(104.51617563888,-37.9023841393221,-3.67872588770445));
#68701=CARTESIAN_POINT('Ctrl Pts',(104.624264068712,-38.0096419822012,-3.69284665060531));
#68702=CARTESIAN_POINT('Ctrl Pts',(104.243382456865,-37.7439503091645,-3.65786767826186));
#68703=CARTESIAN_POINT('Ctrl Pts',(104.351473262604,-37.8512061044813,-3.67198802305841));
#68704=CARTESIAN_POINT('Ctrl Pts',(104.459564357694,-37.9584615504212,-3.68610876488971));
#68705=CARTESIAN_POINT('Ctrl Pts',(104.567655925523,-38.0657165831673,-3.70022901187371));
#68706=CARTESIAN_POINT('Ctrl Pts',(104.13070824621,-37.8644022801433,-3.60540421753156));
#68707=CARTESIAN_POINT('Ctrl Pts',(104.238805139007,-37.9716515954047,-3.61953157877265));
#68708=CARTESIAN_POINT('Ctrl Pts',(104.346902493405,-38.078900468474,-3.63365869985867));
#68709=CARTESIAN_POINT('Ctrl Pts',(104.45500004306,-38.1861491282932,-3.64778584282857));
#68710=CARTESIAN_POINT('Ctrl Pts',(104.086176765826,-37.9295576652633,-3.45136431096224));
#68711=CARTESIAN_POINT('Ctrl Pts',(104.194269413733,-38.0368096023995,-3.46550601417652));
#68712=CARTESIAN_POINT('Ctrl Pts',(104.302362090343,-38.1440615207734,-3.47964747605769));
#68713=CARTESIAN_POINT('Ctrl Pts',(104.410455468831,-38.2513127544414,-3.49378871787997));
#68714=CARTESIAN_POINT('Ctrl Pts',(104.087867965649,-37.9383242460686,-3.37183029953946));
#68715=CARTESIAN_POINT('Ctrl Pts',(104.195955578133,-38.0455806326541,-3.38597666428455));
#68716=CARTESIAN_POINT('Ctrl Pts',(104.304043604524,-38.1528366240337,-3.40012275628983));
#68717=CARTESIAN_POINT('Ctrl Pts',(104.412132034356,-38.2600922303079,-3.41426858245335));
#68718=CARTESIAN_POINT('',(104.624264068712,-38.0096419822012,-3.69284665060532));
#68719=CARTESIAN_POINT('Origin',(104.624264068712,-38.0487998398672,-3.39541319219317));
#68720=CARTESIAN_POINT('',(104.087867965649,-37.938324246066,-3.37183029953923));
#68721=CARTESIAN_POINT('Ctrl Pts',(104.412132034356,-38.2600922303079,-3.41426858245335));
#68722=CARTESIAN_POINT('Ctrl Pts',(104.304043604524,-38.1528366240337,-3.40012275628983));
#68723=CARTESIAN_POINT('Ctrl Pts',(104.195955578133,-38.0455806326541,-3.38597666428455));
#68724=CARTESIAN_POINT('Ctrl Pts',(104.087867965649,-37.9383242460686,-3.37183029953946));
#68725=CARTESIAN_POINT('Origin',(104.300000000005,-37.7270251019518,-3.35305074428608));
#68726=CARTESIAN_POINT('Ctrl Pts',(104.300000000005,-37.6878672442858,-3.65048420269822));
#68727=CARTESIAN_POINT('Ctrl Pts',(104.408087612489,-37.7951258968034,-3.66460507219002));
#68728=CARTESIAN_POINT('Ctrl Pts',(104.51617563888,-37.9023841393221,-3.67872588770445));
#68729=CARTESIAN_POINT('Ctrl Pts',(104.624264068712,-38.0096419822012,-3.69284665060531));
#68730=CARTESIAN_POINT('Origin',(104.624264068712,-38.0487998398672,-3.39541319219318));
#68731=CARTESIAN_POINT('Origin',(104.624264068712,-38.0487998398672,-3.39541319219318));
#68732=CARTESIAN_POINT('Origin',(104.3,-37.7270251019466,-3.35305074428562));
#68733=CARTESIAN_POINT('Origin',(104.3,-37.7270251019466,-3.35305074428562));
#68734=CARTESIAN_POINT('Origin',(121.375735931288,-38.1664774376677,-1.59999999999975));
#68735=CARTESIAN_POINT('Origin',(121.375735931288,-38.1664774376677,-1.59999999999975));
#68736=CARTESIAN_POINT('Origin',(113.,-37.75,-1.3));
#68737=CARTESIAN_POINT('',(104.3,-36.5,-1.3));
#68738=CARTESIAN_POINT('',(103.5,-36.5,-1.3));
#68739=CARTESIAN_POINT('',(104.,-36.2,-1.3));
#68740=CARTESIAN_POINT('Origin',(104.3,-36.2,-1.3));
#68741=CARTESIAN_POINT('',(104.,-37.8534195593564,-1.3));
#68742=CARTESIAN_POINT('',(104.,0.124999999999999,-1.3));
#68743=CARTESIAN_POINT('',(104.087868515434,-38.0656759583793,-1.3));
#68744=CARTESIAN_POINT('Ctrl Pts',(104.087868240379,-38.0656762332744,-1.3));
#68745=CARTESIAN_POINT('Ctrl Pts',(104.061688713442,-38.0394815117177,-1.3));
#68746=CARTESIAN_POINT('Ctrl Pts',(104.037012788768,-38.0025291999168,-1.3));
#68747=CARTESIAN_POINT('Ctrl Pts',(104.008670719845,-37.9340820569223,-1.3));
#68748=CARTESIAN_POINT('Ctrl Pts',(104.,-37.8904723424532,-1.3));
#68749=CARTESIAN_POINT('Ctrl Pts',(104.,-37.8534195593564,-1.3));
#68750=CARTESIAN_POINT('',(104.25,-38.2279011681123,-1.3));
#68751=CARTESIAN_POINT('Origin',(121.7,0.,0.));
#68752=CARTESIAN_POINT('',(121.912132034351,-37.938324246066,-3.37183029953923));
#68753=CARTESIAN_POINT('Origin',(121.912132034356,0.,3.05311331771918E-15));
#68754=CARTESIAN_POINT('Origin',(121.7,-37.7270251019467,-3.35305074428562));
#68755=CARTESIAN_POINT('Origin',(121.75,0.,0.));
#68756=CARTESIAN_POINT('',(121.587867965644,-38.2600922303079,-3.41426858245336));
#68757=CARTESIAN_POINT('Origin',(121.587867965644,0.,2.77555756156289E-15));
#68758=CARTESIAN_POINT('Ctrl Pts',(121.912132034351,-37.9383242460686,-3.37183029953946));
#68759=CARTESIAN_POINT('Ctrl Pts',(121.804044421867,-38.0455806326541,-3.38597666428455));
#68760=CARTESIAN_POINT('Ctrl Pts',(121.695956395476,-38.1528366240338,-3.40012275628983));
#68761=CARTESIAN_POINT('Ctrl Pts',(121.587867965644,-38.2600922303079,-3.41426858245336));
#68762=CARTESIAN_POINT('Origin',(121.375735931288,0.,0.));
#68763=CARTESIAN_POINT('',(121.375735931288,-38.3476124040547,-3.42207874082296));
#68764=CARTESIAN_POINT('Origin',(121.375735931288,0.,0.));
#68765=CARTESIAN_POINT('Origin',(121.375735931288,-38.0487998398672,-3.39541319219318));
#68766=CARTESIAN_POINT('Origin',(113.,0.,0.));
#68767=CARTESIAN_POINT('',(113.,-38.3476124040547,-3.42207874082296));
#68768=CARTESIAN_POINT('Origin',(121.7,1.6,-18.875));
#68769=CARTESIAN_POINT('',(121.7,1.29999999999999,-37.841926118218));
#68770=CARTESIAN_POINT('Origin',(121.7,1.59999999999999,-37.841926118218));
#68771=CARTESIAN_POINT('',(121.7,1.29999999999999,-36.5));
#68772=CARTESIAN_POINT('Origin',(121.7,1.59999999999999,-36.2));
#68773=CARTESIAN_POINT('',(121.7,1.3,-18.875));
#68774=CARTESIAN_POINT('Ctrl Pts',(121.699999999994,1.29999999999999,-37.8419261182243));
#68775=CARTESIAN_POINT('Ctrl Pts',(121.591912387508,1.29999999999999,-37.950110301428));
#68776=CARTESIAN_POINT('Ctrl Pts',(121.483824361116,1.29999999999999,-38.0582940710949));
#68777=CARTESIAN_POINT('Ctrl Pts',(121.375735931282,1.29999999999999,-38.1664774376736));
#68778=CARTESIAN_POINT('Ctrl Pts',(121.756617543134,1.29999999999999,-37.8984931216591));
#68779=CARTESIAN_POINT('Ctrl Pts',(121.648526737394,1.30000014726686,-38.0066744036192));
#68780=CARTESIAN_POINT('Ctrl Pts',(121.540435642302,1.29999985529284,-38.1148553910149));
#68781=CARTESIAN_POINT('Ctrl Pts',(121.432344074471,1.29999999999999,-38.223035904161));
#68782=CARTESIAN_POINT('Ctrl Pts',(121.869289488093,1.3677398741357,-38.0110644898949));
#68783=CARTESIAN_POINT('Ctrl Pts',(121.761192595294,1.36773221916773,-38.1192402630671));
#68784=CARTESIAN_POINT('Ctrl Pts',(121.653095242547,1.36772474312818,-38.2274155681001));
#68785=CARTESIAN_POINT('Ctrl Pts',(121.54499769289,1.36771721901169,-38.3355906629474));
#68786=CARTESIAN_POINT('Ctrl Pts',(121.913823234173,1.52896332380519,-38.0555584828822));
#68787=CARTESIAN_POINT('Ctrl Pts',(121.805730586264,1.52894179178493,-38.1637387275019));
#68788=CARTESIAN_POINT('Ctrl Pts',(121.697637909653,1.52892049658418,-38.2719189220196));
#68789=CARTESIAN_POINT('Ctrl Pts',(121.589544531164,1.52889933018762,-38.3800984089656));
#68790=CARTESIAN_POINT('Ctrl Pts',(121.91213203435,1.60896117914606,-38.0538687927104));
#68791=CARTESIAN_POINT('Ctrl Pts',(121.804044421864,1.6089356062447,-38.1620540571656));
#68792=CARTESIAN_POINT('Ctrl Pts',(121.695956395472,1.60891025216513,-38.2702388941964));
#68793=CARTESIAN_POINT('Ctrl Pts',(121.587867965638,1.60888511138663,-38.3784233147169));
#68794=CARTESIAN_POINT('',(121.375735931282,1.29999999999999,-38.1664774376736));
#68795=CARTESIAN_POINT('',(121.587867965638,1.6088851113865,-38.378423314714));
#68796=CARTESIAN_POINT('Origin',(121.375735931282,1.59999999999999,-38.1664774376736));
#68797=CARTESIAN_POINT('',(121.91213203435,1.60896117914593,-38.0538687927072));
#68798=CARTESIAN_POINT('Ctrl Pts',(121.587867965638,1.60888511138663,-38.3784233147169));
#68799=CARTESIAN_POINT('Ctrl Pts',(121.695956395472,1.60891025216513,-38.2702388941964));
#68800=CARTESIAN_POINT('Ctrl Pts',(121.804044421864,1.6089356062447,-38.1620540571656));
#68801=CARTESIAN_POINT('Ctrl Pts',(121.91213203435,1.60896117914606,-38.0538687927104));
#68802=CARTESIAN_POINT('Origin',(121.699999999994,1.59999999999999,-37.8419261182243));
#68803=CARTESIAN_POINT('Ctrl Pts',(121.699999999994,1.29999999999999,-37.8419261182243));
#68804=CARTESIAN_POINT('Ctrl Pts',(121.591912387508,1.29999999999999,-37.950110301428));
#68805=CARTESIAN_POINT('Ctrl Pts',(121.483824361116,1.29999999999999,-38.0582940710949));
#68806=CARTESIAN_POINT('Ctrl Pts',(121.375735931282,1.29999999999999,-38.1664774376736));
#68807=CARTESIAN_POINT('Origin',(121.7,1.59999999999999,-37.841926118218));
#68808=CARTESIAN_POINT('Origin',(121.7,1.59999999999999,-37.841926118218));
#68809=CARTESIAN_POINT('Origin',(104.3,1.20107475020922,-21.3811445944567));
#68810=CARTESIAN_POINT('',(104.3,3.65048420269754,-37.6878672442806));
#68811=CARTESIAN_POINT('',(104.,3.3530507442854,-37.7270251019467));
#68812=CARTESIAN_POINT('Origin',(104.3,3.3530507442854,-37.7270251019467));
#68813=CARTESIAN_POINT('',(104.,3.13873638016776,-36.099145889284));
#68814=CARTESIAN_POINT('',(104.,1.20107475020922,-21.3811445944567));
#68815=CARTESIAN_POINT('',(104.3,3.47532769624592,-36.3574214900301));
#68816=CARTESIAN_POINT('Origin',(104.3,3.13873638016776,-36.099145889284));
#68817=CARTESIAN_POINT('',(104.3,1.49850820862136,-21.3419867367907));
#68818=CARTESIAN_POINT('Origin',(104.624264068712,0.,0.));
#68819=CARTESIAN_POINT('',(104.412132034356,1.39632770509236,-38.386744539812));
#68820=CARTESIAN_POINT('',(104.412132034356,3.41426858245336,-38.2600922303079));
#68821=CARTESIAN_POINT('Origin',(104.412132034356,2.35922392732846E-15,
0.));
#68822=CARTESIAN_POINT('',(104.624264068712,3.42207874082296,-38.3476124040547));
#68823=CARTESIAN_POINT('Origin',(104.624264068712,3.39541319219317,-38.0487998398672));
#68824=CARTESIAN_POINT('',(104.624264068712,1.61256544502617,-38.4662141714714));
#68825=CARTESIAN_POINT('Origin',(104.624264068712,0.,0.));
#68826=CARTESIAN_POINT('Ctrl Pts',(104.624264068712,1.61256544502617,-38.4662141714714));
#68827=CARTESIAN_POINT('Ctrl Pts',(104.623447602755,1.61174649862239,-38.4662485030193));
#68828=CARTESIAN_POINT('Ctrl Pts',(104.622631133476,1.61092740818286,-38.4662794783954));
#68829=CARTESIAN_POINT('Ctrl Pts',(104.585817132852,1.57398889128999,-38.4675247911796));
#68830=CARTESIAN_POINT('Ctrl Pts',(104.54955560756,1.53733192330198,-38.4622264673224));
#68831=CARTESIAN_POINT('Ctrl Pts',(104.476315456228,1.46272037967021,-38.436448254986));
#68832=CARTESIAN_POINT('Ctrl Pts',(104.441383090819,1.42678484563744,-38.4149070554613));
#68833=CARTESIAN_POINT('Ctrl Pts',(104.412132034356,1.39632770509232,-38.386744539812));
#68834=CARTESIAN_POINT('Origin',(113.,1.59999999999999,-38.1664774376677));
#68835=CARTESIAN_POINT('',(121.375735931288,1.61256544502617,-38.4662141714714));
#68836=CARTESIAN_POINT('',(113.,1.61256544502617,-38.4662141714714));
#68837=CARTESIAN_POINT('Origin',(121.375735931288,1.59999999999999,-38.1664774376677));
#68838=CARTESIAN_POINT('',(104.188611756946,1.29999999999999,-38.1664774376677));
#68839=CARTESIAN_POINT('',(113.,1.29999999999999,-38.1664774376677));
#68840=CARTESIAN_POINT('Ctrl Pts',(104.188611312035,1.30000000000032,-38.1664778823209));
#68841=CARTESIAN_POINT('Ctrl Pts',(104.192037383128,1.30000000508131,-38.1699059400815));
#68842=CARTESIAN_POINT('Ctrl Pts',(104.195442206093,1.30005879098899,-38.1733107348444));
#68843=CARTESIAN_POINT('Ctrl Pts',(104.234593964868,1.30139139994017,-38.2124398080324));
#68844=CARTESIAN_POINT('Ctrl Pts',(104.273440501065,1.30939267959731,-38.2510389834921));
#68845=CARTESIAN_POINT('Ctrl Pts',(104.347490784093,1.34162007078634,-38.3240173010395));
#68846=CARTESIAN_POINT('Ctrl Pts',(104.382711610234,1.36576189057206,-38.3584163096784));
#68847=CARTESIAN_POINT('Ctrl Pts',(104.411969203877,1.39615825493877,-38.3865877651743));
#68848=CARTESIAN_POINT('Ctrl Pts',(104.412050624034,1.39624293804697,-38.3866661590711));
#68849=CARTESIAN_POINT('Ctrl Pts',(104.412132034356,1.39632770509232,-38.386744539812));
#68850=CARTESIAN_POINT('Ctrl Pts',(104.300000000005,3.65048420269822,-37.6878672442858));
#68851=CARTESIAN_POINT('Ctrl Pts',(104.408087612489,3.66460507219002,-37.7951258968034));
#68852=CARTESIAN_POINT('Ctrl Pts',(104.51617563888,3.67872588770445,-37.9023841393222));
#68853=CARTESIAN_POINT('Ctrl Pts',(104.624264068712,3.69284665060531,-38.0096419822012));
#68854=CARTESIAN_POINT('Ctrl Pts',(104.243382456865,3.65786767826186,-37.7439503091645));
#68855=CARTESIAN_POINT('Ctrl Pts',(104.351473262604,3.67198802305841,-37.8512061044813));
#68856=CARTESIAN_POINT('Ctrl Pts',(104.459564357694,3.68610876488971,-37.9584615504213));
#68857=CARTESIAN_POINT('Ctrl Pts',(104.567655925523,3.70022901187371,-38.0657165831673));
#68858=CARTESIAN_POINT('Ctrl Pts',(104.13070824621,3.60540421753156,-37.8644022801433));
#68859=CARTESIAN_POINT('Ctrl Pts',(104.238805139007,3.61953157877264,-37.9716515954047));
#68860=CARTESIAN_POINT('Ctrl Pts',(104.346902493405,3.63365869985867,-38.078900468474));
#68861=CARTESIAN_POINT('Ctrl Pts',(104.45500004306,3.64778584282857,-38.1861491282932));
#68862=CARTESIAN_POINT('Ctrl Pts',(104.086176765826,3.45136431096225,-37.9295576652633));
#68863=CARTESIAN_POINT('Ctrl Pts',(104.194269413733,3.46550601417652,-38.0368096023995));
#68864=CARTESIAN_POINT('Ctrl Pts',(104.302362090343,3.47964747605769,-38.1440615207735));
#68865=CARTESIAN_POINT('Ctrl Pts',(104.410455468831,3.49378871787997,-38.2513127544414));
#68866=CARTESIAN_POINT('Ctrl Pts',(104.087867965649,3.37183029953946,-37.9383242460686));
#68867=CARTESIAN_POINT('Ctrl Pts',(104.195955578133,3.38597666428456,-38.0455806326541));
#68868=CARTESIAN_POINT('Ctrl Pts',(104.304043604524,3.40012275628983,-38.1528366240338));
#68869=CARTESIAN_POINT('Ctrl Pts',(104.412132034356,3.41426858245335,-38.2600922303079));
#68870=CARTESIAN_POINT('',(104.624264068712,3.69284665060531,-38.0096419822012));
#68871=CARTESIAN_POINT('Origin',(104.624264068712,3.39541319219317,-38.0487998398672));
#68872=CARTESIAN_POINT('',(104.087867965649,3.37183029953923,-37.938324246066));
#68873=CARTESIAN_POINT('Ctrl Pts',(104.412132034356,3.41426858245335,-38.2600922303079));
#68874=CARTESIAN_POINT('Ctrl Pts',(104.304043604524,3.40012275628983,-38.1528366240338));
#68875=CARTESIAN_POINT('Ctrl Pts',(104.195955578133,3.38597666428456,-38.0455806326541));
#68876=CARTESIAN_POINT('Ctrl Pts',(104.087867965649,3.37183029953946,-37.9383242460686));
#68877=CARTESIAN_POINT('Origin',(104.300000000005,3.35305074428608,-37.7270251019518));
#68878=CARTESIAN_POINT('Ctrl Pts',(104.300000000005,3.65048420269822,-37.6878672442858));
#68879=CARTESIAN_POINT('Ctrl Pts',(104.408087612489,3.66460507219002,-37.7951258968034));
#68880=CARTESIAN_POINT('Ctrl Pts',(104.51617563888,3.67872588770445,-37.9023841393222));
#68881=CARTESIAN_POINT('Ctrl Pts',(104.624264068712,3.69284665060531,-38.0096419822012));
#68882=CARTESIAN_POINT('Origin',(104.624264068712,3.39541319219317,-38.0487998398672));
#68883=CARTESIAN_POINT('Origin',(104.624264068712,3.39541319219317,-38.0487998398672));
#68884=CARTESIAN_POINT('Origin',(104.3,3.35305074428562,-37.7270251019466));
#68885=CARTESIAN_POINT('Origin',(104.3,3.35305074428562,-37.7270251019466));
#68886=CARTESIAN_POINT('Origin',(121.375735931288,1.59999999999975,-38.1664774376677));
#68887=CARTESIAN_POINT('Origin',(121.375735931288,1.59999999999975,-38.1664774376677));
#68888=CARTESIAN_POINT('Origin',(113.,1.29999999999999,-37.75));
#68889=CARTESIAN_POINT('',(104.3,1.29999999999999,-36.5));
#68890=CARTESIAN_POINT('',(103.5,1.29999999999999,-36.5));
#68891=CARTESIAN_POINT('',(104.,1.29999999999999,-36.2));
#68892=CARTESIAN_POINT('Origin',(104.3,1.29999999999999,-36.2));
#68893=CARTESIAN_POINT('',(104.,1.3,-37.8534195593564));
#68894=CARTESIAN_POINT('',(104.,1.3,-18.875));
#68895=CARTESIAN_POINT('',(104.087868515434,1.29999999999999,-38.0656759583793));
#68896=CARTESIAN_POINT('Ctrl Pts',(104.087868240379,1.29999999999999,-38.0656762332744));
#68897=CARTESIAN_POINT('Ctrl Pts',(104.061688713442,1.29999999999999,-38.0394815117177));
#68898=CARTESIAN_POINT('Ctrl Pts',(104.037012788768,1.29999999999999,-38.0025291999168));
#68899=CARTESIAN_POINT('Ctrl Pts',(104.008670719845,1.29999999999999,-37.9340820569223));
#68900=CARTESIAN_POINT('Ctrl Pts',(104.,1.29999999999999,-37.8904723424532));
#68901=CARTESIAN_POINT('Ctrl Pts',(104.,1.29999999999999,-37.8534195593564));
#68902=CARTESIAN_POINT('',(104.25,1.29999999999999,-38.2279011681123));
#68903=CARTESIAN_POINT('Origin',(121.7,0.,0.));
#68904=CARTESIAN_POINT('',(121.912132034351,3.37183029953923,-37.938324246066));
#68905=CARTESIAN_POINT('Origin',(121.912132034356,2.4980018054066E-15,0.));
#68906=CARTESIAN_POINT('Origin',(121.7,3.35305074428562,-37.7270251019467));
#68907=CARTESIAN_POINT('Origin',(121.75,0.,0.));
#68908=CARTESIAN_POINT('',(121.587867965644,3.41426858245336,-38.2600922303079));
#68909=CARTESIAN_POINT('Origin',(121.587867965644,2.35922392732846E-15,
0.));
#68910=CARTESIAN_POINT('Ctrl Pts',(121.912132034351,3.37183029953946,-37.9383242460686));
#68911=CARTESIAN_POINT('Ctrl Pts',(121.804044421867,3.38597666428456,-38.0455806326541));
#68912=CARTESIAN_POINT('Ctrl Pts',(121.695956395476,3.40012275628983,-38.1528366240338));
#68913=CARTESIAN_POINT('Ctrl Pts',(121.587867965644,3.41426858245336,-38.2600922303079));
#68914=CARTESIAN_POINT('Origin',(121.375735931288,0.,0.));
#68915=CARTESIAN_POINT('',(121.375735931288,3.42207874082296,-38.3476124040547));
#68916=CARTESIAN_POINT('Origin',(121.375735931288,0.,0.));
#68917=CARTESIAN_POINT('Origin',(121.375735931288,3.39541319219317,-38.0487998398672));
#68918=CARTESIAN_POINT('Origin',(113.,0.,0.));
#68919=CARTESIAN_POINT('',(113.,3.42207874082296,-38.3476124040547));
#68920=CARTESIAN_POINT('Origin',(104.3,21.7152696449976,-23.9780113447946));
#68921=CARTESIAN_POINT('',(104.3,25.8390437558097,-27.6775213868948));
#68922=CARTESIAN_POINT('',(104.,25.6269117214538,-27.8896534212507));
#68923=CARTESIAN_POINT('Origin',(104.3,25.6269117214538,-27.8896534212507));
#68924=CARTESIAN_POINT('',(104.,24.4658946290545,-26.7286363288515));
#68925=CARTESIAN_POINT('',(104.,21.7152696449976,-23.9780113447946));
#68926=CARTESIAN_POINT('',(104.3,24.8901586977665,-26.7286363288515));
#68927=CARTESIAN_POINT('Origin',(104.3,24.4658946290545,-26.7286363288515));
#68928=CARTESIAN_POINT('',(104.3,21.9274016793536,-23.7658793104386));
#68929=CARTESIAN_POINT('Ctrl Pts',(104.300000000002,25.8390437558114,-27.6775213868965));
#68930=CARTESIAN_POINT('Ctrl Pts',(104.408087612488,25.9155415253719,-27.754019156457));
#68931=CARTESIAN_POINT('Ctrl Pts',(104.51617563888,25.9920390025178,-27.8305166336028));
#68932=CARTESIAN_POINT('Ctrl Pts',(104.624264068714,26.0685361946373,-27.9070138257223));
#68933=CARTESIAN_POINT('Ctrl Pts',(104.243382456862,25.8790426675315,-27.7175202986166));
#68934=CARTESIAN_POINT('Ctrl Pts',(104.351473262603,25.9555382814697,-27.7940161208215));
#68935=CARTESIAN_POINT('Ctrl Pts',(104.459564357694,26.0320339977095,-27.8705114241477));
#68936=CARTESIAN_POINT('Ctrl Pts',(104.567655925525,26.108529069824,-27.947006700909));
#68937=CARTESIAN_POINT('Ctrl Pts',(104.130710113065,25.9107439897146,-27.8450194956664));
#68938=CARTESIAN_POINT('Ctrl Pts',(104.238807005864,25.9872412253646,-27.9215059055569));
#68939=CARTESIAN_POINT('Ctrl Pts',(104.346904358902,26.0637380030864,-27.9979921109243));
#68940=CARTESIAN_POINT('Ctrl Pts',(104.455001908559,26.1402346665623,-28.0744781336927));
#68941=CARTESIAN_POINT('Ctrl Pts',(104.086176765823,25.8282031306362,-27.9904837995326));
#68942=CARTESIAN_POINT('Ctrl Pts',(104.194269413732,25.9047133406349,-28.0669635586562));
#68943=CARTESIAN_POINT('Ctrl Pts',(104.302362090344,25.9812233477493,-28.1434434498089));
#68944=CARTESIAN_POINT('Ctrl Pts',(104.410455468833,26.0577327634567,-28.2199229317112));
#68945=CARTESIAN_POINT('Ctrl Pts',(104.087867965646,25.7704413132658,-28.045856034146));
#68946=CARTESIAN_POINT('Ctrl Pts',(104.195955578132,25.8469579301585,-28.1223364854948));
#68947=CARTESIAN_POINT('Ctrl Pts',(104.304043604524,25.9234740900862,-28.1988167893393));
#68948=CARTESIAN_POINT('Ctrl Pts',(104.412132034358,25.9999898046701,-28.2752969494932));
#68949=CARTESIAN_POINT('',(104.624264068714,26.0685361946373,-27.9070138257223));
#68950=CARTESIAN_POINT('',(104.412132034358,25.9999898046693,-28.2752969494924));
#68951=CARTESIAN_POINT('Origin',(104.624264068714,25.8564041602813,-28.1191458600783));
#68952=CARTESIAN_POINT('',(104.087867965646,25.770441313265,-28.0458560341451));
#68953=CARTESIAN_POINT('Ctrl Pts',(104.412132034358,25.9999898046701,-28.2752969494932));
#68954=CARTESIAN_POINT('Ctrl Pts',(104.304043604524,25.9234740900862,-28.1988167893393));
#68955=CARTESIAN_POINT('Ctrl Pts',(104.195955578132,25.8469579301585,-28.1223364854948));
#68956=CARTESIAN_POINT('Ctrl Pts',(104.087867965646,25.7704413132658,-28.045856034146));
#68957=CARTESIAN_POINT('Origin',(104.300000000002,25.6269117214555,-27.8896534212524));
#68958=CARTESIAN_POINT('Ctrl Pts',(104.300000000002,25.8390437558114,-27.6775213868965));
#68959=CARTESIAN_POINT('Ctrl Pts',(104.408087612488,25.9155415253719,-27.754019156457));
#68960=CARTESIAN_POINT('Ctrl Pts',(104.51617563888,25.9920390025178,-27.8305166336028));
#68961=CARTESIAN_POINT('Ctrl Pts',(104.624264068714,26.0685361946373,-27.9070138257223));
#68962=CARTESIAN_POINT('Origin',(104.3,25.6269117214538,-27.8896534212507));
#68963=CARTESIAN_POINT('Origin',(104.3,25.6269117214538,-27.8896534212507));
#68964=CARTESIAN_POINT('Origin',(121.375735931288,0.,0.));
#68965=CARTESIAN_POINT('',(121.587867965644,26.1561745827473,-28.1308801608062));
#68966=CARTESIAN_POINT('',(121.587867965644,24.6397181974285,-29.4682231323184));
#68967=CARTESIAN_POINT('Origin',(121.587867965644,-2.22044604925031E-15,
-4.44089209850063E-15));
#68968=CARTESIAN_POINT('',(121.375735931288,24.6960816898302,-29.5356318566107));
#68969=CARTESIAN_POINT('Origin',(121.375735931288,24.5036446896497,-29.3054840759098));
#68970=CARTESIAN_POINT('',(121.375735931288,26.0594649259364,-28.3399768485066));
#68971=CARTESIAN_POINT('Origin',(121.375735931288,0.,0.));
#68972=CARTESIAN_POINT('Ctrl Pts',(121.375735931288,26.0594649259364,-28.3399768485066));
#68973=CARTESIAN_POINT('Ctrl Pts',(121.376552397245,26.0600682845625,-28.3394220420211));
#68974=CARTESIAN_POINT('Ctrl Pts',(121.377368866525,26.0606693718646,-28.3388647605161));
#68975=CARTESIAN_POINT('Ctrl Pts',(121.414182867143,26.0876694167654,-28.3136258538443));
#68976=CARTESIAN_POINT('Ctrl Pts',(121.45044439244,26.109843326675,-28.2839589824776));
#68977=CARTESIAN_POINT('Ctrl Pts',(121.523684543772,26.1443737063816,-28.2129727052716));
#68978=CARTESIAN_POINT('Ctrl Pts',(121.558616909181,26.1545520379231,-28.1723305172127));
#68979=CARTESIAN_POINT('Ctrl Pts',(121.587867965644,26.1561745827473,-28.1308801608062));
#68980=CARTESIAN_POINT('Origin',(113.,25.8564041602797,-28.1191458600767));
#68981=CARTESIAN_POINT('',(104.624264068712,26.0594649259364,-28.3399768485066));
#68982=CARTESIAN_POINT('',(113.,26.0594649259364,-28.3399768485066));
#68983=CARTESIAN_POINT('Origin',(104.624264068712,25.8564041602797,-28.1191458600767));
#68984=CARTESIAN_POINT('',(121.811388243054,26.0685361946357,-27.9070138257207));
#68985=CARTESIAN_POINT('',(113.,26.0685361946357,-27.9070138257207));
#68986=CARTESIAN_POINT('Ctrl Pts',(121.811388687965,26.0685365090528,-27.9070141401383));
#68987=CARTESIAN_POINT('Ctrl Pts',(121.807962616872,26.0709605083488,-27.9094381466199));
#68988=CARTESIAN_POINT('Ctrl Pts',(121.804557793907,26.0733264939002,-27.9118872679992));
#68989=CARTESIAN_POINT('Ctrl Pts',(121.765406035132,26.100052630067,-27.9404979978181));
#68990=CARTESIAN_POINT('Ctrl Pts',(121.726559498935,26.1216886096789,-27.9734494956375));
#68991=CARTESIAN_POINT('Ctrl Pts',(121.652509215907,26.1505038660466,-28.0478411657046));
#68992=CARTESIAN_POINT('Ctrl Pts',(121.617288389766,26.1577567938406,-28.0892357824599));
#68993=CARTESIAN_POINT('Ctrl Pts',(121.588030796123,26.1561835456905,-28.1306494850441));
#68994=CARTESIAN_POINT('Ctrl Pts',(121.587949375966,26.1561790985465,-28.1307647979002));
#68995=CARTESIAN_POINT('Ctrl Pts',(121.587867965644,26.1561745827473,-28.1308801608062));
#68996=CARTESIAN_POINT('Origin',(104.624264068712,25.8564041602798,-28.1191458600766));
#68997=CARTESIAN_POINT('Origin',(104.624264068712,25.8564041602798,-28.1191458600766));
#68998=CARTESIAN_POINT('Origin',(121.7,18.8744801949098,-21.9694140784679));
#68999=CARTESIAN_POINT('',(121.7,24.0680643625474,-29.230628631231));
#69000=CARTESIAN_POINT('Origin',(121.7,24.3060703646347,-29.0480002025284));
#69001=CARTESIAN_POINT('',(121.7,23.2511515011969,-28.1660070629188));
#69002=CARTESIAN_POINT('Origin',(121.7,23.3065290745816,-27.7453726321288));
#69003=CARTESIAN_POINT('',(121.7,18.6364741928224,-22.1520425071705));
#69004=CARTESIAN_POINT('Ctrl Pts',(121.699999999997,24.068064362549,-29.2306286312331));
#69005=CARTESIAN_POINT('Ctrl Pts',(121.591912387512,24.1339227205117,-29.3164569143438));
#69006=CARTESIAN_POINT('Ctrl Pts',(121.483824361121,24.1997808267293,-29.4022848693738));
#69007=CARTESIAN_POINT('Ctrl Pts',(121.375735931288,24.2656386875623,-29.4881125046125));
#69008=CARTESIAN_POINT('Ctrl Pts',(121.756617543138,24.1025001723946,-29.2755062523583));
#69009=CARTESIAN_POINT('Ctrl Pts',(121.648526737398,24.1683568810269,-29.3613321441074));
#69010=CARTESIAN_POINT('Ctrl Pts',(121.540435642307,24.2342130618665,-29.4471580695557));
#69011=CARTESIAN_POINT('Ctrl Pts',(121.432344074477,24.3000693004437,-29.5329833529219));
#69012=CARTESIAN_POINT('Ctrl Pts',(121.869287710261,24.2247717885901,-29.3235748067436));
#69013=CARTESIAN_POINT('Ctrl Pts',(121.761190817463,24.2906189537557,-29.409401077777));
#69014=CARTESIAN_POINT('Ctrl Pts',(121.653093466012,24.3564659757562,-29.4952268701867));
#69015=CARTESIAN_POINT('Ctrl Pts',(121.544995916356,24.4223128317953,-29.5810525234116));
#69016=CARTESIAN_POINT('Ctrl Pts',(121.913823234176,24.3797643238856,-29.2607305411385));
#69017=CARTESIAN_POINT('Ctrl Pts',(121.805730586269,24.4456032016902,-29.3465688074239));
#69018=CARTESIAN_POINT('Ctrl Pts',(121.697637909658,24.5114422368762,-29.4324068897942));
#69019=CARTESIAN_POINT('Ctrl Pts',(121.589544531169,24.577280943507,-29.518244332399));
#69020=CARTESIAN_POINT('Ctrl Pts',(121.912132034353,24.4422022714329,-29.2106904110617));
#69021=CARTESIAN_POINT('Ctrl Pts',(121.804044421868,24.5080409992732,-29.2965351197829));
#69022=CARTESIAN_POINT('Ctrl Pts',(121.695956395477,24.5738796405169,-29.3823793561953));
#69023=CARTESIAN_POINT('Ctrl Pts',(121.587867965644,24.6397181974285,-29.4682231323184));
#69024=CARTESIAN_POINT('',(121.375735931288,24.2656386875623,-29.4881125046124));
#69025=CARTESIAN_POINT('Origin',(121.375735931288,24.5036446896497,-29.3054840759098));
#69026=CARTESIAN_POINT('',(121.912132034353,24.4422022714321,-29.2106904110607));
#69027=CARTESIAN_POINT('Ctrl Pts',(121.587867965644,24.6397181974285,-29.4682231323184));
#69028=CARTESIAN_POINT('Ctrl Pts',(121.695956395477,24.5738796405169,-29.3823793561953));
#69029=CARTESIAN_POINT('Ctrl Pts',(121.804044421868,24.5080409992732,-29.2965351197829));
#69030=CARTESIAN_POINT('Ctrl Pts',(121.912132034353,24.4422022714329,-29.2106904110617));
#69031=CARTESIAN_POINT('Origin',(121.699999999997,24.3060703646363,-29.0480002025305));
#69032=CARTESIAN_POINT('Ctrl Pts',(121.699999999997,24.068064362549,-29.2306286312331));
#69033=CARTESIAN_POINT('Ctrl Pts',(121.591912387512,24.1339227205117,-29.3164569143438));
#69034=CARTESIAN_POINT('Ctrl Pts',(121.483824361121,24.1997808267293,-29.4022848693738));
#69035=CARTESIAN_POINT('Ctrl Pts',(121.375735931288,24.2656386875623,-29.4881125046125));
#69036=CARTESIAN_POINT('Origin',(121.7,24.3060703646347,-29.0480002025284));
#69037=CARTESIAN_POINT('Origin',(121.7,24.3060703646347,-29.0480002025284));
#69038=CARTESIAN_POINT('Origin',(121.375735931288,24.5036446896497,-29.3054840759098));
#69039=CARTESIAN_POINT('Origin',(121.375735931288,24.5036446896497,-29.3054840759098));
#69040=CARTESIAN_POINT('Origin',(104.3,0.,0.));
#69041=CARTESIAN_POINT('',(104.087867965647,24.442202271432,-29.2106904110607));
#69042=CARTESIAN_POINT('Origin',(104.087867965644,-2.22044604925031E-15,
-2.22044604925031E-15));
#69043=CARTESIAN_POINT('',(104.,24.3060703646347,-29.0480002025284));
#69044=CARTESIAN_POINT('Origin',(104.3,24.3060703646347,-29.0480002025284));
#69045=CARTESIAN_POINT('Origin',(104.,0.,0.));
#69046=CARTESIAN_POINT('Origin',(104.25,0.,0.));
#69047=CARTESIAN_POINT('',(104.412132034356,24.6397181974285,-29.4682231323184));
#69048=CARTESIAN_POINT('Origin',(104.412132034356,-2.22044604925031E-15,
-4.44089209850063E-15));
#69049=CARTESIAN_POINT('Ctrl Pts',(104.087867965647,24.4422022714329,-29.2106904110617));
#69050=CARTESIAN_POINT('Ctrl Pts',(104.195955578132,24.5080409992732,-29.2965351197829));
#69051=CARTESIAN_POINT('Ctrl Pts',(104.304043604523,24.573879640517,-29.3823793561953));
#69052=CARTESIAN_POINT('Ctrl Pts',(104.412132034356,24.6397181974285,-29.4682231323184));
#69053=CARTESIAN_POINT('Origin',(104.624264068712,0.,0.));
#69054=CARTESIAN_POINT('',(104.624264068712,24.6960816898302,-29.5356318566107));
#69055=CARTESIAN_POINT('Origin',(104.624264068712,0.,0.));
#69056=CARTESIAN_POINT('Origin',(104.624264068712,24.5036446896497,-29.3054840759098));
#69057=CARTESIAN_POINT('Origin',(113.,0.,0.));
#69058=CARTESIAN_POINT('',(113.,24.6960816898302,-29.5356318566107));
#69059=CARTESIAN_POINT('Origin',(113.,24.5036446896497,-29.3054840759098));
#69060=CARTESIAN_POINT('',(104.624264068712,24.2656386875623,-29.4881125046124));
#69061=CARTESIAN_POINT('',(113.,24.2656386875623,-29.4881125046124));
#69062=CARTESIAN_POINT('Origin',(104.624264068712,24.5036446896497,-29.3054840759098));
#69063=CARTESIAN_POINT('Origin',(113.,24.0121032874578,-29.1576987382828));
#69064=CARTESIAN_POINT('',(104.3,23.2511515011969,-28.1660070629188));
#69065=CARTESIAN_POINT('',(103.5,23.2511515011969,-28.1660070629188));
#69066=CARTESIAN_POINT('',(104.300000000003,24.068064362549,-29.2306286312331));
#69067=CARTESIAN_POINT('',(104.3,19.5629503864442,-23.3594497900319));
#69068=CARTESIAN_POINT('Ctrl Pts',(104.624264068712,24.2656386875623,-29.4881125046124));
#69069=CARTESIAN_POINT('Ctrl Pts',(104.516175638879,24.1997808267293,-29.4022848693738));
#69070=CARTESIAN_POINT('Ctrl Pts',(104.408087612488,24.1339227205117,-29.3164569143438));
#69071=CARTESIAN_POINT('Ctrl Pts',(104.300000000003,24.068064362549,-29.2306286312331));
#69072=CARTESIAN_POINT('Origin',(104.3,-6.0731406460551,-7.3189881604791));
#69073=CARTESIAN_POINT('',(104.3,-20.0467960840288,-32.1220693465106));
#69074=CARTESIAN_POINT('',(104.,-20.3066037051641,-31.9720693465106));
#69075=CARTESIAN_POINT('Origin',(104.3,-20.3066037051641,-31.9720693465106));
#69076=CARTESIAN_POINT('',(104.,-19.4856406460551,-30.5501196169967));
#69077=CARTESIAN_POINT('',(104.,-6.0731406460551,-7.3189881604791));
#69078=CARTESIAN_POINT('',(104.3,-19.3758330249198,-30.959927238132));
#69079=CARTESIAN_POINT('Origin',(104.3,-19.4856406460551,-30.5501196169967));
#69080=CARTESIAN_POINT('',(104.3,-5.81333302491977,-7.4689881604791));
#69081=CARTESIAN_POINT('Ctrl Pts',(104.300000000003,-20.0467960840302,-32.122069346513));
#69082=CARTESIAN_POINT('Ctrl Pts',(104.408087612489,-20.100888175632,-32.2157595974551));
#69083=CARTESIAN_POINT('Ctrl Pts',(104.51617563888,-20.1549800604655,-32.3094494902639));
#69084=CARTESIAN_POINT('Ctrl Pts',(104.624264068715,-20.209071743755,-32.4031390339881));
#69085=CARTESIAN_POINT('Ctrl Pts',(104.243382456862,-20.0750795857475,-32.1710578085035));
#69086=CARTESIAN_POINT('Ctrl Pts',(104.351473262603,-20.1291703542645,-32.2647454732615));
#69087=CARTESIAN_POINT('Ctrl Pts',(104.459564357695,-20.1832605951055,-32.3584331025398));
#69088=CARTESIAN_POINT('Ctrl Pts',(104.567655925525,-20.2373509769986,-32.4521201027652));
#69089=CARTESIAN_POINT('Ctrl Pts',(104.130709934827,-20.1900293243368,-32.2346784312497));
#69090=CARTESIAN_POINT('Ctrl Pts',(104.238806827626,-20.2441105815263,-32.3283652263749));
#69091=CARTESIAN_POINT('Ctrl Pts',(104.346904180794,-20.2981917597176,-32.4220515260737));
#69092=CARTESIAN_POINT('Ctrl Pts',(104.455001730451,-20.3522727910653,-32.5157376683266));
#69093=CARTESIAN_POINT('Ctrl Pts',(104.086176765824,-20.3519003213093,-32.1925987394747));
#69094=CARTESIAN_POINT('Ctrl Pts',(104.194269413732,-20.4059717963427,-32.2862963455132));
#69095=CARTESIAN_POINT('Ctrl Pts',(104.302362090344,-20.4600434514167,-32.3799937897523));
#69096=CARTESIAN_POINT('Ctrl Pts',(104.410455468833,-20.5141148642527,-32.4736905568142));
#69097=CARTESIAN_POINT('Ctrl Pts',(104.087867965647,-20.4203356511969,-32.1511364971909));
#69098=CARTESIAN_POINT('Ctrl Pts',(104.195955578133,-20.4744061366423,-32.244840470975));
#69099=CARTESIAN_POINT('Ctrl Pts',(104.304043604524,-20.5284765978807,-32.3385439651878));
#69100=CARTESIAN_POINT('Ctrl Pts',(104.412132034359,-20.5825470355882,-32.4322469920417));
#69101=CARTESIAN_POINT('',(104.624264068715,-20.209071743755,-32.4031390339881));
#69102=CARTESIAN_POINT('',(104.412132034359,-20.5825470355875,-32.4322469920405));
#69103=CARTESIAN_POINT('Origin',(104.624264068715,-20.4688793648903,-32.2531390339881));
#69104=CARTESIAN_POINT('',(104.087867965647,-20.4203356511961,-32.1511364971898));
#69105=CARTESIAN_POINT('Ctrl Pts',(104.412132034359,-20.5825470355882,-32.4322469920417));
#69106=CARTESIAN_POINT('Ctrl Pts',(104.304043604524,-20.5284765978807,-32.3385439651878));
#69107=CARTESIAN_POINT('Ctrl Pts',(104.195955578133,-20.4744061366423,-32.244840470975));
#69108=CARTESIAN_POINT('Ctrl Pts',(104.087867965647,-20.4203356511969,-32.1511364971909));
#69109=CARTESIAN_POINT('Origin',(104.300000000003,-20.3066037051655,-31.972069346513));
#69110=CARTESIAN_POINT('Ctrl Pts',(104.300000000003,-20.0467960840302,-32.122069346513));
#69111=CARTESIAN_POINT('Ctrl Pts',(104.408087612489,-20.100888175632,-32.2157595974551));
#69112=CARTESIAN_POINT('Ctrl Pts',(104.51617563888,-20.1549800604655,-32.3094494902639));
#69113=CARTESIAN_POINT('Ctrl Pts',(104.624264068715,-20.209071743755,-32.4031390339881));
#69114=CARTESIAN_POINT('Origin',(104.3,-20.3066037051641,-31.9720693465106));
#69115=CARTESIAN_POINT('Origin',(104.3,-20.3066037051641,-31.9720693465106));
#69116=CARTESIAN_POINT('Origin',(121.375735931288,0.,0.));
#69117=CARTESIAN_POINT('',(121.587867965644,-20.402627534524,-32.5457320875146));
#69118=CARTESIAN_POINT('',(121.587867965644,-22.0868894429017,-31.4270775313556));
#69119=CARTESIAN_POINT('Origin',(121.587867965644,2.22044604925031E-15,
-2.22044604925031E-15));
#69120=CARTESIAN_POINT('',(121.375735931288,-22.1374133253307,-31.4989671459791));
#69121=CARTESIAN_POINT('Origin',(121.375735931288,-21.9649140007177,-31.2535206487377));
#69122=CARTESIAN_POINT('',(121.375735931288,-20.6296297263933,-32.5064359373941));
#69123=CARTESIAN_POINT('Origin',(121.375735931288,0.,0.));
#69124=CARTESIAN_POINT('Ctrl Pts',(121.375735931288,-20.6296297263933,-32.5064359373941));
#69125=CARTESIAN_POINT('Ctrl Pts',(121.376552397245,-20.6289376637768,-32.5068751425889));
#69126=CARTESIAN_POINT('Ctrl Pts',(121.377368866524,-20.628243798337,-32.5073115132708));
#69127=CARTESIAN_POINT('Ctrl Pts',(121.414182867149,-20.5968767607222,-32.5268592442237));
#69128=CARTESIAN_POINT('Ctrl Pts',(121.45044439244,-20.5624817332895,-32.5405992451604));
#69129=CARTESIAN_POINT('Ctrl Pts',(121.523684543773,-20.4849771349203,-32.5555804302289));
#69130=CARTESIAN_POINT('Ctrl Pts',(121.558616909182,-20.4430854497869,-32.5548929712287));
#69131=CARTESIAN_POINT('Ctrl Pts',(121.587867965644,-20.402627534524,-32.5457320875146));
#69132=CARTESIAN_POINT('Origin',(113.,-20.468879364889,-32.2531390339859));
#69133=CARTESIAN_POINT('',(104.624264068712,-20.6296297263933,-32.5064359373941));
#69134=CARTESIAN_POINT('',(113.,-20.6296297263933,-32.5064359373941));
#69135=CARTESIAN_POINT('Origin',(104.624264068712,-20.468879364889,-32.2531390339859));
#69136=CARTESIAN_POINT('',(121.811388243054,-20.2090717437537,-32.4031390339859));
#69137=CARTESIAN_POINT('',(113.,-20.2090717437537,-32.4031390339859));
#69138=CARTESIAN_POINT('Ctrl Pts',(121.811388687965,-20.2090719660805,-32.4031394190667));
#69139=CARTESIAN_POINT('Ctrl Pts',(121.807962616872,-20.2107859993611,-32.4061082016325));
#69140=CARTESIAN_POINT('Ctrl Pts',(121.804557793907,-20.212539306832,-32.4090274474379));
#69141=CARTESIAN_POINT('Ctrl Pts',(121.765406035132,-20.233257916631,-32.4422479143698));
#69142=CARTESIAN_POINT('Ctrl Pts',(121.726559498935,-20.2594868158067,-32.4716751410544));
#69143=CARTESIAN_POINT('Ctrl Pts',(121.652509215907,-20.3238857140478,-32.5187625223814));
#69144=CARTESIAN_POINT('Ctrl Pts',(121.617288389766,-20.3619926475953,-32.5364820278348));
#69145=CARTESIAN_POINT('Ctrl Pts',(121.588030796123,-20.4024023990675,-32.5456810417724));
#69146=CARTESIAN_POINT('Ctrl Pts',(121.587949375966,-20.4025149337389,-32.5457065913245));
#69147=CARTESIAN_POINT('Ctrl Pts',(121.587867965644,-20.402627534524,-32.5457320875146));
#69148=CARTESIAN_POINT('Origin',(104.624264068712,-20.4688793648889,-32.2531390339859));
#69149=CARTESIAN_POINT('Origin',(104.624264068712,-20.4688793648889,-32.2531390339859));
#69150=CARTESIAN_POINT('Origin',(121.7,-4.10626375016942,-7.9796745175262));
#69151=CARTESIAN_POINT('',(121.7,-22.0053456777902,-30.8134083466537));
#69152=CARTESIAN_POINT('Origin',(121.7,-21.7673396757028,-30.9960367753563));
#69153=CARTESIAN_POINT('',(121.7,-21.1884328164397,-29.7487867783414));
#69154=CARTESIAN_POINT('Origin',(121.7,-20.7677983856497,-29.6934092049567));
#69155=CARTESIAN_POINT('',(121.7,-4.34426975225679,-7.79704608882358));
#69156=CARTESIAN_POINT('Ctrl Pts',(121.699999999997,-22.0053456777918,-30.8134083466558));
#69157=CARTESIAN_POINT('Ctrl Pts',(121.591912387512,-22.0712040357546,-30.8992366297665));
#69158=CARTESIAN_POINT('Ctrl Pts',(121.483824361121,-22.1370621419721,-30.9850645847965));
#69159=CARTESIAN_POINT('Ctrl Pts',(121.375735931288,-22.2029200028051,-31.0708922200351));
#69160=CARTESIAN_POINT('Ctrl Pts',(121.756617543138,-22.0397814876375,-30.858285967781));
#69161=CARTESIAN_POINT('Ctrl Pts',(121.648526737398,-22.1056379626004,-30.9441120388309));
#69162=CARTESIAN_POINT('Ctrl Pts',(121.540435642307,-22.1714946067171,-31.0299376087941));
#69163=CARTESIAN_POINT('Ctrl Pts',(121.432344074477,-22.2373506156865,-31.1157630683446));
#69164=CARTESIAN_POINT('Ctrl Pts',(121.869287779446,-22.0545660401896,-30.9888323340874));
#69165=CARTESIAN_POINT('Ctrl Pts',(121.761190886648,-22.120425351544,-31.0746492850224));
#69166=CARTESIAN_POINT('Ctrl Pts',(121.653093535148,-22.1862842375719,-31.1604659737814));
#69167=CARTESIAN_POINT('Ctrl Pts',(121.544995985491,-22.2521430321769,-31.2462824662224));
#69168=CARTESIAN_POINT('Ctrl Pts',(121.913823234176,-21.9537480036384,-31.1222783369417));
#69169=CARTESIAN_POINT('Ctrl Pts',(121.805730586268,-22.0196210464434,-31.2080903875002));
#69170=CARTESIAN_POINT('Ctrl Pts',(121.697637909658,-22.0854938708666,-31.2939025424768));
#69171=CARTESIAN_POINT('Ctrl Pts',(121.589544531169,-22.1513661623602,-31.37971421451));
#69172=CARTESIAN_POINT('Ctrl Pts',(121.912132034353,-21.8892528196841,-31.1696374243348));
#69173=CARTESIAN_POINT('Ctrl Pts',(121.804044421868,-21.9551321242177,-31.255450997464));
#69174=CARTESIAN_POINT('Ctrl Pts',(121.695956395477,-22.0210109949489,-31.341264364705));
#69175=CARTESIAN_POINT('Ctrl Pts',(121.587867965644,-22.0868894429017,-31.4270775313556));
#69176=CARTESIAN_POINT('',(121.375735931288,-22.2029200028051,-31.0708922200351));
#69177=CARTESIAN_POINT('Origin',(121.375735931288,-21.9649140007177,-31.2535206487377));
#69178=CARTESIAN_POINT('',(121.912132034353,-21.8892528196833,-31.1696374243337));
#69179=CARTESIAN_POINT('Ctrl Pts',(121.587867965644,-22.0868894429017,-31.4270775313556));
#69180=CARTESIAN_POINT('Ctrl Pts',(121.695956395477,-22.0210109949489,-31.341264364705));
#69181=CARTESIAN_POINT('Ctrl Pts',(121.804044421868,-21.9551321242177,-31.255450997464));
#69182=CARTESIAN_POINT('Ctrl Pts',(121.912132034353,-21.8892528196841,-31.1696374243348));
#69183=CARTESIAN_POINT('Origin',(121.699999999997,-21.7673396757045,-30.9960367753584));
#69184=CARTESIAN_POINT('Ctrl Pts',(121.699999999997,-22.0053456777918,-30.8134083466558));
#69185=CARTESIAN_POINT('Ctrl Pts',(121.591912387512,-22.0712040357546,-30.8992366297665));
#69186=CARTESIAN_POINT('Ctrl Pts',(121.483824361121,-22.1370621419721,-30.9850645847965));
#69187=CARTESIAN_POINT('Ctrl Pts',(121.375735931288,-22.2029200028051,-31.0708922200351));
#69188=CARTESIAN_POINT('Origin',(121.7,-21.7673396757028,-30.9960367753563));
#69189=CARTESIAN_POINT('Origin',(121.7,-21.7673396757028,-30.9960367753563));
#69190=CARTESIAN_POINT('Origin',(121.375735931288,-21.9649140007177,-31.2535206487377));
#69191=CARTESIAN_POINT('Origin',(121.375735931288,-21.9649140007177,-31.2535206487377));
#69192=CARTESIAN_POINT('Origin',(104.3,0.,0.));
#69193=CARTESIAN_POINT('',(104.087867965647,-21.8892528196833,-31.1696374243337));
#69194=CARTESIAN_POINT('Origin',(104.087867965644,-2.22044604925031E-15,
2.22044604925031E-15));
#69195=CARTESIAN_POINT('',(104.,-21.7673396757028,-30.9960367753563));
#69196=CARTESIAN_POINT('Origin',(104.3,-21.7673396757028,-30.9960367753563));
#69197=CARTESIAN_POINT('Origin',(104.,0.,0.));
#69198=CARTESIAN_POINT('Origin',(104.25,0.,0.));
#69199=CARTESIAN_POINT('',(104.412132034356,-22.0868894429017,-31.4270775313556));
#69200=CARTESIAN_POINT('Origin',(104.412132034356,2.22044604925031E-15,
-2.22044604925031E-15));
#69201=CARTESIAN_POINT('Ctrl Pts',(104.087867965647,-21.8892528196841,-31.1696374243348));
#69202=CARTESIAN_POINT('Ctrl Pts',(104.195955578132,-21.9551321242178,-31.255450997464));
#69203=CARTESIAN_POINT('Ctrl Pts',(104.304043604523,-22.0210109949489,-31.341264364705));
#69204=CARTESIAN_POINT('Ctrl Pts',(104.412132034356,-22.0868894429017,-31.4270775313556));
#69205=CARTESIAN_POINT('Origin',(104.624264068712,0.,0.));
#69206=CARTESIAN_POINT('',(104.624264068712,-22.1374133253307,-31.4989671459791));
#69207=CARTESIAN_POINT('Origin',(104.624264068712,0.,0.));
#69208=CARTESIAN_POINT('Origin',(104.624264068712,-21.9649140007177,-31.2535206487377));
#69209=CARTESIAN_POINT('Origin',(113.,0.,0.));
#69210=CARTESIAN_POINT('',(113.,-22.1374133253307,-31.4989671459791));
#69211=CARTESIAN_POINT('Origin',(113.,-21.9649140007177,-31.2535206487377));
#69212=CARTESIAN_POINT('',(104.624264068712,-22.2029200028051,-31.0708922200351));
#69213=CARTESIAN_POINT('',(113.,-22.2029200028051,-31.0708922200351));
#69214=CARTESIAN_POINT('Origin',(104.624264068712,-21.9649140007177,-31.2535206487377));
#69215=CARTESIAN_POINT('Origin',(113.,-21.9493846027006,-30.7404784537055));
#69216=CARTESIAN_POINT('',(104.3,-21.1884328164397,-29.7487867783414));
#69217=CARTESIAN_POINT('',(103.5,-21.1884328164397,-29.7487867783414));
#69218=CARTESIAN_POINT('',(104.300000000003,-22.0053456777918,-30.8134083466558));
#69219=CARTESIAN_POINT('',(104.3,-3.41779355863494,-6.58963880596225));
#69220=CARTESIAN_POINT('Ctrl Pts',(104.624264068712,-22.2029200028051,-31.0708922200351));
#69221=CARTESIAN_POINT('Ctrl Pts',(104.516175638879,-22.1370621419721,-30.9850645847965));
#69222=CARTESIAN_POINT('Ctrl Pts',(104.408087612488,-22.0712040357546,-30.8992366297665));
#69223=CARTESIAN_POINT('Ctrl Pts',(104.300000000003,-22.0053456777918,-30.8134083466558));
#69224=CARTESIAN_POINT('Origin',(104.3,-4.97801134479455,-2.7152696449976));
#69225=CARTESIAN_POINT('',(104.3,-27.6775213868948,-25.8390437558097));
#69226=CARTESIAN_POINT('',(104.,-27.8896534212507,-25.6269117214537));
#69227=CARTESIAN_POINT('Origin',(104.3,-27.8896534212507,-25.6269117214537));
#69228=CARTESIAN_POINT('',(104.,-26.7286363288515,-24.4658946290545));
#69229=CARTESIAN_POINT('',(104.,-4.97801134479455,-2.7152696449976));
#69230=CARTESIAN_POINT('',(104.3,-26.7286363288515,-24.8901586977665));
#69231=CARTESIAN_POINT('Origin',(104.3,-26.7286363288515,-24.4658946290545));
#69232=CARTESIAN_POINT('',(104.3,-4.76587931043859,-2.92740167935356));
#69233=CARTESIAN_POINT('Ctrl Pts',(104.300000000002,-27.6775213868965,-25.8390437558114));
#69234=CARTESIAN_POINT('Ctrl Pts',(104.408087612488,-27.7540191564569,-25.9155415253719));
#69235=CARTESIAN_POINT('Ctrl Pts',(104.51617563888,-27.8305166336028,-25.9920390025178));
#69236=CARTESIAN_POINT('Ctrl Pts',(104.624264068714,-27.9070138257223,-26.0685361946373));
#69237=CARTESIAN_POINT('Ctrl Pts',(104.243382456862,-27.7175202986166,-25.8790426675315));
#69238=CARTESIAN_POINT('Ctrl Pts',(104.351473262602,-27.7940161208215,-25.9555382814696));
#69239=CARTESIAN_POINT('Ctrl Pts',(104.459564357694,-27.8705114241477,-26.0320339977095));
#69240=CARTESIAN_POINT('Ctrl Pts',(104.567655925525,-27.947006700909,-26.108529069824));
#69241=CARTESIAN_POINT('Ctrl Pts',(104.130710113065,-27.8450194956664,-25.9107439897145));
#69242=CARTESIAN_POINT('Ctrl Pts',(104.238807005864,-27.9215059055569,-25.9872412253645));
#69243=CARTESIAN_POINT('Ctrl Pts',(104.346904358902,-27.9979921109243,-26.0637380030864));
#69244=CARTESIAN_POINT('Ctrl Pts',(104.455001908559,-28.0744781336927,-26.1402346665623));
#69245=CARTESIAN_POINT('Ctrl Pts',(104.086176765823,-27.9904837995326,-25.8282031306362));
#69246=CARTESIAN_POINT('Ctrl Pts',(104.194269413732,-28.0669635586561,-25.9047133406348));
#69247=CARTESIAN_POINT('Ctrl Pts',(104.302362090344,-28.1434434498089,-25.9812233477493));
#69248=CARTESIAN_POINT('Ctrl Pts',(104.410455468833,-28.2199229317112,-26.0577327634567));
#69249=CARTESIAN_POINT('Ctrl Pts',(104.087867965646,-28.045856034146,-25.7704413132657));
#69250=CARTESIAN_POINT('Ctrl Pts',(104.195955578132,-28.1223364854948,-25.8469579301585));
#69251=CARTESIAN_POINT('Ctrl Pts',(104.304043604524,-28.1988167893393,-25.9234740900862));
#69252=CARTESIAN_POINT('Ctrl Pts',(104.412132034358,-28.2752969494932,-25.9999898046701));
#69253=CARTESIAN_POINT('',(104.624264068714,-27.9070138257223,-26.0685361946373));
#69254=CARTESIAN_POINT('',(104.412132034358,-28.2752969494924,-25.9999898046693));
#69255=CARTESIAN_POINT('Origin',(104.624264068714,-28.1191458600783,-25.8564041602813));
#69256=CARTESIAN_POINT('',(104.087867965646,-28.0458560341451,-25.7704413132649));
#69257=CARTESIAN_POINT('Ctrl Pts',(104.412132034358,-28.2752969494932,-25.9999898046701));
#69258=CARTESIAN_POINT('Ctrl Pts',(104.304043604524,-28.1988167893393,-25.9234740900862));
#69259=CARTESIAN_POINT('Ctrl Pts',(104.195955578132,-28.1223364854948,-25.8469579301585));
#69260=CARTESIAN_POINT('Ctrl Pts',(104.087867965646,-28.045856034146,-25.7704413132657));
#69261=CARTESIAN_POINT('Origin',(104.300000000002,-27.8896534212524,-25.6269117214554));
#69262=CARTESIAN_POINT('Ctrl Pts',(104.300000000002,-27.6775213868965,-25.8390437558114));
#69263=CARTESIAN_POINT('Ctrl Pts',(104.408087612488,-27.7540191564569,-25.9155415253719));
#69264=CARTESIAN_POINT('Ctrl Pts',(104.51617563888,-27.8305166336028,-25.9920390025178));
#69265=CARTESIAN_POINT('Ctrl Pts',(104.624264068714,-27.9070138257223,-26.0685361946373));
#69266=CARTESIAN_POINT('Origin',(104.3,-27.8896534212507,-25.6269117214537));
#69267=CARTESIAN_POINT('Origin',(104.3,-27.8896534212507,-25.6269117214537));
#69268=CARTESIAN_POINT('Origin',(113.,-28.1191458600767,-25.8564041602797));
#69269=CARTESIAN_POINT('',(121.811388243054,-27.9070138257207,-26.0685361946357));
#69270=CARTESIAN_POINT('',(121.5,-28.3399768485066,-26.0594649259364));
#69271=CARTESIAN_POINT('Ctrl Pts',(121.811388687965,-27.9070141401383,-26.0685365090528));
#69272=CARTESIAN_POINT('Ctrl Pts',(121.80796264376,-27.9094381275961,-26.070960489325));
#69273=CARTESIAN_POINT('Ctrl Pts',(121.80455782351,-27.9118872463663,-26.0733264736922));
#69274=CARTESIAN_POINT('Ctrl Pts',(121.765406035132,-27.9404979978181,-26.1000526300669));
#69275=CARTESIAN_POINT('Ctrl Pts',(121.726559498935,-27.9734494956375,-26.1216886096789));
#69276=CARTESIAN_POINT('Ctrl Pts',(121.652509215907,-28.0478411657046,-26.1505038660466));
#69277=CARTESIAN_POINT('Ctrl Pts',(121.617288389766,-28.0892357824599,-26.1577567938406));
#69278=CARTESIAN_POINT('Ctrl Pts',(121.56412779323,-28.1644838415113,-26.1548982262092));
#69279=CARTESIAN_POINT('Ctrl Pts',(121.541159186122,-28.2029097568319,-26.1472690548682));
#69280=CARTESIAN_POINT('Ctrl Pts',(121.517077828304,-28.2581693569711,-26.123007172468));
#69281=CARTESIAN_POINT('Ctrl Pts',(121.510716614322,-28.2762278500349,-26.1128376379049));
#69282=CARTESIAN_POINT('Ctrl Pts',(121.502178291748,-28.3100940728715,-26.0887190628886));
#69283=CARTESIAN_POINT('Ctrl Pts',(121.5,-28.3259023098338,-26.0747711534923));
#69284=CARTESIAN_POINT('Ctrl Pts',(121.5,-28.3399768485066,-26.0594649259364));
#69285=CARTESIAN_POINT('',(104.624264068712,-28.3399768485066,-26.0594649259364));
#69286=CARTESIAN_POINT('',(113.,-28.3399768485066,-26.0594649259364));
#69287=CARTESIAN_POINT('Origin',(104.624264068712,-28.1191458600767,-25.8564041602797));
#69288=CARTESIAN_POINT('',(113.,-27.9070138257207,-26.0685361946357));
#69289=CARTESIAN_POINT('Origin',(104.624264068712,-28.1191458600766,-25.8564041602798));
#69290=CARTESIAN_POINT('Origin',(104.624264068712,-28.1191458600766,-25.8564041602798));
#69291=CARTESIAN_POINT('Origin',(104.,38.,0.));
#69292=CARTESIAN_POINT('Origin',(104.,0.,0.));
#69293=CARTESIAN_POINT('',(104.,1.6,36.2));
#69294=CARTESIAN_POINT('',(104.,19.,36.2));
#69295=CARTESIAN_POINT('',(104.,1.6,37.8419261182179));
#69296=CARTESIAN_POINT('',(104.,1.6,18.875));
#69297=CARTESIAN_POINT('',(104.,3.35305074428542,37.7270251019467));
#69298=CARTESIAN_POINT('Origin',(104.,0.,0.));
#69299=CARTESIAN_POINT('',(104.,3.13873638016778,36.099145889284));
#69300=CARTESIAN_POINT('',(104.,1.20107475020923,21.3811445944567));
#69301=CARTESIAN_POINT('',(104.,6.31135993656397,35.6814620741799));
#69302=CARTESIAN_POINT('',(104.,23.401343508112,33.431523053258));
#69303=CARTESIAN_POINT('',(104.,6.52567430068161,37.3093412868425));
#69304=CARTESIAN_POINT('',(104.,4.37369830660543,20.9634607793525));
#69305=CARTESIAN_POINT('',(104.,8.24872986069481,36.9666042262736));
#69306=CARTESIAN_POINT('Origin',(104.,0.,0.));
#69307=CARTESIAN_POINT('',(104.,7.82376811064875,35.3806253838283));
#69308=CARTESIAN_POINT('',(104.,4.61248681829541,23.3959604433702));
#69309=CARTESIAN_POINT('',(104.,10.624953006887,34.630050153031));
#69310=CARTESIAN_POINT('',(104.,27.0964907686634,30.2165149116643));
#69311=CARTESIAN_POINT('',(104.,11.0528894783935,36.2271308071048));
#69312=CARTESIAN_POINT('',(104.,7.4136717145337,22.6453852125729));
#69313=CARTESIAN_POINT('',(104.,13.2848331314657,35.4694880285264));
#69314=CARTESIAN_POINT('Origin',(104.,0.,0.));
#69315=CARTESIAN_POINT('',(104.,12.6520968593516,33.9419275389832));
#69316=CARTESIAN_POINT('',(104.,8.8045919723542,24.6532290594974));
#69317=CARTESIAN_POINT('',(104.,15.3313475036343,32.8321455851244));
#69318=CARTESIAN_POINT('',(104.,30.0706546728884,26.7269246556364));
#69319=CARTESIAN_POINT('',(104.,15.9596854262438,34.3490875196417));
#69320=CARTESIAN_POINT('',(104.,11.4838426166369,23.5434471056386));
#69321=CARTESIAN_POINT('',(104.,17.5353224130539,33.5720693465106));
#69322=CARTESIAN_POINT('Origin',(104.,0.,0.));
#69323=CARTESIAN_POINT('',(104.,16.7143593539449,32.1501196169967));
#69324=CARTESIAN_POINT('',(104.,12.8018593539449,25.3734708323834));
#69325=CARTESIAN_POINT('',(104.,19.4856406460551,30.5501196169967));
#69326=CARTESIAN_POINT('',(104.,32.35,23.1228782810445));
#69327=CARTESIAN_POINT('',(104.,20.3066037051641,31.9720693465106));
#69328=CARTESIAN_POINT('',(104.,15.5731406460551,23.7734708323834));
#69329=CARTESIAN_POINT('',(104.,21.7673396757028,30.9960367753563));
#69330=CARTESIAN_POINT('Origin',(104.,0.,0.));
#69331=CARTESIAN_POINT('',(104.,20.7677983856497,29.6934092049567));
#69332=CARTESIAN_POINT('',(104.,17.2622256995997,25.1248579341572));
#69333=CARTESIAN_POINT('',(104.,23.0685230724943,27.9280010608314));
#69334=CARTESIAN_POINT('',(104.,33.9959446585896,19.5430955687966));
#69335=CARTESIAN_POINT('',(104.,24.0750611261991,29.2397469911496));
#69336=CARTESIAN_POINT('',(104.,19.5629503864443,23.3594497900319));
#69337=CARTESIAN_POINT('',(104.,25.8471708459779,27.6856484770629));
#69338=CARTESIAN_POINT('Origin',(104.,0.,0.));
#69339=CARTESIAN_POINT('',(104.,24.6780266634105,26.5165042944955));
#69340=CARTESIAN_POINT('',(104.,21.9274016793536,23.7658793104386));
#69341=CARTESIAN_POINT('',(104.,26.7286363288515,24.4658946290545));
#69342=CARTESIAN_POINT('',(104.,35.097265478953,16.097265478953));
#69343=CARTESIAN_POINT('',(104.,27.8896534212507,25.6269117214538));
#69344=CARTESIAN_POINT('',(104.,23.9780113447946,21.7152696449976));
#69345=CARTESIAN_POINT('',(104.,29.0480002025284,24.3060703646348));
#69346=CARTESIAN_POINT('Origin',(104.,0.,0.));
#69347=CARTESIAN_POINT('',(104.,27.7453726321288,23.3065290745817));
#69348=CARTESIAN_POINT('',(104.,25.9593069400571,21.9360326667517));
#69349=CARTESIAN_POINT('',(104.,29.6934092049567,20.7677983856497));
#69350=CARTESIAN_POINT('',(104.,35.7606099900688,12.8608683803695));
#69351=CARTESIAN_POINT('',(104.,30.9960367753563,21.7673396757028));
#69352=CARTESIAN_POINT('',(104.,27.907343512885,19.3973019778198));
#69353=CARTESIAN_POINT('',(104.,31.9720693465106,20.3066037051641));
#69354=CARTESIAN_POINT('Origin',(104.,0.,0.));
#69355=CARTESIAN_POINT('',(104.,30.5501196169967,19.4856406460551));
#69356=CARTESIAN_POINT('',(104.,29.7962294964313,19.0503819820073));
#69357=CARTESIAN_POINT('',(104.,32.0001196169967,16.9741669750802));
#69358=CARTESIAN_POINT('',(104.,36.1001196169967,9.87275866404783));
#69359=CARTESIAN_POINT('',(104.,33.4320229585134,17.8008767547584));
#69360=CARTESIAN_POINT('',(104.,31.2462294964313,16.5389083110324));
#69361=CARTESIAN_POINT('',(104.,34.4745111043772,15.686919915995));
#69362=CARTESIAN_POINT('Origin',(104.,0.,0.));
#69363=CARTESIAN_POINT('',(104.,32.946950614834,15.0541836438809));
#69364=CARTESIAN_POINT('',(104.,33.1582521353481,15.1417075994279));
#69365=CARTESIAN_POINT('',(104.,34.0567325686927,12.3749329995982));
#69366=CARTESIAN_POINT('',(104.,36.2269246556364,7.13562583034405));
#69367=CARTESIAN_POINT('',(104.,35.57367450321,13.0032709222077));
#69368=CARTESIAN_POINT('',(104.,34.2680340892069,12.4624569551452));
#69369=CARTESIAN_POINT('',(104.,36.2271308071048,11.0528894783935));
#69370=CARTESIAN_POINT('Origin',(104.,0.,0.));
#69371=CARTESIAN_POINT('',(104.,34.630050153031,10.624953006887));
#69372=CARTESIAN_POINT('',(104.,35.622626548525,10.8909130504859));
#69373=CARTESIAN_POINT('',(104.,35.3806253838283,7.82376811064874));
#69374=CARTESIAN_POINT('',(104.,36.2392735757121,4.61924943271125));
#69375=CARTESIAN_POINT('',(104.,36.9666042262736,8.2487298606948));
#69376=CARTESIAN_POINT('',(104.,36.3732017793224,8.08972815424757));
#69377=CARTESIAN_POINT('',(104.,37.3598942576647,6.22974103737677));
#69378=CARTESIAN_POINT('Origin',(104.,0.,0.));
#69379=CARTESIAN_POINT('',(104.,35.7206199318459,6.01392647815182));
#69380=CARTESIAN_POINT('',(104.,37.2201330582908,6.21134112641337));
#69381=CARTESIAN_POINT('',(104.,36.099145889284,3.13873638016777));
#69382=CARTESIAN_POINT('',(104.,36.2140086319858,2.26626722989192));
#69383=CARTESIAN_POINT('',(104.,37.7270251019467,3.35305074428541));
#69384=CARTESIAN_POINT('',(104.,37.5986590157289,3.33615102842932));
#69385=CARTESIAN_POINT('',(104.,37.8534195593564,1.3));
#69386=CARTESIAN_POINT('Origin',(104.,0.,0.));
#69387=CARTESIAN_POINT('',(104.,36.2,1.3));
#69388=CARTESIAN_POINT('',(104.,37.875,1.3));
#69389=CARTESIAN_POINT('',(104.,36.2,-1.6));
#69390=CARTESIAN_POINT('',(104.,36.2,0.));
#69391=CARTESIAN_POINT('',(104.,37.8419261182179,-1.6));
#69392=CARTESIAN_POINT('',(104.,37.875,-1.6));
#69393=CARTESIAN_POINT('',(104.,37.7270251019467,-3.35305074428545));
#69394=CARTESIAN_POINT('Origin',(104.,0.,0.));
#69395=CARTESIAN_POINT('',(104.,36.099145889284,-3.13873638016781));
#69396=CARTESIAN_POINT('',(104.,37.5986590157289,-3.33615102842936));
#69397=CARTESIAN_POINT('',(104.,35.7206199318459,-6.01392647815186));
#69398=CARTESIAN_POINT('',(104.,36.2140086319858,-2.26626722989194));
#69399=CARTESIAN_POINT('',(104.,37.3598942576647,-6.22974103737681));
#69400=CARTESIAN_POINT('',(104.,37.2201330582907,-6.21134112641341));
#69401=CARTESIAN_POINT('',(104.,36.9000603243714,-8.54148233004195));
#69402=CARTESIAN_POINT('Origin',(104.,0.,0.));
#69403=CARTESIAN_POINT('',(104.,35.3029796702975,-8.11354585853549));
#69404=CARTESIAN_POINT('',(104.,36.2955560657916,-8.37950590213432));
#69405=CARTESIAN_POINT('',(104.,34.630050153031,-10.6249530068871));
#69406=CARTESIAN_POINT('',(104.,36.2392735757121,-4.61924943271127));
#69407=CARTESIAN_POINT('',(104.,36.2271308071048,-11.0528894783935));
#69408=CARTESIAN_POINT('',(104.,35.622626548525,-10.8909130504859));
#69409=CARTESIAN_POINT('',(104.,35.4694880285264,-13.2848331314657));
#69410=CARTESIAN_POINT('Origin',(104.,0.,0.));
#69411=CARTESIAN_POINT('',(104.,33.9419275389832,-12.6520968593516));
#69412=CARTESIAN_POINT('',(104.,34.1532290594973,-12.7396208148986));
#69413=CARTESIAN_POINT('',(104.,32.8321455851244,-15.3313475036343));
#69414=CARTESIAN_POINT('',(104.,36.2269246556364,-7.13562583034406));
#69415=CARTESIAN_POINT('',(104.,34.3490875196417,-15.9596854262439));
#69416=CARTESIAN_POINT('',(104.,33.0434471056386,-15.4188714591814));
#69417=CARTESIAN_POINT('',(104.,33.5720693465106,-17.5353224130539));
#69418=CARTESIAN_POINT('Origin',(104.,0.,0.));
#69419=CARTESIAN_POINT('',(104.,32.1501196169967,-16.7143593539449));
#69420=CARTESIAN_POINT('',(104.,31.3962294964313,-16.2791006898971));
#69421=CARTESIAN_POINT('',(104.,30.5501196169967,-19.4856406460551));
#69422=CARTESIAN_POINT('',(104.,36.1001196169967,-9.87275866404784));
#69423=CARTESIAN_POINT('',(104.,31.9720693465106,-20.3066037051641));
#69424=CARTESIAN_POINT('',(104.,29.7962294964313,-19.0503819820073));
#69425=CARTESIAN_POINT('',(104.,30.9960367753563,-21.7673396757028));
#69426=CARTESIAN_POINT('Origin',(104.,0.,0.));
#69427=CARTESIAN_POINT('',(104.,29.6934092049567,-20.7677983856497));
#69428=CARTESIAN_POINT('',(104.,27.907343512885,-19.3973019778198));
#69429=CARTESIAN_POINT('',(104.,27.9280010608314,-23.0685230724943));
#69430=CARTESIAN_POINT('',(104.,35.7606099900688,-12.8608683803695));
#69431=CARTESIAN_POINT('',(104.,29.2397469911496,-24.0750611261991));
#69432=CARTESIAN_POINT('',(104.,26.1419353687597,-21.6980266646644));
#69433=CARTESIAN_POINT('',(104.,27.6856484770629,-25.8471708459779));
#69434=CARTESIAN_POINT('Origin',(104.,0.,0.));
#69435=CARTESIAN_POINT('',(104.,26.5165042944955,-24.6780266634105));
#69436=CARTESIAN_POINT('',(104.,23.7658793104386,-21.9274016793536));
#69437=CARTESIAN_POINT('',(104.,35.097265478953,-16.097265478953));
#69438=CARTESIAN_POINT('',(104.,23.3065290745816,-27.7453726321288));
#69439=CARTESIAN_POINT('',(104.,19.8009563885316,-23.1768213613293));
#69440=CARTESIAN_POINT('',(104.,20.7677983856497,-29.6934092049567));
#69441=CARTESIAN_POINT('',(104.,33.9959446585896,-19.5430955687966));
#69442=CARTESIAN_POINT('',(104.,21.7673396757028,-30.9960367753563));
#69443=CARTESIAN_POINT('',(104.,17.2622256995996,-25.1248579341572));
#69444=CARTESIAN_POINT('',(104.,20.3066037051641,-31.9720693465106));
#69445=CARTESIAN_POINT('Origin',(104.,0.,0.));
#69446=CARTESIAN_POINT('',(104.,19.4856406460551,-30.5501196169967));
#69447=CARTESIAN_POINT('',(104.,15.5731406460551,-23.7734708323834));
#69448=CARTESIAN_POINT('',(104.,16.9741669750802,-32.0001196169967));
#69449=CARTESIAN_POINT('',(104.,32.35,-23.1228782810445));
#69450=CARTESIAN_POINT('',(104.,17.8008767547584,-33.4320229585134));
#69451=CARTESIAN_POINT('',(104.,13.0616669750802,-25.2234708323834));
#69452=CARTESIAN_POINT('',(104.,15.686919915995,-34.4745111043772));
#69453=CARTESIAN_POINT('Origin',(104.,0.,0.));
#69454=CARTESIAN_POINT('',(104.,15.0541836438809,-32.946950614834));
#69455=CARTESIAN_POINT('',(104.,11.2066787568835,-23.6582521353481));
#69456=CARTESIAN_POINT('',(104.,12.3749329995982,-34.0567325686927));
#69457=CARTESIAN_POINT('',(104.,30.0706546728884,-26.7269246556364));
#69458=CARTESIAN_POINT('',(104.,13.0032709222077,-35.57367450321));
#69459=CARTESIAN_POINT('',(104.,8.52742811260079,-24.7680340892069));
#69460=CARTESIAN_POINT('',(104.,11.3396925048198,-36.1383832819455));
#69461=CARTESIAN_POINT('Origin',(104.,0.,0.));
#69462=CARTESIAN_POINT('',(104.,10.9147307547737,-34.5524044395002));
#69463=CARTESIAN_POINT('',(104.,7.70344946242041,-22.5677394990421));
#69464=CARTESIAN_POINT('',(104.,7.82376811064873,-35.3806253838283));
#69465=CARTESIAN_POINT('',(104.,27.0964907686634,-30.2165149116643));
#69466=CARTESIAN_POINT('',(104.,8.24872986069478,-36.9666042262736));
#69467=CARTESIAN_POINT('',(104.,4.61248681829539,-23.3959604433702));
#69468=CARTESIAN_POINT('',(104.,6.52567430068159,-37.3093412868425));
#69469=CARTESIAN_POINT('Origin',(104.,0.,0.));
#69470=CARTESIAN_POINT('',(104.,6.31135993656395,-35.6814620741799));
#69471=CARTESIAN_POINT('',(104.,4.37369830660541,-20.9634607793525));
#69472=CARTESIAN_POINT('',(104.,23.401343508112,-33.431523053258));
#69473=CARTESIAN_POINT('Origin',(104.,0.,0.));
#69474=CARTESIAN_POINT('',(104.,-1.60000000000001,-36.2));
#69475=CARTESIAN_POINT('',(104.,19.,-36.2));
#69476=CARTESIAN_POINT('',(104.,-1.60000000000001,-37.8419261182179));
#69477=CARTESIAN_POINT('',(104.,-1.6,-18.875));
#69478=CARTESIAN_POINT('',(104.,-3.35305074428544,-37.7270251019467));
#69479=CARTESIAN_POINT('Origin',(104.,0.,0.));
#69480=CARTESIAN_POINT('',(104.,-3.1387363801678,-36.099145889284));
#69481=CARTESIAN_POINT('',(104.,-0.553665449701535,-16.4635827375088));
#69482=CARTESIAN_POINT('',(104.,-6.311359936564,-35.6814620741798));
#69483=CARTESIAN_POINT('',(104.,13.9512471913802,-38.3490849102059));
#69484=CARTESIAN_POINT('',(104.,-6.52567430068164,-37.3093412868425));
#69485=CARTESIAN_POINT('',(104.,-3.72628900609773,-16.0458989224046));
#69486=CARTESIAN_POINT('',(104.,-8.24872986069483,-36.9666042262736));
#69487=CARTESIAN_POINT('Origin',(104.,0.,0.));
#69488=CARTESIAN_POINT('',(104.,-7.82376811064877,-35.3806253838283));
#69489=CARTESIAN_POINT('',(104.,-2.06696949019975,-13.8959604433702));
#69490=CARTESIAN_POINT('',(104.,-10.6249530068871,-34.630050153031));
#69491=CARTESIAN_POINT('',(104.,8.35799190324088,-39.7165149116643));
#69492=CARTESIAN_POINT('',(104.,-11.0528894783935,-36.2271308071048));
#69493=CARTESIAN_POINT('',(104.,-4.86815438643804,-13.1453852125729));
#69494=CARTESIAN_POINT('',(104.,-13.2848331314657,-35.4694880285264));
#69495=CARTESIAN_POINT('Origin',(104.,0.,0.));
#69496=CARTESIAN_POINT('',(104.,-12.6520968593516,-33.9419275389832));
#69497=CARTESIAN_POINT('',(104.,-3.2396208148986,-11.2182002169529));
#69498=CARTESIAN_POINT('',(104.,-15.3313475036343,-32.8321455851244));
#69499=CARTESIAN_POINT('',(104.,2.36437416965592,-40.1619534981808));
#69500=CARTESIAN_POINT('',(104.,-15.9596854262439,-34.3490875196417));
#69501=CARTESIAN_POINT('',(104.,-5.91887145918133,-10.1084182630942));
#69502=CARTESIAN_POINT('',(104.,-17.5353224130539,-33.5720693465106));
#69503=CARTESIAN_POINT('Origin',(104.,0.,0.));
#69504=CARTESIAN_POINT('',(104.,-16.7143593539449,-32.1501196169967));
#69505=CARTESIAN_POINT('',(104.,-3.3018593539449,-8.9189881604791));
#69506=CARTESIAN_POINT('',(104.,-3.85000000000002,-39.5773609529488));
#69507=CARTESIAN_POINT('',(104.,-20.7677983856497,-29.6934092049567));
#69508=CARTESIAN_POINT('',(104.,-3.17978755654757,-6.77226723466486));
#69509=CARTESIAN_POINT('',(104.,-23.0685230724943,-27.9280010608314));
#69510=CARTESIAN_POINT('',(104.,-10.0783828016418,-37.8956862682889));
#69511=CARTESIAN_POINT('',(104.,-24.0750611261991,-29.2397469911496));
#69512=CARTESIAN_POINT('',(104.,-5.48051224339215,-5.00685909053957));
#69513=CARTESIAN_POINT('',(104.,-25.8471708459779,-27.6856484770629));
#69514=CARTESIAN_POINT('Origin',(104.,0.,0.));
#69515=CARTESIAN_POINT('',(104.,-24.6780266634105,-26.5165042944955));
#69516=CARTESIAN_POINT('',(104.,-2.92740167935357,-4.76587931043859));
#69517=CARTESIAN_POINT('',(104.,-16.097265478953,-35.097265478953));
#69518=CARTESIAN_POINT('',(104.,-29.0480002025284,-24.3060703646347));
#69519=CARTESIAN_POINT('Origin',(104.,0.,0.));
#69520=CARTESIAN_POINT('',(104.,-27.7453726321288,-23.3065290745817));
#69521=CARTESIAN_POINT('',(104.,-2.04174508310916,-3.58344196725942));
#69522=CARTESIAN_POINT('',(104.,-29.6934092049567,-20.7677983856497));
#69523=CARTESIAN_POINT('',(104.,-21.6781718470167,-31.2134590798618));
#69524=CARTESIAN_POINT('',(104.,-30.9960367753563,-21.7673396757028));
#69525=CARTESIAN_POINT('',(104.,-3.98978165593707,-1.04471127832747));
#69526=CARTESIAN_POINT('',(104.,-31.9720693465106,-20.3066037051641));
#69527=CARTESIAN_POINT('Origin',(104.,0.,0.));
#69528=CARTESIAN_POINT('',(104.,-30.5501196169967,-19.4856406460551));
#69529=CARTESIAN_POINT('',(104.,-1.29622949643128,-2.59589931010293));
#69530=CARTESIAN_POINT('',(104.,-32.0001196169967,-16.9741669750802));
#69531=CARTESIAN_POINT('',(104.,-26.6001196169967,-26.3272413359522));
#69532=CARTESIAN_POINT('',(104.,-33.4320229585134,-17.8008767547584));
#69533=CARTESIAN_POINT('',(104.,-2.74622949643128,-0.0844256391280573));
#69534=CARTESIAN_POINT('',(104.,-34.4745111043772,-15.686919915995));
#69535=CARTESIAN_POINT('Origin',(104.,0.,0.));
#69536=CARTESIAN_POINT('',(104.,-32.946950614834,-15.0541836438809));
#69537=CARTESIAN_POINT('',(104.,-0.723223292803717,-1.70667875688354));
#69538=CARTESIAN_POINT('',(104.,-34.0567325686927,-12.3749329995982));
#69539=CARTESIAN_POINT('',(104.,-30.6619534981808,-20.5706546728884));
#69540=CARTESIAN_POINT('',(104.,-35.57367450321,-13.0032709222077));
#69541=CARTESIAN_POINT('',(104.,-1.83300524666248,0.972571887399195));
#69542=CARTESIAN_POINT('',(104.,-36.1383832819455,-11.3396925048198));
#69543=CARTESIAN_POINT('Origin',(104.,0.,0.));
#69544=CARTESIAN_POINT('',(104.,-34.5524044395002,-10.9147307547737));
#69545=CARTESIAN_POINT('',(104.,-0.0904981630899659,-1.68069079837259));
#69546=CARTESIAN_POINT('',(104.,-35.3806253838283,-7.82376811064873));
#69547=CARTESIAN_POINT('',(104.,-33.6937562476164,-14.1192494327112));
#69548=CARTESIAN_POINT('',(104.,-36.9666042262736,-8.24872986069479));
#69549=CARTESIAN_POINT('',(104.,-0.918719107418027,1.41027184575243));
#69550=CARTESIAN_POINT('',(104.,-37.3093412868425,-6.52567430068159));
#69551=CARTESIAN_POINT('Origin',(104.,0.,0.));
#69552=CARTESIAN_POINT('',(104.,-35.6814620741799,-6.31135993656395));
#69553=CARTESIAN_POINT('',(104.,0.171615498867558,-1.59121272787762));
#69554=CARTESIAN_POINT('',(104.,-35.5665993314781,-7.1838290868398));
#69555=CARTESIAN_POINT('Origin',(104.,0.,0.));
#69556=CARTESIAN_POINT('',(104.,-36.2,1.6));
#69557=CARTESIAN_POINT('',(104.,-36.2,6.76005033129339E-15));
#69558=CARTESIAN_POINT('',(104.,-37.8419261182179,1.6));
#69559=CARTESIAN_POINT('',(104.,0.125,1.6));
#69560=CARTESIAN_POINT('',(104.,-37.7270251019467,3.35305074428542));
#69561=CARTESIAN_POINT('Origin',(104.,0.,0.));
#69562=CARTESIAN_POINT('',(104.,-36.099145889284,3.13873638016779));
#69563=CARTESIAN_POINT('',(104.,-0.24606831623661,-1.58141082851857));
#69564=CARTESIAN_POINT('',(104.,-35.6814620741799,6.31135993656398));
#69565=CARTESIAN_POINT('',(104.,-35.5665993314781,7.18382908683984));
#69566=CARTESIAN_POINT('',(104.,-37.3093412868425,6.52567430068162));
#69567=CARTESIAN_POINT('',(104.,0.171615498867559,1.59121272787762));
#69568=CARTESIAN_POINT('',(104.,-36.9666042262736,8.24872986069481));
#69569=CARTESIAN_POINT('Origin',(104.,0.,0.));
#69570=CARTESIAN_POINT('',(104.,-35.3806253838283,7.82376811064875));
#69571=CARTESIAN_POINT('',(104.,-0.918719107418034,-1.41027184575243));
#69572=CARTESIAN_POINT('',(104.,-34.630050153031,10.624953006887));
#69573=CARTESIAN_POINT('',(104.,-33.6937562476164,14.1192494327113));
#69574=CARTESIAN_POINT('',(104.,-36.2271308071048,11.0528894783935));
#69575=CARTESIAN_POINT('',(104.,-0.16814387662072,1.39091305048587));
#69576=CARTESIAN_POINT('',(104.,-35.4694880285264,13.2848331314657));
#69577=CARTESIAN_POINT('Origin',(104.,0.,0.));
#69578=CARTESIAN_POINT('',(104.,-33.9419275389832,12.6520968593516));
#69579=CARTESIAN_POINT('',(104.,-1.71820021695296,-0.695408027645805));
#69580=CARTESIAN_POINT('',(104.,-32.8321455851244,15.3313475036343));
#69581=CARTESIAN_POINT('',(104.,-30.6619534981808,20.5706546728885));
#69582=CARTESIAN_POINT('',(104.,-34.3490875196417,15.9596854262438));
#69583=CARTESIAN_POINT('',(104.,-0.608418263094196,1.98384261663693));
#69584=CARTESIAN_POINT('',(104.,-33.5720693465106,17.5353224130539));
#69585=CARTESIAN_POINT('Origin',(104.,0.,0.));
#69586=CARTESIAN_POINT('',(104.,-32.1501196169967,16.7143593539449));
#69587=CARTESIAN_POINT('',(104.,-2.89622949643128,-0.175381982007262));
#69588=CARTESIAN_POINT('',(104.,-30.5501196169967,19.4856406460551));
#69589=CARTESIAN_POINT('',(104.,-26.6001196169967,26.3272413359522));
#69590=CARTESIAN_POINT('',(104.,-31.9720693465106,20.3066037051641));
#69591=CARTESIAN_POINT('',(104.,-1.29622949643128,2.59589931010294));
#69592=CARTESIAN_POINT('',(104.,-30.9960367753563,21.7673396757028));
#69593=CARTESIAN_POINT('Origin',(104.,0.,0.));
#69594=CARTESIAN_POINT('',(104.,-29.6934092049567,20.7677983856497));
#69595=CARTESIAN_POINT('',(104.,-3.98978165593707,1.04471127832749));
#69596=CARTESIAN_POINT('',(104.,-27.9280010608314,23.0685230724943));
#69597=CARTESIAN_POINT('',(104.,-21.6781718470166,31.2134590798618));
#69598=CARTESIAN_POINT('',(104.,-29.2397469911496,24.0750611261991));
#69599=CARTESIAN_POINT('',(104.,-2.22437351181178,3.34543596517206));
#69600=CARTESIAN_POINT('',(104.,-27.6856484770629,25.8471708459779));
#69601=CARTESIAN_POINT('Origin',(104.,0.,0.));
#69602=CARTESIAN_POINT('',(104.,-26.5165042944955,24.6780266634105));
#69603=CARTESIAN_POINT('',(104.,-4.7658793104386,2.92740167935357));
#69604=CARTESIAN_POINT('',(104.,-24.4658946290545,26.7286363288515));
#69605=CARTESIAN_POINT('',(104.,-16.097265478953,35.097265478953));
#69606=CARTESIAN_POINT('',(104.,-25.6269117214538,27.8896534212507));
#69607=CARTESIAN_POINT('',(104.,-2.71526964499761,4.97801134479456));
#69608=CARTESIAN_POINT('',(104.,-24.3060703646347,29.0480002025284));
#69609=CARTESIAN_POINT('Origin',(104.,0.,0.));
#69610=CARTESIAN_POINT('',(104.,-23.3065290745816,27.7453726321288));
#69611=CARTESIAN_POINT('',(104.,-5.71851824547952,4.82423066183697));
#69612=CARTESIAN_POINT('',(104.,-20.7677983856497,29.6934092049567));
#69613=CARTESIAN_POINT('',(104.,-10.0783828016417,37.8956862682889));
#69614=CARTESIAN_POINT('',(104.,-21.7673396757028,30.9960367753563));
#69615=CARTESIAN_POINT('',(104.,-3.17978755654757,6.77226723466488));
#69616=CARTESIAN_POINT('',(104.,-20.3066037051641,31.9720693465106));
#69617=CARTESIAN_POINT('Origin',(104.,0.,0.));
#69618=CARTESIAN_POINT('',(104.,-19.4856406460551,30.5501196169967));
#69619=CARTESIAN_POINT('',(104.,-6.0731406460551,7.31898816047912));
#69620=CARTESIAN_POINT('',(104.,-16.9741669750802,32.0001196169967));
#69621=CARTESIAN_POINT('',(104.,-3.84999999999999,39.5773609529488));
#69622=CARTESIAN_POINT('',(104.,-17.8008767547584,33.4320229585134));
#69623=CARTESIAN_POINT('',(104.,-3.56166697508023,8.76898816047912));
#69624=CARTESIAN_POINT('',(104.,-15.686919915995,34.4745111043772));
#69625=CARTESIAN_POINT('Origin',(104.,0.,0.));
#69626=CARTESIAN_POINT('',(104.,-15.0541836438809,32.946950614834));
#69627=CARTESIAN_POINT('',(104.,-5.64170759942794,10.2232232928037));
#69628=CARTESIAN_POINT('',(104.,-12.3749329995982,34.0567325686927));
#69629=CARTESIAN_POINT('',(104.,2.36437416965597,40.1619534981808));
#69630=CARTESIAN_POINT('',(104.,-13.0032709222077,35.57367450321));
#69631=CARTESIAN_POINT('',(104.,-2.96245695514521,11.3330052466625));
#69632=CARTESIAN_POINT('',(104.,-11.3396925048198,36.1383832819455));
#69633=CARTESIAN_POINT('Origin',(104.,0.,0.));
#69634=CARTESIAN_POINT('',(104.,-10.9147307547738,34.5524044395002));
#69635=CARTESIAN_POINT('',(104.,-5.15793213432475,13.0677394990421));
#69636=CARTESIAN_POINT('',(104.,-7.82376811064874,35.3806253838283));
#69637=CARTESIAN_POINT('',(104.,8.35799190324092,39.7165149116643));
#69638=CARTESIAN_POINT('',(104.,-8.24872986069479,36.9666042262736));
#69639=CARTESIAN_POINT('',(104.,-2.06696949019973,13.8959604433702));
#69640=CARTESIAN_POINT('',(104.,-6.52567430068159,37.3093412868425));
#69641=CARTESIAN_POINT('Origin',(104.,0.,0.));
#69642=CARTESIAN_POINT('',(104.,-6.31135993656396,35.6814620741799));
#69643=CARTESIAN_POINT('',(104.,-3.72628900609772,16.0458989224046));
#69644=CARTESIAN_POINT('',(104.,13.9512471913803,38.3490849102059));
#69645=CARTESIAN_POINT('',(104.,-4.07807384116069E-15,33.3));
#69646=CARTESIAN_POINT('Origin',(104.,0.,0.));
#69647=CARTESIAN_POINT('Origin',(104.3,0.,0.));
#69648=CARTESIAN_POINT('',(104.087867965647,-29.2106904110607,-24.442202271432));
#69649=CARTESIAN_POINT('Origin',(104.087867965644,0.,2.22044604925031E-15));
#69650=CARTESIAN_POINT('Origin',(104.3,-29.0480002025284,-24.3060703646347));
#69651=CARTESIAN_POINT('Origin',(104.25,0.,0.));
#69652=CARTESIAN_POINT('',(104.412132034356,-29.4682231323184,-24.6397181974285));
#69653=CARTESIAN_POINT('Origin',(104.412132034356,-2.22044604925031E-15,
2.22044604925031E-15));
#69654=CARTESIAN_POINT('Ctrl Pts',(104.087867965647,-29.2106904110617,-24.4422022714329));
#69655=CARTESIAN_POINT('Ctrl Pts',(104.195955578132,-29.2965351197829,-24.5080409992732));
#69656=CARTESIAN_POINT('Ctrl Pts',(104.304043604523,-29.3823793561953,-24.5738796405169));
#69657=CARTESIAN_POINT('Ctrl Pts',(104.412132034356,-29.4682231323184,-24.6397181974285));
#69658=CARTESIAN_POINT('Origin',(104.624264068712,0.,0.));
#69659=CARTESIAN_POINT('',(104.624264068712,-29.5356318566107,-24.6960816898302));
#69660=CARTESIAN_POINT('Origin',(104.624264068712,0.,0.));
#69661=CARTESIAN_POINT('Origin',(104.624264068712,-29.3054840759098,-24.5036446896497));
#69662=CARTESIAN_POINT('Origin',(113.,0.,0.));
#69663=CARTESIAN_POINT('',(121.5,-29.5356318566107,-24.6960816898302));
#69664=CARTESIAN_POINT('Origin',(121.5,0.,0.));
#69665=CARTESIAN_POINT('',(113.,-29.5356318566107,-24.6960816898302));
#69666=CARTESIAN_POINT('Origin',(104.3,0.171615498867559,1.59121272787762));
#69667=CARTESIAN_POINT('',(104.3,-37.3484991445085,6.22824084226948));
#69668=CARTESIAN_POINT('Origin',(104.3,-37.3093412868425,6.52567430068162));
#69669=CARTESIAN_POINT('',(104.3,-36.018053390258,6.05308433581785));
#69670=CARTESIAN_POINT('Origin',(104.3,-35.6814620741799,6.31135993656398));
#69671=CARTESIAN_POINT('',(104.3,0.132457641201544,1.29377926946548));
#69672=CARTESIAN_POINT('Ctrl Pts',(104.300000000005,-37.3484991445135,6.22824084227013));
#69673=CARTESIAN_POINT('Ctrl Pts',(104.408087612491,-37.4557577970327,6.24236171176215));
#69674=CARTESIAN_POINT('Ctrl Pts',(104.516175638883,-37.5630160395531,6.25648252727679));
#69675=CARTESIAN_POINT('Ctrl Pts',(104.624264068717,-37.6702738824338,6.27060329017787));
#69676=CARTESIAN_POINT('Ctrl Pts',(104.243382456865,-37.4045822093922,6.23562431783377));
#69677=CARTESIAN_POINT('Ctrl Pts',(104.351473262605,-37.5118379662662,6.24974495464449));
#69678=CARTESIAN_POINT('Ctrl Pts',(104.459564357697,-37.6190934884284,6.26386511752372));
#69679=CARTESIAN_POINT('Ctrl Pts',(104.567655925528,-37.7263484833998,6.27798565144626));
#69680=CARTESIAN_POINT('Ctrl Pts',(104.130708651008,-37.5073508627116,6.31747589142947));
#69681=CARTESIAN_POINT('Ctrl Pts',(104.238805543807,-37.6146021763222,6.33158807371345));
#69682=CARTESIAN_POINT('Ctrl Pts',(104.346902897911,-37.7218530009717,6.34570037330175));
#69683=CARTESIAN_POINT('Ctrl Pts',(104.455000447568,-37.829103624981,6.35981259677859));
#69684=CARTESIAN_POINT('Ctrl Pts',(104.086176765826,-37.5304181438623,6.48312997219362));
#69685=CARTESIAN_POINT('Ctrl Pts',(104.194269413735,-37.6376757019853,6.49722897978643));
#69686=CARTESIAN_POINT('Ctrl Pts',(104.302362090346,-37.7449331795239,6.5113282156331));
#69687=CARTESIAN_POINT('Ctrl Pts',(104.410455468835,-37.8521899387317,6.52542748682538));
#69688=CARTESIAN_POINT('Ctrl Pts',(104.087867965649,-37.5183010937808,6.5622228859681));
#69689=CARTESIAN_POINT('Ctrl Pts',(104.195955578135,-37.6255641562347,6.57631854247011));
#69690=CARTESIAN_POINT('Ctrl Pts',(104.304043604527,-37.732826766359,6.59041436013179));
#69691=CARTESIAN_POINT('Ctrl Pts',(104.412132034361,-37.8400889356949,6.60451033490422));
#69692=CARTESIAN_POINT('',(104.624264068717,-37.6702738824338,6.27060329017787));
#69693=CARTESIAN_POINT('',(104.412132034361,-37.8400889356926,6.60451033490381));
#69694=CARTESIAN_POINT('Origin',(104.624264068717,-37.6311160247677,6.56803674859001));
#69695=CARTESIAN_POINT('',(104.087867965649,-37.5183010937783,6.56222288596766));
#69696=CARTESIAN_POINT('Ctrl Pts',(104.412132034361,-37.8400889356949,6.60451033490422));
#69697=CARTESIAN_POINT('Ctrl Pts',(104.304043604527,-37.732826766359,6.59041436013179));
#69698=CARTESIAN_POINT('Ctrl Pts',(104.195955578135,-37.6255641562347,6.57631854247011));
#69699=CARTESIAN_POINT('Ctrl Pts',(104.087867965649,-37.5183010937808,6.5622228859681));
#69700=CARTESIAN_POINT('Origin',(104.300000000005,-37.3093412868475,6.52567430068228));
#69701=CARTESIAN_POINT('Ctrl Pts',(104.300000000005,-37.3484991445135,6.22824084227013));
#69702=CARTESIAN_POINT('Ctrl Pts',(104.408087612491,-37.4557577970327,6.24236171176215));
#69703=CARTESIAN_POINT('Ctrl Pts',(104.516175638883,-37.5630160395531,6.25648252727679));
#69704=CARTESIAN_POINT('Ctrl Pts',(104.624264068717,-37.6702738824338,6.27060329017787));
#69705=CARTESIAN_POINT('Origin',(104.3,-37.3093412868425,6.52567430068162));
#69706=CARTESIAN_POINT('Origin',(104.3,-37.3093412868425,6.52567430068162));
#69707=CARTESIAN_POINT('Origin',(113.,-37.6311160247631,6.5680367485894));
#69708=CARTESIAN_POINT('',(121.811388243054,-37.6702738824291,6.27060329017725));
#69709=CARTESIAN_POINT('',(121.5,-37.9266483495649,6.61961818902335));
#69710=CARTESIAN_POINT('Ctrl Pts',(121.811388687965,-37.6702743232782,6.27060334821647));
#69711=CARTESIAN_POINT('Ctrl Pts',(121.80796264376,-37.6736730261927,6.27105080106852));
#69712=CARTESIAN_POINT('Ctrl Pts',(121.80455782351,-37.6770410168358,6.27155349760124));
#69713=CARTESIAN_POINT('Ctrl Pts',(121.765406035132,-37.7156614242077,6.27798207968717));
#69714=CARTESIAN_POINT('Ctrl Pts',(121.726559498935,-37.7528860018039,6.29095311068324));
#69715=CARTESIAN_POINT('Ctrl Pts',(121.652509215907,-37.8210334610709,6.33243037397718));
#69716=CARTESIAN_POINT('Ctrl Pts',(121.617288389766,-37.8519870416124,6.36085562876172));
#69717=CARTESIAN_POINT('Ctrl Pts',(121.56412779323,-37.8955273033918,6.4222941134767));
#69718=CARTESIAN_POINT('Ctrl Pts',(121.541159186122,-37.9128668899463,6.45742378699773));
#69719=CARTESIAN_POINT('Ctrl Pts',(121.517077828304,-37.9272585576496,6.51603387355182));
#69720=CARTESIAN_POINT('Ctrl Pts',(121.510716614322,-37.930183837478,6.53655145973755));
#69721=CARTESIAN_POINT('Ctrl Pts',(121.502178291748,-37.9316657356348,6.57810179894059));
#69722=CARTESIAN_POINT('Ctrl Pts',(121.5,-37.9302235600485,6.59913426579453));
#69723=CARTESIAN_POINT('Ctrl Pts',(121.5,-37.9266483495649,6.61961818902335));
#69724=CARTESIAN_POINT('',(104.624264068712,-37.9266483495649,6.61961818902335));
#69725=CARTESIAN_POINT('',(113.,-37.9266483495649,6.61961818902335));
#69726=CARTESIAN_POINT('Origin',(104.624264068712,-37.6311160247631,6.5680367485894));
#69727=CARTESIAN_POINT('',(113.,-37.6702738824291,6.27060329017725));
#69728=CARTESIAN_POINT('Origin',(104.624264068712,-37.6311160247631,6.5680367485892));
#69729=CARTESIAN_POINT('Origin',(104.624264068712,-37.6311160247631,6.5680367485892));
#69730=CARTESIAN_POINT('Origin',(104.3,0.,0.));
#69731=CARTESIAN_POINT('',(104.087867965648,-37.173644453084,8.29492882695119));
#69732=CARTESIAN_POINT('Origin',(104.087867965644,0.,-5.55111512312578E-16));
#69733=CARTESIAN_POINT('Origin',(104.3,-36.9666042262736,8.24872986069481));
#69734=CARTESIAN_POINT('Origin',(104.25,0.,0.));
#69735=CARTESIAN_POINT('',(104.412132034356,-37.4871203601426,8.37900319423351));
#69736=CARTESIAN_POINT('Origin',(104.412132034356,0.,-1.11022302462516E-15));
#69737=CARTESIAN_POINT('Ctrl Pts',(104.087867965648,-37.173644453086,8.29492882695164));
#69738=CARTESIAN_POINT('Ctrl Pts',(104.195955578133,-37.2781367752921,8.32295393531766));
#69739=CARTESIAN_POINT('Ctrl Pts',(104.304043604523,-37.3826287412732,8.35097872169248));
#69740=CARTESIAN_POINT('Ctrl Pts',(104.412132034356,-37.4871203601426,8.37900319423351));
#69741=CARTESIAN_POINT('Origin',(104.624264068712,0.,0.));
#69742=CARTESIAN_POINT('',(104.624264068712,-37.5728723564378,8.39817021063717));
#69743=CARTESIAN_POINT('Origin',(104.624264068712,0.,0.));
#69744=CARTESIAN_POINT('Origin',(104.624264068712,-37.2800967276863,8.33272992328156));
#69745=CARTESIAN_POINT('Origin',(113.,0.,0.));
#69746=CARTESIAN_POINT('',(121.5,-37.5728723564378,8.39817021063717));
#69747=CARTESIAN_POINT('Origin',(121.5,0.,0.));
#69748=CARTESIAN_POINT('',(113.,-37.5728723564378,8.39817021063717));
#69749=CARTESIAN_POINT('Origin',(104.3,23.9780113447946,21.7152696449976));
#69750=CARTESIAN_POINT('',(104.3,27.6775213868948,25.8390437558097));
#69751=CARTESIAN_POINT('Origin',(104.3,27.8896534212507,25.6269117214538));
#69752=CARTESIAN_POINT('',(104.3,26.7286363288515,24.8901586977665));
#69753=CARTESIAN_POINT('Origin',(104.3,26.7286363288515,24.4658946290545));
#69754=CARTESIAN_POINT('',(104.3,23.7658793104386,21.9274016793536));
#69755=CARTESIAN_POINT('Ctrl Pts',(104.300000000002,27.6775213868965,25.8390437558114));
#69756=CARTESIAN_POINT('Ctrl Pts',(104.408087612488,27.754019156457,25.9155415253719));
#69757=CARTESIAN_POINT('Ctrl Pts',(104.51617563888,27.8305166336028,25.9920390025178));
#69758=CARTESIAN_POINT('Ctrl Pts',(104.624264068714,27.9070138257223,26.0685361946373));
#69759=CARTESIAN_POINT('Ctrl Pts',(104.243382456862,27.7175202986166,25.8790426675316));
#69760=CARTESIAN_POINT('Ctrl Pts',(104.351473262603,27.7940161208215,25.9555382814697));
#69761=CARTESIAN_POINT('Ctrl Pts',(104.459564357694,27.8705114241477,26.0320339977095));
#69762=CARTESIAN_POINT('Ctrl Pts',(104.567655925525,27.947006700909,26.108529069824));
#69763=CARTESIAN_POINT('Ctrl Pts',(104.130710113065,27.8450194956664,25.9107439897146));
#69764=CARTESIAN_POINT('Ctrl Pts',(104.238807005864,27.9215059055569,25.9872412253646));
#69765=CARTESIAN_POINT('Ctrl Pts',(104.346904358902,27.9979921109243,26.0637380030864));
#69766=CARTESIAN_POINT('Ctrl Pts',(104.455001908559,28.0744781336926,26.1402346665624));
#69767=CARTESIAN_POINT('Ctrl Pts',(104.086176765823,27.9904837995326,25.8282031306363));
#69768=CARTESIAN_POINT('Ctrl Pts',(104.194269413732,28.0669635586562,25.9047133406349));
#69769=CARTESIAN_POINT('Ctrl Pts',(104.302362090344,28.1434434498089,25.9812233477494));
#69770=CARTESIAN_POINT('Ctrl Pts',(104.410455468833,28.2199229317112,26.0577327634568));
#69771=CARTESIAN_POINT('Ctrl Pts',(104.087867965646,28.045856034146,25.7704413132658));
#69772=CARTESIAN_POINT('Ctrl Pts',(104.195955578132,28.1223364854948,25.8469579301586));
#69773=CARTESIAN_POINT('Ctrl Pts',(104.304043604524,28.1988167893393,25.9234740900863));
#69774=CARTESIAN_POINT('Ctrl Pts',(104.412132034358,28.2752969494932,25.9999898046701));
#69775=CARTESIAN_POINT('',(104.624264068714,27.9070138257223,26.0685361946373));
#69776=CARTESIAN_POINT('',(104.412132034358,28.2752969494924,25.9999898046693));
#69777=CARTESIAN_POINT('Origin',(104.624264068714,28.1191458600783,25.8564041602813));
#69778=CARTESIAN_POINT('',(104.087867965646,28.0458560341451,25.770441313265));
#69779=CARTESIAN_POINT('Ctrl Pts',(104.412132034358,28.2752969494932,25.9999898046701));
#69780=CARTESIAN_POINT('Ctrl Pts',(104.304043604524,28.1988167893393,25.9234740900863));
#69781=CARTESIAN_POINT('Ctrl Pts',(104.195955578132,28.1223364854948,25.8469579301586));
#69782=CARTESIAN_POINT('Ctrl Pts',(104.087867965646,28.045856034146,25.7704413132658));
#69783=CARTESIAN_POINT('Origin',(104.300000000002,27.8896534212524,25.6269117214555));
#69784=CARTESIAN_POINT('Ctrl Pts',(104.300000000002,27.6775213868965,25.8390437558114));
#69785=CARTESIAN_POINT('Ctrl Pts',(104.408087612488,27.754019156457,25.9155415253719));
#69786=CARTESIAN_POINT('Ctrl Pts',(104.51617563888,27.8305166336028,25.9920390025178));
#69787=CARTESIAN_POINT('Ctrl Pts',(104.624264068714,27.9070138257223,26.0685361946373));
#69788=CARTESIAN_POINT('Origin',(104.3,27.8896534212507,25.6269117214538));
#69789=CARTESIAN_POINT('Origin',(104.3,27.8896534212507,25.6269117214538));
#69790=CARTESIAN_POINT('Origin',(113.,28.1191458600767,25.8564041602797));
#69791=CARTESIAN_POINT('',(121.811388243054,27.9070138257207,26.0685361946357));
#69792=CARTESIAN_POINT('',(121.5,28.3399768485066,26.0594649259364));
#69793=CARTESIAN_POINT('Ctrl Pts',(121.811388687965,27.9070141401383,26.0685365090528));
#69794=CARTESIAN_POINT('Ctrl Pts',(121.80796264376,27.9094381275961,26.070960489325));
#69795=CARTESIAN_POINT('Ctrl Pts',(121.80455782351,27.9118872463663,26.0733264736922));
#69796=CARTESIAN_POINT('Ctrl Pts',(121.765406035132,27.9404979978181,26.100052630067));
#69797=CARTESIAN_POINT('Ctrl Pts',(121.726559498935,27.9734494956375,26.1216886096789));
#69798=CARTESIAN_POINT('Ctrl Pts',(121.652509215907,28.0478411657046,26.1505038660466));
#69799=CARTESIAN_POINT('Ctrl Pts',(121.617288389766,28.0892357824599,26.1577567938406));
#69800=CARTESIAN_POINT('Ctrl Pts',(121.56412779323,28.1644838415113,26.1548982262093));
#69801=CARTESIAN_POINT('Ctrl Pts',(121.541159186122,28.2029097568318,26.1472690548683));
#69802=CARTESIAN_POINT('Ctrl Pts',(121.517077828304,28.2581693569711,26.123007172468));
#69803=CARTESIAN_POINT('Ctrl Pts',(121.510716614322,28.2762278500349,26.1128376379049));
#69804=CARTESIAN_POINT('Ctrl Pts',(121.502178291748,28.3100940728715,26.0887190628886));
#69805=CARTESIAN_POINT('Ctrl Pts',(121.5,28.3259023098338,26.0747711534923));
#69806=CARTESIAN_POINT('Ctrl Pts',(121.5,28.3399768485066,26.0594649259364));
#69807=CARTESIAN_POINT('',(104.624264068712,28.3399768485066,26.0594649259364));
#69808=CARTESIAN_POINT('',(113.,28.3399768485066,26.0594649259364));
#69809=CARTESIAN_POINT('Origin',(104.624264068712,28.1191458600767,25.8564041602797));
#69810=CARTESIAN_POINT('',(113.,27.9070138257207,26.0685361946357));
#69811=CARTESIAN_POINT('Origin',(104.624264068712,28.1191458600766,25.8564041602798));
#69812=CARTESIAN_POINT('Origin',(104.624264068712,28.1191458600766,25.8564041602798));
#69813=CARTESIAN_POINT('Origin',(104.3,0.,0.));
#69814=CARTESIAN_POINT('',(104.087867965647,29.2106904110607,24.4422022714321));
#69815=CARTESIAN_POINT('Origin',(104.087867965644,2.22044604925031E-15,
-2.22044604925031E-15));
#69816=CARTESIAN_POINT('Origin',(104.3,29.0480002025284,24.3060703646348));
#69817=CARTESIAN_POINT('Origin',(104.25,0.,0.));
#69818=CARTESIAN_POINT('',(104.412132034356,29.4682231323184,24.6397181974285));
#69819=CARTESIAN_POINT('Origin',(104.412132034356,2.22044604925031E-15,
-2.22044604925031E-15));
#69820=CARTESIAN_POINT('Ctrl Pts',(104.087867965647,29.2106904110617,24.4422022714329));
#69821=CARTESIAN_POINT('Ctrl Pts',(104.195955578132,29.2965351197829,24.5080409992732));
#69822=CARTESIAN_POINT('Ctrl Pts',(104.304043604523,29.3823793561953,24.573879640517));
#69823=CARTESIAN_POINT('Ctrl Pts',(104.412132034356,29.4682231323184,24.6397181974285));
#69824=CARTESIAN_POINT('Origin',(104.624264068712,0.,0.));
#69825=CARTESIAN_POINT('',(104.624264068712,29.5356318566107,24.6960816898302));
#69826=CARTESIAN_POINT('Origin',(104.624264068712,0.,0.));
#69827=CARTESIAN_POINT('Origin',(104.624264068712,29.3054840759098,24.5036446896497));
#69828=CARTESIAN_POINT('Origin',(113.,0.,0.));
#69829=CARTESIAN_POINT('',(121.5,29.5356318566107,24.6960816898302));
#69830=CARTESIAN_POINT('Origin',(121.5,0.,0.));
#69831=CARTESIAN_POINT('',(113.,29.5356318566107,24.6960816898302));
#69832=CARTESIAN_POINT('Origin',(104.3,34.2680340892069,12.4624569551452));
#69833=CARTESIAN_POINT('',(104.3,35.4588694735005,13.2804347819611));
#69834=CARTESIAN_POINT('Origin',(104.3,35.57367450321,13.0032709222077));
#69835=CARTESIAN_POINT('',(104.3,34.2190913987366,12.7669018890611));
#69836=CARTESIAN_POINT('Origin',(104.3,34.0567325686927,12.3749329995982));
#69837=CARTESIAN_POINT('',(104.3,34.1532290594974,12.7396208148986));
#69838=CARTESIAN_POINT('Origin',(121.7,33.2124490802637,10.5556907983726));
#69839=CARTESIAN_POINT('',(121.7,36.2160289954763,11.0499147569331));
#69840=CARTESIAN_POINT('Origin',(121.7,36.1383832819455,11.3396925048198));
#69841=CARTESIAN_POINT('',(121.7,34.9198279009177,10.7025987204178));
#69842=CARTESIAN_POINT('Origin',(121.7,34.5524044395002,10.9147307547738));
#69843=CARTESIAN_POINT('',(121.7,33.2900947937945,10.2659130504859));
#69844=CARTESIAN_POINT('Ctrl Pts',(121.699999999996,36.2160289954802,11.0499147569342));
#69845=CARTESIAN_POINT('Ctrl Pts',(121.59191238751,36.3205268920326,11.0779148839261));
#69846=CARTESIAN_POINT('Ctrl Pts',(121.483824361118,36.4250243891393,11.1059149038869));
#69847=CARTESIAN_POINT('Ctrl Pts',(121.375735931284,36.5295214968926,11.1339148195208));
#69848=CARTESIAN_POINT('Ctrl Pts',(121.756617543136,36.2706685250136,11.0645553747474));
#69849=CARTESIAN_POINT('Ctrl Pts',(121.648526737396,36.3751635810645,11.0925548930912));
#69850=CARTESIAN_POINT('Ctrl Pts',(121.540435642304,36.4796584662719,11.120553910922));
#69851=CARTESIAN_POINT('Ctrl Pts',(121.432344074473,36.584152780368,11.1485532278095));
#69852=CARTESIAN_POINT('Ctrl Pts',(121.869288428606,36.3618703486632,11.1591238127641));
#69853=CARTESIAN_POINT('Ctrl Pts',(121.761191535807,36.4663621030006,11.1871143689486));
#69854=CARTESIAN_POINT('Ctrl Pts',(121.653094183832,36.5708533597461,11.2151049763399));
#69855=CARTESIAN_POINT('Ctrl Pts',(121.544996634175,36.6753444250052,11.2430954833537));
#69856=CARTESIAN_POINT('Ctrl Pts',(121.913823234175,36.3631219450037,11.3263684692943));
#69857=CARTESIAN_POINT('Ctrl Pts',(121.805730586266,36.4676216100731,11.3543467785713));
#69858=CARTESIAN_POINT('Ctrl Pts',(121.697637909655,36.5721211654543,11.382325303631));
#69859=CARTESIAN_POINT('Ctrl Pts',(121.589544531166,36.6766200040367,11.410303769973));
#69860=CARTESIAN_POINT('Ctrl Pts',(121.912132034352,36.3407848610987,11.403203139819));
#69861=CARTESIAN_POINT('Ctrl Pts',(121.804044421866,36.4452904208139,11.4311788451336));
#69862=CARTESIAN_POINT('Ctrl Pts',(121.695956395474,36.5497955110335,11.4591546511882));
#69863=CARTESIAN_POINT('Ctrl Pts',(121.58786796564,36.6543001437287,11.4871305554751));
#69864=CARTESIAN_POINT('',(121.375735931284,36.5295214968926,11.1339148195208));
#69865=CARTESIAN_POINT('',(121.58786796564,36.6543001437269,11.4871305554746));
#69866=CARTESIAN_POINT('Origin',(121.375735931284,36.4518757833619,11.4236925674075));
#69867=CARTESIAN_POINT('',(121.912132034352,36.3407848610968,11.4032031398184));
#69868=CARTESIAN_POINT('Ctrl Pts',(121.58786796564,36.6543001437287,11.4871305554751));
#69869=CARTESIAN_POINT('Ctrl Pts',(121.695956395474,36.5497955110335,11.4591546511882));
#69870=CARTESIAN_POINT('Ctrl Pts',(121.804044421866,36.4452904208139,11.4311788451336));
#69871=CARTESIAN_POINT('Ctrl Pts',(121.912132034352,36.3407848610987,11.403203139819));
#69872=CARTESIAN_POINT('Origin',(121.699999999996,36.1383832819494,11.3396925048209));
#69873=CARTESIAN_POINT('Ctrl Pts',(121.699999999996,36.2160289954802,11.0499147569342));
#69874=CARTESIAN_POINT('Ctrl Pts',(121.59191238751,36.3205268920326,11.0779148839261));
#69875=CARTESIAN_POINT('Ctrl Pts',(121.483824361118,36.4250243891393,11.1059149038869));
#69876=CARTESIAN_POINT('Ctrl Pts',(121.375735931284,36.5295214968926,11.1339148195208));
#69877=CARTESIAN_POINT('Origin',(121.7,36.1383832819455,11.3396925048198));
#69878=CARTESIAN_POINT('Origin',(121.7,36.1383832819455,11.3396925048198));
#69879=CARTESIAN_POINT('Origin',(104.624264068712,0.,0.));
#69880=CARTESIAN_POINT('',(104.412132034356,36.7173517348831,11.2839695587002));
#69881=CARTESIAN_POINT('',(104.412132034356,36.072733467222,13.2003707382617));
#69882=CARTESIAN_POINT('Origin',(104.412132034356,-2.22044604925031E-15,
2.22044604925031E-15));
#69883=CARTESIAN_POINT('',(104.624264068712,36.155250045634,13.2305666597347));
#69884=CARTESIAN_POINT('Origin',(104.624264068712,35.8735208244992,13.1274713351134));
#69885=CARTESIAN_POINT('',(104.624264068712,36.7381470591438,11.5134074305014));
#69886=CARTESIAN_POINT('Origin',(104.624264068712,0.,0.));
#69887=CARTESIAN_POINT('Ctrl Pts',(104.624264068712,36.7381470591438,11.5134074305014));
#69888=CARTESIAN_POINT('Ctrl Pts',(104.623447602755,36.7383921797988,11.5126252746777));
#69889=CARTESIAN_POINT('Ctrl Pts',(104.622631133476,36.7386340959198,11.5118421110862));
#69890=CARTESIAN_POINT('Ctrl Pts',(104.585817132853,36.7493973673699,11.4764845542992));
#69891=CARTESIAN_POINT('Ctrl Pts',(104.54955560756,36.753767100971,11.4397053350853));
#69892=CARTESIAN_POINT('Ctrl Pts',(104.476315456228,36.7481781483961,11.3609642258508));
#69893=CARTESIAN_POINT('Ctrl Pts',(104.441383090819,36.7366717480496,11.3206778927557));
#69894=CARTESIAN_POINT('Ctrl Pts',(104.412132034356,36.7173517348831,11.2839695587002));
#69895=CARTESIAN_POINT('Origin',(113.,36.4518757833583,11.4236925674066));
#69896=CARTESIAN_POINT('',(121.375735931288,36.7381470591438,11.5134074305014));
#69897=CARTESIAN_POINT('',(113.,36.7381470591438,11.5134074305014));
#69898=CARTESIAN_POINT('Origin',(121.375735931288,36.4518757833583,11.4236925674066));
#69899=CARTESIAN_POINT('',(104.188611756946,36.529521496889,11.1339148195199));
#69900=CARTESIAN_POINT('',(113.,36.529521496889,11.1339148195199));
#69901=CARTESIAN_POINT('Ctrl Pts',(104.188611312035,36.5295219263909,11.1339149346049));
#69902=CARTESIAN_POINT('Ctrl Pts',(104.192037383128,36.5328331746008,11.1348021861489));
#69903=CARTESIAN_POINT('Ctrl Pts',(104.195442206093,36.536106738883,11.1357401947046));
#69904=CARTESIAN_POINT('Ctrl Pts',(104.234593964868,36.5735576166579,11.1471547454652));
#69905=CARTESIAN_POINT('Ctrl Pts',(104.273440501065,36.6087706735473,11.1648735898636));
#69906=CARTESIAN_POINT('Ctrl Pts',(104.347490784093,36.6709212526118,11.2148910377878));
#69907=CARTESIAN_POINT('Ctrl Pts',(104.382711610234,36.6978997807109,11.2471133635809));
#69908=CARTESIAN_POINT('Ctrl Pts',(104.411969203877,36.7172441591385,11.2837653061586));
#69909=CARTESIAN_POINT('Ctrl Pts',(104.412050624034,36.7172979642269,11.2838673935933));
#69910=CARTESIAN_POINT('Ctrl Pts',(104.412132034356,36.7173517348831,11.2839695587002));
#69911=CARTESIAN_POINT('Origin',(121.375735931288,36.4518757833583,11.4236925674064));
#69912=CARTESIAN_POINT('Origin',(121.375735931288,36.4518757833583,11.4236925674064));
#69913=CARTESIAN_POINT('Ctrl Pts',(104.300000000003,35.4588694735036,13.2804347819624));
#69914=CARTESIAN_POINT('Ctrl Pts',(104.408087612488,35.558818626106,13.321835076518));
#69915=CARTESIAN_POINT('Ctrl Pts',(104.516175638879,35.6587673966503,13.36323521282));
#69916=CARTESIAN_POINT('Ctrl Pts',(104.624264068712,35.7587157947897,13.4046351948668));
#69917=CARTESIAN_POINT('Ctrl Pts',(104.243382456863,35.5111305701924,13.3020820369954));
#69918=CARTESIAN_POINT('Ctrl Pts',(104.351473262602,35.6110770987519,13.3434810852363));
#69919=CARTESIAN_POINT('Ctrl Pts',(104.459564357693,35.7110231870791,13.384880426558));
#69920=CARTESIAN_POINT('Ctrl Pts',(104.567655925523,35.8109690043675,13.4262791829515));
#69921=CARTESIAN_POINT('Ctrl Pts',(104.130709407258,35.641056320471,13.2825795738598));
#69922=CARTESIAN_POINT('Ctrl Pts',(104.238806300055,35.7409947737881,13.323983722304));
#69923=CARTESIAN_POINT('Ctrl Pts',(104.346903653607,35.8409328626172,13.365387525334));
#69924=CARTESIAN_POINT('Ctrl Pts',(104.455001203263,35.9408707393185,13.4067912933035));
#69925=CARTESIAN_POINT('Ctrl Pts',(104.086176765824,35.7438605133325,13.1506538199746));
#69926=CARTESIAN_POINT('Ctrl Pts',(104.194269413732,35.8437977872103,13.1920725002922));
#69927=CARTESIAN_POINT('Ctrl Pts',(104.302362090342,35.9437351054269,13.2334909426439));
#69928=CARTESIAN_POINT('Ctrl Pts',(104.410455468831,36.0436718192237,13.2749089952201));
#69929=CARTESIAN_POINT('Ctrl Pts',(104.087867965647,35.7729132970301,13.0760988223458));
#69930=CARTESIAN_POINT('Ctrl Pts',(104.195955578132,35.8728536622531,13.1175231569586));
#69931=CARTESIAN_POINT('Ctrl Pts',(104.304043604523,35.9727937163268,13.1589471258382));
#69932=CARTESIAN_POINT('Ctrl Pts',(104.412132034356,36.072733467222,13.2003707382617));
#69933=CARTESIAN_POINT('',(104.624264068712,35.7587157947897,13.4046351948668));
#69934=CARTESIAN_POINT('Origin',(104.624264068712,35.8735208244992,13.1274713351134));
#69935=CARTESIAN_POINT('',(104.087867965647,35.7729132970286,13.0760988223452));
#69936=CARTESIAN_POINT('Ctrl Pts',(104.412132034356,36.072733467222,13.2003707382617));
#69937=CARTESIAN_POINT('Ctrl Pts',(104.304043604523,35.9727937163268,13.1589471258382));
#69938=CARTESIAN_POINT('Ctrl Pts',(104.195955578132,35.8728536622531,13.1175231569586));
#69939=CARTESIAN_POINT('Ctrl Pts',(104.087867965647,35.7729132970301,13.0760988223458));
#69940=CARTESIAN_POINT('Origin',(104.300000000003,35.5736745032131,13.003270922209));
#69941=CARTESIAN_POINT('Ctrl Pts',(104.300000000003,35.4588694735036,13.2804347819624));
#69942=CARTESIAN_POINT('Ctrl Pts',(104.408087612488,35.558818626106,13.321835076518));
#69943=CARTESIAN_POINT('Ctrl Pts',(104.516175638879,35.6587673966503,13.36323521282));
#69944=CARTESIAN_POINT('Ctrl Pts',(104.624264068712,35.7587157947897,13.4046351948668));
#69945=CARTESIAN_POINT('Origin',(104.624264068712,35.8735208244992,13.1274713351134));
#69946=CARTESIAN_POINT('Origin',(104.624264068712,35.8735208244992,13.1274713351134));
#69947=CARTESIAN_POINT('Origin',(104.3,35.57367450321,13.0032709222079));
#69948=CARTESIAN_POINT('Origin',(104.3,35.57367450321,13.0032709222079));
#69949=CARTESIAN_POINT('Origin',(113.,0.,0.));
#69950=CARTESIAN_POINT('',(121.375735931288,36.155250045634,13.2305666597347));
#69951=CARTESIAN_POINT('',(113.,36.155250045634,13.2305666597347));
#69952=CARTESIAN_POINT('Origin',(121.375735931288,0.,0.));
#69953=CARTESIAN_POINT('Origin',(113.,35.8735208244992,13.1274713351134));
#69954=CARTESIAN_POINT('',(121.375735931288,35.7587157947897,13.4046351948668));
#69955=CARTESIAN_POINT('',(113.,35.7587157947897,13.4046351948668));
#69956=CARTESIAN_POINT('Origin',(121.375735931288,35.8735208244992,13.1274713351134));
#69957=CARTESIAN_POINT('Origin',(113.,35.3739408143757,13.2452561795175));
#69958=CARTESIAN_POINT('',(121.7,34.2190913987366,12.7669018890611));
#69959=CARTESIAN_POINT('',(103.5,34.2190913987366,12.7669018890611));
#69960=CARTESIAN_POINT('Origin',(121.7,33.9419275389832,12.6520968593516));
#69961=CARTESIAN_POINT('Ctrl Pts',(121.375735931288,35.7587157947897,13.4046351948668));
#69962=CARTESIAN_POINT('Ctrl Pts',(121.583825474459,35.5662972672787,13.3249328311199));
#69963=CARTESIAN_POINT('Ctrl Pts',(121.79191352265,35.3738773597987,13.2452298957711));
#69964=CARTESIAN_POINT('Ctrl Pts',(122.,35.1814560023665,13.1655263598324));
#69965=CARTESIAN_POINT('Origin',(104.3,0.,0.));
#69966=CARTESIAN_POINT('',(104.087868515434,36.4321547447161,11.1078254769055));
#69967=CARTESIAN_POINT('Origin',(104.087867965644,-2.22044604925031E-15,
4.44089209850063E-15));
#69968=CARTESIAN_POINT('Ctrl Pts',(104.087868240379,36.4321550102444,11.1078255480536));
#69969=CARTESIAN_POINT('Ctrl Pts',(104.061688713442,36.4068528521804,11.1010458552336));
#69970=CARTESIAN_POINT('Ctrl Pts',(104.037012788768,36.3711596598708,11.0914818931789));
#69971=CARTESIAN_POINT('Ctrl Pts',(104.008670719845,36.3050447967167,11.0737664689891));
#69972=CARTESIAN_POINT('Ctrl Pts',(104.,36.2629210472339,11.062479444333));
#69973=CARTESIAN_POINT('Ctrl Pts',(104.,36.2271308071048,11.0528894783935));
#69974=CARTESIAN_POINT('Origin',(104.25,0.,0.));
#69975=CARTESIAN_POINT('',(104.25,36.5888522644724,11.1498124507801));
#69976=CARTESIAN_POINT('Origin',(104.3,15.5731406460551,23.7734708323834));
#69977=CARTESIAN_POINT('',(104.3,20.0467960840287,32.1220693465106));
#69978=CARTESIAN_POINT('Origin',(104.3,20.3066037051641,31.9720693465106));
#69979=CARTESIAN_POINT('',(104.3,19.3758330249198,30.959927238132));
#69980=CARTESIAN_POINT('Origin',(104.3,19.4856406460551,30.5501196169967));
#69981=CARTESIAN_POINT('',(104.3,15.3133330249198,23.9234708323834));
#69982=CARTESIAN_POINT('Ctrl Pts',(104.300000000003,20.0467960840302,32.122069346513));
#69983=CARTESIAN_POINT('Ctrl Pts',(104.408087612489,20.100888175632,32.2157595974551));
#69984=CARTESIAN_POINT('Ctrl Pts',(104.51617563888,20.1549800604655,32.3094494902639));
#69985=CARTESIAN_POINT('Ctrl Pts',(104.624264068715,20.209071743755,32.4031390339881));
#69986=CARTESIAN_POINT('Ctrl Pts',(104.243382456862,20.0750795857475,32.1710578085035));
#69987=CARTESIAN_POINT('Ctrl Pts',(104.351473262603,20.1291703542645,32.2647454732615));
#69988=CARTESIAN_POINT('Ctrl Pts',(104.459564357695,20.1832605951054,32.3584331025398));
#69989=CARTESIAN_POINT('Ctrl Pts',(104.567655925525,20.2373509769986,32.4521201027653));
#69990=CARTESIAN_POINT('Ctrl Pts',(104.130709934827,20.1900293243368,32.2346784312497));
#69991=CARTESIAN_POINT('Ctrl Pts',(104.238806827626,20.2441105815262,32.3283652263749));
#69992=CARTESIAN_POINT('Ctrl Pts',(104.346904180794,20.2981917597176,32.4220515260737));
#69993=CARTESIAN_POINT('Ctrl Pts',(104.455001730451,20.3522727910653,32.5157376683266));
#69994=CARTESIAN_POINT('Ctrl Pts',(104.086176765824,20.3519003213093,32.1925987394747));
#69995=CARTESIAN_POINT('Ctrl Pts',(104.194269413732,20.4059717963426,32.2862963455131));
#69996=CARTESIAN_POINT('Ctrl Pts',(104.302362090344,20.4600434514167,32.3799937897523));
#69997=CARTESIAN_POINT('Ctrl Pts',(104.410455468833,20.5141148642526,32.4736905568143));
#69998=CARTESIAN_POINT('Ctrl Pts',(104.087867965647,20.4203356511969,32.151136497191));
#69999=CARTESIAN_POINT('Ctrl Pts',(104.195955578133,20.4744061366423,32.244840470975));
#70000=CARTESIAN_POINT('Ctrl Pts',(104.304043604524,20.5284765978807,32.3385439651879));
#70001=CARTESIAN_POINT('Ctrl Pts',(104.412132034359,20.5825470355882,32.4322469920417));
#70002=CARTESIAN_POINT('',(104.624264068715,20.209071743755,32.4031390339881));
#70003=CARTESIAN_POINT('',(104.412132034359,20.5825470355875,32.4322469920406));
#70004=CARTESIAN_POINT('Origin',(104.624264068715,20.4688793648903,32.2531390339881));
#70005=CARTESIAN_POINT('',(104.087867965647,20.4203356511961,32.1511364971898));
#70006=CARTESIAN_POINT('Ctrl Pts',(104.412132034359,20.5825470355882,32.4322469920417));
#70007=CARTESIAN_POINT('Ctrl Pts',(104.304043604524,20.5284765978807,32.3385439651879));
#70008=CARTESIAN_POINT('Ctrl Pts',(104.195955578133,20.4744061366423,32.244840470975));
#70009=CARTESIAN_POINT('Ctrl Pts',(104.087867965647,20.4203356511969,32.151136497191));
#70010=CARTESIAN_POINT('Origin',(104.300000000003,20.3066037051655,31.972069346513));
#70011=CARTESIAN_POINT('Ctrl Pts',(104.300000000003,20.0467960840302,32.122069346513));
#70012=CARTESIAN_POINT('Ctrl Pts',(104.408087612489,20.100888175632,32.2157595974551));
#70013=CARTESIAN_POINT('Ctrl Pts',(104.51617563888,20.1549800604655,32.3094494902639));
#70014=CARTESIAN_POINT('Ctrl Pts',(104.624264068715,20.209071743755,32.4031390339881));
#70015=CARTESIAN_POINT('Origin',(104.3,20.3066037051641,31.9720693465106));
#70016=CARTESIAN_POINT('Origin',(104.3,20.3066037051641,31.9720693465106));
#70017=CARTESIAN_POINT('Origin',(113.,20.468879364889,32.2531390339859));
#70018=CARTESIAN_POINT('',(121.811388243054,20.2090717437536,32.4031390339859));
#70019=CARTESIAN_POINT('',(121.5,20.6296297263933,32.5064359373941));
#70020=CARTESIAN_POINT('Ctrl Pts',(121.811388687965,20.2090719660805,32.4031394190667));
#70021=CARTESIAN_POINT('Ctrl Pts',(121.80796264376,20.2107859859092,32.4061081783332));
#70022=CARTESIAN_POINT('Ctrl Pts',(121.80455782351,20.2125392911663,32.4090274223195));
#70023=CARTESIAN_POINT('Ctrl Pts',(121.765406035132,20.233257916631,32.4422479143698));
#70024=CARTESIAN_POINT('Ctrl Pts',(121.726559498935,20.2594868158067,32.4716751410544));
#70025=CARTESIAN_POINT('Ctrl Pts',(121.652509215907,20.3238857140478,32.5187625223814));
#70026=CARTESIAN_POINT('Ctrl Pts',(121.617288389766,20.3619926475953,32.5364820278348));
#70027=CARTESIAN_POINT('Ctrl Pts',(121.56412779323,20.4354165429558,32.553196494323));
#70028=CARTESIAN_POINT('Ctrl Pts',(121.541159186122,20.4745077018041,32.555772639402));
#70029=CARTESIAN_POINT('Ctrl Pts',(121.517077828304,20.5341638139643,32.546639697538));
#70030=CARTESIAN_POINT('Ctrl Pts',(121.510716614322,20.5542390480232,32.5414905633929));
#70031=CARTESIAN_POINT('Ctrl Pts',(121.502178291748,20.5931936538549,32.5269590323472));
#70032=CARTESIAN_POINT('Ctrl Pts',(121.5,20.612073222796,32.5175778592339));
#70033=CARTESIAN_POINT('Ctrl Pts',(121.5,20.6296297263933,32.5064359373941));
#70034=CARTESIAN_POINT('',(104.624264068712,20.6296297263933,32.5064359373941));
#70035=CARTESIAN_POINT('',(113.,20.6296297263933,32.5064359373941));
#70036=CARTESIAN_POINT('Origin',(104.624264068712,20.468879364889,32.2531390339859));
#70037=CARTESIAN_POINT('',(113.,20.2090717437536,32.4031390339859));
#70038=CARTESIAN_POINT('Origin',(104.624264068712,20.4688793648889,32.2531390339859));
#70039=CARTESIAN_POINT('Origin',(104.624264068712,20.4688793648889,32.2531390339859));
#70040=CARTESIAN_POINT('Origin',(104.3,0.,0.));
#70041=CARTESIAN_POINT('',(104.087867965647,21.8892528196833,31.1696374243337));
#70042=CARTESIAN_POINT('Origin',(104.087867965644,-2.22044604925031E-15,
2.22044604925031E-15));
#70043=CARTESIAN_POINT('Origin',(104.3,21.7673396757028,30.9960367753563));
#70044=CARTESIAN_POINT('Origin',(104.25,0.,0.));
#70045=CARTESIAN_POINT('',(104.412132034356,22.0868894429017,31.4270775313556));
#70046=CARTESIAN_POINT('Origin',(104.412132034356,0.,0.));
#70047=CARTESIAN_POINT('Ctrl Pts',(104.087867965647,21.8892528196841,31.1696374243348));
#70048=CARTESIAN_POINT('Ctrl Pts',(104.195955578132,21.9551321242177,31.2554509974641));
#70049=CARTESIAN_POINT('Ctrl Pts',(104.304043604523,22.0210109949489,31.341264364705));
#70050=CARTESIAN_POINT('Ctrl Pts',(104.412132034356,22.0868894429017,31.4270775313556));
#70051=CARTESIAN_POINT('Origin',(104.624264068712,0.,0.));
#70052=CARTESIAN_POINT('',(104.624264068712,22.1374133253307,31.4989671459791));
#70053=CARTESIAN_POINT('Origin',(104.624264068712,0.,0.));
#70054=CARTESIAN_POINT('Origin',(104.624264068712,21.9649140007177,31.2535206487377));
#70055=CARTESIAN_POINT('Origin',(113.,0.,0.));
#70056=CARTESIAN_POINT('',(121.5,22.1374133253307,31.4989671459791));
#70057=CARTESIAN_POINT('Origin',(121.5,0.,0.));
#70058=CARTESIAN_POINT('',(113.,22.1374133253307,31.4989671459791));
#70059=CARTESIAN_POINT('Origin',(104.3,27.907343512885,19.3973019778198));
#70060=CARTESIAN_POINT('',(104.3,30.8134083466537,22.0053456777902));
#70061=CARTESIAN_POINT('Origin',(104.3,30.9960367753563,21.7673396757028));
#70062=CARTESIAN_POINT('',(104.3,29.7487867783414,21.1884328164397));
#70063=CARTESIAN_POINT('Origin',(104.3,29.6934092049567,20.7677983856497));
#70064=CARTESIAN_POINT('',(104.3,27.7247150841823,19.6353079799071));
#70065=CARTESIAN_POINT('Ctrl Pts',(104.300000000003,30.8134083466557,22.0053456777917));
#70066=CARTESIAN_POINT('Ctrl Pts',(104.408087612488,30.899236629767,22.0712040357549));
#70067=CARTESIAN_POINT('Ctrl Pts',(104.51617563888,30.9850645847977,22.137062141973));
#70068=CARTESIAN_POINT('Ctrl Pts',(104.624264068714,31.0708922200369,22.2029200028065));
#70069=CARTESIAN_POINT('Ctrl Pts',(104.243382456862,30.8582859677809,22.0397814876374));
#70070=CARTESIAN_POINT('Ctrl Pts',(104.351473262603,30.9441120388314,22.1056379626008));
#70071=CARTESIAN_POINT('Ctrl Pts',(104.459564357694,31.0299376087953,22.171494606718));
#70072=CARTESIAN_POINT('Ctrl Pts',(104.567655925525,31.1157630683464,22.2373506156879));
#70073=CARTESIAN_POINT('Ctrl Pts',(104.130710008275,30.9888322399386,22.0545697937069));
#70074=CARTESIAN_POINT('Ctrl Pts',(104.238806901074,31.0746491908742,22.1204291050618));
#70075=CARTESIAN_POINT('Ctrl Pts',(104.346904254189,31.1604658792464,22.1862879890029));
#70076=CARTESIAN_POINT('Ctrl Pts',(104.455001803846,31.2462823716881,22.2521467836084));
#70077=CARTESIAN_POINT('Ctrl Pts',(104.086176765824,31.1222783369416,21.9537480036383));
#70078=CARTESIAN_POINT('Ctrl Pts',(104.194269413732,31.2080903875008,22.0196210464437));
#70079=CARTESIAN_POINT('Ctrl Pts',(104.302362090344,31.293902542478,22.0854938708675));
#70080=CARTESIAN_POINT('Ctrl Pts',(104.410455468833,31.3797142145118,22.1513661623616));
#70081=CARTESIAN_POINT('Ctrl Pts',(104.087867965647,31.1696374243347,21.8892528196839));
#70082=CARTESIAN_POINT('Ctrl Pts',(104.195955578132,31.2554509974646,21.9551321242181));
#70083=CARTESIAN_POINT('Ctrl Pts',(104.304043604524,31.3412643647062,22.0210109949498));
#70084=CARTESIAN_POINT('Ctrl Pts',(104.412132034358,31.4270775313574,22.0868894429031));
#70085=CARTESIAN_POINT('',(104.624264068714,31.0708922200369,22.2029200028065));
#70086=CARTESIAN_POINT('',(104.412132034358,31.4270775313565,22.0868894429024));
#70087=CARTESIAN_POINT('Origin',(104.624264068714,31.2535206487395,21.9649140007191));
#70088=CARTESIAN_POINT('',(104.087867965647,31.1696374243336,21.8892528196832));
#70089=CARTESIAN_POINT('Ctrl Pts',(104.412132034358,31.4270775313574,22.0868894429031));
#70090=CARTESIAN_POINT('Ctrl Pts',(104.304043604524,31.3412643647062,22.0210109949498));
#70091=CARTESIAN_POINT('Ctrl Pts',(104.195955578132,31.2554509974646,21.9551321242181));
#70092=CARTESIAN_POINT('Ctrl Pts',(104.087867965647,31.1696374243347,21.8892528196839));
#70093=CARTESIAN_POINT('Origin',(104.300000000003,30.9960367753583,21.7673396757043));
#70094=CARTESIAN_POINT('Ctrl Pts',(104.300000000003,30.8134083466557,22.0053456777917));
#70095=CARTESIAN_POINT('Ctrl Pts',(104.408087612488,30.899236629767,22.0712040357549));
#70096=CARTESIAN_POINT('Ctrl Pts',(104.51617563888,30.9850645847977,22.137062141973));
#70097=CARTESIAN_POINT('Ctrl Pts',(104.624264068714,31.0708922200369,22.2029200028065));
#70098=CARTESIAN_POINT('Origin',(104.3,30.9960367753563,21.7673396757028));
#70099=CARTESIAN_POINT('Origin',(104.3,30.9960367753563,21.7673396757028));
#70100=CARTESIAN_POINT('Origin',(113.,31.2535206487377,21.9649140007177));
#70101=CARTESIAN_POINT('',(121.811388243054,31.0708922200351,22.2029200028051));
#70102=CARTESIAN_POINT('',(121.5,31.4989671459791,22.1374133253307));
#70103=CARTESIAN_POINT('Ctrl Pts',(121.811388687965,31.0708925728024,22.2029202734925));
#70104=CARTESIAN_POINT('Ctrl Pts',(121.80796264376,31.0736122156265,22.2050071224247));
#70105=CARTESIAN_POINT('Ctrl Pts',(121.80455782351,31.0763492047763,22.2070331913203));
#70106=CARTESIAN_POINT('Ctrl Pts',(121.765406035132,31.1082036507075,22.2297962492787));
#70107=CARTESIAN_POINT('Ctrl Pts',(121.726559498935,31.1436973059289,22.2469460965475));
#70108=CARTESIAN_POINT('Ctrl Pts',(121.652509215907,31.2212136906374,22.2658047729756));
#70109=CARTESIAN_POINT('Ctrl Pts',(121.617288389766,31.2632008677555,22.2675925692634));
#70110=CARTESIAN_POINT('Ctrl Pts',(121.56412779323,31.3374320512821,22.2549366144545));
#70111=CARTESIAN_POINT('Ctrl Pts',(121.541159186122,31.3745334208854,22.2423571233226));
#70112=CARTESIAN_POINT('Ctrl Pts',(121.517077828304,31.4261534563592,22.2110899794998));
#70113=CARTESIAN_POINT('Ctrl Pts',(121.510716614322,31.4427300658883,22.1986503403778));
#70114=CARTESIAN_POINT('Ctrl Pts',(121.502178291748,31.4731584527351,22.1703176740025));
#70115=CARTESIAN_POINT('Ctrl Pts',(121.5,31.4870108805358,22.1544257019282));
#70116=CARTESIAN_POINT('Ctrl Pts',(121.5,31.4989671459791,22.1374133253307));
#70117=CARTESIAN_POINT('',(104.624264068712,31.4989671459791,22.1374133253307));
#70118=CARTESIAN_POINT('',(113.,31.4989671459791,22.1374133253307));
#70119=CARTESIAN_POINT('Origin',(104.624264068712,31.2535206487377,21.9649140007177));
#70120=CARTESIAN_POINT('',(113.,31.0708922200351,22.2029200028051));
#70121=CARTESIAN_POINT('Origin',(104.624264068712,31.2535206487377,21.9649140007178));
#70122=CARTESIAN_POINT('Origin',(104.624264068712,31.2535206487377,21.9649140007178));
#70123=CARTESIAN_POINT('Origin',(104.3,0.,0.));
#70124=CARTESIAN_POINT('',(104.087867965647,32.1511364971898,20.4203356511962));
#70125=CARTESIAN_POINT('Origin',(104.087867965644,2.22044604925031E-15,
-2.22044604925031E-15));
#70126=CARTESIAN_POINT('Origin',(104.3,31.9720693465106,20.3066037051641));
#70127=CARTESIAN_POINT('Origin',(104.25,0.,0.));
#70128=CARTESIAN_POINT('',(104.412132034356,32.4322469920394,20.5825470355869));
#70129=CARTESIAN_POINT('Origin',(104.412132034356,-2.22044604925031E-15,
2.22044604925031E-15));
#70130=CARTESIAN_POINT('Ctrl Pts',(104.087867965647,32.1511364971911,20.4203356511969));
#70131=CARTESIAN_POINT('Ctrl Pts',(104.195955578132,32.2448404709744,20.4744061366419));
#70132=CARTESIAN_POINT('Ctrl Pts',(104.304043604523,32.3385439651864,20.5284765978799));
#70133=CARTESIAN_POINT('Ctrl Pts',(104.412132034356,32.4322469920394,20.5825470355869));
#70134=CARTESIAN_POINT('Origin',(104.624264068712,0.,0.));
#70135=CARTESIAN_POINT('',(104.624264068712,32.5064359373941,20.6296297263933));
#70136=CARTESIAN_POINT('Origin',(104.624264068712,0.,0.));
#70137=CARTESIAN_POINT('Origin',(104.624264068712,32.2531390339859,20.468879364889));
#70138=CARTESIAN_POINT('Origin',(113.,0.,0.));
#70139=CARTESIAN_POINT('',(121.5,32.5064359373941,20.6296297263933));
#70140=CARTESIAN_POINT('Origin',(121.5,0.,0.));
#70141=CARTESIAN_POINT('',(113.,32.5064359373941,20.6296297263933));
#70142=CARTESIAN_POINT('Origin',(121.7,30.9095636291554,14.5349879826981));
#70143=CARTESIAN_POINT('',(121.7,34.4638925493513,15.6825215664905));
#70144=CARTESIAN_POINT('Origin',(121.7,34.3490875196417,15.9596854262439));
#70145=CARTESIAN_POINT('',(121.7,33.2241144745873,15.1689886735905));
#70146=CARTESIAN_POINT('Origin',(121.7,32.8321455851244,15.3313475036343));
#70147=CARTESIAN_POINT('',(121.7,31.0243686588649,14.2578241229448));
#70148=CARTESIAN_POINT('Ctrl Pts',(121.699999999997,34.4638925493544,15.6825215664918));
#70149=CARTESIAN_POINT('Ctrl Pts',(121.591912387511,34.5638417019577,15.7239218610478));
#70150=CARTESIAN_POINT('Ctrl Pts',(121.483824361119,34.6637904725029,15.7653219973501));
#70151=CARTESIAN_POINT('Ctrl Pts',(121.375735931285,34.7637388706433,15.8067219793973));
#70152=CARTESIAN_POINT('Ctrl Pts',(121.756617543137,34.5161536460432,15.7041688215248));
#70153=CARTESIAN_POINT('Ctrl Pts',(121.648526737397,34.6161000618905,15.7455681418798));
#70154=CARTESIAN_POINT('Ctrl Pts',(121.540435642305,34.7160463736859,15.7869669437042));
#70155=CARTESIAN_POINT('Ctrl Pts',(121.432344074474,34.8159920802211,15.828365967482));
#70156=CARTESIAN_POINT('Ctrl Pts',(121.869288077041,34.5942310582327,15.8098327514129));
#70157=CARTESIAN_POINT('Ctrl Pts',(121.761191184242,34.6941753704096,15.851222755321));
#70158=CARTESIAN_POINT('Ctrl Pts',(121.653093832523,34.7941191828858,15.8926127449365));
#70159=CARTESIAN_POINT('Ctrl Pts',(121.544996282866,34.8940628182975,15.9340026101519));
#70160=CARTESIAN_POINT('Ctrl Pts',(121.913823234176,34.5736426479043,15.9758096616227));
#70161=CARTESIAN_POINT('Ctrl Pts',(121.805730586267,34.6735964016779,16.017188555955));
#70162=CARTESIAN_POINT('Ctrl Pts',(121.697637909656,34.7735500185365,16.0585676499069));
#70163=CARTESIAN_POINT('Ctrl Pts',(121.589544531166,34.8735029323928,16.0999465920823));
#70164=CARTESIAN_POINT('Ctrl Pts',(121.912132034353,34.5414677238746,16.0490714263823));
#70165=CARTESIAN_POINT('Ctrl Pts',(121.804044421867,34.6414276617498,16.0904485084352));
#70166=CARTESIAN_POINT('Ctrl Pts',(121.695956395475,34.7413871209968,16.1318256290849));
#70167=CARTESIAN_POINT('Ctrl Pts',(121.587867965641,34.8413461138118,16.1732027874074));
#70168=CARTESIAN_POINT('',(121.375735931285,34.7637388706433,15.8067219793973));
#70169=CARTESIAN_POINT('',(121.587867965641,34.8413461138104,16.1732027874068));
#70170=CARTESIAN_POINT('Origin',(121.375735931285,34.6489338409337,16.0838858391507));
#70171=CARTESIAN_POINT('',(121.912132034353,34.541467723873,16.0490714263816));
#70172=CARTESIAN_POINT('Ctrl Pts',(121.587867965641,34.8413461138118,16.1732027874074));
#70173=CARTESIAN_POINT('Ctrl Pts',(121.695956395475,34.7413871209968,16.1318256290849));
#70174=CARTESIAN_POINT('Ctrl Pts',(121.804044421867,34.6414276617498,16.0904485084352));
#70175=CARTESIAN_POINT('Ctrl Pts',(121.912132034353,34.5414677238746,16.0490714263823));
#70176=CARTESIAN_POINT('Origin',(121.699999999997,34.3490875196448,15.9596854262451));
#70177=CARTESIAN_POINT('Ctrl Pts',(121.699999999997,34.4638925493544,15.6825215664918));
#70178=CARTESIAN_POINT('Ctrl Pts',(121.591912387511,34.5638417019577,15.7239218610478));
#70179=CARTESIAN_POINT('Ctrl Pts',(121.483824361119,34.6637904725029,15.7653219973501));
#70180=CARTESIAN_POINT('Ctrl Pts',(121.375735931285,34.7637388706433,15.8067219793973));
#70181=CARTESIAN_POINT('Origin',(121.7,34.3490875196417,15.9596854262438));
#70182=CARTESIAN_POINT('Origin',(121.7,34.3490875196417,15.9596854262438));
#70183=CARTESIAN_POINT('Origin',(113.,34.6489338409309,16.0838858391495));
#70184=CARTESIAN_POINT('',(104.188611756946,34.7637388706404,15.8067219793961));
#70185=CARTESIAN_POINT('',(104.5,34.9210458868021,16.210199078724));
#70186=CARTESIAN_POINT('Ctrl Pts',(104.188611312035,34.7637392814463,15.8067221495578));
#70187=CARTESIAN_POINT('Ctrl Pts',(104.19203735624,34.7669063670474,15.8080340048666));
#70188=CARTESIAN_POINT('Ctrl Pts',(104.19544217649,34.7700294887557,15.8093912725525));
#70189=CARTESIAN_POINT('Ctrl Pts',(104.234593964868,34.8056700981812,15.8255965029732));
#70190=CARTESIAN_POINT('Ctrl Pts',(104.273440501065,34.8382691291976,15.8477599864337));
#70191=CARTESIAN_POINT('Ctrl Pts',(104.347490784093,34.8933594144204,15.9054618065867));
#70192=CARTESIAN_POINT('Ctrl Pts',(104.382711610234,34.9159012799814,15.9409298704602));
#70193=CARTESIAN_POINT('Ctrl Pts',(104.43587220677,34.9420564933711,16.0115439385518));
#70194=CARTESIAN_POINT('Ctrl Pts',(104.458840813878,34.9497130192858,16.0499644127093));
#70195=CARTESIAN_POINT('Ctrl Pts',(104.482922171696,34.9484448961684,16.1103022466853));
#70196=CARTESIAN_POINT('Ctrl Pts',(104.489283385678,34.9459601574395,16.1308778312071));
#70197=CARTESIAN_POINT('Ctrl Pts',(104.497821708252,34.9366375420249,16.1713959204003));
#70198=CARTESIAN_POINT('Ctrl Pts',(104.5,34.9298009043927,16.1913384608169));
#70199=CARTESIAN_POINT('Ctrl Pts',(104.5,34.9210458868021,16.210199078724));
#70200=CARTESIAN_POINT('',(121.375735931288,34.9210458868021,16.210199078724));
#70201=CARTESIAN_POINT('',(113.,34.9210458868021,16.210199078724));
#70202=CARTESIAN_POINT('Origin',(121.375735931288,34.6489338409309,16.0838858391495));
#70203=CARTESIAN_POINT('',(113.,34.7637388706404,15.8067219793961));
#70204=CARTESIAN_POINT('Origin',(121.375735931288,34.6489338409309,16.0838858391494));
#70205=CARTESIAN_POINT('Origin',(121.375735931288,34.6489338409309,16.0838858391494));
#70206=CARTESIAN_POINT('Origin',(121.7,0.,0.));
#70207=CARTESIAN_POINT('',(121.912132034353,33.7600976763358,17.6335331415093));
#70208=CARTESIAN_POINT('Origin',(121.912132034356,2.22044604925031E-15,
-3.33066907387547E-15));
#70209=CARTESIAN_POINT('Origin',(121.7,33.5720693465105,17.535322413054));
#70210=CARTESIAN_POINT('Origin',(121.75,0.,0.));
#70211=CARTESIAN_POINT('',(121.587867965644,34.0411321034261,17.7958762791241));
#70212=CARTESIAN_POINT('Origin',(121.587867965644,0.,-2.22044604925031E-15));
#70213=CARTESIAN_POINT('Ctrl Pts',(121.912132034353,33.7600976763372,17.63353314151));
#70214=CARTESIAN_POINT('Ctrl Pts',(121.804044421868,33.8537760772191,17.6876479205194));
#70215=CARTESIAN_POINT('Ctrl Pts',(121.695956395477,33.9474542173515,17.7417622963114));
#70216=CARTESIAN_POINT('Ctrl Pts',(121.587867965644,34.0411321034261,17.7958762791241));
#70217=CARTESIAN_POINT('Origin',(104.3,36.3732017793224,8.08972815424757));
#70218=CARTESIAN_POINT('',(104.3,36.8889585127428,8.53850760858152));
#70219=CARTESIAN_POINT('Origin',(104.3,36.9666042262736,8.2487298606948));
#70220=CARTESIAN_POINT('',(104.3,35.5927574181843,8.19119157206622));
#70221=CARTESIAN_POINT('Origin',(104.3,35.3806253838283,7.82376811064874));
#70222=CARTESIAN_POINT('',(104.3,36.2955560657916,8.37950590213429));
#70223=CARTESIAN_POINT('Origin',(121.7,34.7235679177634,6.18525077844737));
#70224=CARTESIAN_POINT('',(121.7,37.3484991445085,6.22824084226946));
#70225=CARTESIAN_POINT('Origin',(121.7,37.3093412868425,6.5256743006816));
#70226=CARTESIAN_POINT('',(121.7,36.018053390258,6.05308433581784));
#70227=CARTESIAN_POINT('Origin',(121.7,35.6814620741799,6.31135993656396));
#70228=CARTESIAN_POINT('',(121.7,34.7627257754294,5.88781732003522));
#70229=CARTESIAN_POINT('Ctrl Pts',(121.699999999995,37.3484991445135,6.22824084227012));
#70230=CARTESIAN_POINT('Ctrl Pts',(121.591912387509,37.4557577970327,6.24236171176213));
#70231=CARTESIAN_POINT('Ctrl Pts',(121.483824361117,37.5630160395531,6.25648252727677));
#70232=CARTESIAN_POINT('Ctrl Pts',(121.375735931283,37.6702738824338,6.27060329017785));
#70233=CARTESIAN_POINT('Ctrl Pts',(121.756617543135,37.4045822093922,6.23562431783376));
#70234=CARTESIAN_POINT('Ctrl Pts',(121.648526737395,37.5118379662662,6.24974495464447));
#70235=CARTESIAN_POINT('Ctrl Pts',(121.540435642303,37.6190934884284,6.2638651175237));
#70236=CARTESIAN_POINT('Ctrl Pts',(121.432344074473,37.7263484833998,6.27798565144624));
#70237=CARTESIAN_POINT('Ctrl Pts',(121.869288897228,37.5073479950356,6.31747890666536));
#70238=CARTESIAN_POINT('Ctrl Pts',(121.761192004429,37.6145993086462,6.33159108894933));
#70239=CARTESIAN_POINT('Ctrl Pts',(121.653094652113,37.721850135235,6.3457033872055));
#70240=CARTESIAN_POINT('Ctrl Pts',(121.544997102456,37.8291007592444,6.35981561068234));
#70241=CARTESIAN_POINT('Ctrl Pts',(121.913823234174,37.5304181438624,6.48312997219361));
#70242=CARTESIAN_POINT('Ctrl Pts',(121.805730586265,37.6376757019854,6.49722897978641));
#70243=CARTESIAN_POINT('Ctrl Pts',(121.697637909654,37.7449331795239,6.51132821563309));
#70244=CARTESIAN_POINT('Ctrl Pts',(121.589544531165,37.8521899387317,6.52542748682536));
#70245=CARTESIAN_POINT('Ctrl Pts',(121.912132034351,37.5183010937808,6.56222288596809));
#70246=CARTESIAN_POINT('Ctrl Pts',(121.804044421865,37.6255641562348,6.5763185424701));
#70247=CARTESIAN_POINT('Ctrl Pts',(121.695956395473,37.732826766359,6.59041436013177));
#70248=CARTESIAN_POINT('Ctrl Pts',(121.587867965639,37.8400889356949,6.6045103349042));
#70249=CARTESIAN_POINT('',(121.375735931283,37.6702738824338,6.27060329017785));
#70250=CARTESIAN_POINT('',(121.587867965639,37.8400889356926,6.6045103349038));
#70251=CARTESIAN_POINT('Origin',(121.375735931283,37.6311160247677,6.56803674858999));
#70252=CARTESIAN_POINT('',(121.912132034351,37.5183010937783,6.56222288596765));
#70253=CARTESIAN_POINT('Ctrl Pts',(121.587867965639,37.8400889356949,6.6045103349042));
#70254=CARTESIAN_POINT('Ctrl Pts',(121.695956395473,37.732826766359,6.59041436013177));
#70255=CARTESIAN_POINT('Ctrl Pts',(121.804044421865,37.6255641562348,6.5763185424701));
#70256=CARTESIAN_POINT('Ctrl Pts',(121.912132034351,37.5183010937808,6.56222288596809));
#70257=CARTESIAN_POINT('Origin',(121.699999999995,37.3093412868475,6.52567430068227));
#70258=CARTESIAN_POINT('Ctrl Pts',(121.699999999995,37.3484991445135,6.22824084227012));
#70259=CARTESIAN_POINT('Ctrl Pts',(121.591912387509,37.4557577970327,6.24236171176213));
#70260=CARTESIAN_POINT('Ctrl Pts',(121.483824361117,37.5630160395531,6.25648252727677));
#70261=CARTESIAN_POINT('Ctrl Pts',(121.375735931283,37.6702738824338,6.27060329017785));
#70262=CARTESIAN_POINT('Origin',(121.7,37.3093412868425,6.5256743006816));
#70263=CARTESIAN_POINT('Origin',(121.7,37.3093412868425,6.5256743006816));
#70264=CARTESIAN_POINT('Origin',(104.624264068712,0.,0.));
#70265=CARTESIAN_POINT('',(104.412132034356,37.8760832804287,6.39485752451323));
#70266=CARTESIAN_POINT('',(104.412132034356,37.4871203601426,8.3790031942335));
#70267=CARTESIAN_POINT('Origin',(104.412132034356,0.,1.11022302462516E-15));
#70268=CARTESIAN_POINT('',(104.624264068712,37.5728723564378,8.39817021063717));
#70269=CARTESIAN_POINT('Origin',(104.624264068712,37.2800967276863,8.33272992328155));
#70270=CARTESIAN_POINT('',(104.624264068712,37.9266483495649,6.61961818902333));
#70271=CARTESIAN_POINT('Origin',(104.624264068712,0.,0.));
#70272=CARTESIAN_POINT('Ctrl Pts',(104.624264068712,37.9266483495649,6.61961818902332));
#70273=CARTESIAN_POINT('Ctrl Pts',(104.623447602755,37.9267892813573,6.61881072998547));
#70274=CARTESIAN_POINT('Ctrl Pts',(104.622631133477,37.9269269044908,6.61800269007741));
#70275=CARTESIAN_POINT('Ctrl Pts',(104.585817132853,37.9329830074081,6.58154273325167));
#70276=CARTESIAN_POINT('Ctrl Pts',(104.54955560756,37.9325147058957,6.54450780066875));
#70277=CARTESIAN_POINT('Ctrl Pts',(104.476315456228,37.9166957904252,6.46716983723704));
#70278=CARTESIAN_POINT('Ctrl Pts',(104.441383090819,37.9000294072712,6.42873004592974));
#70279=CARTESIAN_POINT('Ctrl Pts',(104.412132034356,37.8760832804287,6.3948575245132));
#70280=CARTESIAN_POINT('Origin',(113.,37.6311160247631,6.56803674858938));
#70281=CARTESIAN_POINT('',(121.375735931288,37.9266483495649,6.61961818902333));
#70282=CARTESIAN_POINT('',(113.,37.9266483495649,6.61961818902333));
#70283=CARTESIAN_POINT('Origin',(121.375735931288,37.6311160247631,6.56803674858938));
#70284=CARTESIAN_POINT('',(104.188611756946,37.6702738824291,6.27060329017723));
#70285=CARTESIAN_POINT('',(113.,37.6702738824291,6.27060329017723));
#70286=CARTESIAN_POINT('Ctrl Pts',(104.188611312035,37.6702743232782,6.27060334821645));
#70287=CARTESIAN_POINT('Ctrl Pts',(104.192037383128,37.6736730528662,6.27105080458017));
#70288=CARTESIAN_POINT('Ctrl Pts',(104.195442206093,37.6770410460372,6.27155350246194));
#70289=CARTESIAN_POINT('Ctrl Pts',(104.234593964868,37.7156614242077,6.27798207968715));
#70290=CARTESIAN_POINT('Ctrl Pts',(104.273440501065,37.7528860018039,6.29095311068323));
#70291=CARTESIAN_POINT('Ctrl Pts',(104.347490784093,37.8210334610709,6.33243037397716));
#70292=CARTESIAN_POINT('Ctrl Pts',(104.382711610234,37.8519870416124,6.3608556287617));
#70293=CARTESIAN_POINT('Ctrl Pts',(104.411969203877,37.8759499647031,6.3946690608327));
#70294=CARTESIAN_POINT('Ctrl Pts',(104.412050624034,37.8760166345656,6.39476325192201));
#70295=CARTESIAN_POINT('Ctrl Pts',(104.412132034356,37.8760832804287,6.39485752451319));
#70296=CARTESIAN_POINT('Origin',(121.375735931288,37.6311160247631,6.56803674858918));
#70297=CARTESIAN_POINT('Origin',(121.375735931288,37.6311160247631,6.56803674858918));
#70298=CARTESIAN_POINT('Ctrl Pts',(104.300000000004,36.8889585127468,8.53850760858258));
#70299=CARTESIAN_POINT('Ctrl Pts',(104.408087612489,36.993456409298,8.56650773557422));
#70300=CARTESIAN_POINT('Ctrl Pts',(104.516175638879,37.0979539064034,8.59450775553469));
#70301=CARTESIAN_POINT('Ctrl Pts',(104.624264068712,37.2024510141555,8.62250767116827));
#70302=CARTESIAN_POINT('Ctrl Pts',(104.243382456864,36.9435980422802,8.55314822639587));
#70303=CARTESIAN_POINT('Ctrl Pts',(104.351473262603,37.0480931745608,8.58114746024157));
#70304=CARTESIAN_POINT('Ctrl Pts',(104.459564357693,37.1525879086301,8.6091470421225));
#70305=CARTESIAN_POINT('Ctrl Pts',(104.567655925523,37.257082297631,8.63714607945698));
#70306=CARTESIAN_POINT('Ctrl Pts',(104.130708900332,37.0698669867127,8.51685469895559));
#70307=CARTESIAN_POINT('Ctrl Pts',(104.23880579313,37.1743547785458,8.5448600434022));
#70308=CARTESIAN_POINT('Ctrl Pts',(104.346903147051,37.2788421636586,8.57286509255704));
#70309=CARTESIAN_POINT('Ctrl Pts',(104.455000696706,37.3833293341471,8.60087013504744));
#70310=CARTESIAN_POINT('Ctrl Pts',(104.086176765825,37.1545715999318,8.37263814546989));
#70311=CARTESIAN_POINT('Ctrl Pts',(104.194269413732,37.2590601192061,8.40065805141547));
#70312=CARTESIAN_POINT('Ctrl Pts',(104.302362090343,37.363548651379,8.42867771564361));
#70313=CARTESIAN_POINT('Ctrl Pts',(104.410455468831,37.4680365334272,8.45669707232343));
#70314=CARTESIAN_POINT('Ctrl Pts',(104.087867965648,37.173644453086,8.29492882695163));
#70315=CARTESIAN_POINT('Ctrl Pts',(104.195955578133,37.2781367752921,8.32295393531765));
#70316=CARTESIAN_POINT('Ctrl Pts',(104.304043604523,37.3826287412732,8.35097872169247));
#70317=CARTESIAN_POINT('Ctrl Pts',(104.412132034356,37.4871203601426,8.3790031942335));
#70318=CARTESIAN_POINT('',(104.624264068712,37.2024510141556,8.62250767116827));
#70319=CARTESIAN_POINT('Origin',(104.624264068712,37.2800967276863,8.33272992328155));
#70320=CARTESIAN_POINT('',(104.087867965648,37.173644453084,8.29492882695118));
#70321=CARTESIAN_POINT('Ctrl Pts',(104.412132034356,37.4871203601426,8.3790031942335));
#70322=CARTESIAN_POINT('Ctrl Pts',(104.304043604523,37.3826287412732,8.35097872169247));
#70323=CARTESIAN_POINT('Ctrl Pts',(104.195955578133,37.2781367752921,8.32295393531765));
#70324=CARTESIAN_POINT('Ctrl Pts',(104.087867965648,37.173644453086,8.29492882695163));
#70325=CARTESIAN_POINT('Origin',(104.300000000004,36.9666042262775,8.24872986069586));
#70326=CARTESIAN_POINT('Ctrl Pts',(104.300000000004,36.8889585127468,8.53850760858258));
#70327=CARTESIAN_POINT('Ctrl Pts',(104.408087612489,36.993456409298,8.56650773557422));
#70328=CARTESIAN_POINT('Ctrl Pts',(104.516175638879,37.0979539064034,8.59450775553469));
#70329=CARTESIAN_POINT('Ctrl Pts',(104.624264068712,37.2024510141555,8.62250767116827));
#70330=CARTESIAN_POINT('Origin',(104.624264068712,37.2800967276863,8.33272992328155));
#70331=CARTESIAN_POINT('Origin',(104.624264068712,37.2800967276863,8.33272992328155));
#70332=CARTESIAN_POINT('Origin',(104.3,36.9666042262735,8.24872986069497));
#70333=CARTESIAN_POINT('Origin',(104.3,36.9666042262735,8.24872986069497));
#70334=CARTESIAN_POINT('Origin',(113.,0.,0.));
#70335=CARTESIAN_POINT('',(121.375735931288,37.5728723564378,8.39817021063717));
#70336=CARTESIAN_POINT('',(113.,37.5728723564378,8.39817021063717));
#70337=CARTESIAN_POINT('Origin',(121.375735931288,0.,0.));
#70338=CARTESIAN_POINT('Origin',(113.,37.2800967276863,8.33272992328155));
#70339=CARTESIAN_POINT('',(121.375735931288,37.2024510141556,8.62250767116828));
#70340=CARTESIAN_POINT('',(113.,37.2024510141556,8.62250767116828));
#70341=CARTESIAN_POINT('Origin',(121.375735931288,37.2800967276863,8.33272992328155));
#70342=CARTESIAN_POINT('Origin',(113.,36.8001647010456,8.51471537844437));
#70343=CARTESIAN_POINT('',(121.7,35.5927574181843,8.19119157206622));
#70344=CARTESIAN_POINT('',(103.5,35.5927574181843,8.19119157206622));
#70345=CARTESIAN_POINT('Origin',(121.7,35.3029796702975,8.11354585853546));
#70346=CARTESIAN_POINT('Ctrl Pts',(121.375735931288,37.2024510141556,8.62250767116828));
#70347=CARTESIAN_POINT('Ctrl Pts',(121.583825474459,37.0012754077709,8.56860282990067));
#70348=CARTESIAN_POINT('Ctrl Pts',(121.79191352265,36.800098358614,8.51469760204339));
#70349=CARTESIAN_POINT('Ctrl Pts',(122.,36.5989197935167,8.46079196799113));
#70350=CARTESIAN_POINT('Origin',(104.3,0.,0.));
#70351=CARTESIAN_POINT('',(104.087868515434,37.5703347737696,6.25744605691556));
#70352=CARTESIAN_POINT('Origin',(104.087867965644,0.,5.55111512312578E-16));
#70353=CARTESIAN_POINT('Ctrl Pts',(104.087868240379,37.570335046313,6.25744609279657));
#70354=CARTESIAN_POINT('Ctrl Pts',(104.061688713442,37.5443644242305,6.25402699553551));
#70355=CARTESIAN_POINT('Ctrl Pts',(104.037012788768,37.5077282445796,6.24920375098241));
#70356=CARTESIAN_POINT('Ctrl Pts',(104.008670719845,37.439866676382,6.240269606039));
#70357=CARTESIAN_POINT('Ctrl Pts',(104.,37.3966300490656,6.23457739606555));
#70358=CARTESIAN_POINT('Ctrl Pts',(104.,37.3598942576647,6.22974103737677));
#70359=CARTESIAN_POINT('Origin',(104.25,0.,0.));
#70360=CARTESIAN_POINT('',(104.25,37.7311721243447,6.27862069582411));
#70361=CARTESIAN_POINT('Ctrl Pts',(121.375735931288,33.7031390339859,17.9574056939141));
#70362=CARTESIAN_POINT('Ctrl Pts',(121.483824361121,33.6094494902625,17.9033140106251));
#70363=CARTESIAN_POINT('Ctrl Pts',(121.591912387512,33.5157595974544,17.8492221257921));
#70364=CARTESIAN_POINT('Ctrl Pts',(121.699999999997,33.4220693465132,17.7951300341907));
#70365=CARTESIAN_POINT('Ctrl Pts',(121.432344074477,33.752120102763,17.9856849271578));
#70366=CARTESIAN_POINT('Ctrl Pts',(121.540435642307,33.6584329578312,17.9315947959052));
#70367=CARTESIAN_POINT('Ctrl Pts',(121.648526737398,33.5647456205277,17.8775040493508));
#70368=CARTESIAN_POINT('Ctrl Pts',(121.756617543138,33.4710578085036,17.8234135359081));
#70369=CARTESIAN_POINT('Ctrl Pts',(121.544996182435,33.8834537221696,17.9833149249054));
#70370=CARTESIAN_POINT('Ctrl Pts',(121.653093732091,33.7897751040339,17.929220861406));
#70371=CARTESIAN_POINT('Ctrl Pts',(121.761191083735,33.6960962793851,17.8751267330704));
#70372=CARTESIAN_POINT('Ctrl Pts',(121.869287976533,33.6024171392287,17.821032217088));
#70373=CARTESIAN_POINT('Ctrl Pts',(121.589544531169,34.0025898869996,17.8659835447083));
#70374=CARTESIAN_POINT('Ctrl Pts',(121.697637909658,33.908914286335,17.8118754705986));
#70375=CARTESIAN_POINT('Ctrl Pts',(121.805730586268,33.8152381372974,17.7577669311554));
#70376=CARTESIAN_POINT('Ctrl Pts',(121.913823234176,33.72156206328,17.7036581615694));
#70377=CARTESIAN_POINT('Ctrl Pts',(121.587867965644,34.0411321034261,17.7958762791241));
#70378=CARTESIAN_POINT('Ctrl Pts',(121.695956395477,33.9474542173515,17.7417622963114));
#70379=CARTESIAN_POINT('Ctrl Pts',(121.804044421868,33.8537760772191,17.6876479205194));
#70380=CARTESIAN_POINT('Ctrl Pts',(121.912132034353,33.7600976763372,17.63353314151));
#70381=CARTESIAN_POINT('',(121.699999999997,33.4220693465132,17.7951300341907));
#70382=CARTESIAN_POINT('Origin',(121.699999999997,33.5720693465132,17.5353224130554));
#70383=CARTESIAN_POINT('',(121.375735931288,33.7031390339859,17.9574056939141));
#70384=CARTESIAN_POINT('Origin',(121.375735931288,33.8531390339859,17.6975980727788));
#70385=CARTESIAN_POINT('Ctrl Pts',(121.375735931288,33.7031390339859,17.9574056939141));
#70386=CARTESIAN_POINT('Ctrl Pts',(121.483824361121,33.6094494902625,17.9033140106251));
#70387=CARTESIAN_POINT('Ctrl Pts',(121.591912387512,33.5157595974544,17.8492221257921));
#70388=CARTESIAN_POINT('Ctrl Pts',(121.699999999997,33.4220693465132,17.7951300341907));
#70389=CARTESIAN_POINT('Origin',(121.375735931288,0.,0.));
#70390=CARTESIAN_POINT('',(121.375735931288,34.1190013824203,17.8365844450781));
#70391=CARTESIAN_POINT('Origin',(121.375735931288,0.,0.));
#70392=CARTESIAN_POINT('Origin',(121.375735931288,33.8531390339859,17.6975980727788));
#70393=CARTESIAN_POINT('Origin',(121.375735931288,33.8531390339859,17.6975980727788));
#70394=CARTESIAN_POINT('Origin',(121.375735931288,33.8531390339859,17.6975980727788));
#70395=CARTESIAN_POINT('Origin',(121.7,29.5212294964313,15.1965689351665));
#70396=CARTESIAN_POINT('Origin',(121.7,33.5720693465106,17.5353224130539));
#70397=CARTESIAN_POINT('',(121.7,32.259927238132,17.1241669750802));
#70398=CARTESIAN_POINT('',(121.7,29.3712294964313,15.4563765563018));
#70399=CARTESIAN_POINT('Origin',(121.7,32.1501196169967,16.7143593539449));
#70400=CARTESIAN_POINT('Origin',(121.7,33.5720693465105,17.535322413054));
#70401=CARTESIAN_POINT('Origin',(113.,34.3789638902265,15.6473429640468));
#70402=CARTESIAN_POINT('',(104.3,33.2241144745873,15.1689886735905));
#70403=CARTESIAN_POINT('',(103.5,33.2241144745873,15.1689886735905));
#70404=CARTESIAN_POINT('Origin',(104.3,32.946950614834,15.0541836438809));
#70405=CARTESIAN_POINT('',(104.087868515434,34.6706104470789,15.7681469233145));
#70406=CARTESIAN_POINT('Ctrl Pts',(104.087868240379,34.6706107010489,15.7681470285123));
#70407=CARTESIAN_POINT('Ctrl Pts',(104.061688713442,34.6464099339429,15.7581227425572));
#70408=CARTESIAN_POINT('Ctrl Pts',(104.037012788768,34.612270449391,15.7439817050434));
#70409=CARTESIAN_POINT('Ctrl Pts',(104.008670719845,34.5490335349196,15.7177881174267));
#70410=CARTESIAN_POINT('Ctrl Pts',(104.,34.5087434123029,15.7010994022092));
#70411=CARTESIAN_POINT('Ctrl Pts',(104.,34.4745111043772,15.686919915995));
#70412=CARTESIAN_POINT('',(104.25,34.8204869980086,15.8302278233913));
#70413=CARTESIAN_POINT('Ctrl Pts',(104.624264068712,32.4031390339858,20.2090717437536));
#70414=CARTESIAN_POINT('Ctrl Pts',(104.516175638879,32.3094494902624,20.1549800604647));
#70415=CARTESIAN_POINT('Ctrl Pts',(104.408087612488,32.2157595974544,20.1008881756316));
#70416=CARTESIAN_POINT('Ctrl Pts',(104.300000000003,32.1220693465131,20.0467960840302));
#70417=CARTESIAN_POINT('Ctrl Pts',(104.567655925523,32.452120102763,20.2373509769973));
#70418=CARTESIAN_POINT('Ctrl Pts',(104.459564357693,32.3584331025383,20.1832605951046));
#70419=CARTESIAN_POINT('Ctrl Pts',(104.351473262602,32.2647454732608,20.1291703542641));
#70420=CARTESIAN_POINT('Ctrl Pts',(104.243382456862,32.1710578085036,20.0750795857476));
#70421=CARTESIAN_POINT('Ctrl Pts',(104.455001730448,32.5157376683243,20.352272791064));
#70422=CARTESIAN_POINT('Ctrl Pts',(104.346904180792,32.4220515260722,20.2981917597167));
#70423=CARTESIAN_POINT('Ctrl Pts',(104.238806827625,32.3283652263742,20.2441105815259));
#70424=CARTESIAN_POINT('Ctrl Pts',(104.130709934827,32.2346784312498,20.1900293243369));
#70425=CARTESIAN_POINT('Ctrl Pts',(104.410455468831,32.473690556812,20.5141148642513));
#70426=CARTESIAN_POINT('Ctrl Pts',(104.302362090342,32.3799937897508,20.4600434514159));
#70427=CARTESIAN_POINT('Ctrl Pts',(104.194269413732,32.2862963455125,20.4059717963423));
#70428=CARTESIAN_POINT('Ctrl Pts',(104.086176765824,32.1925987394748,20.3519003213094));
#70429=CARTESIAN_POINT('Ctrl Pts',(104.412132034356,32.4322469920394,20.5825470355869));
#70430=CARTESIAN_POINT('Ctrl Pts',(104.304043604523,32.3385439651864,20.5284765978799));
#70431=CARTESIAN_POINT('Ctrl Pts',(104.195955578132,32.2448404709744,20.4744061366419));
#70432=CARTESIAN_POINT('Ctrl Pts',(104.087867965647,32.1511364971911,20.4203356511969));
#70433=CARTESIAN_POINT('',(104.300000000003,32.1220693465131,20.0467960840302));
#70434=CARTESIAN_POINT('Origin',(104.300000000003,31.9720693465131,20.3066037051655));
#70435=CARTESIAN_POINT('',(104.624264068712,32.4031390339859,20.2090717437536));
#70436=CARTESIAN_POINT('Origin',(104.624264068712,32.2531390339858,20.468879364889));
#70437=CARTESIAN_POINT('Ctrl Pts',(104.624264068712,32.4031390339858,20.2090717437536));
#70438=CARTESIAN_POINT('Ctrl Pts',(104.516175638879,32.3094494902624,20.1549800604647));
#70439=CARTESIAN_POINT('Ctrl Pts',(104.408087612488,32.2157595974544,20.1008881756316));
#70440=CARTESIAN_POINT('Ctrl Pts',(104.300000000003,32.1220693465131,20.0467960840302));
#70441=CARTESIAN_POINT('Origin',(104.3,29.7962294964313,19.0503819820073));
#70442=CARTESIAN_POINT('Origin',(104.3,31.9720693465106,20.3066037051641));
#70443=CARTESIAN_POINT('',(104.3,30.959927238132,19.3758330249198));
#70444=CARTESIAN_POINT('',(104.3,29.9462294964313,18.7905743608719));
#70445=CARTESIAN_POINT('Origin',(104.3,30.5501196169967,19.4856406460551));
#70446=CARTESIAN_POINT('Origin',(104.3,31.9720693465106,20.3066037051641));
#70447=CARTESIAN_POINT('Origin',(104.624264068712,32.2531390339859,20.468879364889));
#70448=CARTESIAN_POINT('Origin',(104.624264068712,32.2531390339859,20.468879364889));
#70449=CARTESIAN_POINT('Origin',(113.,30.7404784537055,21.9493846027006));
#70450=CARTESIAN_POINT('',(121.7,29.7487867783414,21.1884328164397));
#70451=CARTESIAN_POINT('',(103.5,29.7487867783414,21.1884328164397));
#70452=CARTESIAN_POINT('Origin',(121.7,29.5107807762541,21.0058043877371));
#70453=CARTESIAN_POINT('',(121.912131484566,30.9909210297353,22.1415559502273));
#70454=CARTESIAN_POINT('Ctrl Pts',(121.912131759621,30.9909212478242,22.1415561175728));
#70455=CARTESIAN_POINT('Ctrl Pts',(121.938311286558,30.9701395779793,22.1256097814455));
#70456=CARTESIAN_POINT('Ctrl Pts',(121.962987211232,30.9408233379805,22.1031146393084));
#70457=CARTESIAN_POINT('Ctrl Pts',(121.991329280155,30.8865205684525,22.0614466587275));
#70458=CARTESIAN_POINT('Ctrl Pts',(122.,30.8519226558093,22.0348987466286));
#70459=CARTESIAN_POINT('Ctrl Pts',(122.,30.8225267065723,22.0123424414419));
#70460=CARTESIAN_POINT('',(121.75,31.1196229417564,22.2403124007256));
#70461=CARTESIAN_POINT('Origin',(104.3,4.37369830660543,20.9634607793525));
#70462=CARTESIAN_POINT('',(104.3,6.22824084226947,37.3484991445085));
#70463=CARTESIAN_POINT('Origin',(104.3,6.52567430068161,37.3093412868425));
#70464=CARTESIAN_POINT('',(104.3,6.05308433581784,36.018053390258));
#70465=CARTESIAN_POINT('Origin',(104.3,6.31135993656397,35.6814620741799));
#70466=CARTESIAN_POINT('',(104.3,4.07626484819328,21.0026186370186));
#70467=CARTESIAN_POINT('Ctrl Pts',(104.300000000005,6.22824084227012,37.3484991445135));
#70468=CARTESIAN_POINT('Ctrl Pts',(104.408087612491,6.24236171176213,37.4557577970327));
#70469=CARTESIAN_POINT('Ctrl Pts',(104.516175638883,6.25648252727678,37.5630160395531));
#70470=CARTESIAN_POINT('Ctrl Pts',(104.624264068717,6.27060329017785,37.6702738824337));
#70471=CARTESIAN_POINT('Ctrl Pts',(104.243382456864,6.23562431783376,37.4045822093922));
#70472=CARTESIAN_POINT('Ctrl Pts',(104.351473262605,6.24974495464448,37.5118379662662));
#70473=CARTESIAN_POINT('Ctrl Pts',(104.459564357697,6.26386511752371,37.6190934884283));
#70474=CARTESIAN_POINT('Ctrl Pts',(104.567655925527,6.27798565144625,37.7263484833998));
#70475=CARTESIAN_POINT('Ctrl Pts',(104.130708651008,6.31747589142946,37.5073508627116));
#70476=CARTESIAN_POINT('Ctrl Pts',(104.238805543807,6.33158807371344,37.6146021763222));
#70477=CARTESIAN_POINT('Ctrl Pts',(104.346902897911,6.34570037330174,37.7218530009716));
#70478=CARTESIAN_POINT('Ctrl Pts',(104.455000447568,6.35981259677858,37.829103624981));
#70479=CARTESIAN_POINT('Ctrl Pts',(104.086176765826,6.48312997219361,37.5304181438623));
#70480=CARTESIAN_POINT('Ctrl Pts',(104.194269413735,6.49722897978642,37.6376757019854));
#70481=CARTESIAN_POINT('Ctrl Pts',(104.302362090346,6.51132821563309,37.7449331795239));
#70482=CARTESIAN_POINT('Ctrl Pts',(104.410455468835,6.52542748682536,37.8521899387317));
#70483=CARTESIAN_POINT('Ctrl Pts',(104.087867965649,6.56222288596809,37.5183010937808));
#70484=CARTESIAN_POINT('Ctrl Pts',(104.195955578135,6.57631854247011,37.6255641562347));
#70485=CARTESIAN_POINT('Ctrl Pts',(104.304043604527,6.59041436013178,37.732826766359));
#70486=CARTESIAN_POINT('Ctrl Pts',(104.412132034361,6.60451033490421,37.8400889356949));
#70487=CARTESIAN_POINT('',(104.624264068717,6.27060329017785,37.6702738824337));
#70488=CARTESIAN_POINT('',(104.412132034361,6.6045103349038,37.8400889356926));
#70489=CARTESIAN_POINT('Origin',(104.624264068717,6.56803674859,37.6311160247677));
#70490=CARTESIAN_POINT('',(104.087867965649,6.56222288596766,37.5183010937783));
#70491=CARTESIAN_POINT('Ctrl Pts',(104.412132034361,6.60451033490421,37.8400889356949));
#70492=CARTESIAN_POINT('Ctrl Pts',(104.304043604527,6.59041436013178,37.732826766359));
#70493=CARTESIAN_POINT('Ctrl Pts',(104.195955578135,6.57631854247011,37.6255641562347));
#70494=CARTESIAN_POINT('Ctrl Pts',(104.087867965649,6.56222288596809,37.5183010937808));
#70495=CARTESIAN_POINT('Origin',(104.300000000005,6.52567430068227,37.3093412868475));
#70496=CARTESIAN_POINT('Ctrl Pts',(104.300000000005,6.22824084227012,37.3484991445135));
#70497=CARTESIAN_POINT('Ctrl Pts',(104.408087612491,6.24236171176213,37.4557577970327));
#70498=CARTESIAN_POINT('Ctrl Pts',(104.516175638883,6.25648252727678,37.5630160395531));
#70499=CARTESIAN_POINT('Ctrl Pts',(104.624264068717,6.27060329017785,37.6702738824337));
#70500=CARTESIAN_POINT('Origin',(104.3,6.52567430068161,37.3093412868425));
#70501=CARTESIAN_POINT('Origin',(104.3,6.52567430068161,37.3093412868425));
#70502=CARTESIAN_POINT('Origin',(113.,6.56803674858938,37.6311160247631));
#70503=CARTESIAN_POINT('',(121.811388243054,6.27060329017724,37.6702738824291));
#70504=CARTESIAN_POINT('',(121.5,6.61961818902333,37.9266483495649));
#70505=CARTESIAN_POINT('Ctrl Pts',(121.811388687965,6.27060334821645,37.6702743232782));
#70506=CARTESIAN_POINT('Ctrl Pts',(121.80796264376,6.2710508010685,37.6736730261927));
#70507=CARTESIAN_POINT('Ctrl Pts',(121.80455782351,6.27155349760121,37.6770410168358));
#70508=CARTESIAN_POINT('Ctrl Pts',(121.765406035132,6.27798207968715,37.7156614242077));
#70509=CARTESIAN_POINT('Ctrl Pts',(121.726559498935,6.29095311068322,37.7528860018039));
#70510=CARTESIAN_POINT('Ctrl Pts',(121.652509215907,6.33243037397716,37.8210334610709));
#70511=CARTESIAN_POINT('Ctrl Pts',(121.617288389766,6.3608556287617,37.8519870416124));
#70512=CARTESIAN_POINT('Ctrl Pts',(121.56412779323,6.42229411347668,37.8955273033918));
#70513=CARTESIAN_POINT('Ctrl Pts',(121.541159186122,6.45742378699771,37.9128668899463));
#70514=CARTESIAN_POINT('Ctrl Pts',(121.517077828304,6.5160338735518,37.9272585576496));
#70515=CARTESIAN_POINT('Ctrl Pts',(121.510716614322,6.53655145973753,37.930183837478));
#70516=CARTESIAN_POINT('Ctrl Pts',(121.502178291748,6.57810179894057,37.9316657356349));
#70517=CARTESIAN_POINT('Ctrl Pts',(121.5,6.59913426579451,37.9302235600485));
#70518=CARTESIAN_POINT('Ctrl Pts',(121.5,6.61961818902333,37.9266483495649));
#70519=CARTESIAN_POINT('',(104.624264068712,6.61961818902333,37.9266483495649));
#70520=CARTESIAN_POINT('',(113.,6.61961818902333,37.9266483495649));
#70521=CARTESIAN_POINT('Origin',(104.624264068712,6.56803674858938,37.6311160247631));
#70522=CARTESIAN_POINT('',(113.,6.27060329017724,37.6702738824291));
#70523=CARTESIAN_POINT('Origin',(104.624264068712,6.56803674858919,37.6311160247631));
#70524=CARTESIAN_POINT('Origin',(104.624264068712,6.56803674858919,37.6311160247631));
#70525=CARTESIAN_POINT('Origin',(104.3,0.,0.));
#70526=CARTESIAN_POINT('',(104.087867965648,8.29492882695119,37.173644453084));
#70527=CARTESIAN_POINT('Origin',(104.087867965644,-1.66533453693773E-15,
0.));
#70528=CARTESIAN_POINT('Origin',(104.3,8.24872986069481,36.9666042262736));
#70529=CARTESIAN_POINT('Origin',(104.25,0.,0.));
#70530=CARTESIAN_POINT('',(104.412132034356,8.37900319423351,37.4871203601426));
#70531=CARTESIAN_POINT('Origin',(104.412132034356,-1.66533453693773E-15,
0.));
#70532=CARTESIAN_POINT('Ctrl Pts',(104.087867965648,8.29492882695164,37.173644453086));
#70533=CARTESIAN_POINT('Ctrl Pts',(104.195955578133,8.32295393531766,37.2781367752921));
#70534=CARTESIAN_POINT('Ctrl Pts',(104.304043604523,8.35097872169249,37.3826287412732));
#70535=CARTESIAN_POINT('Ctrl Pts',(104.412132034356,8.37900319423351,37.4871203601426));
#70536=CARTESIAN_POINT('Origin',(104.624264068712,0.,0.));
#70537=CARTESIAN_POINT('',(104.624264068712,8.39817021063718,37.5728723564378));
#70538=CARTESIAN_POINT('Origin',(104.624264068712,0.,0.));
#70539=CARTESIAN_POINT('Origin',(104.624264068712,8.33272992328157,37.2800967276863));
#70540=CARTESIAN_POINT('Origin',(113.,0.,0.));
#70541=CARTESIAN_POINT('',(121.5,8.39817021063718,37.5728723564378));
#70542=CARTESIAN_POINT('Origin',(121.5,0.,0.));
#70543=CARTESIAN_POINT('',(113.,8.39817021063718,37.5728723564378));
#70544=CARTESIAN_POINT('Ctrl Pts',(104.624264068712,22.2029200028051,31.0708922200351));
#70545=CARTESIAN_POINT('Ctrl Pts',(104.516175638879,22.1370621419721,30.9850645847965));
#70546=CARTESIAN_POINT('Ctrl Pts',(104.408087612488,22.0712040357546,30.8992366297665));
#70547=CARTESIAN_POINT('Ctrl Pts',(104.300000000003,22.0053456777918,30.8134083466558));
#70548=CARTESIAN_POINT('Ctrl Pts',(104.567655925523,22.2373506156865,31.1157630683446));
#70549=CARTESIAN_POINT('Ctrl Pts',(104.459564357693,22.1714946067171,31.0299376087941));
#70550=CARTESIAN_POINT('Ctrl Pts',(104.351473262602,22.1056379626004,30.9441120388309));
#70551=CARTESIAN_POINT('Ctrl Pts',(104.243382456862,22.0397814876375,30.8582859677811));
#70552=CARTESIAN_POINT('Ctrl Pts',(104.455001803843,22.252146783607,31.2462823716862));
#70553=CARTESIAN_POINT('Ctrl Pts',(104.346904254187,22.186287989002,31.1604658792452));
#70554=CARTESIAN_POINT('Ctrl Pts',(104.238806901073,22.1204291050614,31.0746491908737));
#70555=CARTESIAN_POINT('Ctrl Pts',(104.130710008275,22.054569793707,30.9888322399387));
#70556=CARTESIAN_POINT('Ctrl Pts',(104.410455468831,22.1513661623602,31.37971421451));
#70557=CARTESIAN_POINT('Ctrl Pts',(104.302362090342,22.0854938708666,31.2939025424768));
#70558=CARTESIAN_POINT('Ctrl Pts',(104.194269413732,22.0196210464434,31.2080903875002));
#70559=CARTESIAN_POINT('Ctrl Pts',(104.086176765824,21.9537480036384,31.1222783369417));
#70560=CARTESIAN_POINT('Ctrl Pts',(104.412132034356,22.0868894429017,31.4270775313556));
#70561=CARTESIAN_POINT('Ctrl Pts',(104.304043604523,22.0210109949489,31.341264364705));
#70562=CARTESIAN_POINT('Ctrl Pts',(104.195955578132,21.9551321242177,31.2554509974641));
#70563=CARTESIAN_POINT('Ctrl Pts',(104.087867965647,21.8892528196841,31.1696374243348));
#70564=CARTESIAN_POINT('',(104.300000000003,22.0053456777918,30.8134083466558));
#70565=CARTESIAN_POINT('Origin',(104.300000000003,21.7673396757045,30.9960367753584));
#70566=CARTESIAN_POINT('',(104.624264068712,22.2029200028051,31.0708922200351));
#70567=CARTESIAN_POINT('Origin',(104.624264068712,21.9649140007177,31.2535206487377));
#70568=CARTESIAN_POINT('Ctrl Pts',(104.624264068712,22.2029200028051,31.0708922200351));
#70569=CARTESIAN_POINT('Ctrl Pts',(104.516175638879,22.1370621419721,30.9850645847965));
#70570=CARTESIAN_POINT('Ctrl Pts',(104.408087612488,22.0712040357546,30.8992366297665));
#70571=CARTESIAN_POINT('Ctrl Pts',(104.300000000003,22.0053456777918,30.8134083466558));
#70572=CARTESIAN_POINT('Origin',(104.3,17.2622256995997,25.1248579341572));
#70573=CARTESIAN_POINT('Origin',(104.3,21.7673396757028,30.9960367753563));
#70574=CARTESIAN_POINT('',(104.3,21.1884328164397,29.7487867783414));
#70575=CARTESIAN_POINT('',(104.3,17.500231701687,24.9422295054545));
#70576=CARTESIAN_POINT('Origin',(104.3,20.7677983856497,29.6934092049567));
#70577=CARTESIAN_POINT('Origin',(104.3,21.7673396757028,30.9960367753563));
#70578=CARTESIAN_POINT('Origin',(104.624264068712,21.9649140007177,31.2535206487377));
#70579=CARTESIAN_POINT('Origin',(104.624264068712,21.9649140007177,31.2535206487377));
#70580=CARTESIAN_POINT('Origin',(113.,20.0008330249198,32.0424589928626));
#70581=CARTESIAN_POINT('',(121.7,19.3758330249198,30.959927238132));
#70582=CARTESIAN_POINT('',(103.5,19.3758330249198,30.959927238132));
#70583=CARTESIAN_POINT('Origin',(121.7,19.2258330249198,30.7001196169967));
#70584=CARTESIAN_POINT('',(121.912131484566,20.1586710041094,32.315842392183));
#70585=CARTESIAN_POINT('Ctrl Pts',(121.912131759621,20.158671141557,32.3158426302491));
#70586=CARTESIAN_POINT('Ctrl Pts',(121.938311286558,20.1455737807786,32.293157335936));
#70587=CARTESIAN_POINT('Ctrl Pts',(121.962987211232,20.1270976248782,32.2611556951879));
#70588=CARTESIAN_POINT('Ctrl Pts',(121.991329280155,20.0928740533809,32.2018787305382));
#70589=CARTESIAN_POINT('Ctrl Pts',(122.,20.0710691961464,32.1641116099562));
#70590=CARTESIAN_POINT('Ctrl Pts',(122.,20.052542804598,32.1320229585134));
#70591=CARTESIAN_POINT('',(121.75,20.2397836089759,32.4563335449461));
#70592=CARTESIAN_POINT('Origin',(121.7,20.4652696449976,22.7280113447946));
#70593=CARTESIAN_POINT('',(121.7,25.8390437558097,27.6775213868948));
#70594=CARTESIAN_POINT('Origin',(121.7,25.6269117214538,27.8896534212507));
#70595=CARTESIAN_POINT('',(121.7,24.8901586977665,26.7286363288515));
#70596=CARTESIAN_POINT('Origin',(121.7,24.4658946290545,26.7286363288515));
#70597=CARTESIAN_POINT('',(121.7,20.6774016793536,22.5158793104386));
#70598=CARTESIAN_POINT('Ctrl Pts',(121.699999999998,25.8390437558114,27.6775213868965));
#70599=CARTESIAN_POINT('Ctrl Pts',(121.591912387512,25.9155415253719,27.7540191564569));
#70600=CARTESIAN_POINT('Ctrl Pts',(121.48382436112,25.9920390025178,27.8305166336028));
#70601=CARTESIAN_POINT('Ctrl Pts',(121.375735931286,26.0685361946373,27.9070138257223));
#70602=CARTESIAN_POINT('Ctrl Pts',(121.756617543138,25.8790426675315,27.7175202986166));
#70603=CARTESIAN_POINT('Ctrl Pts',(121.648526737398,25.9555382814697,27.7940161208215));
#70604=CARTESIAN_POINT('Ctrl Pts',(121.540435642306,26.0320339977095,27.8705114241477));
#70605=CARTESIAN_POINT('Ctrl Pts',(121.432344074475,26.108529069824,27.947006700909));
#70606=CARTESIAN_POINT('Ctrl Pts',(121.869287690755,25.910740307588,27.8450200746977));
#70607=CARTESIAN_POINT('Ctrl Pts',(121.761190797956,25.987237543238,27.9215064845882));
#70608=CARTESIAN_POINT('Ctrl Pts',(121.653093446519,26.0637343230645,27.9979926900665));
#70609=CARTESIAN_POINT('Ctrl Pts',(121.544995896862,26.1402309865404,28.0744787128348));
#70610=CARTESIAN_POINT('Ctrl Pts',(121.913823234177,25.8282031306362,27.9904837995326));
#70611=CARTESIAN_POINT('Ctrl Pts',(121.805730586268,25.9047133406349,28.0669635586561));
#70612=CARTESIAN_POINT('Ctrl Pts',(121.697637909656,25.9812233477494,28.1434434498089));
#70613=CARTESIAN_POINT('Ctrl Pts',(121.589544531167,26.0577327634567,28.2199229317112));
#70614=CARTESIAN_POINT('Ctrl Pts',(121.912132034354,25.7704413132658,28.0458560341459));
#70615=CARTESIAN_POINT('Ctrl Pts',(121.804044421868,25.8469579301585,28.1223364854948));
#70616=CARTESIAN_POINT('Ctrl Pts',(121.695956395476,25.9234740900862,28.1988167893393));
#70617=CARTESIAN_POINT('Ctrl Pts',(121.587867965642,25.9999898046701,28.2752969494932));
#70618=CARTESIAN_POINT('',(121.375735931286,26.0685361946373,27.9070138257223));
#70619=CARTESIAN_POINT('',(121.587867965642,25.9999898046693,28.2752969494924));
#70620=CARTESIAN_POINT('Origin',(121.375735931286,25.8564041602813,28.1191458600783));
#70621=CARTESIAN_POINT('',(121.912132034354,25.770441313265,28.0458560341451));
#70622=CARTESIAN_POINT('Ctrl Pts',(121.587867965642,25.9999898046701,28.2752969494932));
#70623=CARTESIAN_POINT('Ctrl Pts',(121.695956395476,25.9234740900862,28.1988167893393));
#70624=CARTESIAN_POINT('Ctrl Pts',(121.804044421868,25.8469579301585,28.1223364854948));
#70625=CARTESIAN_POINT('Ctrl Pts',(121.912132034354,25.7704413132658,28.0458560341459));
#70626=CARTESIAN_POINT('Origin',(121.699999999998,25.6269117214555,27.8896534212524));
#70627=CARTESIAN_POINT('Ctrl Pts',(121.699999999998,25.8390437558114,27.6775213868965));
#70628=CARTESIAN_POINT('Ctrl Pts',(121.591912387512,25.9155415253719,27.7540191564569));
#70629=CARTESIAN_POINT('Ctrl Pts',(121.48382436112,25.9920390025178,27.8305166336028));
#70630=CARTESIAN_POINT('Ctrl Pts',(121.375735931286,26.0685361946373,27.9070138257223));
#70631=CARTESIAN_POINT('Origin',(121.7,25.6269117214538,27.8896534212507));
#70632=CARTESIAN_POINT('Origin',(121.7,25.6269117214538,27.8896534212507));
#70633=CARTESIAN_POINT('Origin',(113.,25.8564041602797,28.1191458600767));
#70634=CARTESIAN_POINT('',(104.188611756946,26.0685361946357,27.9070138257207));
#70635=CARTESIAN_POINT('',(104.5,26.0594649259364,28.3399768485066));
#70636=CARTESIAN_POINT('Ctrl Pts',(104.188611312035,26.0685365090528,27.9070141401383));
#70637=CARTESIAN_POINT('Ctrl Pts',(104.19203735624,26.070960489325,27.9094381275961));
#70638=CARTESIAN_POINT('Ctrl Pts',(104.19544217649,26.0733264736922,27.9118872463663));
#70639=CARTESIAN_POINT('Ctrl Pts',(104.234593964868,26.100052630067,27.9404979978181));
#70640=CARTESIAN_POINT('Ctrl Pts',(104.273440501065,26.1216886096789,27.9734494956375));
#70641=CARTESIAN_POINT('Ctrl Pts',(104.347490784093,26.1505038660466,28.0478411657046));
#70642=CARTESIAN_POINT('Ctrl Pts',(104.382711610234,26.1577567938406,28.0892357824599));
#70643=CARTESIAN_POINT('Ctrl Pts',(104.43587220677,26.1548982262093,28.1644838415113));
#70644=CARTESIAN_POINT('Ctrl Pts',(104.458840813878,26.1472690548682,28.2029097568319));
#70645=CARTESIAN_POINT('Ctrl Pts',(104.482922171696,26.123007172468,28.2581693569711));
#70646=CARTESIAN_POINT('Ctrl Pts',(104.489283385678,26.1128376379049,28.2762278500349));
#70647=CARTESIAN_POINT('Ctrl Pts',(104.497821708252,26.0887190628886,28.3100940728715));
#70648=CARTESIAN_POINT('Ctrl Pts',(104.5,26.0747711534923,28.3259023098338));
#70649=CARTESIAN_POINT('Ctrl Pts',(104.5,26.0594649259364,28.3399768485066));
#70650=CARTESIAN_POINT('',(121.375735931288,26.0594649259364,28.3399768485066));
#70651=CARTESIAN_POINT('',(113.,26.0594649259364,28.3399768485066));
#70652=CARTESIAN_POINT('Origin',(121.375735931288,25.8564041602797,28.1191458600767));
#70653=CARTESIAN_POINT('',(113.,26.0685361946357,27.9070138257207));
#70654=CARTESIAN_POINT('Origin',(121.375735931288,25.8564041602798,28.1191458600766));
#70655=CARTESIAN_POINT('Origin',(121.375735931288,25.8564041602798,28.1191458600766));
#70656=CARTESIAN_POINT('Origin',(121.7,0.,0.));
#70657=CARTESIAN_POINT('',(121.912132034353,24.4422022714321,29.2106904110607));
#70658=CARTESIAN_POINT('Origin',(121.912132034356,2.22044604925031E-15,
-2.22044604925031E-15));
#70659=CARTESIAN_POINT('Origin',(121.7,24.3060703646347,29.0480002025285));
#70660=CARTESIAN_POINT('Origin',(121.75,0.,0.));
#70661=CARTESIAN_POINT('',(121.587867965644,24.6397181974285,29.4682231323184));
#70662=CARTESIAN_POINT('Origin',(121.587867965644,2.22044604925031E-15,
-2.22044604925031E-15));
#70663=CARTESIAN_POINT('Ctrl Pts',(121.912132034353,24.4422022714329,29.2106904110617));
#70664=CARTESIAN_POINT('Ctrl Pts',(121.804044421868,24.5080409992732,29.2965351197829));
#70665=CARTESIAN_POINT('Ctrl Pts',(121.695956395477,24.573879640517,29.3823793561953));
#70666=CARTESIAN_POINT('Ctrl Pts',(121.587867965644,24.6397181974285,29.4682231323184));
#70667=CARTESIAN_POINT('Ctrl Pts',(104.624264068712,29.4881125046124,24.2656386875623));
#70668=CARTESIAN_POINT('Ctrl Pts',(104.516175638879,29.4022848693738,24.1997808267293));
#70669=CARTESIAN_POINT('Ctrl Pts',(104.408087612488,29.3164569143438,24.1339227205117));
#70670=CARTESIAN_POINT('Ctrl Pts',(104.300000000003,29.2306286312331,24.068064362549));
#70671=CARTESIAN_POINT('Ctrl Pts',(104.567655925523,29.5329833529219,24.3000693004437));
#70672=CARTESIAN_POINT('Ctrl Pts',(104.459564357693,29.4471580695557,24.2342130618665));
#70673=CARTESIAN_POINT('Ctrl Pts',(104.351473262602,29.3613321441074,24.1683568810269));
#70674=CARTESIAN_POINT('Ctrl Pts',(104.243382456862,29.2755062523583,24.1025001723946));
#70675=CARTESIAN_POINT('Ctrl Pts',(104.455001885058,29.5810561028804,24.4223117753432));
#70676=CARTESIAN_POINT('Ctrl Pts',(104.346904335402,29.4952304496556,24.3564649193042));
#70677=CARTESIAN_POINT('Ctrl Pts',(104.238806982348,29.4094046593508,24.2906178971386));
#70678=CARTESIAN_POINT('Ctrl Pts',(104.13071008955,29.3235783883173,24.224770731973));
#70679=CARTESIAN_POINT('Ctrl Pts',(104.410455468831,29.518244332399,24.577280943507));
#70680=CARTESIAN_POINT('Ctrl Pts',(104.302362090342,29.4324068897941,24.5114422368762));
#70681=CARTESIAN_POINT('Ctrl Pts',(104.194269413731,29.3465688074239,24.4456032016902));
#70682=CARTESIAN_POINT('Ctrl Pts',(104.086176765824,29.2607305411385,24.3797643238856));
#70683=CARTESIAN_POINT('Ctrl Pts',(104.412132034356,29.4682231323184,24.6397181974285));
#70684=CARTESIAN_POINT('Ctrl Pts',(104.304043604523,29.3823793561953,24.573879640517));
#70685=CARTESIAN_POINT('Ctrl Pts',(104.195955578132,29.2965351197829,24.5080409992732));
#70686=CARTESIAN_POINT('Ctrl Pts',(104.087867965647,29.2106904110617,24.4422022714329));
#70687=CARTESIAN_POINT('',(104.300000000003,29.2306286312331,24.068064362549));
#70688=CARTESIAN_POINT('Origin',(104.300000000003,29.0480002025304,24.3060703646363));
#70689=CARTESIAN_POINT('',(104.624264068712,29.4881125046124,24.2656386875623));
#70690=CARTESIAN_POINT('Origin',(104.624264068712,29.3054840759098,24.5036446896497));
#70691=CARTESIAN_POINT('Ctrl Pts',(104.624264068712,29.4881125046124,24.2656386875623));
#70692=CARTESIAN_POINT('Ctrl Pts',(104.516175638879,29.4022848693738,24.1997808267293));
#70693=CARTESIAN_POINT('Ctrl Pts',(104.408087612488,29.3164569143438,24.1339227205117));
#70694=CARTESIAN_POINT('Ctrl Pts',(104.300000000003,29.2306286312331,24.068064362549));
#70695=CARTESIAN_POINT('Origin',(104.3,25.9593069400571,21.9360326667517));
#70696=CARTESIAN_POINT('Origin',(104.3,29.0480002025284,24.3060703646348));
#70697=CARTESIAN_POINT('',(104.3,28.1660070629188,23.2511515011969));
#70698=CARTESIAN_POINT('',(104.3,26.1419353687597,21.6980266646644));
#70699=CARTESIAN_POINT('Origin',(104.3,27.7453726321288,23.3065290745817));
#70700=CARTESIAN_POINT('Origin',(104.3,29.0480002025284,24.3060703646348));
#70701=CARTESIAN_POINT('Origin',(104.624264068712,29.3054840759098,24.5036446896497));
#70702=CARTESIAN_POINT('Origin',(104.624264068712,29.3054840759098,24.5036446896497));
#70703=CARTESIAN_POINT('Origin',(113.,29.3054840759098,24.5036446896497));
#70704=CARTESIAN_POINT('',(121.811388243054,29.4881125046124,24.2656386875623));
#70705=CARTESIAN_POINT('Ctrl Pts',(121.5,29.5356318566107,24.6960816898302));
#70706=CARTESIAN_POINT('Ctrl Pts',(121.5,29.5489700413278,24.6801296971867));
#70707=CARTESIAN_POINT('Ctrl Pts',(121.502178291748,29.5607352354492,24.6626361343801));
#70708=CARTESIAN_POINT('Ctrl Pts',(121.510716614322,29.5802270436011,24.625911536016));
#70709=CARTESIAN_POINT('Ctrl Pts',(121.517077828304,29.5879524700494,24.6066801452406));
#70710=CARTESIAN_POINT('Ctrl Pts',(121.541159186122,29.6047939634926,24.5487264875151));
#70711=CARTESIAN_POINT('Ctrl Pts',(121.56412779323,29.6073422778058,24.509633504542));
#70712=CARTESIAN_POINT('Ctrl Pts',(121.617288389766,29.6003545473749,24.4346560851191));
#70713=CARTESIAN_POINT('Ctrl Pts',(121.652509215907,29.5877605876801,24.3945623020958));
#70714=CARTESIAN_POINT('Ctrl Pts',(121.726559498935,29.5494817883985,24.3245682087703));
#70715=CARTESIAN_POINT('Ctrl Pts',(121.765406035132,29.5237298740531,24.2947226776164));
#70716=CARTESIAN_POINT('Ctrl Pts',(121.804557793905,29.4934979340675,24.2698451773449));
#70717=CARTESIAN_POINT('Ctrl Pts',(121.807962616873,29.49083251536,24.2677258316214));
#70718=CARTESIAN_POINT('Ctrl Pts',(121.811388687965,29.4881128573793,24.2656389582503));
#70719=CARTESIAN_POINT('',(113.,29.4881125046124,24.2656386875623));
#70720=CARTESIAN_POINT('Origin',(113.,29.1576987382828,24.0121032874578));
#70721=CARTESIAN_POINT('',(121.912131484566,29.4081413143126,24.2042746349845));
#70722=CARTESIAN_POINT('',(121.75,29.5368432263338,24.3030310854828));
#70723=CARTESIAN_POINT('Ctrl Pts',(122.,29.2397469911497,24.0750611261991));
#70724=CARTESIAN_POINT('Ctrl Pts',(122.,29.2691429403866,24.0976174313858));
#70725=CARTESIAN_POINT('Ctrl Pts',(121.991329280155,29.3037408530298,24.1241653434847));
#70726=CARTESIAN_POINT('Ctrl Pts',(121.962987211232,29.3580436225578,24.1658333240656));
#70727=CARTESIAN_POINT('Ctrl Pts',(121.938311286558,29.3873598625566,24.1883284662027));
#70728=CARTESIAN_POINT('Ctrl Pts',(121.912131759621,29.4081415324016,24.20427480233));
#70729=CARTESIAN_POINT('',(121.7,28.1660070629188,23.2511515011969));
#70730=CARTESIAN_POINT('Origin',(121.7,27.9280010608314,23.0685230724943));
#70731=CARTESIAN_POINT('',(103.5,28.1660070629188,23.2511515011969));
#70732=CARTESIAN_POINT('Ctrl Pts',(121.375735931288,24.2656386875623,29.4881125046124));
#70733=CARTESIAN_POINT('Ctrl Pts',(121.483824361121,24.1997808267293,29.4022848693738));
#70734=CARTESIAN_POINT('Ctrl Pts',(121.591912387512,24.1339227205117,29.3164569143438));
#70735=CARTESIAN_POINT('Ctrl Pts',(121.699999999997,24.068064362549,29.2306286312331));
#70736=CARTESIAN_POINT('Ctrl Pts',(121.432344074477,24.3000693004437,29.5329833529219));
#70737=CARTESIAN_POINT('Ctrl Pts',(121.540435642307,24.2342130618665,29.4471580695557));
#70738=CARTESIAN_POINT('Ctrl Pts',(121.648526737398,24.1683568810269,29.3613321441074));
#70739=CARTESIAN_POINT('Ctrl Pts',(121.756617543138,24.1025001723947,29.2755062523583));
#70740=CARTESIAN_POINT('Ctrl Pts',(121.544995916356,24.4223128317953,29.5810525234115));
#70741=CARTESIAN_POINT('Ctrl Pts',(121.653093466012,24.3564659757563,29.4952268701867));
#70742=CARTESIAN_POINT('Ctrl Pts',(121.761190817463,24.2906189537557,29.409401077777));
#70743=CARTESIAN_POINT('Ctrl Pts',(121.869287710261,24.2247717885901,29.3235748067435));
#70744=CARTESIAN_POINT('Ctrl Pts',(121.589544531169,24.577280943507,29.518244332399));
#70745=CARTESIAN_POINT('Ctrl Pts',(121.697637909658,24.5114422368762,29.4324068897941));
#70746=CARTESIAN_POINT('Ctrl Pts',(121.805730586269,24.4456032016902,29.3465688074239));
#70747=CARTESIAN_POINT('Ctrl Pts',(121.913823234176,24.3797643238856,29.2607305411385));
#70748=CARTESIAN_POINT('Ctrl Pts',(121.587867965644,24.6397181974285,29.4682231323184));
#70749=CARTESIAN_POINT('Ctrl Pts',(121.695956395477,24.573879640517,29.3823793561953));
#70750=CARTESIAN_POINT('Ctrl Pts',(121.804044421868,24.5080409992732,29.2965351197829));
#70751=CARTESIAN_POINT('Ctrl Pts',(121.912132034353,24.4422022714329,29.2106904110617));
#70752=CARTESIAN_POINT('',(121.699999999997,24.068064362549,29.2306286312331));
#70753=CARTESIAN_POINT('Origin',(121.699999999997,24.3060703646363,29.0480002025305));
#70754=CARTESIAN_POINT('',(121.375735931288,24.2656386875623,29.4881125046124));
#70755=CARTESIAN_POINT('Origin',(121.375735931288,24.5036446896497,29.3054840759098));
#70756=CARTESIAN_POINT('Ctrl Pts',(121.375735931288,24.2656386875623,29.4881125046124));
#70757=CARTESIAN_POINT('Ctrl Pts',(121.483824361121,24.1997808267293,29.4022848693738));
#70758=CARTESIAN_POINT('Ctrl Pts',(121.591912387512,24.1339227205117,29.3164569143438));
#70759=CARTESIAN_POINT('Ctrl Pts',(121.699999999997,24.068064362549,29.2306286312331));
#70760=CARTESIAN_POINT('Origin',(121.375735931288,0.,0.));
#70761=CARTESIAN_POINT('',(121.375735931288,24.6960816898302,29.5356318566107));
#70762=CARTESIAN_POINT('Origin',(121.375735931288,0.,0.));
#70763=CARTESIAN_POINT('Origin',(121.375735931288,24.5036446896497,29.3054840759098));
#70764=CARTESIAN_POINT('Origin',(121.375735931288,24.5036446896497,29.3054840759098));
#70765=CARTESIAN_POINT('Origin',(121.375735931288,24.5036446896497,29.3054840759098));
#70766=CARTESIAN_POINT('Origin',(121.7,18.8744801949098,21.9694140784679));
#70767=CARTESIAN_POINT('Origin',(121.7,24.3060703646348,29.0480002025284));
#70768=CARTESIAN_POINT('',(121.7,23.2511515011969,28.1660070629187));
#70769=CARTESIAN_POINT('',(121.7,18.6364741928224,22.1520425071705));
#70770=CARTESIAN_POINT('Origin',(121.7,23.3065290745817,27.7453726321288));
#70771=CARTESIAN_POINT('Origin',(121.7,24.3060703646347,29.0480002025285));
#70772=CARTESIAN_POINT('Origin',(113.,25.7740421742497,27.6125198053347));
#70773=CARTESIAN_POINT('',(104.3,24.8901586977665,26.7286363288515));
#70774=CARTESIAN_POINT('',(103.5,24.8901586977665,26.7286363288515));
#70775=CARTESIAN_POINT('Origin',(104.3,24.6780266634105,26.5165042944955));
#70776=CARTESIAN_POINT('',(104.087868515434,25.9972587850772,27.8357364161622));
#70777=CARTESIAN_POINT('Ctrl Pts',(104.087868240379,25.9972589794574,27.8357366105424));
#70778=CARTESIAN_POINT('Ctrl Pts',(104.061688713442,25.9787365142134,27.8172141452984));
#70779=CARTESIAN_POINT('Ctrl Pts',(104.037012788768,25.9526072839584,27.7910849150434));
#70780=CARTESIAN_POINT('Ctrl Pts',(104.008670719845,25.9042078449942,27.7426854760792));
#70781=CARTESIAN_POINT('Ctrl Pts',(104.,25.8733711201675,27.7118487512525));
#70782=CARTESIAN_POINT('Ctrl Pts',(104.,25.8471708459779,27.6856484770629));
#70783=CARTESIAN_POINT('',(104.25,26.1119693309588,27.9504469620439));
#70784=CARTESIAN_POINT('Origin',(113.,21.9649140007177,31.2535206487377));
#70785=CARTESIAN_POINT('',(121.811388243054,22.2029200028051,31.0708922200351));
#70786=CARTESIAN_POINT('Ctrl Pts',(121.5,22.1374133253307,31.4989671459791));
#70787=CARTESIAN_POINT('Ctrl Pts',(121.5,22.1544257019282,31.4870108805358));
#70788=CARTESIAN_POINT('Ctrl Pts',(121.502178291748,22.1703176740025,31.4731584527351));
#70789=CARTESIAN_POINT('Ctrl Pts',(121.510716614322,22.1986503403778,31.4427300658883));
#70790=CARTESIAN_POINT('Ctrl Pts',(121.517077828304,22.2110899794998,31.4261534563593));
#70791=CARTESIAN_POINT('Ctrl Pts',(121.541159186122,22.2423571233226,31.3745334208854));
#70792=CARTESIAN_POINT('Ctrl Pts',(121.56412779323,22.2549366144545,31.3374320512821));
#70793=CARTESIAN_POINT('Ctrl Pts',(121.617288389766,22.2675925692634,31.2632008677555));
#70794=CARTESIAN_POINT('Ctrl Pts',(121.652509215907,22.2658047729756,31.2212136906374));
#70795=CARTESIAN_POINT('Ctrl Pts',(121.726559498935,22.2469460965475,31.1436973059289));
#70796=CARTESIAN_POINT('Ctrl Pts',(121.765406035132,22.2297962492787,31.1082036507075));
#70797=CARTESIAN_POINT('Ctrl Pts',(121.804557793905,22.2070332085326,31.0763492288632));
#70798=CARTESIAN_POINT('Ctrl Pts',(121.807962616873,22.2050071388016,31.0736122369693));
#70799=CARTESIAN_POINT('Ctrl Pts',(121.811388687965,22.2029202734926,31.0708925728024));
#70800=CARTESIAN_POINT('',(113.,22.2029200028051,31.0708922200351));
#70801=CARTESIAN_POINT('Origin',(113.,21.9493846027006,30.7404784537055));
#70802=CARTESIAN_POINT('',(121.912131484566,22.1415559502273,30.9909210297353));
#70803=CARTESIAN_POINT('',(121.75,22.2403124007256,31.1196229417564));
#70804=CARTESIAN_POINT('Ctrl Pts',(122.,22.0123424414419,30.8225267065723));
#70805=CARTESIAN_POINT('Ctrl Pts',(122.,22.0348987466286,30.8519226558093));
#70806=CARTESIAN_POINT('Ctrl Pts',(121.991329280155,22.0614466587275,30.8865205684525));
#70807=CARTESIAN_POINT('Ctrl Pts',(121.962987211232,22.1031146393084,30.9408233379805));
#70808=CARTESIAN_POINT('Ctrl Pts',(121.938311286558,22.1256097814455,30.9701395779793));
#70809=CARTESIAN_POINT('Ctrl Pts',(121.912131759621,22.1415561175728,30.9909212478242));
#70810=CARTESIAN_POINT('',(121.7,21.1884328164397,29.7487867783414));
#70811=CARTESIAN_POINT('Origin',(121.7,21.0058043877371,29.510780776254));
#70812=CARTESIAN_POINT('',(103.5,21.1884328164397,29.7487867783414));
#70813=CARTESIAN_POINT('Origin',(121.7,8.161311589084,23.8841506127237));
#70814=CARTESIAN_POINT('',(121.7,13.2804347819611,35.4588694735005));
#70815=CARTESIAN_POINT('Origin',(121.7,13.0032709222077,35.57367450321));
#70816=CARTESIAN_POINT('',(121.7,12.7669018890611,34.2190913987366));
#70817=CARTESIAN_POINT('Origin',(121.7,12.3749329995982,34.0567325686927));
#70818=CARTESIAN_POINT('',(121.7,8.43847544883738,23.7693455830142));
#70819=CARTESIAN_POINT('Ctrl Pts',(121.699999999997,13.2804347819624,35.4588694735035));
#70820=CARTESIAN_POINT('Ctrl Pts',(121.591912387511,13.3218350765184,35.5588186261068));
#70821=CARTESIAN_POINT('Ctrl Pts',(121.483824361119,13.3632352128207,35.6587673966521));
#70822=CARTESIAN_POINT('Ctrl Pts',(121.375735931285,13.4046351948679,35.7587157947924));
#70823=CARTESIAN_POINT('Ctrl Pts',(121.756617543137,13.3020820369954,35.5111305701923));
#70824=CARTESIAN_POINT('Ctrl Pts',(121.648526737397,13.3434810852367,35.6110770987528));
#70825=CARTESIAN_POINT('Ctrl Pts',(121.540435642305,13.3848804265588,35.711023187081));
#70826=CARTESIAN_POINT('Ctrl Pts',(121.432344074474,13.4262791829526,35.8109690043703));
#70827=CARTESIAN_POINT('Ctrl Pts',(121.86928828501,13.2825757663851,35.6410554019366));
#70828=CARTESIAN_POINT('Ctrl Pts',(121.761191392211,13.3239799148296,35.7409938552547));
#70829=CARTESIAN_POINT('Ctrl Pts',(121.653094040341,13.3653837198587,35.8409319450387));
#70830=CARTESIAN_POINT('Ctrl Pts',(121.544996490684,13.4067874878285,35.940869821741));
#70831=CARTESIAN_POINT('Ctrl Pts',(121.913823234176,13.1506538199745,35.7438605133324));
#70832=CARTESIAN_POINT('Ctrl Pts',(121.805730586267,13.1920725002925,35.8437977872112));
#70833=CARTESIAN_POINT('Ctrl Pts',(121.697637909656,13.2334909426446,35.9437351054288));
#70834=CARTESIAN_POINT('Ctrl Pts',(121.589544531166,13.2749089952212,36.0436718192265));
#70835=CARTESIAN_POINT('Ctrl Pts',(121.912132034353,13.0760988223457,35.77291329703));
#70836=CARTESIAN_POINT('Ctrl Pts',(121.804044421867,13.1175231569589,35.8728536622539));
#70837=CARTESIAN_POINT('Ctrl Pts',(121.695956395475,13.158947125839,35.9727937163286));
#70838=CARTESIAN_POINT('Ctrl Pts',(121.587867965641,13.2003707382629,36.0727334672248));
#70839=CARTESIAN_POINT('',(121.375735931285,13.4046351948679,35.7587157947924));
#70840=CARTESIAN_POINT('',(121.587867965641,13.2003707382624,36.0727334672234));
#70841=CARTESIAN_POINT('Origin',(121.375735931285,13.1274713351145,35.873520824502));
#70842=CARTESIAN_POINT('',(121.912132034353,13.0760988223452,35.7729132970285));
#70843=CARTESIAN_POINT('Ctrl Pts',(121.587867965641,13.2003707382629,36.0727334672248));
#70844=CARTESIAN_POINT('Ctrl Pts',(121.695956395475,13.158947125839,35.9727937163286));
#70845=CARTESIAN_POINT('Ctrl Pts',(121.804044421867,13.1175231569589,35.8728536622539));
#70846=CARTESIAN_POINT('Ctrl Pts',(121.912132034353,13.0760988223457,35.77291329703));
#70847=CARTESIAN_POINT('Origin',(121.699999999997,13.003270922209,35.573674503213));
#70848=CARTESIAN_POINT('Ctrl Pts',(121.699999999997,13.2804347819624,35.4588694735035));
#70849=CARTESIAN_POINT('Ctrl Pts',(121.591912387511,13.3218350765184,35.5588186261068));
#70850=CARTESIAN_POINT('Ctrl Pts',(121.483824361119,13.3632352128207,35.6587673966521));
#70851=CARTESIAN_POINT('Ctrl Pts',(121.375735931285,13.4046351948679,35.7587157947924));
#70852=CARTESIAN_POINT('Origin',(121.7,13.0032709222077,35.57367450321));
#70853=CARTESIAN_POINT('Origin',(121.7,13.0032709222077,35.57367450321));
#70854=CARTESIAN_POINT('Origin',(113.,13.1274713351134,35.8735208244992));
#70855=CARTESIAN_POINT('',(104.188611756946,13.4046351948668,35.7587157947897));
#70856=CARTESIAN_POINT('',(104.5,13.2305666597347,36.155250045634));
#70857=CARTESIAN_POINT('Ctrl Pts',(104.188611312035,13.4046353650279,35.7587162055958));
#70858=CARTESIAN_POINT('Ctrl Pts',(104.19203735624,13.4059472109483,35.7618832950857));
#70859=CARTESIAN_POINT('Ctrl Pts',(104.19544217649,13.4071958583021,35.7650514088087));
#70860=CARTESIAN_POINT('Ctrl Pts',(104.234593964868,13.4209387465913,35.8017119537402));
#70861=CARTESIAN_POINT('Ctrl Pts',(104.273440501065,13.4283177930335,35.8404348990817));
#70862=CARTESIAN_POINT('Ctrl Pts',(104.347490784093,13.426471158975,35.9201909616572));
#70863=CARTESIAN_POINT('Ctrl Pts',(104.382711610234,13.4173309564933,35.9612101761365));
#70864=CARTESIAN_POINT('Ctrl Pts',(104.43587220677,13.3858937988499,36.0296363912825));
#70865=CARTESIAN_POINT('Ctrl Pts',(104.458840813878,13.3641404024312,36.0622177504903));
#70866=CARTESIAN_POINT('Ctrl Pts',(104.482922171696,13.320578412409,36.1039863436012));
#70867=CARTESIAN_POINT('Ctrl Pts',(104.489283385678,13.3042723014621,36.1167785033386));
#70868=CARTESIAN_POINT('Ctrl Pts',(104.497821708253,13.2690296012548,36.1388370343898));
#70869=CARTESIAN_POINT('Ctrl Pts',(104.5,13.2500938628618,36.1481043071223));
#70870=CARTESIAN_POINT('Ctrl Pts',(104.5,13.2305666597347,36.155250045634));
#70871=CARTESIAN_POINT('',(121.375735931288,13.2305666597347,36.155250045634));
#70872=CARTESIAN_POINT('',(113.,13.2305666597347,36.155250045634));
#70873=CARTESIAN_POINT('Origin',(121.375735931288,13.1274713351134,35.8735208244992));
#70874=CARTESIAN_POINT('',(113.,13.4046351948668,35.7587157947897));
#70875=CARTESIAN_POINT('Origin',(121.375735931288,13.1274713351135,35.8735208244991));
#70876=CARTESIAN_POINT('Origin',(121.375735931288,13.1274713351135,35.8735208244991));
#70877=CARTESIAN_POINT('Origin',(121.7,0.,0.));
#70878=CARTESIAN_POINT('',(121.912132034352,11.4032031398184,36.3407848610969));
#70879=CARTESIAN_POINT('Origin',(121.912132034356,2.22044604925031E-15,
0.));
#70880=CARTESIAN_POINT('Origin',(121.7,11.3396925048197,36.1383832819456));
#70881=CARTESIAN_POINT('Origin',(121.75,0.,0.));
#70882=CARTESIAN_POINT('',(121.587867965644,11.4871305554742,36.6543001437251));
#70883=CARTESIAN_POINT('Origin',(121.587867965644,-1.11022302462516E-15,
0.));
#70884=CARTESIAN_POINT('Ctrl Pts',(121.912132034352,11.4032031398191,36.3407848610988));
#70885=CARTESIAN_POINT('Ctrl Pts',(121.804044421867,11.4311788451333,36.4452904208128));
#70886=CARTESIAN_POINT('Ctrl Pts',(121.695956395477,11.4591546511876,36.5497955110311));
#70887=CARTESIAN_POINT('Ctrl Pts',(121.587867965644,11.4871305554741,36.6543001437251));
#70888=CARTESIAN_POINT('Origin',(104.3,-2.06696949019973,13.8959604433702));
#70889=CARTESIAN_POINT('',(104.3,-8.53850760858151,36.8889585127428));
#70890=CARTESIAN_POINT('Origin',(104.3,-8.24872986069479,36.9666042262736));
#70891=CARTESIAN_POINT('',(104.3,-8.19119157206621,35.5927574181843));
#70892=CARTESIAN_POINT('Origin',(104.3,-7.82376811064874,35.3806253838283));
#70893=CARTESIAN_POINT('',(104.3,-2.35674723808646,13.8183147298394));
#70894=CARTESIAN_POINT('Ctrl Pts',(104.300000000004,-8.53850760858254,36.8889585127467));
#70895=CARTESIAN_POINT('Ctrl Pts',(104.40808761249,-8.56650773557452,36.9934564092991));
#70896=CARTESIAN_POINT('Ctrl Pts',(104.516175638882,-8.59450775553533,37.0979539064058));
#70897=CARTESIAN_POINT('Ctrl Pts',(104.624264068716,-8.62250767116923,37.2024510141591));
#70898=CARTESIAN_POINT('Ctrl Pts',(104.243382456863,-8.55314822639583,36.9435980422801));
#70899=CARTESIAN_POINT('Ctrl Pts',(104.351473262604,-8.58114746024187,37.0480931745619));
#70900=CARTESIAN_POINT('Ctrl Pts',(104.459564357696,-8.60914704212313,37.1525879086325));
#70901=CARTESIAN_POINT('Ctrl Pts',(104.567655925526,-8.63714607945794,37.2570822976346));
#70902=CARTESIAN_POINT('Ctrl Pts',(104.130708900332,-8.51685469895555,37.0698669867126));
#70903=CARTESIAN_POINT('Ctrl Pts',(104.238805793131,-8.5448600434025,37.174354778547));
#70904=CARTESIAN_POINT('Ctrl Pts',(104.346903147053,-8.57286509255767,37.278842163661));
#70905=CARTESIAN_POINT('Ctrl Pts',(104.45500069671,-8.6008701350484,37.3833293341507));
#70906=CARTESIAN_POINT('Ctrl Pts',(104.086176765825,-8.37263814546985,37.1545715999316));
#70907=CARTESIAN_POINT('Ctrl Pts',(104.194269413734,-8.40065805141576,37.2590601192072));
#70908=CARTESIAN_POINT('Ctrl Pts',(104.302362090345,-8.42867771564423,37.3635486513814));
#70909=CARTESIAN_POINT('Ctrl Pts',(104.410455468834,-8.45669707232439,37.4680365334307));
#70910=CARTESIAN_POINT('Ctrl Pts',(104.087867965648,-8.29492882695159,37.1736444530859));
#70911=CARTESIAN_POINT('Ctrl Pts',(104.195955578134,-8.32295393531795,37.2781367752932));
#70912=CARTESIAN_POINT('Ctrl Pts',(104.304043604526,-8.3509787216931,37.3826287412755));
#70913=CARTESIAN_POINT('Ctrl Pts',(104.41213203436,-8.37900319423446,37.4871203601462));
#70914=CARTESIAN_POINT('',(104.624264068716,-8.62250767116923,37.2024510141591));
#70915=CARTESIAN_POINT('',(104.41213203436,-8.37900319423406,37.4871203601444));
#70916=CARTESIAN_POINT('Origin',(104.624264068716,-8.33272992328251,37.2800967276899));
#70917=CARTESIAN_POINT('',(104.087867965648,-8.29492882695116,37.1736444530839));
#70918=CARTESIAN_POINT('Ctrl Pts',(104.41213203436,-8.37900319423446,37.4871203601462));
#70919=CARTESIAN_POINT('Ctrl Pts',(104.304043604526,-8.3509787216931,37.3826287412755));
#70920=CARTESIAN_POINT('Ctrl Pts',(104.195955578134,-8.32295393531795,37.2781367752932));
#70921=CARTESIAN_POINT('Ctrl Pts',(104.087867965648,-8.29492882695159,37.1736444530859));
#70922=CARTESIAN_POINT('Origin',(104.300000000004,-8.24872986069582,36.9666042262774));
#70923=CARTESIAN_POINT('Ctrl Pts',(104.300000000004,-8.53850760858254,36.8889585127467));
#70924=CARTESIAN_POINT('Ctrl Pts',(104.40808761249,-8.56650773557452,36.9934564092991));
#70925=CARTESIAN_POINT('Ctrl Pts',(104.516175638882,-8.59450775553533,37.0979539064058));
#70926=CARTESIAN_POINT('Ctrl Pts',(104.624264068716,-8.62250767116923,37.2024510141591));
#70927=CARTESIAN_POINT('Origin',(104.3,-8.2487298606948,36.9666042262736));
#70928=CARTESIAN_POINT('Origin',(104.3,-8.2487298606948,36.9666042262736));
#70929=CARTESIAN_POINT('Origin',(113.,-8.33272992328155,37.2800967276863));
#70930=CARTESIAN_POINT('',(121.811388243054,-8.62250767116827,37.2024510141556));
#70931=CARTESIAN_POINT('',(121.5,-8.39817021063716,37.5728723564378));
#70932=CARTESIAN_POINT('Ctrl Pts',(121.811388687965,-8.62250778625267,37.2024514436577));
#70933=CARTESIAN_POINT('Ctrl Pts',(121.80796264376,-8.62339502101782,37.2057626685107));
#70934=CARTESIAN_POINT('Ctrl Pts',(121.80455782351,-8.62421946419966,37.2090666597662));
#70935=CARTESIAN_POINT('Ctrl Pts',(121.765406035132,-8.6330596188398,37.2472073755322));
#70936=CARTESIAN_POINT('Ctrl Pts',(121.726559498935,-8.63532117790981,37.2865621995426));
#70937=CARTESIAN_POINT('Ctrl Pts',(121.652509215907,-8.62308008690722,37.3653949038344));
#70938=CARTESIAN_POINT('Ctrl Pts',(121.617288389766,-8.60866399825098,37.4048701574215));
#70939=CARTESIAN_POINT('Ctrl Pts',(121.56412779323,-8.56856437653814,37.4686076043297));
#70940=CARTESIAN_POINT('Ctrl Pts',(121.541159186122,-8.54274436268671,37.4980708374905));
#70941=CARTESIAN_POINT('Ctrl Pts',(121.517077828304,-8.4941031561148,37.533796113814));
#70942=CARTESIAN_POINT('Ctrl Pts',(121.510716614322,-8.47626683430664,37.5443504602798));
#70943=CARTESIAN_POINT('Ctrl Pts',(121.502178291748,-8.43844642422114,37.5616201820783));
#70944=CARTESIAN_POINT('Ctrl Pts',(121.5,-8.41846306187311,37.5683365621785));
#70945=CARTESIAN_POINT('Ctrl Pts',(121.5,-8.39817021063716,37.5728723564378));
#70946=CARTESIAN_POINT('',(104.624264068712,-8.39817021063716,37.5728723564378));
#70947=CARTESIAN_POINT('',(113.,-8.39817021063716,37.5728723564378));
#70948=CARTESIAN_POINT('Origin',(104.624264068712,-8.33272992328155,37.2800967276863));
#70949=CARTESIAN_POINT('',(113.,-8.62250767116827,37.2024510141556));
#70950=CARTESIAN_POINT('Origin',(104.624264068712,-8.3327299232817,37.2800967276863));
#70951=CARTESIAN_POINT('Origin',(104.624264068712,-8.3327299232817,37.2800967276863));
#70952=CARTESIAN_POINT('Origin',(104.3,0.,0.));
#70953=CARTESIAN_POINT('',(104.087867965649,-6.56222288596765,37.5183010937784));
#70954=CARTESIAN_POINT('Origin',(104.087867965644,-1.66533453693773E-15,
0.));
#70955=CARTESIAN_POINT('Origin',(104.3,-6.52567430068159,37.3093412868425));
#70956=CARTESIAN_POINT('Origin',(104.25,0.,0.));
#70957=CARTESIAN_POINT('',(104.412132034356,-6.60451033490358,37.8400889356902));
#70958=CARTESIAN_POINT('Origin',(104.412132034356,-1.66533453693773E-15,
0.));
#70959=CARTESIAN_POINT('Ctrl Pts',(104.087867965649,-6.56222288596809,37.5183010937809));
#70960=CARTESIAN_POINT('Ctrl Pts',(104.195955578133,-6.5763185424699,37.6255641562333));
#70961=CARTESIAN_POINT('Ctrl Pts',(104.304043604524,-6.59041436013136,37.7328267663559));
#70962=CARTESIAN_POINT('Ctrl Pts',(104.412132034356,-6.60451033490358,37.8400889356902));
#70963=CARTESIAN_POINT('Origin',(104.624264068712,0.,0.));
#70964=CARTESIAN_POINT('',(104.624264068712,-6.61961818902332,37.9266483495649));
#70965=CARTESIAN_POINT('Origin',(104.624264068712,0.,0.));
#70966=CARTESIAN_POINT('Origin',(104.624264068712,-6.56803674858937,37.6311160247631));
#70967=CARTESIAN_POINT('Origin',(113.,0.,0.));
#70968=CARTESIAN_POINT('',(121.5,-6.61961818902332,37.9266483495649));
#70969=CARTESIAN_POINT('Origin',(121.5,0.,0.));
#70970=CARTESIAN_POINT('',(113.,-6.61961818902332,37.9266483495649));
#70971=CARTESIAN_POINT('Origin',(104.3,-2.96245695514521,11.3330052466625));
#70972=CARTESIAN_POINT('',(104.3,-13.2804347819611,35.4588694735005));
#70973=CARTESIAN_POINT('Origin',(104.3,-13.0032709222077,35.57367450321));
#70974=CARTESIAN_POINT('',(104.3,-12.7669018890611,34.2190913987366));
#70975=CARTESIAN_POINT('Origin',(104.3,-12.3749329995982,34.0567325686927));
#70976=CARTESIAN_POINT('',(104.3,-3.23962081489859,11.218200216953));
#70977=CARTESIAN_POINT('Ctrl Pts',(104.300000000003,-13.2804347819623,35.4588694735034));
#70978=CARTESIAN_POINT('Ctrl Pts',(104.408087612489,-13.3218350765183,35.5588186261068));
#70979=CARTESIAN_POINT('Ctrl Pts',(104.516175638881,-13.3632352128207,35.6587673966521));
#70980=CARTESIAN_POINT('Ctrl Pts',(104.624264068715,-13.4046351948679,35.7587157947924));
#70981=CARTESIAN_POINT('Ctrl Pts',(104.243382456863,-13.3020820369953,35.5111305701923));
#70982=CARTESIAN_POINT('Ctrl Pts',(104.351473262603,-13.3434810852367,35.6110770987527));
#70983=CARTESIAN_POINT('Ctrl Pts',(104.459564357695,-13.3848804265588,35.7110231870809));
#70984=CARTESIAN_POINT('Ctrl Pts',(104.567655925526,-13.4262791829526,35.8109690043703));
#70985=CARTESIAN_POINT('Ctrl Pts',(104.130709407257,-13.2825795738598,35.6410563204708));
#70986=CARTESIAN_POINT('Ctrl Pts',(104.238806300056,-13.3239837223043,35.7409947737889));
#70987=CARTESIAN_POINT('Ctrl Pts',(104.346903653609,-13.3653875253347,35.8409328626189));
#70988=CARTESIAN_POINT('Ctrl Pts',(104.455001203266,-13.4067912933046,35.9408707393212));
#70989=CARTESIAN_POINT('Ctrl Pts',(104.086176765824,-13.1506538199745,35.7438605133323));
#70990=CARTESIAN_POINT('Ctrl Pts',(104.194269413733,-13.1920725002925,35.8437977872111));
#70991=CARTESIAN_POINT('Ctrl Pts',(104.302362090344,-13.2334909426446,35.9437351054287));
#70992=CARTESIAN_POINT('Ctrl Pts',(104.410455468834,-13.2749089952212,36.0436718192265));
#70993=CARTESIAN_POINT('Ctrl Pts',(104.087867965647,-13.0760988223457,35.77291329703));
#70994=CARTESIAN_POINT('Ctrl Pts',(104.195955578133,-13.1175231569589,35.8728536622539));
#70995=CARTESIAN_POINT('Ctrl Pts',(104.304043604525,-13.1589471258389,35.9727937163286));
#70996=CARTESIAN_POINT('Ctrl Pts',(104.412132034359,-13.2003707382629,36.0727334672248));
#70997=CARTESIAN_POINT('',(104.624264068715,-13.4046351948679,35.7587157947924));
#70998=CARTESIAN_POINT('',(104.412132034359,-13.2003707382624,36.0727334672234));
#70999=CARTESIAN_POINT('Origin',(104.624264068715,-13.1274713351145,35.873520824502));
#71000=CARTESIAN_POINT('',(104.087867965647,-13.0760988223451,35.7729132970285));
#71001=CARTESIAN_POINT('Ctrl Pts',(104.412132034359,-13.2003707382629,36.0727334672248));
#71002=CARTESIAN_POINT('Ctrl Pts',(104.304043604525,-13.1589471258389,35.9727937163286));
#71003=CARTESIAN_POINT('Ctrl Pts',(104.195955578133,-13.1175231569589,35.8728536622539));
#71004=CARTESIAN_POINT('Ctrl Pts',(104.087867965647,-13.0760988223457,35.77291329703));
#71005=CARTESIAN_POINT('Origin',(104.300000000003,-13.0032709222089,35.5736745032129));
#71006=CARTESIAN_POINT('Ctrl Pts',(104.300000000003,-13.2804347819623,35.4588694735034));
#71007=CARTESIAN_POINT('Ctrl Pts',(104.408087612489,-13.3218350765183,35.5588186261068));
#71008=CARTESIAN_POINT('Ctrl Pts',(104.516175638881,-13.3632352128207,35.6587673966521));
#71009=CARTESIAN_POINT('Ctrl Pts',(104.624264068715,-13.4046351948679,35.7587157947924));
#71010=CARTESIAN_POINT('Origin',(104.3,-13.0032709222077,35.57367450321));
#71011=CARTESIAN_POINT('Origin',(104.3,-13.0032709222077,35.57367450321));
#71012=CARTESIAN_POINT('Origin',(113.,-13.1274713351134,35.8735208244992));
#71013=CARTESIAN_POINT('',(121.811388243054,-13.4046351948668,35.7587157947897));
#71014=CARTESIAN_POINT('',(121.5,-13.2305666597347,36.155250045634));
#71015=CARTESIAN_POINT('Ctrl Pts',(121.811388687965,-13.4046353650279,35.7587162055958));
#71016=CARTESIAN_POINT('Ctrl Pts',(121.80796264376,-13.4059472109483,35.7618832950857));
#71017=CARTESIAN_POINT('Ctrl Pts',(121.80455782351,-13.4071958583021,35.7650514088087));
#71018=CARTESIAN_POINT('Ctrl Pts',(121.765406035132,-13.4209387465913,35.8017119537402));
#71019=CARTESIAN_POINT('Ctrl Pts',(121.726559498935,-13.4283177930335,35.8404348990817));
#71020=CARTESIAN_POINT('Ctrl Pts',(121.652509215907,-13.426471158975,35.9201909616573));
#71021=CARTESIAN_POINT('Ctrl Pts',(121.617288389766,-13.4173309564933,35.9612101761366));
#71022=CARTESIAN_POINT('Ctrl Pts',(121.56412779323,-13.3858937988498,36.0296363912825));
#71023=CARTESIAN_POINT('Ctrl Pts',(121.541159186122,-13.3641404024312,36.0622177504903));
#71024=CARTESIAN_POINT('Ctrl Pts',(121.517077828304,-13.320578412409,36.1039863436012));
#71025=CARTESIAN_POINT('Ctrl Pts',(121.510716614322,-13.304272301462,36.1167785033386));
#71026=CARTESIAN_POINT('Ctrl Pts',(121.502178291748,-13.2690296012548,36.1388370343898));
#71027=CARTESIAN_POINT('Ctrl Pts',(121.5,-13.2500938628618,36.1481043071223));
#71028=CARTESIAN_POINT('Ctrl Pts',(121.5,-13.2305666597347,36.155250045634));
#71029=CARTESIAN_POINT('',(104.624264068712,-13.2305666597347,36.155250045634));
#71030=CARTESIAN_POINT('',(113.,-13.2305666597347,36.155250045634));
#71031=CARTESIAN_POINT('Origin',(104.624264068712,-13.1274713351134,35.8735208244992));
#71032=CARTESIAN_POINT('',(113.,-13.4046351948668,35.7587157947897));
#71033=CARTESIAN_POINT('Origin',(104.624264068712,-13.1274713351135,35.8735208244991));
#71034=CARTESIAN_POINT('Origin',(104.624264068712,-13.1274713351135,35.8735208244991));
#71035=CARTESIAN_POINT('Origin',(104.3,0.,0.));
#71036=CARTESIAN_POINT('',(104.087867965648,-11.4032031398184,36.3407848610969));
#71037=CARTESIAN_POINT('Origin',(104.087867965644,-1.11022302462516E-15,
0.));
#71038=CARTESIAN_POINT('Origin',(104.3,-11.3396925048198,36.1383832819455));
#71039=CARTESIAN_POINT('Origin',(104.25,0.,0.));
#71040=CARTESIAN_POINT('',(104.412132034356,-11.4871305554741,36.6543001437251));
#71041=CARTESIAN_POINT('Origin',(104.412132034356,-1.11022302462516E-15,
-2.22044604925031E-15));
#71042=CARTESIAN_POINT('Ctrl Pts',(104.087867965648,-11.403203139819,36.3407848610988));
#71043=CARTESIAN_POINT('Ctrl Pts',(104.195955578133,-11.4311788451333,36.4452904208127));
#71044=CARTESIAN_POINT('Ctrl Pts',(104.304043604523,-11.4591546511876,36.5497955110311));
#71045=CARTESIAN_POINT('Ctrl Pts',(104.412132034356,-11.4871305554741,36.6543001437251));
#71046=CARTESIAN_POINT('Origin',(104.624264068712,0.,0.));
#71047=CARTESIAN_POINT('',(104.624264068712,-11.5134074305014,36.7381470591438));
#71048=CARTESIAN_POINT('Origin',(104.624264068712,0.,0.));
#71049=CARTESIAN_POINT('Origin',(104.624264068712,-11.4236925674066,36.4518757833583));
#71050=CARTESIAN_POINT('Origin',(113.,0.,0.));
#71051=CARTESIAN_POINT('',(121.5,-11.5134074305014,36.7381470591438));
#71052=CARTESIAN_POINT('Origin',(121.5,0.,0.));
#71053=CARTESIAN_POINT('',(113.,-11.5134074305014,36.7381470591438));
#71054=CARTESIAN_POINT('Ctrl Pts',(104.624264068712,8.62250767116828,37.2024510141555));
#71055=CARTESIAN_POINT('Ctrl Pts',(104.516175638879,8.59450775553471,37.0979539064034));
#71056=CARTESIAN_POINT('Ctrl Pts',(104.408087612489,8.56650773557423,36.993456409298));
#71057=CARTESIAN_POINT('Ctrl Pts',(104.300000000004,8.53850760858259,36.8889585127468));
#71058=CARTESIAN_POINT('Ctrl Pts',(104.567655925523,8.63714607945699,37.257082297631));
#71059=CARTESIAN_POINT('Ctrl Pts',(104.459564357693,8.60914704212251,37.1525879086302));
#71060=CARTESIAN_POINT('Ctrl Pts',(104.351473262603,8.58114746024157,37.0480931745608));
#71061=CARTESIAN_POINT('Ctrl Pts',(104.243382456864,8.55314822639588,36.9435980422802));
#71062=CARTESIAN_POINT('Ctrl Pts',(104.455000696706,8.60087013504745,37.3833293341471));
#71063=CARTESIAN_POINT('Ctrl Pts',(104.346903147051,8.57286509255706,37.2788421636586));
#71064=CARTESIAN_POINT('Ctrl Pts',(104.238805793129,8.5448600434022,37.1743547785458));
#71065=CARTESIAN_POINT('Ctrl Pts',(104.130708900332,8.5168546989556,37.0698669867127));
#71066=CARTESIAN_POINT('Ctrl Pts',(104.410455468831,8.45669707232344,37.4680365334272));
#71067=CARTESIAN_POINT('Ctrl Pts',(104.302362090343,8.42867771564362,37.363548651379));
#71068=CARTESIAN_POINT('Ctrl Pts',(104.194269413732,8.40065805141547,37.2590601192061));
#71069=CARTESIAN_POINT('Ctrl Pts',(104.086176765825,8.3726381454699,37.1545715999318));
#71070=CARTESIAN_POINT('Ctrl Pts',(104.412132034356,8.37900319423351,37.4871203601426));
#71071=CARTESIAN_POINT('Ctrl Pts',(104.304043604523,8.35097872169249,37.3826287412732));
#71072=CARTESIAN_POINT('Ctrl Pts',(104.195955578133,8.32295393531766,37.2781367752921));
#71073=CARTESIAN_POINT('Ctrl Pts',(104.087867965648,8.29492882695164,37.173644453086));
#71074=CARTESIAN_POINT('',(104.300000000004,8.53850760858259,36.8889585127468));
#71075=CARTESIAN_POINT('Origin',(104.300000000004,8.24872986069587,36.9666042262775));
#71076=CARTESIAN_POINT('',(104.624264068712,8.62250767116828,37.2024510141556));
#71077=CARTESIAN_POINT('Origin',(104.624264068712,8.33272992328156,37.2800967276863));
#71078=CARTESIAN_POINT('Ctrl Pts',(104.624264068712,8.62250767116828,37.2024510141555));
#71079=CARTESIAN_POINT('Ctrl Pts',(104.516175638879,8.59450775553471,37.0979539064034));
#71080=CARTESIAN_POINT('Ctrl Pts',(104.408087612489,8.56650773557423,36.993456409298));
#71081=CARTESIAN_POINT('Ctrl Pts',(104.300000000004,8.53850760858259,36.8889585127468));
#71082=CARTESIAN_POINT('Origin',(104.3,4.61248681829541,23.3959604433702));
#71083=CARTESIAN_POINT('Origin',(104.3,8.24872986069481,36.9666042262736));
#71084=CARTESIAN_POINT('',(104.3,8.19119157206623,35.5927574181843));
#71085=CARTESIAN_POINT('',(104.3,4.90226456618213,23.3183147298394));
#71086=CARTESIAN_POINT('Origin',(104.3,7.82376811064875,35.3806253838283));
#71087=CARTESIAN_POINT('Origin',(104.3,8.24872986069481,36.9666042262736));
#71088=CARTESIAN_POINT('Origin',(104.624264068712,8.33272992328157,37.2800967276863));
#71089=CARTESIAN_POINT('Origin',(104.624264068712,8.33272992328157,37.2800967276863));
#71090=CARTESIAN_POINT('Origin',(113.,6.21624207609291,37.2573594669753));
#71091=CARTESIAN_POINT('',(121.7,6.05308433581784,36.018053390258));
#71092=CARTESIAN_POINT('',(103.5,6.05308433581784,36.018053390258));
#71093=CARTESIAN_POINT('Origin',(121.7,6.01392647815183,35.7206199318459));
#71094=CARTESIAN_POINT('',(121.912131484566,6.25744605691557,37.5703347737697));
#71095=CARTESIAN_POINT('Ctrl Pts',(121.912131759621,6.25744609279658,37.570335046313));
#71096=CARTESIAN_POINT('Ctrl Pts',(121.938311286558,6.25402699553552,37.5443644242305));
#71097=CARTESIAN_POINT('Ctrl Pts',(121.962987211232,6.24920375098242,37.5077282445796));
#71098=CARTESIAN_POINT('Ctrl Pts',(121.991329280155,6.24026960603901,37.439866676382));
#71099=CARTESIAN_POINT('Ctrl Pts',(122.,6.23457739606556,37.3966300490657));
#71100=CARTESIAN_POINT('Ctrl Pts',(122.,6.22974103737678,37.3598942576648));
#71101=CARTESIAN_POINT('',(121.75,6.27862069582412,37.7311721243447));
#71102=CARTESIAN_POINT('Origin',(104.3,11.4838426166369,23.5434471056386));
#71103=CARTESIAN_POINT('',(104.3,15.6825215664905,34.4638925493512));
#71104=CARTESIAN_POINT('Origin',(104.3,15.9596854262438,34.3490875196417));
#71105=CARTESIAN_POINT('',(104.3,15.1689886735905,33.2241144745873));
#71106=CARTESIAN_POINT('Origin',(104.3,15.3313475036343,32.8321455851244));
#71107=CARTESIAN_POINT('',(104.3,11.2066787568835,23.6582521353481));
#71108=CARTESIAN_POINT('Ctrl Pts',(104.300000000003,15.6825215664917,34.4638925493543));
#71109=CARTESIAN_POINT('Ctrl Pts',(104.408087612489,15.7239218610477,34.5638417019577));
#71110=CARTESIAN_POINT('Ctrl Pts',(104.516175638881,15.7653219973501,34.6637904725029));
#71111=CARTESIAN_POINT('Ctrl Pts',(104.624264068715,15.8067219793973,34.7637388706433));
#71112=CARTESIAN_POINT('Ctrl Pts',(104.243382456863,15.7041688215248,34.5161536460432));
#71113=CARTESIAN_POINT('Ctrl Pts',(104.351473262603,15.7455681418798,34.6161000618904));
#71114=CARTESIAN_POINT('Ctrl Pts',(104.459564357695,15.7869669437042,34.7160463736859));
#71115=CARTESIAN_POINT('Ctrl Pts',(104.567655925526,15.828365967482,34.8159920802212));
#71116=CARTESIAN_POINT('Ctrl Pts',(104.130709646627,15.8098307364183,34.5942343545562));
#71117=CARTESIAN_POINT('Ctrl Pts',(104.238806539425,15.8512207403264,34.6941786667331));
#71118=CARTESIAN_POINT('Ctrl Pts',(104.346903892804,15.8926107306706,34.7941224771499));
#71119=CARTESIAN_POINT('Ctrl Pts',(104.455001442461,15.934000595886,34.8940661125617));
#71120=CARTESIAN_POINT('Ctrl Pts',(104.086176765824,15.9758096616227,34.5736426479042));
#71121=CARTESIAN_POINT('Ctrl Pts',(104.194269413733,16.017188555955,34.6735964016779));
#71122=CARTESIAN_POINT('Ctrl Pts',(104.302362090344,16.0585676499069,34.7735500185365));
#71123=CARTESIAN_POINT('Ctrl Pts',(104.410455468834,16.0999465920824,34.8735029323928));
#71124=CARTESIAN_POINT('Ctrl Pts',(104.087867965647,16.0490714263823,34.5414677238745));
#71125=CARTESIAN_POINT('Ctrl Pts',(104.195955578133,16.0904485084352,34.6414276617498));
#71126=CARTESIAN_POINT('Ctrl Pts',(104.304043604525,16.1318256290849,34.7413871209968));
#71127=CARTESIAN_POINT('Ctrl Pts',(104.412132034359,16.1732027874074,34.8413461138118));
#71128=CARTESIAN_POINT('',(104.624264068715,15.8067219793973,34.7637388706433));
#71129=CARTESIAN_POINT('',(104.412132034359,16.1732027874068,34.8413461138104));
#71130=CARTESIAN_POINT('Origin',(104.624264068715,16.0838858391507,34.6489338409338));
#71131=CARTESIAN_POINT('',(104.087867965647,16.0490714263816,34.541467723873));
#71132=CARTESIAN_POINT('Ctrl Pts',(104.412132034359,16.1732027874074,34.8413461138118));
#71133=CARTESIAN_POINT('Ctrl Pts',(104.304043604525,16.1318256290849,34.7413871209968));
#71134=CARTESIAN_POINT('Ctrl Pts',(104.195955578133,16.0904485084352,34.6414276617498));
#71135=CARTESIAN_POINT('Ctrl Pts',(104.087867965647,16.0490714263823,34.5414677238745));
#71136=CARTESIAN_POINT('Origin',(104.300000000003,15.9596854262451,34.3490875196448));
#71137=CARTESIAN_POINT('Ctrl Pts',(104.300000000003,15.6825215664917,34.4638925493543));
#71138=CARTESIAN_POINT('Ctrl Pts',(104.408087612489,15.7239218610477,34.5638417019577));
#71139=CARTESIAN_POINT('Ctrl Pts',(104.516175638881,15.7653219973501,34.6637904725029));
#71140=CARTESIAN_POINT('Ctrl Pts',(104.624264068715,15.8067219793973,34.7637388706433));
#71141=CARTESIAN_POINT('Origin',(104.3,15.9596854262438,34.3490875196417));
#71142=CARTESIAN_POINT('Origin',(104.3,15.9596854262438,34.3490875196417));
#71143=CARTESIAN_POINT('Origin',(113.,16.0838858391495,34.6489338409309));
#71144=CARTESIAN_POINT('',(121.811388243054,15.8067219793961,34.7637388706404));
#71145=CARTESIAN_POINT('',(121.5,16.210199078724,34.9210458868021));
#71146=CARTESIAN_POINT('Ctrl Pts',(121.811388687965,15.8067221495578,34.7637392814463));
#71147=CARTESIAN_POINT('Ctrl Pts',(121.80796264376,15.8080340048666,34.7669063670474));
#71148=CARTESIAN_POINT('Ctrl Pts',(121.80455782351,15.8093912725525,34.7700294887557));
#71149=CARTESIAN_POINT('Ctrl Pts',(121.765406035132,15.8255965029732,34.8056700981812));
#71150=CARTESIAN_POINT('Ctrl Pts',(121.726559498935,15.8477599864337,34.8382691291976));
#71151=CARTESIAN_POINT('Ctrl Pts',(121.652509215907,15.9054618065867,34.8933594144204));
#71152=CARTESIAN_POINT('Ctrl Pts',(121.617288389766,15.9409298704602,34.9159012799814));
#71153=CARTESIAN_POINT('Ctrl Pts',(121.56412779323,16.0115439385518,34.9420564933711));
#71154=CARTESIAN_POINT('Ctrl Pts',(121.541159186122,16.0499644127093,34.9497130192858));
#71155=CARTESIAN_POINT('Ctrl Pts',(121.517077828304,16.1103022466854,34.9484448961684));
#71156=CARTESIAN_POINT('Ctrl Pts',(121.510716614322,16.1308778312071,34.9459601574395));
#71157=CARTESIAN_POINT('Ctrl Pts',(121.502178291748,16.1713959204003,34.9366375420249));
#71158=CARTESIAN_POINT('Ctrl Pts',(121.5,16.1913384608169,34.9298009043927));
#71159=CARTESIAN_POINT('Ctrl Pts',(121.5,16.210199078724,34.9210458868021));
#71160=CARTESIAN_POINT('',(104.624264068712,16.210199078724,34.9210458868021));
#71161=CARTESIAN_POINT('',(113.,16.210199078724,34.9210458868021));
#71162=CARTESIAN_POINT('Origin',(104.624264068712,16.0838858391495,34.6489338409309));
#71163=CARTESIAN_POINT('',(113.,15.8067219793961,34.7637388706404));
#71164=CARTESIAN_POINT('Origin',(104.624264068712,16.0838858391494,34.648933840931));
#71165=CARTESIAN_POINT('Origin',(104.624264068712,16.0838858391494,34.648933840931));
#71166=CARTESIAN_POINT('Origin',(104.3,0.,0.));
#71167=CARTESIAN_POINT('',(104.087867965647,17.6335331415094,33.7600976763358));
#71168=CARTESIAN_POINT('Origin',(104.087867965644,-4.44089209850063E-15,
2.22044604925031E-15));
#71169=CARTESIAN_POINT('Origin',(104.3,17.5353224130539,33.5720693465106));
#71170=CARTESIAN_POINT('Origin',(104.25,0.,0.));
#71171=CARTESIAN_POINT('',(104.412132034356,17.7958762791241,34.041132103426));
#71172=CARTESIAN_POINT('Origin',(104.412132034356,2.22044604925031E-15,
0.));
#71173=CARTESIAN_POINT('Ctrl Pts',(104.087867965647,17.63353314151,33.7600976763372));
#71174=CARTESIAN_POINT('Ctrl Pts',(104.195955578132,17.6876479205194,33.8537760772191));
#71175=CARTESIAN_POINT('Ctrl Pts',(104.304043604523,17.7417622963114,33.9474542173515));
#71176=CARTESIAN_POINT('Ctrl Pts',(104.412132034356,17.7958762791241,34.041132103426));
#71177=CARTESIAN_POINT('Origin',(104.624264068712,0.,0.));
#71178=CARTESIAN_POINT('',(104.624264068712,17.8365844450781,34.1190013824203));
#71179=CARTESIAN_POINT('Origin',(104.624264068712,0.,0.));
#71180=CARTESIAN_POINT('Origin',(104.624264068712,17.6975980727788,33.8531390339859));
#71181=CARTESIAN_POINT('Origin',(113.,0.,0.));
#71182=CARTESIAN_POINT('',(121.5,17.8365844450781,34.1190013824203));
#71183=CARTESIAN_POINT('Origin',(121.5,0.,0.));
#71184=CARTESIAN_POINT('',(113.,17.8365844450781,34.1190013824203));
#71185=CARTESIAN_POINT('Ctrl Pts',(104.624264068712,17.9574056939141,33.7031390339859));
#71186=CARTESIAN_POINT('Ctrl Pts',(104.516175638879,17.9033140106251,33.6094494902625));
#71187=CARTESIAN_POINT('Ctrl Pts',(104.408087612488,17.8492221257921,33.5157595974544));
#71188=CARTESIAN_POINT('Ctrl Pts',(104.300000000003,17.7951300341907,33.4220693465132));
#71189=CARTESIAN_POINT('Ctrl Pts',(104.567655925523,17.9856849271578,33.752120102763));
#71190=CARTESIAN_POINT('Ctrl Pts',(104.459564357693,17.9315947959052,33.6584329578312));
#71191=CARTESIAN_POINT('Ctrl Pts',(104.351473262602,17.8775040493509,33.5647456205277));
#71192=CARTESIAN_POINT('Ctrl Pts',(104.243382456862,17.8234135359081,33.4710578085036));
#71193=CARTESIAN_POINT('Ctrl Pts',(104.455001570347,17.9833187182834,33.8834541246487));
#71194=CARTESIAN_POINT('Ctrl Pts',(104.346904020691,17.9292246547841,33.789775506513));
#71195=CARTESIAN_POINT('Ctrl Pts',(104.238806667407,17.8751305285007,33.6960966825317));
#71196=CARTESIAN_POINT('Ctrl Pts',(104.130709774609,17.8210360125183,33.6024175423752));
#71197=CARTESIAN_POINT('Ctrl Pts',(104.410455468831,17.8659835447084,34.0025898869996));
#71198=CARTESIAN_POINT('Ctrl Pts',(104.302362090342,17.8118754705986,33.908914286335));
#71199=CARTESIAN_POINT('Ctrl Pts',(104.194269413732,17.7577669311554,33.8152381372974));
#71200=CARTESIAN_POINT('Ctrl Pts',(104.086176765824,17.7036581615694,33.72156206328));
#71201=CARTESIAN_POINT('Ctrl Pts',(104.412132034356,17.7958762791241,34.041132103426));
#71202=CARTESIAN_POINT('Ctrl Pts',(104.304043604523,17.7417622963114,33.9474542173515));
#71203=CARTESIAN_POINT('Ctrl Pts',(104.195955578132,17.6876479205194,33.8537760772191));
#71204=CARTESIAN_POINT('Ctrl Pts',(104.087867965647,17.63353314151,33.7600976763372));
#71205=CARTESIAN_POINT('',(104.300000000003,17.7951300341907,33.4220693465132));
#71206=CARTESIAN_POINT('Origin',(104.300000000003,17.5353224130554,33.5720693465132));
#71207=CARTESIAN_POINT('',(104.624264068712,17.9574056939141,33.7031390339859));
#71208=CARTESIAN_POINT('Origin',(104.624264068712,17.6975980727788,33.8531390339859));
#71209=CARTESIAN_POINT('Ctrl Pts',(104.624264068712,17.9574056939141,33.7031390339859));
#71210=CARTESIAN_POINT('Ctrl Pts',(104.516175638879,17.9033140106251,33.6094494902625));
#71211=CARTESIAN_POINT('Ctrl Pts',(104.408087612488,17.8492221257921,33.5157595974544));
#71212=CARTESIAN_POINT('Ctrl Pts',(104.300000000003,17.7951300341907,33.4220693465132));
#71213=CARTESIAN_POINT('Origin',(104.3,12.8018593539449,25.3734708323834));
#71214=CARTESIAN_POINT('Origin',(104.3,17.5353224130539,33.5720693465106));
#71215=CARTESIAN_POINT('',(104.3,17.1241669750802,32.259927238132));
#71216=CARTESIAN_POINT('',(104.3,13.0616669750802,25.2234708323834));
#71217=CARTESIAN_POINT('Origin',(104.3,16.7143593539449,32.1501196169967));
#71218=CARTESIAN_POINT('Origin',(104.3,17.5353224130539,33.5720693465106));
#71219=CARTESIAN_POINT('Origin',(104.624264068712,17.6975980727788,33.8531390339859));
#71220=CARTESIAN_POINT('Origin',(104.624264068712,17.6975980727788,33.8531390339859));
#71221=CARTESIAN_POINT('Origin',(113.,15.6473429640468,34.3789638902265));
#71222=CARTESIAN_POINT('',(121.7,15.1689886735905,33.2241144745873));
#71223=CARTESIAN_POINT('',(103.5,15.1689886735905,33.2241144745873));
#71224=CARTESIAN_POINT('Origin',(121.7,15.0541836438809,32.946950614834));
#71225=CARTESIAN_POINT('',(121.912131484566,15.7681469233145,34.670610447079));
#71226=CARTESIAN_POINT('Ctrl Pts',(121.912131759621,15.7681470285123,34.6706107010489));
#71227=CARTESIAN_POINT('Ctrl Pts',(121.938311286558,15.7581227425572,34.6464099339429));
#71228=CARTESIAN_POINT('Ctrl Pts',(121.962987211232,15.7439817050434,34.612270449391));
#71229=CARTESIAN_POINT('Ctrl Pts',(121.991329280155,15.7177881174267,34.5490335349196));
#71230=CARTESIAN_POINT('Ctrl Pts',(122.,15.7010994022092,34.5087434123029));
#71231=CARTESIAN_POINT('Ctrl Pts',(122.,15.686919915995,34.4745111043772));
#71232=CARTESIAN_POINT('',(121.75,15.8302278233913,34.8204869980086));
#71233=CARTESIAN_POINT('Origin',(113.,8.33272992328157,37.2800967276863));
#71234=CARTESIAN_POINT('',(121.811388243054,8.62250767116829,37.2024510141556));
#71235=CARTESIAN_POINT('Ctrl Pts',(121.5,8.39817021063718,37.5728723564378));
#71236=CARTESIAN_POINT('Ctrl Pts',(121.5,8.41846306187312,37.5683365621785));
#71237=CARTESIAN_POINT('Ctrl Pts',(121.502178291748,8.43844642422115,37.5616201820783));
#71238=CARTESIAN_POINT('Ctrl Pts',(121.510716614322,8.47626683430665,37.5443504602798));
#71239=CARTESIAN_POINT('Ctrl Pts',(121.517077828304,8.49410315611481,37.533796113814));
#71240=CARTESIAN_POINT('Ctrl Pts',(121.541159186122,8.54274436268672,37.4980708374905));
#71241=CARTESIAN_POINT('Ctrl Pts',(121.56412779323,8.56856437653815,37.4686076043297));
#71242=CARTESIAN_POINT('Ctrl Pts',(121.617288389766,8.60866399825099,37.4048701574215));
#71243=CARTESIAN_POINT('Ctrl Pts',(121.652509215907,8.62308008690723,37.3653949038344));
#71244=CARTESIAN_POINT('Ctrl Pts',(121.726559498935,8.63532117790983,37.2865621995426));
#71245=CARTESIAN_POINT('Ctrl Pts',(121.765406035132,8.63305961883982,37.2472073755322));
#71246=CARTESIAN_POINT('Ctrl Pts',(121.804557793905,8.62421947088419,37.2090666886064));
#71247=CARTESIAN_POINT('Ctrl Pts',(121.807962616873,8.62339502798056,37.2057626944961));
#71248=CARTESIAN_POINT('Ctrl Pts',(121.811388687965,8.62250778625268,37.2024514436577));
#71249=CARTESIAN_POINT('',(113.,8.62250767116829,37.2024510141556));
#71250=CARTESIAN_POINT('Origin',(113.,8.51471537844438,36.8001647010456));
#71251=CARTESIAN_POINT('',(121.912131484566,8.59641832855392,37.1050842619827));
#71252=CARTESIAN_POINT('',(121.75,8.63840530242858,37.261781781739));
#71253=CARTESIAN_POINT('Ctrl Pts',(122.,8.54148233004193,36.9000603243714));
#71254=CARTESIAN_POINT('Ctrl Pts',(122.,8.55107229598144,36.9358505645005));
#71255=CARTESIAN_POINT('Ctrl Pts',(121.991329280155,8.56235932063752,36.9779743139833));
#71256=CARTESIAN_POINT('Ctrl Pts',(121.962987211232,8.58007474482734,37.0440891771373));
#71257=CARTESIAN_POINT('Ctrl Pts',(121.938311286558,8.58963870688199,37.0797823694469));
#71258=CARTESIAN_POINT('Ctrl Pts',(121.912131759621,8.59641839970201,37.105084527511));
#71259=CARTESIAN_POINT('',(121.7,8.19119157206623,35.5927574181843));
#71260=CARTESIAN_POINT('Origin',(121.7,8.11354585853547,35.3029796702975));
#71261=CARTESIAN_POINT('',(103.5,8.19119157206623,35.5927574181843));
#71262=CARTESIAN_POINT('Origin',(104.3,-2.71526964499761,4.97801134479456));
#71263=CARTESIAN_POINT('',(104.3,-25.8390437558097,27.6775213868948));
#71264=CARTESIAN_POINT('Origin',(104.3,-25.6269117214538,27.8896534212507));
#71265=CARTESIAN_POINT('',(104.3,-24.8901586977665,26.7286363288515));
#71266=CARTESIAN_POINT('Origin',(104.3,-24.4658946290545,26.7286363288515));
#71267=CARTESIAN_POINT('',(104.3,-2.92740167935357,4.7658793104386));
#71268=CARTESIAN_POINT('Ctrl Pts',(104.300000000002,-25.8390437558114,27.6775213868965));
#71269=CARTESIAN_POINT('Ctrl Pts',(104.408087612488,-25.9155415253719,27.7540191564569));
#71270=CARTESIAN_POINT('Ctrl Pts',(104.51617563888,-25.9920390025178,27.8305166336028));
#71271=CARTESIAN_POINT('Ctrl Pts',(104.624264068714,-26.0685361946373,27.9070138257223));
#71272=CARTESIAN_POINT('Ctrl Pts',(104.243382456862,-25.8790426675315,27.7175202986166));
#71273=CARTESIAN_POINT('Ctrl Pts',(104.351473262603,-25.9555382814697,27.7940161208215));
#71274=CARTESIAN_POINT('Ctrl Pts',(104.459564357694,-26.0320339977095,27.8705114241477));
#71275=CARTESIAN_POINT('Ctrl Pts',(104.567655925525,-26.108529069824,27.947006700909));
#71276=CARTESIAN_POINT('Ctrl Pts',(104.130710113065,-25.9107439897146,27.8450194956664));
#71277=CARTESIAN_POINT('Ctrl Pts',(104.238807005864,-25.9872412253646,27.9215059055569));
#71278=CARTESIAN_POINT('Ctrl Pts',(104.346904358902,-26.0637380030864,27.9979921109243));
#71279=CARTESIAN_POINT('Ctrl Pts',(104.455001908559,-26.1402346665623,28.0744781336926));
#71280=CARTESIAN_POINT('Ctrl Pts',(104.086176765823,-25.8282031306363,27.9904837995326));
#71281=CARTESIAN_POINT('Ctrl Pts',(104.194269413732,-25.9047133406349,28.0669635586562));
#71282=CARTESIAN_POINT('Ctrl Pts',(104.302362090344,-25.9812233477493,28.1434434498089));
#71283=CARTESIAN_POINT('Ctrl Pts',(104.410455468833,-26.0577327634567,28.2199229317112));
#71284=CARTESIAN_POINT('Ctrl Pts',(104.087867965646,-25.7704413132658,28.045856034146));
#71285=CARTESIAN_POINT('Ctrl Pts',(104.195955578132,-25.8469579301585,28.1223364854948));
#71286=CARTESIAN_POINT('Ctrl Pts',(104.304043604524,-25.9234740900862,28.1988167893393));
#71287=CARTESIAN_POINT('Ctrl Pts',(104.412132034358,-25.9999898046701,28.2752969494932));
#71288=CARTESIAN_POINT('',(104.624264068714,-26.0685361946373,27.9070138257223));
#71289=CARTESIAN_POINT('',(104.412132034358,-25.9999898046693,28.2752969494924));
#71290=CARTESIAN_POINT('Origin',(104.624264068714,-25.8564041602813,28.1191458600783));
#71291=CARTESIAN_POINT('',(104.087867965646,-25.770441313265,28.0458560341451));
#71292=CARTESIAN_POINT('Ctrl Pts',(104.412132034358,-25.9999898046701,28.2752969494932));
#71293=CARTESIAN_POINT('Ctrl Pts',(104.304043604524,-25.9234740900862,28.1988167893393));
#71294=CARTESIAN_POINT('Ctrl Pts',(104.195955578132,-25.8469579301585,28.1223364854948));
#71295=CARTESIAN_POINT('Ctrl Pts',(104.087867965646,-25.7704413132658,28.045856034146));
#71296=CARTESIAN_POINT('Origin',(104.300000000002,-25.6269117214555,27.8896534212524));
#71297=CARTESIAN_POINT('Ctrl Pts',(104.300000000002,-25.8390437558114,27.6775213868965));
#71298=CARTESIAN_POINT('Ctrl Pts',(104.408087612488,-25.9155415253719,27.7540191564569));
#71299=CARTESIAN_POINT('Ctrl Pts',(104.51617563888,-25.9920390025178,27.8305166336028));
#71300=CARTESIAN_POINT('Ctrl Pts',(104.624264068714,-26.0685361946373,27.9070138257223));
#71301=CARTESIAN_POINT('Origin',(104.3,-25.6269117214538,27.8896534212507));
#71302=CARTESIAN_POINT('Origin',(104.3,-25.6269117214538,27.8896534212507));
#71303=CARTESIAN_POINT('Origin',(113.,-25.8564041602797,28.1191458600767));
#71304=CARTESIAN_POINT('',(121.811388243054,-26.0685361946357,27.9070138257207));
#71305=CARTESIAN_POINT('',(121.5,-26.0594649259364,28.3399768485066));
#71306=CARTESIAN_POINT('Ctrl Pts',(121.811388687965,-26.0685365090528,27.9070141401383));
#71307=CARTESIAN_POINT('Ctrl Pts',(121.80796264376,-26.070960489325,27.9094381275961));
#71308=CARTESIAN_POINT('Ctrl Pts',(121.80455782351,-26.0733264736922,27.9118872463663));
#71309=CARTESIAN_POINT('Ctrl Pts',(121.765406035132,-26.1000526300669,27.9404979978181));
#71310=CARTESIAN_POINT('Ctrl Pts',(121.726559498935,-26.1216886096789,27.9734494956375));
#71311=CARTESIAN_POINT('Ctrl Pts',(121.652509215907,-26.1505038660466,28.0478411657046));
#71312=CARTESIAN_POINT('Ctrl Pts',(121.617288389766,-26.1577567938406,28.0892357824599));
#71313=CARTESIAN_POINT('Ctrl Pts',(121.56412779323,-26.1548982262093,28.1644838415113));
#71314=CARTESIAN_POINT('Ctrl Pts',(121.541159186122,-26.1472690548682,28.2029097568319));
#71315=CARTESIAN_POINT('Ctrl Pts',(121.517077828304,-26.123007172468,28.2581693569711));
#71316=CARTESIAN_POINT('Ctrl Pts',(121.510716614322,-26.1128376379049,28.2762278500349));
#71317=CARTESIAN_POINT('Ctrl Pts',(121.502178291748,-26.0887190628886,28.3100940728715));
#71318=CARTESIAN_POINT('Ctrl Pts',(121.5,-26.0747711534923,28.3259023098338));
#71319=CARTESIAN_POINT('Ctrl Pts',(121.5,-26.0594649259364,28.3399768485066));
#71320=CARTESIAN_POINT('',(104.624264068712,-26.0594649259364,28.3399768485066));
#71321=CARTESIAN_POINT('',(113.,-26.0594649259364,28.3399768485066));
#71322=CARTESIAN_POINT('Origin',(104.624264068712,-25.8564041602797,28.1191458600767));
#71323=CARTESIAN_POINT('',(113.,-26.0685361946357,27.9070138257207));
#71324=CARTESIAN_POINT('Origin',(104.624264068712,-25.8564041602798,28.1191458600766));
#71325=CARTESIAN_POINT('Origin',(104.624264068712,-25.8564041602798,28.1191458600766));
#71326=CARTESIAN_POINT('Origin',(104.3,0.,0.));
#71327=CARTESIAN_POINT('',(104.087867965647,-24.4422022714321,29.2106904110607));
#71328=CARTESIAN_POINT('Origin',(104.087867965644,0.,0.));
#71329=CARTESIAN_POINT('Origin',(104.3,-24.3060703646347,29.0480002025284));
#71330=CARTESIAN_POINT('Origin',(104.25,0.,0.));
#71331=CARTESIAN_POINT('',(104.412132034356,-24.6397181974285,29.4682231323184));
#71332=CARTESIAN_POINT('Origin',(104.412132034356,-2.22044604925031E-15,
-2.22044604925031E-15));
#71333=CARTESIAN_POINT('Ctrl Pts',(104.087867965647,-24.4422022714329,29.2106904110617));
#71334=CARTESIAN_POINT('Ctrl Pts',(104.195955578132,-24.5080409992732,29.2965351197829));
#71335=CARTESIAN_POINT('Ctrl Pts',(104.304043604523,-24.5738796405169,29.3823793561953));
#71336=CARTESIAN_POINT('Ctrl Pts',(104.412132034356,-24.6397181974285,29.4682231323184));
#71337=CARTESIAN_POINT('Origin',(104.624264068712,0.,0.));
#71338=CARTESIAN_POINT('',(104.624264068712,-24.6960816898302,29.5356318566107));
#71339=CARTESIAN_POINT('Origin',(104.624264068712,0.,0.));
#71340=CARTESIAN_POINT('Origin',(104.624264068712,-24.5036446896497,29.3054840759098));
#71341=CARTESIAN_POINT('Origin',(113.,0.,0.));
#71342=CARTESIAN_POINT('',(121.5,-24.6960816898302,29.5356318566107));
#71343=CARTESIAN_POINT('Origin',(121.5,0.,0.));
#71344=CARTESIAN_POINT('',(113.,-24.6960816898302,29.5356318566107));
#71345=CARTESIAN_POINT('Origin',(104.3,-1.29622949643128,2.59589931010294));
#71346=CARTESIAN_POINT('',(104.3,-32.1220693465106,20.0467960840288));
#71347=CARTESIAN_POINT('Origin',(104.3,-31.9720693465106,20.3066037051641));
#71348=CARTESIAN_POINT('',(104.3,-30.959927238132,19.3758330249198));
#71349=CARTESIAN_POINT('Origin',(104.3,-30.5501196169967,19.4856406460551));
#71350=CARTESIAN_POINT('',(104.3,-1.44622949643128,2.3360916889676));
#71351=CARTESIAN_POINT('Ctrl Pts',(104.300000000003,-32.122069346513,20.0467960840302));
#71352=CARTESIAN_POINT('Ctrl Pts',(104.408087612489,-32.2157595974551,20.100888175632));
#71353=CARTESIAN_POINT('Ctrl Pts',(104.51617563888,-32.3094494902639,20.1549800604655));
#71354=CARTESIAN_POINT('Ctrl Pts',(104.624264068715,-32.4031390339881,20.2090717437549));
#71355=CARTESIAN_POINT('Ctrl Pts',(104.243382456862,-32.1710578085035,20.0750795857475));
#71356=CARTESIAN_POINT('Ctrl Pts',(104.351473262603,-32.2647454732615,20.1291703542645));
#71357=CARTESIAN_POINT('Ctrl Pts',(104.459564357695,-32.3584331025398,20.1832605951055));
#71358=CARTESIAN_POINT('Ctrl Pts',(104.567655925525,-32.4521201027652,20.2373509769986));
#71359=CARTESIAN_POINT('Ctrl Pts',(104.130709934827,-32.2346784312497,20.1900293243368));
#71360=CARTESIAN_POINT('Ctrl Pts',(104.238806827626,-32.3283652263749,20.2441105815263));
#71361=CARTESIAN_POINT('Ctrl Pts',(104.346904180794,-32.4220515260737,20.2981917597176));
#71362=CARTESIAN_POINT('Ctrl Pts',(104.455001730451,-32.5157376683266,20.3522727910653));
#71363=CARTESIAN_POINT('Ctrl Pts',(104.086176765824,-32.1925987394747,20.3519003213093));
#71364=CARTESIAN_POINT('Ctrl Pts',(104.194269413732,-32.2862963455132,20.4059717963427));
#71365=CARTESIAN_POINT('Ctrl Pts',(104.302362090344,-32.3799937897523,20.4600434514167));
#71366=CARTESIAN_POINT('Ctrl Pts',(104.410455468833,-32.4736905568142,20.5141148642526));
#71367=CARTESIAN_POINT('Ctrl Pts',(104.087867965647,-32.151136497191,20.4203356511969));
#71368=CARTESIAN_POINT('Ctrl Pts',(104.195955578133,-32.2448404709751,20.4744061366423));
#71369=CARTESIAN_POINT('Ctrl Pts',(104.304043604524,-32.3385439651879,20.5284765978808));
#71370=CARTESIAN_POINT('Ctrl Pts',(104.412132034359,-32.4322469920416,20.5825470355882));
#71371=CARTESIAN_POINT('',(104.624264068715,-32.4031390339881,20.2090717437549));
#71372=CARTESIAN_POINT('',(104.412132034359,-32.4322469920405,20.5825470355875));
#71373=CARTESIAN_POINT('Origin',(104.624264068715,-32.2531390339881,20.4688793648903));
#71374=CARTESIAN_POINT('',(104.087867965647,-32.1511364971898,20.4203356511961));
#71375=CARTESIAN_POINT('Ctrl Pts',(104.412132034359,-32.4322469920416,20.5825470355882));
#71376=CARTESIAN_POINT('Ctrl Pts',(104.304043604524,-32.3385439651879,20.5284765978808));
#71377=CARTESIAN_POINT('Ctrl Pts',(104.195955578133,-32.2448404709751,20.4744061366423));
#71378=CARTESIAN_POINT('Ctrl Pts',(104.087867965647,-32.151136497191,20.4203356511969));
#71379=CARTESIAN_POINT('Origin',(104.300000000003,-31.972069346513,20.3066037051655));
#71380=CARTESIAN_POINT('Ctrl Pts',(104.300000000003,-32.122069346513,20.0467960840302));
#71381=CARTESIAN_POINT('Ctrl Pts',(104.408087612489,-32.2157595974551,20.100888175632));
#71382=CARTESIAN_POINT('Ctrl Pts',(104.51617563888,-32.3094494902639,20.1549800604655));
#71383=CARTESIAN_POINT('Ctrl Pts',(104.624264068715,-32.4031390339881,20.2090717437549));
#71384=CARTESIAN_POINT('Origin',(104.3,-31.9720693465106,20.3066037051641));
#71385=CARTESIAN_POINT('Origin',(104.3,-31.9720693465106,20.3066037051641));
#71386=CARTESIAN_POINT('Origin',(113.,-32.2531390339859,20.468879364889));
#71387=CARTESIAN_POINT('',(121.811388243054,-32.4031390339859,20.2090717437537));
#71388=CARTESIAN_POINT('',(121.5,-32.5064359373941,20.6296297263933));
#71389=CARTESIAN_POINT('Ctrl Pts',(121.811388687965,-32.4031394190667,20.2090719660805));
#71390=CARTESIAN_POINT('Ctrl Pts',(121.80796264376,-32.4061081783332,20.2107859859092));
#71391=CARTESIAN_POINT('Ctrl Pts',(121.80455782351,-32.4090274223195,20.2125392911663));
#71392=CARTESIAN_POINT('Ctrl Pts',(121.765406035132,-32.4422479143698,20.233257916631));
#71393=CARTESIAN_POINT('Ctrl Pts',(121.726559498935,-32.4716751410544,20.2594868158067));
#71394=CARTESIAN_POINT('Ctrl Pts',(121.652509215907,-32.5187625223814,20.3238857140478));
#71395=CARTESIAN_POINT('Ctrl Pts',(121.617288389766,-32.5364820278348,20.3619926475953));
#71396=CARTESIAN_POINT('Ctrl Pts',(121.56412779323,-32.553196494323,20.4354165429558));
#71397=CARTESIAN_POINT('Ctrl Pts',(121.541159186122,-32.555772639402,20.4745077018041));
#71398=CARTESIAN_POINT('Ctrl Pts',(121.517077828304,-32.546639697538,20.5341638139643));
#71399=CARTESIAN_POINT('Ctrl Pts',(121.510716614322,-32.5414905633929,20.5542390480232));
#71400=CARTESIAN_POINT('Ctrl Pts',(121.502178291748,-32.5269590323472,20.5931936538549));
#71401=CARTESIAN_POINT('Ctrl Pts',(121.5,-32.5175778592339,20.612073222796));
#71402=CARTESIAN_POINT('Ctrl Pts',(121.5,-32.5064359373941,20.6296297263933));
#71403=CARTESIAN_POINT('',(104.624264068712,-32.5064359373941,20.6296297263933));
#71404=CARTESIAN_POINT('',(113.,-32.5064359373941,20.6296297263933));
#71405=CARTESIAN_POINT('Origin',(104.624264068712,-32.2531390339859,20.468879364889));
#71406=CARTESIAN_POINT('',(113.,-32.4031390339859,20.2090717437536));
#71407=CARTESIAN_POINT('Origin',(104.624264068712,-32.2531390339859,20.4688793648889));
#71408=CARTESIAN_POINT('Origin',(104.624264068712,-32.2531390339859,20.4688793648889));
#71409=CARTESIAN_POINT('Origin',(104.3,0.,0.));
#71410=CARTESIAN_POINT('',(104.087867965647,-31.1696374243337,21.8892528196833));
#71411=CARTESIAN_POINT('Origin',(104.087867965644,0.,0.));
#71412=CARTESIAN_POINT('Origin',(104.3,-30.9960367753563,21.7673396757028));
#71413=CARTESIAN_POINT('Origin',(104.25,0.,0.));
#71414=CARTESIAN_POINT('',(104.412132034356,-31.4270775313556,22.0868894429017));
#71415=CARTESIAN_POINT('Origin',(104.412132034356,2.22044604925031E-15,
2.22044604925031E-15));
#71416=CARTESIAN_POINT('Ctrl Pts',(104.087867965647,-31.1696374243348,21.889252819684));
#71417=CARTESIAN_POINT('Ctrl Pts',(104.195955578132,-31.255450997464,21.9551321242177));
#71418=CARTESIAN_POINT('Ctrl Pts',(104.304043604523,-31.341264364705,22.021010994949));
#71419=CARTESIAN_POINT('Ctrl Pts',(104.412132034356,-31.4270775313556,22.0868894429017));
#71420=CARTESIAN_POINT('Origin',(104.624264068712,0.,0.));
#71421=CARTESIAN_POINT('',(104.624264068712,-31.4989671459791,22.1374133253307));
#71422=CARTESIAN_POINT('Origin',(104.624264068712,0.,0.));
#71423=CARTESIAN_POINT('Origin',(104.624264068712,-31.2535206487377,21.9649140007177));
#71424=CARTESIAN_POINT('Origin',(113.,0.,0.));
#71425=CARTESIAN_POINT('',(121.5,-31.4989671459791,22.1374133253307));
#71426=CARTESIAN_POINT('Origin',(121.5,0.,0.));
#71427=CARTESIAN_POINT('',(113.,-31.4989671459791,22.1374133253307));
#71428=CARTESIAN_POINT('Origin',(121.7,-6.28498798269814,10.9923017395774));
#71429=CARTESIAN_POINT('',(121.7,-15.6825215664905,34.4638925493513));
#71430=CARTESIAN_POINT('Origin',(121.7,-15.9596854262438,34.3490875196417));
#71431=CARTESIAN_POINT('',(121.7,-15.1689886735904,33.2241144745874));
#71432=CARTESIAN_POINT('Origin',(121.7,-15.3313475036343,32.8321455851244));
#71433=CARTESIAN_POINT('',(121.7,-6.00782412294476,11.1071067692869));
#71434=CARTESIAN_POINT('Ctrl Pts',(121.699999999997,-15.6825215664917,34.4638925493543));
#71435=CARTESIAN_POINT('Ctrl Pts',(121.591912387511,-15.7239218610477,34.5638417019577));
#71436=CARTESIAN_POINT('Ctrl Pts',(121.483824361119,-15.7653219973501,34.6637904725029));
#71437=CARTESIAN_POINT('Ctrl Pts',(121.375735931285,-15.8067219793973,34.7637388706433));
#71438=CARTESIAN_POINT('Ctrl Pts',(121.756617543137,-15.7041688215247,34.5161536460432));
#71439=CARTESIAN_POINT('Ctrl Pts',(121.648526737397,-15.7455681418798,34.6161000618904));
#71440=CARTESIAN_POINT('Ctrl Pts',(121.540435642305,-15.7869669437042,34.7160463736859));
#71441=CARTESIAN_POINT('Ctrl Pts',(121.432344074474,-15.828365967482,34.8159920802212));
#71442=CARTESIAN_POINT('Ctrl Pts',(121.869288077041,-15.8098327514129,34.5942310582327));
#71443=CARTESIAN_POINT('Ctrl Pts',(121.761191184242,-15.851222755321,34.6941753704096));
#71444=CARTESIAN_POINT('Ctrl Pts',(121.653093832523,-15.8926127449365,34.7941191828858));
#71445=CARTESIAN_POINT('Ctrl Pts',(121.544996282866,-15.9340026101519,34.8940628182975));
#71446=CARTESIAN_POINT('Ctrl Pts',(121.913823234176,-15.9758096616226,34.5736426479042));
#71447=CARTESIAN_POINT('Ctrl Pts',(121.805730586267,-16.017188555955,34.6735964016779));
#71448=CARTESIAN_POINT('Ctrl Pts',(121.697637909656,-16.0585676499069,34.7735500185365));
#71449=CARTESIAN_POINT('Ctrl Pts',(121.589544531166,-16.0999465920823,34.8735029323928));
#71450=CARTESIAN_POINT('Ctrl Pts',(121.912132034353,-16.0490714263823,34.5414677238745));
#71451=CARTESIAN_POINT('Ctrl Pts',(121.804044421867,-16.0904485084352,34.6414276617498));
#71452=CARTESIAN_POINT('Ctrl Pts',(121.695956395475,-16.1318256290849,34.7413871209968));
#71453=CARTESIAN_POINT('Ctrl Pts',(121.587867965641,-16.1732027874074,34.8413461138118));
#71454=CARTESIAN_POINT('',(121.375735931285,-15.8067219793973,34.7637388706433));
#71455=CARTESIAN_POINT('',(121.587867965641,-16.1732027874068,34.8413461138104));
#71456=CARTESIAN_POINT('Origin',(121.375735931285,-16.0838858391507,34.6489338409338));
#71457=CARTESIAN_POINT('',(121.912132034353,-16.0490714263816,34.541467723873));
#71458=CARTESIAN_POINT('Ctrl Pts',(121.587867965641,-16.1732027874074,34.8413461138118));
#71459=CARTESIAN_POINT('Ctrl Pts',(121.695956395475,-16.1318256290849,34.7413871209968));
#71460=CARTESIAN_POINT('Ctrl Pts',(121.804044421867,-16.0904485084352,34.6414276617498));
#71461=CARTESIAN_POINT('Ctrl Pts',(121.912132034353,-16.0490714263823,34.5414677238745));
#71462=CARTESIAN_POINT('Origin',(121.699999999997,-15.9596854262451,34.3490875196448));
#71463=CARTESIAN_POINT('Ctrl Pts',(121.699999999997,-15.6825215664917,34.4638925493543));
#71464=CARTESIAN_POINT('Ctrl Pts',(121.591912387511,-15.7239218610477,34.5638417019577));
#71465=CARTESIAN_POINT('Ctrl Pts',(121.483824361119,-15.7653219973501,34.6637904725029));
#71466=CARTESIAN_POINT('Ctrl Pts',(121.375735931285,-15.8067219793973,34.7637388706433));
#71467=CARTESIAN_POINT('Origin',(121.7,-15.9596854262438,34.3490875196417));
#71468=CARTESIAN_POINT('Origin',(121.7,-15.9596854262438,34.3490875196417));
#71469=CARTESIAN_POINT('Origin',(113.,-16.0838858391495,34.6489338409309));
#71470=CARTESIAN_POINT('',(104.188611756946,-15.8067219793961,34.7637388706404));
#71471=CARTESIAN_POINT('',(104.5,-16.210199078724,34.9210458868021));
#71472=CARTESIAN_POINT('Ctrl Pts',(104.188611312035,-15.8067221495578,34.7637392814463));
#71473=CARTESIAN_POINT('Ctrl Pts',(104.19203735624,-15.8080340048666,34.7669063670474));
#71474=CARTESIAN_POINT('Ctrl Pts',(104.19544217649,-15.8093912725525,34.7700294887557));
#71475=CARTESIAN_POINT('Ctrl Pts',(104.234593964868,-15.8255965029732,34.8056700981812));
#71476=CARTESIAN_POINT('Ctrl Pts',(104.273440501065,-15.8477599864337,34.8382691291977));
#71477=CARTESIAN_POINT('Ctrl Pts',(104.347490784093,-15.9054618065867,34.8933594144204));
#71478=CARTESIAN_POINT('Ctrl Pts',(104.382711610234,-15.9409298704602,34.9159012799815));
#71479=CARTESIAN_POINT('Ctrl Pts',(104.43587220677,-16.0115439385517,34.9420564933711));
#71480=CARTESIAN_POINT('Ctrl Pts',(104.458840813878,-16.0499644127093,34.9497130192858));
#71481=CARTESIAN_POINT('Ctrl Pts',(104.482922171696,-16.1103022466853,34.9484448961684));
#71482=CARTESIAN_POINT('Ctrl Pts',(104.489283385678,-16.1308778312071,34.9459601574395));
#71483=CARTESIAN_POINT('Ctrl Pts',(104.497821708252,-16.1713959204003,34.9366375420249));
#71484=CARTESIAN_POINT('Ctrl Pts',(104.5,-16.1913384608169,34.9298009043927));
#71485=CARTESIAN_POINT('Ctrl Pts',(104.5,-16.210199078724,34.9210458868021));
#71486=CARTESIAN_POINT('',(121.375735931288,-16.210199078724,34.9210458868021));
#71487=CARTESIAN_POINT('',(113.,-16.210199078724,34.9210458868021));
#71488=CARTESIAN_POINT('Origin',(121.375735931288,-16.0838858391495,34.6489338409309));
#71489=CARTESIAN_POINT('',(113.,-15.8067219793961,34.7637388706404));
#71490=CARTESIAN_POINT('Origin',(121.375735931288,-16.0838858391494,34.648933840931));
#71491=CARTESIAN_POINT('Origin',(121.375735931288,-16.0838858391494,34.648933840931));
#71492=CARTESIAN_POINT('Origin',(121.7,0.,0.));
#71493=CARTESIAN_POINT('',(121.912132034353,-17.6335331415093,33.7600976763358));
#71494=CARTESIAN_POINT('Origin',(121.912132034356,-1.11022302462516E-15,
0.));
#71495=CARTESIAN_POINT('Origin',(121.7,-17.535322413054,33.5720693465106));
#71496=CARTESIAN_POINT('Origin',(121.75,0.,0.));
#71497=CARTESIAN_POINT('',(121.587867965644,-17.7958762791241,34.041132103426));
#71498=CARTESIAN_POINT('Origin',(121.587867965644,-2.22044604925031E-15,
0.));
#71499=CARTESIAN_POINT('Ctrl Pts',(121.912132034353,-17.63353314151,33.7600976763372));
#71500=CARTESIAN_POINT('Ctrl Pts',(121.804044421868,-17.6876479205194,33.8537760772191));
#71501=CARTESIAN_POINT('Ctrl Pts',(121.695956395477,-17.7417622963114,33.9474542173515));
#71502=CARTESIAN_POINT('Ctrl Pts',(121.587867965644,-17.7958762791241,34.041132103426));
#71503=CARTESIAN_POINT('Ctrl Pts',(104.624264068712,-11.1339148195199,36.529521496889));
#71504=CARTESIAN_POINT('Ctrl Pts',(104.516175638879,-11.1059149038863,36.4250243891369));
#71505=CARTESIAN_POINT('Ctrl Pts',(104.408087612489,-11.0779148839258,36.3205268920315));
#71506=CARTESIAN_POINT('Ctrl Pts',(104.300000000004,-11.0499147569342,36.2160289954803));
#71507=CARTESIAN_POINT('Ctrl Pts',(104.567655925523,-11.1485532278086,36.5841527803644));
#71508=CARTESIAN_POINT('Ctrl Pts',(104.459564357693,-11.1205539109213,36.4796584662696));
#71509=CARTESIAN_POINT('Ctrl Pts',(104.351473262603,-11.0925548930909,36.3751635810633));
#71510=CARTESIAN_POINT('Ctrl Pts',(104.243382456864,-11.0645553747475,36.2706685250137));
#71511=CARTESIAN_POINT('Ctrl Pts',(104.455001016882,-11.2430929770909,36.6753475262196));
#71512=CARTESIAN_POINT('Ctrl Pts',(104.346903467226,-11.2151024700774,36.5708564609618));
#71513=CARTESIAN_POINT('Ctrl Pts',(104.238806113538,-11.1871118616628,36.4663652062277));
#71514=CARTESIAN_POINT('Ctrl Pts',(104.130709220741,-11.1591213054788,36.3618734518916));
#71515=CARTESIAN_POINT('Ctrl Pts',(104.410455468831,-11.410303769972,36.6766200040331));
#71516=CARTESIAN_POINT('Ctrl Pts',(104.302362090343,-11.3823253036304,36.5721211654519));
#71517=CARTESIAN_POINT('Ctrl Pts',(104.194269413732,-11.354346778571,36.4676216100719));
#71518=CARTESIAN_POINT('Ctrl Pts',(104.086176765825,-11.3263684692943,36.3631219450038));
#71519=CARTESIAN_POINT('Ctrl Pts',(104.412132034356,-11.4871305554741,36.6543001437251));
#71520=CARTESIAN_POINT('Ctrl Pts',(104.304043604523,-11.4591546511876,36.5497955110311));
#71521=CARTESIAN_POINT('Ctrl Pts',(104.195955578133,-11.4311788451333,36.4452904208127));
#71522=CARTESIAN_POINT('Ctrl Pts',(104.087867965648,-11.403203139819,36.3407848610988));
#71523=CARTESIAN_POINT('',(104.300000000004,-11.0499147569342,36.2160289954803));
#71524=CARTESIAN_POINT('Origin',(104.300000000004,-11.3396925048209,36.1383832819495));
#71525=CARTESIAN_POINT('',(104.624264068712,-11.1339148195199,36.529521496889));
#71526=CARTESIAN_POINT('Origin',(104.624264068712,-11.4236925674066,36.4518757833583));
#71527=CARTESIAN_POINT('Ctrl Pts',(104.624264068712,-11.1339148195199,36.529521496889));
#71528=CARTESIAN_POINT('Ctrl Pts',(104.516175638879,-11.1059149038863,36.4250243891369));
#71529=CARTESIAN_POINT('Ctrl Pts',(104.408087612489,-11.0779148839258,36.3205268920315));
#71530=CARTESIAN_POINT('Ctrl Pts',(104.300000000004,-11.0499147569342,36.2160289954803));
#71531=CARTESIAN_POINT('Origin',(104.3,-5.15793213432475,13.0677394990421));
#71532=CARTESIAN_POINT('Origin',(104.3,-11.3396925048198,36.1383832819455));
#71533=CARTESIAN_POINT('',(104.3,-10.7025987204178,34.9198279009177));
#71534=CARTESIAN_POINT('',(104.3,-4.86815438643803,13.1453852125729));
#71535=CARTESIAN_POINT('Origin',(104.3,-10.9147307547738,34.5524044395002));
#71536=CARTESIAN_POINT('Origin',(104.3,-11.3396925048198,36.1383832819455));
#71537=CARTESIAN_POINT('Origin',(104.624264068712,-11.4236925674066,36.4518757833583));
#71538=CARTESIAN_POINT('Origin',(104.624264068712,-11.4236925674066,36.4518757833583));
#71539=CARTESIAN_POINT('Origin',(113.,-13.2452561795175,35.3739408143757));
#71540=CARTESIAN_POINT('',(121.7,-12.7669018890611,34.2190913987366));
#71541=CARTESIAN_POINT('',(103.5,-12.7669018890611,34.2190913987366));
#71542=CARTESIAN_POINT('Origin',(121.7,-12.6520968593516,33.9419275389832));
#71543=CARTESIAN_POINT('',(121.912131484566,-13.3660601387852,35.6655873712282));
#71544=CARTESIAN_POINT('Ctrl Pts',(121.912131759621,-13.366060243983,35.6655876251982));
#71545=CARTESIAN_POINT('Ctrl Pts',(121.938311286558,-13.3560359580278,35.6413868580921));
#71546=CARTESIAN_POINT('Ctrl Pts',(121.962987211232,-13.341894920514,35.6072473735403));
#71547=CARTESIAN_POINT('Ctrl Pts',(121.991329280155,-13.3157013328973,35.5440104590688));
#71548=CARTESIAN_POINT('Ctrl Pts',(122.,-13.2990126176798,35.5037203364522));
#71549=CARTESIAN_POINT('Ctrl Pts',(122.,-13.2848331314657,35.4694880285264));
#71550=CARTESIAN_POINT('',(121.75,-13.428141038862,35.8154639221579));
#71551=CARTESIAN_POINT('Ctrl Pts',(104.624264068712,-6.27060329017723,37.6702738824291));
#71552=CARTESIAN_POINT('Ctrl Pts',(104.51617563888,-6.25648252727636,37.56301603955));
#71553=CARTESIAN_POINT('Ctrl Pts',(104.408087612489,-6.24236171176192,37.4557577970312));
#71554=CARTESIAN_POINT('Ctrl Pts',(104.300000000005,-6.22824084227012,37.3484991445136));
#71555=CARTESIAN_POINT('Ctrl Pts',(104.567655925523,-6.27798565144562,37.7263484833951));
#71556=CARTESIAN_POINT('Ctrl Pts',(104.459564357694,-6.26386511752329,37.6190934884253));
#71557=CARTESIAN_POINT('Ctrl Pts',(104.351473262604,-6.24974495464427,37.5118379662647));
#71558=CARTESIAN_POINT('Ctrl Pts',(104.243382456865,-6.23562431783376,37.4045822093923));
#71559=CARTESIAN_POINT('Ctrl Pts',(104.455000447563,-6.35981259677795,37.8291036249763));
#71560=CARTESIAN_POINT('Ctrl Pts',(104.346902897908,-6.34570037330132,37.7218530009686));
#71561=CARTESIAN_POINT('Ctrl Pts',(104.238805543805,-6.33158807371323,37.6146021763207));
#71562=CARTESIAN_POINT('Ctrl Pts',(104.130708651008,-6.31747589142946,37.5073508627117));
#71563=CARTESIAN_POINT('Ctrl Pts',(104.410455468831,-6.52542748682474,37.8521899387271));
#71564=CARTESIAN_POINT('Ctrl Pts',(104.302362090343,-6.51132821563267,37.7449331795208));
#71565=CARTESIAN_POINT('Ctrl Pts',(104.194269413733,-6.49722897978621,37.6376757019839));
#71566=CARTESIAN_POINT('Ctrl Pts',(104.086176765826,-6.48312997219361,37.5304181438624));
#71567=CARTESIAN_POINT('Ctrl Pts',(104.412132034356,-6.60451033490358,37.8400889356902));
#71568=CARTESIAN_POINT('Ctrl Pts',(104.304043604524,-6.59041436013136,37.7328267663559));
#71569=CARTESIAN_POINT('Ctrl Pts',(104.195955578133,-6.5763185424699,37.6255641562333));
#71570=CARTESIAN_POINT('Ctrl Pts',(104.087867965649,-6.56222288596809,37.5183010937809));
#71571=CARTESIAN_POINT('',(104.300000000005,-6.22824084227012,37.3484991445136));
#71572=CARTESIAN_POINT('Origin',(104.300000000005,-6.52567430068227,37.3093412868476));
#71573=CARTESIAN_POINT('',(104.624264068712,-6.27060329017723,37.6702738824291));
#71574=CARTESIAN_POINT('Origin',(104.624264068712,-6.56803674858937,37.6311160247631));
#71575=CARTESIAN_POINT('Ctrl Pts',(104.624264068712,-6.27060329017723,37.6702738824291));
#71576=CARTESIAN_POINT('Ctrl Pts',(104.51617563888,-6.25648252727636,37.56301603955));
#71577=CARTESIAN_POINT('Ctrl Pts',(104.408087612489,-6.24236171176192,37.4557577970312));
#71578=CARTESIAN_POINT('Ctrl Pts',(104.300000000005,-6.22824084227012,37.3484991445136));
#71579=CARTESIAN_POINT('Origin',(104.3,-3.72628900609772,16.0458989224046));
#71580=CARTESIAN_POINT('Origin',(104.3,-6.52567430068159,37.3093412868425));
#71581=CARTESIAN_POINT('',(104.3,-6.05308433581783,36.018053390258));
#71582=CARTESIAN_POINT('',(104.3,-3.42885554768557,16.0850567800707));
#71583=CARTESIAN_POINT('Origin',(104.3,-6.31135993656396,35.6814620741799));
#71584=CARTESIAN_POINT('Origin',(104.3,-6.52567430068159,37.3093412868425));
#71585=CARTESIAN_POINT('Origin',(104.624264068712,-6.56803674858937,37.6311160247631));
#71586=CARTESIAN_POINT('Origin',(104.624264068712,-6.56803674858937,37.6311160247631));
#71587=CARTESIAN_POINT('Origin',(113.,-8.51471537844436,36.8001647010456));
#71588=CARTESIAN_POINT('',(121.7,-8.19119157206621,35.5927574181843));
#71589=CARTESIAN_POINT('',(103.5,-8.19119157206621,35.5927574181843));
#71590=CARTESIAN_POINT('Origin',(121.7,-8.11354585853546,35.3029796702975));
#71591=CARTESIAN_POINT('',(121.912131484566,-8.59641832855391,37.1050842619827));
#71592=CARTESIAN_POINT('Ctrl Pts',(121.912131759621,-8.596418399702,37.105084527511));
#71593=CARTESIAN_POINT('Ctrl Pts',(121.938311286558,-8.58963870688198,37.0797823694469));
#71594=CARTESIAN_POINT('Ctrl Pts',(121.962987211232,-8.58007474482733,37.0440891771373));
#71595=CARTESIAN_POINT('Ctrl Pts',(121.991329280155,-8.56235932063751,36.9779743139833));
#71596=CARTESIAN_POINT('Ctrl Pts',(122.,-8.55107229598143,36.9358505645005));
#71597=CARTESIAN_POINT('Ctrl Pts',(122.,-8.54148233004192,36.9000603243714));
#71598=CARTESIAN_POINT('',(121.75,-8.63840530242857,37.261781781739));
#71599=CARTESIAN_POINT('Origin',(104.3,1.6,18.875));
#71600=CARTESIAN_POINT('',(104.3,1.3,37.8419261182179));
#71601=CARTESIAN_POINT('Origin',(104.3,1.6,37.8419261182179));
#71602=CARTESIAN_POINT('',(104.3,1.3,36.5));
#71603=CARTESIAN_POINT('Origin',(104.3,1.6,36.2));
#71604=CARTESIAN_POINT('',(104.3,1.3,18.875));
#71605=CARTESIAN_POINT('Ctrl Pts',(104.300000000006,1.3,37.8419261182243));
#71606=CARTESIAN_POINT('Ctrl Pts',(104.408087612492,1.3,37.950110301428));
#71607=CARTESIAN_POINT('Ctrl Pts',(104.516175638884,1.3,38.0582940710949));
#71608=CARTESIAN_POINT('Ctrl Pts',(104.624264068718,1.3,38.1664774376736));
#71609=CARTESIAN_POINT('Ctrl Pts',(104.243382456866,1.3,37.8984931216591));
#71610=CARTESIAN_POINT('Ctrl Pts',(104.351473262606,1.30000014726687,38.0066744036192));
#71611=CARTESIAN_POINT('Ctrl Pts',(104.459564357698,1.29999985529285,38.1148553910149));
#71612=CARTESIAN_POINT('Ctrl Pts',(104.567655925529,1.3,38.223035904161));
#71613=CARTESIAN_POINT('Ctrl Pts',(104.130707929307,1.36773633088588,38.0110670701893));
#71614=CARTESIAN_POINT('Ctrl Pts',(104.238804822106,1.36772867591791,38.1192428433615));
#71615=CARTESIAN_POINT('Ctrl Pts',(104.346902176736,1.36772120153623,38.2274181465522));
#71616=CARTESIAN_POINT('Ctrl Pts',(104.454999726393,1.36771367741974,38.3355932413996));
#71617=CARTESIAN_POINT('Ctrl Pts',(104.086176765827,1.5289633238052,38.0555584828822));
#71618=CARTESIAN_POINT('Ctrl Pts',(104.194269413736,1.52894179178494,38.1637387275019));
#71619=CARTESIAN_POINT('Ctrl Pts',(104.302362090347,1.52892049658419,38.2719189220196));
#71620=CARTESIAN_POINT('Ctrl Pts',(104.410455468836,1.52889933018763,38.3800984089656));
#71621=CARTESIAN_POINT('Ctrl Pts',(104.08786796565,1.60896117914607,38.0538687927104));
#71622=CARTESIAN_POINT('Ctrl Pts',(104.195955578136,1.60893560624471,38.1620540571656));
#71623=CARTESIAN_POINT('Ctrl Pts',(104.304043604528,1.60891025216514,38.2702388941964));
#71624=CARTESIAN_POINT('Ctrl Pts',(104.412132034362,1.60888511138664,38.3784233147169));
#71625=CARTESIAN_POINT('',(104.624264068718,1.3,38.1664774376736));
#71626=CARTESIAN_POINT('',(104.412132034362,1.60888511138651,38.378423314714));
#71627=CARTESIAN_POINT('Origin',(104.624264068718,1.6,38.1664774376736));
#71628=CARTESIAN_POINT('',(104.08786796565,1.60896117914594,38.0538687927072));
#71629=CARTESIAN_POINT('Ctrl Pts',(104.412132034362,1.60888511138664,38.3784233147169));
#71630=CARTESIAN_POINT('Ctrl Pts',(104.304043604528,1.60891025216514,38.2702388941964));
#71631=CARTESIAN_POINT('Ctrl Pts',(104.195955578136,1.60893560624471,38.1620540571656));
#71632=CARTESIAN_POINT('Ctrl Pts',(104.08786796565,1.60896117914607,38.0538687927104));
#71633=CARTESIAN_POINT('Origin',(104.300000000006,1.6,37.8419261182243));
#71634=CARTESIAN_POINT('Ctrl Pts',(104.300000000006,1.3,37.8419261182243));
#71635=CARTESIAN_POINT('Ctrl Pts',(104.408087612492,1.3,37.950110301428));
#71636=CARTESIAN_POINT('Ctrl Pts',(104.516175638884,1.3,38.0582940710949));
#71637=CARTESIAN_POINT('Ctrl Pts',(104.624264068718,1.3,38.1664774376736));
#71638=CARTESIAN_POINT('Origin',(104.3,1.6,37.8419261182179));
#71639=CARTESIAN_POINT('Origin',(104.3,1.6,37.8419261182179));
#71640=CARTESIAN_POINT('Origin',(113.,1.6,38.1664774376677));
#71641=CARTESIAN_POINT('',(121.811388243054,1.3,38.1664774376677));
#71642=CARTESIAN_POINT('',(121.5,1.61256544502618,38.4662141714714));
#71643=CARTESIAN_POINT('Ctrl Pts',(121.811388687965,1.30000000000033,38.1664778823209));
#71644=CARTESIAN_POINT('Ctrl Pts',(121.80796264376,1.30000000508128,38.1699059131779));
#71645=CARTESIAN_POINT('Ctrl Pts',(121.80455782351,1.30005878998139,38.1733107052584));
#71646=CARTESIAN_POINT('Ctrl Pts',(121.765406035132,1.30139139994017,38.2124398080324));
#71647=CARTESIAN_POINT('Ctrl Pts',(121.726559498935,1.30939267959732,38.2510389834921));
#71648=CARTESIAN_POINT('Ctrl Pts',(121.652509215907,1.34162007078635,38.3240173010395));
#71649=CARTESIAN_POINT('Ctrl Pts',(121.617288389766,1.36576189057207,38.3584163096784));
#71650=CARTESIAN_POINT('Ctrl Pts',(121.56412779323,1.42099161595499,38.4096034099481));
#71651=CARTESIAN_POINT('Ctrl Pts',(121.541159186122,1.45355748004153,38.4313799964546));
#71652=CARTESIAN_POINT('Ctrl Pts',(121.517077828304,1.50978765959526,38.4532986928691));
#71653=CARTESIAN_POINT('Ctrl Pts',(121.510716614322,1.52974788934972,38.4588770289215));
#71654=CARTESIAN_POINT('Ctrl Pts',(121.502178291748,1.57074933311724,38.4657696567958));
#71655=CARTESIAN_POINT('Ctrl Pts',(121.5,1.59179010598938,38.4670851070329));
#71656=CARTESIAN_POINT('Ctrl Pts',(121.5,1.61256544502618,38.4662141714714));
#71657=CARTESIAN_POINT('',(104.624264068712,1.61256544502618,38.4662141714714));
#71658=CARTESIAN_POINT('',(113.,1.61256544502618,38.4662141714714));
#71659=CARTESIAN_POINT('Origin',(104.624264068712,1.6,38.1664774376677));
#71660=CARTESIAN_POINT('',(113.,1.3,38.1664774376677));
#71661=CARTESIAN_POINT('Origin',(104.624264068712,1.59999999999975,38.1664774376677));
#71662=CARTESIAN_POINT('Origin',(104.624264068712,1.59999999999975,38.1664774376677));
#71663=CARTESIAN_POINT('Origin',(104.3,0.,0.));
#71664=CARTESIAN_POINT('',(104.087867965649,3.37183029953925,37.938324246066));
#71665=CARTESIAN_POINT('Origin',(104.087867965644,-1.66533453693773E-15,
0.));
#71666=CARTESIAN_POINT('Origin',(104.3,3.35305074428542,37.7270251019467));
#71667=CARTESIAN_POINT('Origin',(104.25,0.,0.));
#71668=CARTESIAN_POINT('',(104.412132034356,3.41426858245337,38.2600922303079));
#71669=CARTESIAN_POINT('Origin',(104.412132034356,-1.80411241501588E-15,
0.));
#71670=CARTESIAN_POINT('Ctrl Pts',(104.087867965649,3.37183029953948,37.9383242460686));
#71671=CARTESIAN_POINT('Ctrl Pts',(104.195955578133,3.38597666428457,38.0455806326541));
#71672=CARTESIAN_POINT('Ctrl Pts',(104.304043604524,3.40012275628985,38.1528366240338));
#71673=CARTESIAN_POINT('Ctrl Pts',(104.412132034356,3.41426858245337,38.2600922303079));
#71674=CARTESIAN_POINT('Origin',(104.624264068712,0.,0.));
#71675=CARTESIAN_POINT('',(104.624264068712,3.42207874082298,38.3476124040547));
#71676=CARTESIAN_POINT('Origin',(104.624264068712,0.,0.));
#71677=CARTESIAN_POINT('Origin',(104.624264068712,3.39541319219319,38.0487998398672));
#71678=CARTESIAN_POINT('Origin',(113.,0.,0.));
#71679=CARTESIAN_POINT('',(121.5,3.42207874082298,38.3476124040547));
#71680=CARTESIAN_POINT('Origin',(121.5,0.,0.));
#71681=CARTESIAN_POINT('',(113.,3.42207874082298,38.3476124040547));
#71682=CARTESIAN_POINT('Ctrl Pts',(104.624264068712,3.69284665060533,38.0096419822012));
#71683=CARTESIAN_POINT('Ctrl Pts',(104.51617563888,3.67872588770447,37.9023841393222));
#71684=CARTESIAN_POINT('Ctrl Pts',(104.408087612489,3.66460507219004,37.7951258968034));
#71685=CARTESIAN_POINT('Ctrl Pts',(104.300000000005,3.65048420269824,37.6878672442858));
#71686=CARTESIAN_POINT('Ctrl Pts',(104.567655925523,3.70022901187373,38.0657165831673));
#71687=CARTESIAN_POINT('Ctrl Pts',(104.459564357694,3.68610876488973,37.9584615504213));
#71688=CARTESIAN_POINT('Ctrl Pts',(104.351473262604,3.67198802305843,37.8512061044813));
#71689=CARTESIAN_POINT('Ctrl Pts',(104.243382456865,3.65786767826188,37.7439503091645));
#71690=CARTESIAN_POINT('Ctrl Pts',(104.45500004306,3.64778584282859,38.1861491282933));
#71691=CARTESIAN_POINT('Ctrl Pts',(104.346902493405,3.63365869985869,38.078900468474));
#71692=CARTESIAN_POINT('Ctrl Pts',(104.238805139007,3.61953157877266,37.9716515954047));
#71693=CARTESIAN_POINT('Ctrl Pts',(104.13070824621,3.60540421753158,37.8644022801433));
#71694=CARTESIAN_POINT('Ctrl Pts',(104.410455468831,3.49378871787999,38.2513127544414));
#71695=CARTESIAN_POINT('Ctrl Pts',(104.302362090343,3.47964747605771,38.1440615207735));
#71696=CARTESIAN_POINT('Ctrl Pts',(104.194269413733,3.46550601417654,38.0368096023995));
#71697=CARTESIAN_POINT('Ctrl Pts',(104.086176765826,3.45136431096226,37.9295576652633));
#71698=CARTESIAN_POINT('Ctrl Pts',(104.412132034356,3.41426858245337,38.2600922303079));
#71699=CARTESIAN_POINT('Ctrl Pts',(104.304043604524,3.40012275628985,38.1528366240338));
#71700=CARTESIAN_POINT('Ctrl Pts',(104.195955578133,3.38597666428457,38.0455806326541));
#71701=CARTESIAN_POINT('Ctrl Pts',(104.087867965649,3.37183029953948,37.9383242460686));
#71702=CARTESIAN_POINT('',(104.300000000005,3.65048420269824,37.6878672442858));
#71703=CARTESIAN_POINT('Origin',(104.300000000005,3.3530507442861,37.7270251019518));
#71704=CARTESIAN_POINT('',(104.624264068712,3.69284665060533,38.0096419822012));
#71705=CARTESIAN_POINT('Origin',(104.624264068712,3.39541319219319,38.0487998398672));
#71706=CARTESIAN_POINT('Ctrl Pts',(104.624264068712,3.69284665060533,38.0096419822012));
#71707=CARTESIAN_POINT('Ctrl Pts',(104.51617563888,3.67872588770447,37.9023841393222));
#71708=CARTESIAN_POINT('Ctrl Pts',(104.408087612489,3.66460507219004,37.7951258968034));
#71709=CARTESIAN_POINT('Ctrl Pts',(104.300000000005,3.65048420269824,37.6878672442858));
#71710=CARTESIAN_POINT('Origin',(104.3,1.20107475020923,21.3811445944567));
#71711=CARTESIAN_POINT('Origin',(104.3,3.35305074428542,37.7270251019467));
#71712=CARTESIAN_POINT('',(104.3,3.47532769624593,36.3574214900301));
#71713=CARTESIAN_POINT('',(104.3,1.49850820862137,21.3419867367907));
#71714=CARTESIAN_POINT('Origin',(104.3,3.13873638016778,36.099145889284));
#71715=CARTESIAN_POINT('Origin',(104.3,3.35305074428542,37.7270251019467));
#71716=CARTESIAN_POINT('Origin',(104.624264068712,3.39541319219319,38.0487998398672));
#71717=CARTESIAN_POINT('Origin',(104.624264068712,3.39541319219319,38.0487998398672));
#71718=CARTESIAN_POINT('Origin',(113.,1.3,37.75));
#71719=CARTESIAN_POINT('',(121.7,1.3,36.5));
#71720=CARTESIAN_POINT('',(103.5,1.3,36.5));
#71721=CARTESIAN_POINT('Origin',(121.7,1.3,36.2));
#71722=CARTESIAN_POINT('',(121.912131484566,1.3,38.0656759583793));
#71723=CARTESIAN_POINT('Ctrl Pts',(121.912131759621,1.3,38.0656762332744));
#71724=CARTESIAN_POINT('Ctrl Pts',(121.938311286558,1.3,38.0394815117177));
#71725=CARTESIAN_POINT('Ctrl Pts',(121.962987211232,1.3,38.0025291999168));
#71726=CARTESIAN_POINT('Ctrl Pts',(121.991329280155,1.3,37.9340820569223));
#71727=CARTESIAN_POINT('Ctrl Pts',(122.,1.3,37.8904723424532));
#71728=CARTESIAN_POINT('Ctrl Pts',(122.,1.3,37.8534195593564));
#71729=CARTESIAN_POINT('',(121.75,1.3,38.2279011681123));
#71730=CARTESIAN_POINT('Origin',(113.,-6.56803674858937,37.6311160247631));
#71731=CARTESIAN_POINT('',(121.811388243054,-6.27060329017723,37.6702738824291));
#71732=CARTESIAN_POINT('Ctrl Pts',(121.5,-6.61961818902332,37.9266483495649));
#71733=CARTESIAN_POINT('Ctrl Pts',(121.5,-6.59913426579449,37.9302235600485));
#71734=CARTESIAN_POINT('Ctrl Pts',(121.502178291748,-6.57810179894056,37.9316657356349));
#71735=CARTESIAN_POINT('Ctrl Pts',(121.510716614322,-6.53655145973753,37.930183837478));
#71736=CARTESIAN_POINT('Ctrl Pts',(121.517077828304,-6.51603387355179,37.9272585576496));
#71737=CARTESIAN_POINT('Ctrl Pts',(121.541159186122,-6.4574237869977,37.9128668899463));
#71738=CARTESIAN_POINT('Ctrl Pts',(121.56412779323,-6.42229411347666,37.8955273033918));
#71739=CARTESIAN_POINT('Ctrl Pts',(121.617288389766,-6.36085562876169,37.8519870416124));
#71740=CARTESIAN_POINT('Ctrl Pts',(121.652509215907,-6.33243037397715,37.8210334610709));
#71741=CARTESIAN_POINT('Ctrl Pts',(121.726559498935,-6.29095311068322,37.7528860018039));
#71742=CARTESIAN_POINT('Ctrl Pts',(121.765406035132,-6.27798207968714,37.7156614242077));
#71743=CARTESIAN_POINT('Ctrl Pts',(121.804557793905,-6.27155350246219,37.6770410460388));
#71744=CARTESIAN_POINT('Ctrl Pts',(121.807962616873,-6.27105080457995,37.6736730528646));
#71745=CARTESIAN_POINT('Ctrl Pts',(121.811388687965,-6.27060334821644,37.6702743232782));
#71746=CARTESIAN_POINT('',(113.,-6.27060329017723,37.6702738824291));
#71747=CARTESIAN_POINT('Origin',(113.,-6.21624207609289,37.2573594669753));
#71748=CARTESIAN_POINT('',(121.912131484566,-6.25744605691555,37.5703347737697));
#71749=CARTESIAN_POINT('',(121.75,-6.2786206958241,37.7311721243448));
#71750=CARTESIAN_POINT('Ctrl Pts',(122.,-6.22974103737676,37.3598942576648));
#71751=CARTESIAN_POINT('Ctrl Pts',(122.,-6.23457739606555,37.3966300490657));
#71752=CARTESIAN_POINT('Ctrl Pts',(121.991329280155,-6.240269606039,37.4398666763821));
#71753=CARTESIAN_POINT('Ctrl Pts',(121.962987211232,-6.24920375098241,37.5077282445796));
#71754=CARTESIAN_POINT('Ctrl Pts',(121.938311286558,-6.25402699553551,37.5443644242305));
#71755=CARTESIAN_POINT('Ctrl Pts',(121.912131759621,-6.25744609279656,37.570335046313));
#71756=CARTESIAN_POINT('',(121.7,-6.05308433581783,36.018053390258));
#71757=CARTESIAN_POINT('Origin',(121.7,-6.01392647815181,35.7206199318459));
#71758=CARTESIAN_POINT('',(103.5,-6.05308433581783,36.018053390258));
#71759=CARTESIAN_POINT('Origin',(113.,-11.4236925674066,36.4518757833583));
#71760=CARTESIAN_POINT('',(121.811388243054,-11.1339148195199,36.529521496889));
#71761=CARTESIAN_POINT('Ctrl Pts',(121.5,-11.5134074305014,36.7381470591438));
#71762=CARTESIAN_POINT('Ctrl Pts',(121.5,-11.4935654086862,36.7443653717069));
#71763=CARTESIAN_POINT('Ctrl Pts',(121.502178291748,-11.4729011191897,36.7485404970926));
#71764=CARTESIAN_POINT('Ctrl Pts',(121.510716614322,-11.4315128223748,36.7524946843416));
#71765=CARTESIAN_POINT('Ctrl Pts',(121.517077828304,-11.410788941346,36.7522725130859));
#71766=CARTESIAN_POINT('Ctrl Pts',(121.541159186122,-11.3508017826222,36.7456541195186));
#71767=CARTESIAN_POINT('Ctrl Pts',(121.56412779323,-11.3137093781204,36.7330482180494));
#71768=CARTESIAN_POINT('Ctrl Pts',(121.617288389766,-11.2471133635809,36.6978997807109));
#71769=CARTESIAN_POINT('Ctrl Pts',(121.652509215907,-11.2148910377878,36.6709212526118));
#71770=CARTESIAN_POINT('Ctrl Pts',(121.726559498935,-11.1648735898636,36.6087706735474));
#71771=CARTESIAN_POINT('Ctrl Pts',(121.765406035132,-11.1471547454652,36.5735576166579));
#71772=CARTESIAN_POINT('Ctrl Pts',(121.804557793905,-11.1357401947051,36.5361067388845));
#71773=CARTESIAN_POINT('Ctrl Pts',(121.807962616873,-11.1348021861485,36.5328331745993));
#71774=CARTESIAN_POINT('Ctrl Pts',(121.811388687965,-11.1339149346049,36.5295219263909));
#71775=CARTESIAN_POINT('',(113.,-11.1339148195199,36.529521496889));
#71776=CARTESIAN_POINT('Origin',(113.,-11.0261225267959,36.1272351837791));
#71777=CARTESIAN_POINT('',(121.912131484566,-11.1078254769055,36.4321547447161));
#71778=CARTESIAN_POINT('',(121.75,-11.1498124507801,36.5888522644724));
#71779=CARTESIAN_POINT('Ctrl Pts',(122.,-11.0528894783935,36.2271308071049));
#71780=CARTESIAN_POINT('Ctrl Pts',(122.,-11.062479444333,36.262921047234));
#71781=CARTESIAN_POINT('Ctrl Pts',(121.991329280155,-11.0737664689891,36.3050447967167));
#71782=CARTESIAN_POINT('Ctrl Pts',(121.962987211232,-11.0914818931789,36.3711596598708));
#71783=CARTESIAN_POINT('Ctrl Pts',(121.938311286558,-11.1010458552335,36.4068528521804));
#71784=CARTESIAN_POINT('Ctrl Pts',(121.912131759621,-11.1078255480536,36.4321550102444));
#71785=CARTESIAN_POINT('',(121.7,-10.7025987204178,34.9198279009177));
#71786=CARTESIAN_POINT('Origin',(121.7,-10.624953006887,34.630050153031));
#71787=CARTESIAN_POINT('',(103.5,-10.7025987204178,34.9198279009177));
#71788=CARTESIAN_POINT('Ctrl Pts',(121.375735931288,-17.9574056939141,33.7031390339859));
#71789=CARTESIAN_POINT('Ctrl Pts',(121.483824361121,-17.9033140106251,33.6094494902625));
#71790=CARTESIAN_POINT('Ctrl Pts',(121.591912387512,-17.8492221257921,33.5157595974544));
#71791=CARTESIAN_POINT('Ctrl Pts',(121.699999999997,-17.7951300341907,33.4220693465132));
#71792=CARTESIAN_POINT('Ctrl Pts',(121.432344074477,-17.9856849271578,33.752120102763));
#71793=CARTESIAN_POINT('Ctrl Pts',(121.540435642307,-17.9315947959052,33.6584329578312));
#71794=CARTESIAN_POINT('Ctrl Pts',(121.648526737398,-17.8775040493508,33.5647456205277));
#71795=CARTESIAN_POINT('Ctrl Pts',(121.756617543138,-17.8234135359081,33.4710578085036));
#71796=CARTESIAN_POINT('Ctrl Pts',(121.544996182435,-17.9833149249053,33.8834537221695));
#71797=CARTESIAN_POINT('Ctrl Pts',(121.653093732091,-17.929220861406,33.7897751040339));
#71798=CARTESIAN_POINT('Ctrl Pts',(121.761191083735,-17.8751267330704,33.6960962793851));
#71799=CARTESIAN_POINT('Ctrl Pts',(121.869287976533,-17.8210322170879,33.6024171392287));
#71800=CARTESIAN_POINT('Ctrl Pts',(121.589544531169,-17.8659835447083,34.0025898869996));
#71801=CARTESIAN_POINT('Ctrl Pts',(121.697637909658,-17.8118754705986,33.908914286335));
#71802=CARTESIAN_POINT('Ctrl Pts',(121.805730586268,-17.7577669311554,33.8152381372974));
#71803=CARTESIAN_POINT('Ctrl Pts',(121.913823234176,-17.7036581615694,33.72156206328));
#71804=CARTESIAN_POINT('Ctrl Pts',(121.587867965644,-17.7958762791241,34.041132103426));
#71805=CARTESIAN_POINT('Ctrl Pts',(121.695956395477,-17.7417622963114,33.9474542173515));
#71806=CARTESIAN_POINT('Ctrl Pts',(121.804044421868,-17.6876479205194,33.8537760772191));
#71807=CARTESIAN_POINT('Ctrl Pts',(121.912132034353,-17.63353314151,33.7600976763372));
#71808=CARTESIAN_POINT('',(121.699999999997,-17.7951300341907,33.4220693465132));
#71809=CARTESIAN_POINT('Origin',(121.699999999997,-17.5353224130553,33.5720693465132));
#71810=CARTESIAN_POINT('',(121.375735931288,-17.9574056939141,33.7031390339859));
#71811=CARTESIAN_POINT('Origin',(121.375735931288,-17.6975980727788,33.8531390339859));
#71812=CARTESIAN_POINT('Ctrl Pts',(121.375735931288,-17.9574056939141,33.7031390339859));
#71813=CARTESIAN_POINT('Ctrl Pts',(121.483824361121,-17.9033140106251,33.6094494902625));
#71814=CARTESIAN_POINT('Ctrl Pts',(121.591912387512,-17.8492221257921,33.5157595974544));
#71815=CARTESIAN_POINT('Ctrl Pts',(121.699999999997,-17.7951300341907,33.4220693465132));
#71816=CARTESIAN_POINT('Origin',(121.375735931288,0.,0.));
#71817=CARTESIAN_POINT('',(121.375735931288,-17.8365844450781,34.1190013824203));
#71818=CARTESIAN_POINT('Origin',(121.375735931288,0.,0.));
#71819=CARTESIAN_POINT('Origin',(121.375735931288,-17.6975980727788,33.8531390339859));
#71820=CARTESIAN_POINT('Origin',(121.375735931288,-17.6975980727787,33.8531390339859));
#71821=CARTESIAN_POINT('Origin',(121.375735931288,-17.6975980727787,33.8531390339859));
#71822=CARTESIAN_POINT('Origin',(121.7,-3.9268593539449,10.0015199152097));
#71823=CARTESIAN_POINT('Origin',(121.7,-17.5353224130539,33.5720693465106));
#71824=CARTESIAN_POINT('',(121.7,-17.1241669750802,32.259927238132));
#71825=CARTESIAN_POINT('',(121.7,-4.18666697508023,9.85151991520967));
#71826=CARTESIAN_POINT('Origin',(121.7,-16.7143593539449,32.1501196169967));
#71827=CARTESIAN_POINT('Origin',(121.7,-17.535322413054,33.5720693465106));
#71828=CARTESIAN_POINT('Origin',(113.,-15.6473429640468,34.3789638902265));
#71829=CARTESIAN_POINT('',(104.3,-15.1689886735904,33.2241144745874));
#71830=CARTESIAN_POINT('',(103.5,-15.1689886735904,33.2241144745874));
#71831=CARTESIAN_POINT('Origin',(104.3,-15.0541836438809,32.946950614834));
#71832=CARTESIAN_POINT('',(104.087868515434,-15.7681469233145,34.6706104470789));
#71833=CARTESIAN_POINT('Ctrl Pts',(104.087868240379,-15.7681470285123,34.6706107010489));
#71834=CARTESIAN_POINT('Ctrl Pts',(104.061688713442,-15.7581227425572,34.6464099339429));
#71835=CARTESIAN_POINT('Ctrl Pts',(104.037012788768,-15.7439817050434,34.612270449391));
#71836=CARTESIAN_POINT('Ctrl Pts',(104.008670719845,-15.7177881174267,34.5490335349196));
#71837=CARTESIAN_POINT('Ctrl Pts',(104.,-15.7010994022092,34.5087434123029));
#71838=CARTESIAN_POINT('Ctrl Pts',(104.,-15.686919915995,34.4745111043772));
#71839=CARTESIAN_POINT('',(104.25,-15.8302278233913,34.8204869980086));
#71840=CARTESIAN_POINT('Ctrl Pts',(104.624264068712,-31.0708922200351,22.2029200028051));
#71841=CARTESIAN_POINT('Ctrl Pts',(104.516175638879,-30.9850645847965,22.1370621419721));
#71842=CARTESIAN_POINT('Ctrl Pts',(104.408087612488,-30.8992366297665,22.0712040357546));
#71843=CARTESIAN_POINT('Ctrl Pts',(104.300000000003,-30.8134083466558,22.0053456777918));
#71844=CARTESIAN_POINT('Ctrl Pts',(104.567655925523,-31.1157630683446,22.2373506156865));
#71845=CARTESIAN_POINT('Ctrl Pts',(104.459564357693,-31.0299376087941,22.1714946067171));
#71846=CARTESIAN_POINT('Ctrl Pts',(104.351473262602,-30.9441120388309,22.1056379626004));
#71847=CARTESIAN_POINT('Ctrl Pts',(104.243382456862,-30.858285967781,22.0397814876375));
#71848=CARTESIAN_POINT('Ctrl Pts',(104.455001803843,-31.2462823716862,22.252146783607));
#71849=CARTESIAN_POINT('Ctrl Pts',(104.346904254187,-31.1604658792452,22.186287989002));
#71850=CARTESIAN_POINT('Ctrl Pts',(104.238806901073,-31.0746491908736,22.1204291050614));
#71851=CARTESIAN_POINT('Ctrl Pts',(104.130710008275,-30.9888322399387,22.054569793707));
#71852=CARTESIAN_POINT('Ctrl Pts',(104.410455468831,-31.37971421451,22.1513661623603));
#71853=CARTESIAN_POINT('Ctrl Pts',(104.302362090342,-31.2939025424768,22.0854938708666));
#71854=CARTESIAN_POINT('Ctrl Pts',(104.194269413732,-31.2080903875002,22.0196210464434));
#71855=CARTESIAN_POINT('Ctrl Pts',(104.086176765824,-31.1222783369417,21.9537480036384));
#71856=CARTESIAN_POINT('Ctrl Pts',(104.412132034356,-31.4270775313556,22.0868894429017));
#71857=CARTESIAN_POINT('Ctrl Pts',(104.304043604523,-31.341264364705,22.021010994949));
#71858=CARTESIAN_POINT('Ctrl Pts',(104.195955578132,-31.255450997464,21.9551321242177));
#71859=CARTESIAN_POINT('Ctrl Pts',(104.087867965647,-31.1696374243348,21.889252819684));
#71860=CARTESIAN_POINT('',(104.300000000003,-30.8134083466558,22.0053456777918));
#71861=CARTESIAN_POINT('Origin',(104.300000000003,-30.9960367753584,21.7673396757045));
#71862=CARTESIAN_POINT('',(104.624264068712,-31.0708922200351,22.2029200028051));
#71863=CARTESIAN_POINT('Origin',(104.624264068712,-31.2535206487377,21.9649140007177));
#71864=CARTESIAN_POINT('Ctrl Pts',(104.624264068712,-31.0708922200351,22.2029200028051));
#71865=CARTESIAN_POINT('Ctrl Pts',(104.516175638879,-30.9850645847965,22.1370621419721));
#71866=CARTESIAN_POINT('Ctrl Pts',(104.408087612488,-30.8992366297665,22.0712040357546));
#71867=CARTESIAN_POINT('Ctrl Pts',(104.300000000003,-30.8134083466558,22.0053456777918));
#71868=CARTESIAN_POINT('Origin',(104.3,-3.98978165593707,1.04471127832749));
#71869=CARTESIAN_POINT('Origin',(104.3,-30.9960367753563,21.7673396757028));
#71870=CARTESIAN_POINT('',(104.3,-29.7487867783414,21.1884328164397));
#71871=CARTESIAN_POINT('',(104.3,-3.80715322723445,1.28271728041485));
#71872=CARTESIAN_POINT('Origin',(104.3,-29.6934092049566,20.7677983856497));
#71873=CARTESIAN_POINT('Origin',(104.3,-30.9960367753563,21.7673396757028));
#71874=CARTESIAN_POINT('Origin',(104.624264068712,-31.2535206487377,21.9649140007177));
#71875=CARTESIAN_POINT('Origin',(104.624264068712,-31.2535206487377,21.9649140007177));
#71876=CARTESIAN_POINT('Origin',(113.,-32.0424589928626,20.0008330249198));
#71877=CARTESIAN_POINT('',(121.7,-30.959927238132,19.3758330249198));
#71878=CARTESIAN_POINT('',(103.5,-30.959927238132,19.3758330249198));
#71879=CARTESIAN_POINT('Origin',(121.7,-30.7001196169967,19.2258330249198));
#71880=CARTESIAN_POINT('',(121.912131484566,-32.315842392183,20.1586710041094));
#71881=CARTESIAN_POINT('Ctrl Pts',(121.912131759621,-32.3158426302491,20.158671141557));
#71882=CARTESIAN_POINT('Ctrl Pts',(121.938311286558,-32.293157335936,20.1455737807786));
#71883=CARTESIAN_POINT('Ctrl Pts',(121.962987211232,-32.2611556951879,20.1270976248782));
#71884=CARTESIAN_POINT('Ctrl Pts',(121.991329280155,-32.2018787305382,20.092874053381));
#71885=CARTESIAN_POINT('Ctrl Pts',(122.,-32.1641116099562,20.0710691961464));
#71886=CARTESIAN_POINT('Ctrl Pts',(122.,-32.1320229585134,20.052542804598));
#71887=CARTESIAN_POINT('',(121.75,-32.456333544946,20.2397836089759));
#71888=CARTESIAN_POINT('Origin',(121.7,-6.22801134479456,3.96526964499761));
#71889=CARTESIAN_POINT('',(121.7,-27.6775213868948,25.8390437558097));
#71890=CARTESIAN_POINT('Origin',(121.7,-27.8896534212507,25.6269117214538));
#71891=CARTESIAN_POINT('',(121.7,-26.7286363288515,24.8901586977665));
#71892=CARTESIAN_POINT('Origin',(121.7,-26.7286363288515,24.4658946290545));
#71893=CARTESIAN_POINT('',(121.7,-6.0158793104386,4.17740167935357));
#71894=CARTESIAN_POINT('Ctrl Pts',(121.699999999998,-27.6775213868965,25.8390437558114));
#71895=CARTESIAN_POINT('Ctrl Pts',(121.591912387512,-27.7540191564569,25.9155415253719));
#71896=CARTESIAN_POINT('Ctrl Pts',(121.48382436112,-27.8305166336028,25.9920390025178));
#71897=CARTESIAN_POINT('Ctrl Pts',(121.375735931286,-27.9070138257223,26.0685361946373));
#71898=CARTESIAN_POINT('Ctrl Pts',(121.756617543138,-27.7175202986166,25.8790426675316));
#71899=CARTESIAN_POINT('Ctrl Pts',(121.648526737397,-27.7940161208215,25.9555382814697));
#71900=CARTESIAN_POINT('Ctrl Pts',(121.540435642306,-27.8705114241477,26.0320339977095));
#71901=CARTESIAN_POINT('Ctrl Pts',(121.432344074475,-27.947006700909,26.108529069824));
#71902=CARTESIAN_POINT('Ctrl Pts',(121.869287690755,-27.8450200746977,25.910740307588));
#71903=CARTESIAN_POINT('Ctrl Pts',(121.761190797956,-27.9215064845882,25.987237543238));
#71904=CARTESIAN_POINT('Ctrl Pts',(121.653093446519,-27.9979926900664,26.0637343230645));
#71905=CARTESIAN_POINT('Ctrl Pts',(121.544995896862,-28.0744787128348,26.1402309865404));
#71906=CARTESIAN_POINT('Ctrl Pts',(121.913823234177,-27.9904837995326,25.8282031306363));
#71907=CARTESIAN_POINT('Ctrl Pts',(121.805730586268,-28.0669635586561,25.9047133406349));
#71908=CARTESIAN_POINT('Ctrl Pts',(121.697637909656,-28.1434434498089,25.9812233477493));
#71909=CARTESIAN_POINT('Ctrl Pts',(121.589544531167,-28.2199229317112,26.0577327634567));
#71910=CARTESIAN_POINT('Ctrl Pts',(121.912132034354,-28.045856034146,25.7704413132658));
#71911=CARTESIAN_POINT('Ctrl Pts',(121.804044421868,-28.1223364854948,25.8469579301585));
#71912=CARTESIAN_POINT('Ctrl Pts',(121.695956395476,-28.1988167893393,25.9234740900862));
#71913=CARTESIAN_POINT('Ctrl Pts',(121.587867965642,-28.2752969494932,25.9999898046701));
#71914=CARTESIAN_POINT('',(121.375735931286,-27.9070138257223,26.0685361946373));
#71915=CARTESIAN_POINT('',(121.587867965642,-28.2752969494924,25.9999898046693));
#71916=CARTESIAN_POINT('Origin',(121.375735931286,-28.1191458600783,25.8564041602813));
#71917=CARTESIAN_POINT('',(121.912132034354,-28.0458560341451,25.770441313265));
#71918=CARTESIAN_POINT('Ctrl Pts',(121.587867965642,-28.2752969494932,25.9999898046701));
#71919=CARTESIAN_POINT('Ctrl Pts',(121.695956395476,-28.1988167893393,25.9234740900862));
#71920=CARTESIAN_POINT('Ctrl Pts',(121.804044421868,-28.1223364854948,25.8469579301585));
#71921=CARTESIAN_POINT('Ctrl Pts',(121.912132034354,-28.045856034146,25.7704413132658));
#71922=CARTESIAN_POINT('Origin',(121.699999999998,-27.8896534212524,25.6269117214555));
#71923=CARTESIAN_POINT('Ctrl Pts',(121.699999999998,-27.6775213868965,25.8390437558114));
#71924=CARTESIAN_POINT('Ctrl Pts',(121.591912387512,-27.7540191564569,25.9155415253719));
#71925=CARTESIAN_POINT('Ctrl Pts',(121.48382436112,-27.8305166336028,25.9920390025178));
#71926=CARTESIAN_POINT('Ctrl Pts',(121.375735931286,-27.9070138257223,26.0685361946373));
#71927=CARTESIAN_POINT('Origin',(121.7,-27.8896534212507,25.6269117214538));
#71928=CARTESIAN_POINT('Origin',(121.7,-27.8896534212507,25.6269117214538));
#71929=CARTESIAN_POINT('Origin',(113.,-28.1191458600767,25.8564041602797));
#71930=CARTESIAN_POINT('',(104.188611756946,-27.9070138257207,26.0685361946357));
#71931=CARTESIAN_POINT('',(104.5,-28.3399768485066,26.0594649259364));
#71932=CARTESIAN_POINT('Ctrl Pts',(104.188611312035,-27.9070141401383,26.0685365090528));
#71933=CARTESIAN_POINT('Ctrl Pts',(104.19203735624,-27.9094381275961,26.070960489325));
#71934=CARTESIAN_POINT('Ctrl Pts',(104.19544217649,-27.9118872463662,26.0733264736922));
#71935=CARTESIAN_POINT('Ctrl Pts',(104.234593964868,-27.9404979978181,26.100052630067));
#71936=CARTESIAN_POINT('Ctrl Pts',(104.273440501065,-27.9734494956375,26.1216886096789));
#71937=CARTESIAN_POINT('Ctrl Pts',(104.347490784093,-28.0478411657046,26.1505038660466));
#71938=CARTESIAN_POINT('Ctrl Pts',(104.382711610234,-28.0892357824599,26.1577567938406));
#71939=CARTESIAN_POINT('Ctrl Pts',(104.43587220677,-28.1644838415113,26.1548982262093));
#71940=CARTESIAN_POINT('Ctrl Pts',(104.458840813878,-28.2029097568318,26.1472690548683));
#71941=CARTESIAN_POINT('Ctrl Pts',(104.482922171696,-28.2581693569711,26.123007172468));
#71942=CARTESIAN_POINT('Ctrl Pts',(104.489283385678,-28.2762278500349,26.1128376379049));
#71943=CARTESIAN_POINT('Ctrl Pts',(104.497821708252,-28.3100940728715,26.0887190628886));
#71944=CARTESIAN_POINT('Ctrl Pts',(104.5,-28.3259023098338,26.0747711534923));
#71945=CARTESIAN_POINT('Ctrl Pts',(104.5,-28.3399768485066,26.0594649259364));
#71946=CARTESIAN_POINT('',(121.375735931288,-28.3399768485066,26.0594649259364));
#71947=CARTESIAN_POINT('',(113.,-28.3399768485066,26.0594649259364));
#71948=CARTESIAN_POINT('Origin',(121.375735931288,-28.1191458600767,25.8564041602797));
#71949=CARTESIAN_POINT('',(113.,-27.9070138257207,26.0685361946357));
#71950=CARTESIAN_POINT('Origin',(121.375735931288,-28.1191458600766,25.8564041602798));
#71951=CARTESIAN_POINT('Origin',(121.375735931288,-28.1191458600766,25.8564041602798));
#71952=CARTESIAN_POINT('Origin',(121.7,0.,0.));
#71953=CARTESIAN_POINT('',(121.912132034353,-29.2106904110607,24.4422022714321));
#71954=CARTESIAN_POINT('Origin',(121.912132034356,-2.22044604925031E-15,
-2.22044604925031E-15));
#71955=CARTESIAN_POINT('Origin',(121.7,-29.0480002025285,24.3060703646347));
#71956=CARTESIAN_POINT('Origin',(121.75,0.,0.));
#71957=CARTESIAN_POINT('',(121.587867965644,-29.4682231323184,24.6397181974285));
#71958=CARTESIAN_POINT('Origin',(121.587867965644,0.,0.));
#71959=CARTESIAN_POINT('Ctrl Pts',(121.912132034353,-29.2106904110617,24.4422022714329));
#71960=CARTESIAN_POINT('Ctrl Pts',(121.804044421868,-29.2965351197829,24.5080409992732));
#71961=CARTESIAN_POINT('Ctrl Pts',(121.695956395477,-29.3823793561953,24.573879640517));
#71962=CARTESIAN_POINT('Ctrl Pts',(121.587867965644,-29.4682231323184,24.6397181974285));
#71963=CARTESIAN_POINT('Ctrl Pts',(104.624264068712,-24.2656386875623,29.4881125046124));
#71964=CARTESIAN_POINT('Ctrl Pts',(104.516175638879,-24.1997808267293,29.4022848693738));
#71965=CARTESIAN_POINT('Ctrl Pts',(104.408087612488,-24.1339227205117,29.3164569143438));
#71966=CARTESIAN_POINT('Ctrl Pts',(104.300000000003,-24.068064362549,29.2306286312331));
#71967=CARTESIAN_POINT('Ctrl Pts',(104.567655925523,-24.3000693004437,29.5329833529219));
#71968=CARTESIAN_POINT('Ctrl Pts',(104.459564357693,-24.2342130618665,29.4471580695557));
#71969=CARTESIAN_POINT('Ctrl Pts',(104.351473262602,-24.1683568810269,29.3613321441074));
#71970=CARTESIAN_POINT('Ctrl Pts',(104.243382456862,-24.1025001723946,29.2755062523583));
#71971=CARTESIAN_POINT('Ctrl Pts',(104.455001885058,-24.4223117753432,29.5810561028804));
#71972=CARTESIAN_POINT('Ctrl Pts',(104.346904335402,-24.3564649193042,29.4952304496556));
#71973=CARTESIAN_POINT('Ctrl Pts',(104.238806982348,-24.2906178971386,29.4094046593508));
#71974=CARTESIAN_POINT('Ctrl Pts',(104.130710089549,-24.224770731973,29.3235783883173));
#71975=CARTESIAN_POINT('Ctrl Pts',(104.410455468831,-24.577280943507,29.518244332399));
#71976=CARTESIAN_POINT('Ctrl Pts',(104.302362090342,-24.5114422368762,29.4324068897941));
#71977=CARTESIAN_POINT('Ctrl Pts',(104.194269413731,-24.4456032016902,29.3465688074239));
#71978=CARTESIAN_POINT('Ctrl Pts',(104.086176765824,-24.3797643238856,29.2607305411385));
#71979=CARTESIAN_POINT('Ctrl Pts',(104.412132034356,-24.6397181974285,29.4682231323184));
#71980=CARTESIAN_POINT('Ctrl Pts',(104.304043604523,-24.5738796405169,29.3823793561953));
#71981=CARTESIAN_POINT('Ctrl Pts',(104.195955578132,-24.5080409992732,29.2965351197829));
#71982=CARTESIAN_POINT('Ctrl Pts',(104.087867965647,-24.4422022714329,29.2106904110617));
#71983=CARTESIAN_POINT('',(104.300000000003,-24.068064362549,29.2306286312331));
#71984=CARTESIAN_POINT('Origin',(104.300000000003,-24.3060703646363,29.0480002025304));
#71985=CARTESIAN_POINT('',(104.624264068712,-24.2656386875623,29.4881125046124));
#71986=CARTESIAN_POINT('Origin',(104.624264068712,-24.5036446896497,29.3054840759098));
#71987=CARTESIAN_POINT('Ctrl Pts',(104.624264068712,-24.2656386875623,29.4881125046124));
#71988=CARTESIAN_POINT('Ctrl Pts',(104.516175638879,-24.1997808267293,29.4022848693738));
#71989=CARTESIAN_POINT('Ctrl Pts',(104.408087612488,-24.1339227205117,29.3164569143438));
#71990=CARTESIAN_POINT('Ctrl Pts',(104.300000000003,-24.068064362549,29.2306286312331));
#71991=CARTESIAN_POINT('Origin',(104.3,-5.71851824547952,4.82423066183697));
#71992=CARTESIAN_POINT('Origin',(104.3,-24.3060703646347,29.0480002025284));
#71993=CARTESIAN_POINT('',(104.3,-23.2511515011969,28.1660070629188));
#71994=CARTESIAN_POINT('',(104.3,-5.48051224339216,5.00685909053959));
#71995=CARTESIAN_POINT('Origin',(104.3,-23.3065290745816,27.7453726321288));
#71996=CARTESIAN_POINT('Origin',(104.3,-24.3060703646347,29.0480002025284));
#71997=CARTESIAN_POINT('Origin',(104.624264068712,-24.5036446896497,29.3054840759098));
#71998=CARTESIAN_POINT('Origin',(104.624264068712,-24.5036446896497,29.3054840759098));
#71999=CARTESIAN_POINT('Origin',(113.,-25.7740421742497,27.6125198053347));
#72000=CARTESIAN_POINT('',(121.7,-24.8901586977665,26.7286363288515));
#72001=CARTESIAN_POINT('',(103.5,-24.8901586977665,26.7286363288515));
#72002=CARTESIAN_POINT('Origin',(121.7,-24.6780266634105,26.5165042944955));
#72003=CARTESIAN_POINT('',(121.912131484566,-25.9972587850772,27.8357364161622));
#72004=CARTESIAN_POINT('Ctrl Pts',(121.912131759621,-25.9972589794574,27.8357366105424));
#72005=CARTESIAN_POINT('Ctrl Pts',(121.938311286558,-25.9787365142134,27.8172141452984));
#72006=CARTESIAN_POINT('Ctrl Pts',(121.962987211232,-25.9526072839584,27.7910849150435));
#72007=CARTESIAN_POINT('Ctrl Pts',(121.991329280155,-25.9042078449942,27.7426854760792));
#72008=CARTESIAN_POINT('Ctrl Pts',(122.,-25.8733711201675,27.7118487512525));
#72009=CARTESIAN_POINT('Ctrl Pts',(122.,-25.8471708459779,27.6856484770629));
#72010=CARTESIAN_POINT('',(121.75,-26.1119693309588,27.9504469620439));
#72011=CARTESIAN_POINT('Origin',(104.3,-3.17978755654757,6.77226723466488));
#72012=CARTESIAN_POINT('',(104.3,-22.0053456777902,30.8134083466537));
#72013=CARTESIAN_POINT('Origin',(104.3,-21.7673396757028,30.9960367753563));
#72014=CARTESIAN_POINT('',(104.3,-21.1884328164397,29.7487867783414));
#72015=CARTESIAN_POINT('Origin',(104.3,-20.7677983856497,29.6934092049567));
#72016=CARTESIAN_POINT('',(104.3,-3.41779355863494,6.58963880596226));
#72017=CARTESIAN_POINT('Ctrl Pts',(104.300000000003,-22.0053456777917,30.8134083466557));
#72018=CARTESIAN_POINT('Ctrl Pts',(104.408087612488,-22.0712040357549,30.899236629767));
#72019=CARTESIAN_POINT('Ctrl Pts',(104.51617563888,-22.137062141973,30.9850645847977));
#72020=CARTESIAN_POINT('Ctrl Pts',(104.624264068714,-22.2029200028065,31.070892220037));
#72021=CARTESIAN_POINT('Ctrl Pts',(104.243382456862,-22.0397814876374,30.8582859677809));
#72022=CARTESIAN_POINT('Ctrl Pts',(104.351473262603,-22.1056379626008,30.9441120388314));
#72023=CARTESIAN_POINT('Ctrl Pts',(104.459564357694,-22.171494606718,31.0299376087953));
#72024=CARTESIAN_POINT('Ctrl Pts',(104.567655925525,-22.2373506156879,31.1157630683464));
#72025=CARTESIAN_POINT('Ctrl Pts',(104.130710008275,-22.0545697937069,30.9888322399386));
#72026=CARTESIAN_POINT('Ctrl Pts',(104.238806901074,-22.1204291050618,31.0746491908742));
#72027=CARTESIAN_POINT('Ctrl Pts',(104.346904254189,-22.1862879890029,31.1604658792464));
#72028=CARTESIAN_POINT('Ctrl Pts',(104.455001803846,-22.2521467836084,31.2462823716881));
#72029=CARTESIAN_POINT('Ctrl Pts',(104.086176765824,-21.9537480036383,31.1222783369416));
#72030=CARTESIAN_POINT('Ctrl Pts',(104.194269413732,-22.0196210464437,31.2080903875008));
#72031=CARTESIAN_POINT('Ctrl Pts',(104.302362090344,-22.0854938708675,31.293902542478));
#72032=CARTESIAN_POINT('Ctrl Pts',(104.410455468833,-22.1513661623616,31.3797142145118));
#72033=CARTESIAN_POINT('Ctrl Pts',(104.087867965647,-21.8892528196839,31.1696374243347));
#72034=CARTESIAN_POINT('Ctrl Pts',(104.195955578132,-21.9551321242181,31.2554509974646));
#72035=CARTESIAN_POINT('Ctrl Pts',(104.304043604524,-22.0210109949498,31.3412643647062));
#72036=CARTESIAN_POINT('Ctrl Pts',(104.412132034358,-22.0868894429031,31.4270775313574));
#72037=CARTESIAN_POINT('',(104.624264068714,-22.2029200028065,31.070892220037));
#72038=CARTESIAN_POINT('',(104.412132034358,-22.0868894429024,31.4270775313565));
#72039=CARTESIAN_POINT('Origin',(104.624264068714,-21.9649140007191,31.2535206487396));
#72040=CARTESIAN_POINT('',(104.087867965647,-21.8892528196832,31.1696374243336));
#72041=CARTESIAN_POINT('Ctrl Pts',(104.412132034358,-22.0868894429031,31.4270775313574));
#72042=CARTESIAN_POINT('Ctrl Pts',(104.304043604524,-22.0210109949498,31.3412643647062));
#72043=CARTESIAN_POINT('Ctrl Pts',(104.195955578132,-21.9551321242181,31.2554509974646));
#72044=CARTESIAN_POINT('Ctrl Pts',(104.087867965647,-21.8892528196839,31.1696374243347));
#72045=CARTESIAN_POINT('Origin',(104.300000000003,-21.7673396757043,30.9960367753583));
#72046=CARTESIAN_POINT('Ctrl Pts',(104.300000000003,-22.0053456777917,30.8134083466557));
#72047=CARTESIAN_POINT('Ctrl Pts',(104.408087612488,-22.0712040357549,30.899236629767));
#72048=CARTESIAN_POINT('Ctrl Pts',(104.51617563888,-22.137062141973,30.9850645847977));
#72049=CARTESIAN_POINT('Ctrl Pts',(104.624264068714,-22.2029200028065,31.070892220037));
#72050=CARTESIAN_POINT('Origin',(104.3,-21.7673396757028,30.9960367753563));
#72051=CARTESIAN_POINT('Origin',(104.3,-21.7673396757028,30.9960367753563));
#72052=CARTESIAN_POINT('Origin',(113.,-21.9649140007177,31.2535206487377));
#72053=CARTESIAN_POINT('',(121.811388243054,-22.2029200028051,31.0708922200351));
#72054=CARTESIAN_POINT('',(121.5,-22.1374133253307,31.4989671459791));
#72055=CARTESIAN_POINT('Ctrl Pts',(121.811388687965,-22.2029202734925,31.0708925728024));
#72056=CARTESIAN_POINT('Ctrl Pts',(121.80796264376,-22.2050071224247,31.0736122156265));
#72057=CARTESIAN_POINT('Ctrl Pts',(121.80455782351,-22.2070331913202,31.0763492047763));
#72058=CARTESIAN_POINT('Ctrl Pts',(121.765406035132,-22.2297962492787,31.1082036507075));
#72059=CARTESIAN_POINT('Ctrl Pts',(121.726559498935,-22.2469460965475,31.1436973059289));
#72060=CARTESIAN_POINT('Ctrl Pts',(121.652509215907,-22.2658047729756,31.2212136906375));
#72061=CARTESIAN_POINT('Ctrl Pts',(121.617288389766,-22.2675925692634,31.2632008677555));
#72062=CARTESIAN_POINT('Ctrl Pts',(121.56412779323,-22.2549366144545,31.3374320512821));
#72063=CARTESIAN_POINT('Ctrl Pts',(121.541159186122,-22.2423571233226,31.3745334208854));
#72064=CARTESIAN_POINT('Ctrl Pts',(121.517077828304,-22.2110899794998,31.4261534563592));
#72065=CARTESIAN_POINT('Ctrl Pts',(121.510716614322,-22.1986503403778,31.4427300658883));
#72066=CARTESIAN_POINT('Ctrl Pts',(121.502178291748,-22.1703176740025,31.4731584527351));
#72067=CARTESIAN_POINT('Ctrl Pts',(121.5,-22.1544257019282,31.4870108805359));
#72068=CARTESIAN_POINT('Ctrl Pts',(121.5,-22.1374133253307,31.4989671459791));
#72069=CARTESIAN_POINT('',(104.624264068712,-22.1374133253307,31.4989671459791));
#72070=CARTESIAN_POINT('',(113.,-22.1374133253307,31.4989671459791));
#72071=CARTESIAN_POINT('Origin',(104.624264068712,-21.9649140007177,31.2535206487377));
#72072=CARTESIAN_POINT('',(113.,-22.2029200028051,31.0708922200351));
#72073=CARTESIAN_POINT('Origin',(104.624264068712,-21.9649140007178,31.2535206487377));
#72074=CARTESIAN_POINT('Origin',(104.624264068712,-21.9649140007178,31.2535206487377));
#72075=CARTESIAN_POINT('Origin',(104.3,0.,0.));
#72076=CARTESIAN_POINT('',(104.087867965647,-20.4203356511961,32.1511364971898));
#72077=CARTESIAN_POINT('Origin',(104.087867965644,-2.22044604925031E-15,
-2.22044604925031E-15));
#72078=CARTESIAN_POINT('Origin',(104.3,-20.3066037051641,31.9720693465106));
#72079=CARTESIAN_POINT('Origin',(104.25,0.,0.));
#72080=CARTESIAN_POINT('',(104.412132034356,-20.5825470355869,32.4322469920394));
#72081=CARTESIAN_POINT('Origin',(104.412132034356,0.,0.));
#72082=CARTESIAN_POINT('Ctrl Pts',(104.087867965647,-20.4203356511969,32.151136497191));
#72083=CARTESIAN_POINT('Ctrl Pts',(104.195955578132,-20.4744061366419,32.2448404709743));
#72084=CARTESIAN_POINT('Ctrl Pts',(104.304043604523,-20.5284765978799,32.3385439651864));
#72085=CARTESIAN_POINT('Ctrl Pts',(104.412132034356,-20.5825470355869,32.4322469920394));
#72086=CARTESIAN_POINT('Origin',(104.624264068712,0.,0.));
#72087=CARTESIAN_POINT('',(104.624264068712,-20.6296297263933,32.5064359373941));
#72088=CARTESIAN_POINT('Origin',(104.624264068712,0.,0.));
#72089=CARTESIAN_POINT('Origin',(104.624264068712,-20.468879364889,32.2531390339859));
#72090=CARTESIAN_POINT('Origin',(113.,0.,0.));
#72091=CARTESIAN_POINT('',(121.5,-20.6296297263933,32.5064359373941));
#72092=CARTESIAN_POINT('Origin',(121.5,0.,0.));
#72093=CARTESIAN_POINT('',(113.,-20.6296297263933,32.5064359373941));
#72094=CARTESIAN_POINT('Ctrl Pts',(104.624264068712,-20.2090717437536,32.4031390339859));
#72095=CARTESIAN_POINT('Ctrl Pts',(104.516175638879,-20.1549800604647,32.3094494902624));
#72096=CARTESIAN_POINT('Ctrl Pts',(104.408087612488,-20.1008881756316,32.2157595974544));
#72097=CARTESIAN_POINT('Ctrl Pts',(104.300000000003,-20.0467960840302,32.1220693465131));
#72098=CARTESIAN_POINT('Ctrl Pts',(104.567655925523,-20.2373509769973,32.452120102763));
#72099=CARTESIAN_POINT('Ctrl Pts',(104.459564357693,-20.1832605951046,32.3584331025383));
#72100=CARTESIAN_POINT('Ctrl Pts',(104.351473262602,-20.129170354264,32.2647454732608));
#72101=CARTESIAN_POINT('Ctrl Pts',(104.243382456862,-20.0750795857476,32.1710578085036));
#72102=CARTESIAN_POINT('Ctrl Pts',(104.455001730448,-20.352272791064,32.5157376683244));
#72103=CARTESIAN_POINT('Ctrl Pts',(104.346904180792,-20.2981917597167,32.4220515260722));
#72104=CARTESIAN_POINT('Ctrl Pts',(104.238806827625,-20.2441105815258,32.3283652263742));
#72105=CARTESIAN_POINT('Ctrl Pts',(104.130709934827,-20.1900293243369,32.2346784312498));
#72106=CARTESIAN_POINT('Ctrl Pts',(104.410455468831,-20.5141148642513,32.473690556812));
#72107=CARTESIAN_POINT('Ctrl Pts',(104.302362090342,-20.4600434514159,32.3799937897508));
#72108=CARTESIAN_POINT('Ctrl Pts',(104.194269413732,-20.4059717963422,32.2862963455124));
#72109=CARTESIAN_POINT('Ctrl Pts',(104.086176765824,-20.3519003213093,32.1925987394748));
#72110=CARTESIAN_POINT('Ctrl Pts',(104.412132034356,-20.5825470355869,32.4322469920394));
#72111=CARTESIAN_POINT('Ctrl Pts',(104.304043604523,-20.5284765978799,32.3385439651864));
#72112=CARTESIAN_POINT('Ctrl Pts',(104.195955578132,-20.4744061366419,32.2448404709743));
#72113=CARTESIAN_POINT('Ctrl Pts',(104.087867965647,-20.4203356511969,32.151136497191));
#72114=CARTESIAN_POINT('',(104.300000000003,-20.0467960840302,32.1220693465131));
#72115=CARTESIAN_POINT('Origin',(104.300000000003,-20.3066037051655,31.9720693465131));
#72116=CARTESIAN_POINT('',(104.624264068712,-20.2090717437536,32.4031390339859));
#72117=CARTESIAN_POINT('Origin',(104.624264068712,-20.468879364889,32.2531390339859));
#72118=CARTESIAN_POINT('Ctrl Pts',(104.624264068712,-20.2090717437536,32.4031390339859));
#72119=CARTESIAN_POINT('Ctrl Pts',(104.516175638879,-20.1549800604647,32.3094494902624));
#72120=CARTESIAN_POINT('Ctrl Pts',(104.408087612488,-20.1008881756316,32.2157595974544));
#72121=CARTESIAN_POINT('Ctrl Pts',(104.300000000003,-20.0467960840302,32.1220693465131));
#72122=CARTESIAN_POINT('Origin',(104.3,-6.0731406460551,7.31898816047912));
#72123=CARTESIAN_POINT('Origin',(104.3,-20.3066037051641,31.9720693465106));
#72124=CARTESIAN_POINT('',(104.3,-19.3758330249198,30.959927238132));
#72125=CARTESIAN_POINT('',(104.3,-5.81333302491977,7.46898816047912));
#72126=CARTESIAN_POINT('Origin',(104.3,-19.4856406460551,30.5501196169967));
#72127=CARTESIAN_POINT('Origin',(104.3,-20.3066037051641,31.9720693465106));
#72128=CARTESIAN_POINT('Origin',(104.624264068712,-20.468879364889,32.2531390339859));
#72129=CARTESIAN_POINT('Origin',(104.624264068712,-20.468879364889,32.2531390339859));
#72130=CARTESIAN_POINT('Origin',(113.,-21.9493846027006,30.7404784537055));
#72131=CARTESIAN_POINT('',(121.7,-21.1884328164397,29.7487867783414));
#72132=CARTESIAN_POINT('',(103.5,-21.1884328164397,29.7487867783414));
#72133=CARTESIAN_POINT('Origin',(121.7,-21.0058043877371,29.5107807762541));
#72134=CARTESIAN_POINT('',(121.912131484566,-22.1415559502272,30.9909210297353));
#72135=CARTESIAN_POINT('Ctrl Pts',(121.912131759621,-22.1415561175728,30.9909212478243));
#72136=CARTESIAN_POINT('Ctrl Pts',(121.938311286558,-22.1256097814455,30.9701395779793));
#72137=CARTESIAN_POINT('Ctrl Pts',(121.962987211232,-22.1031146393084,30.9408233379805));
#72138=CARTESIAN_POINT('Ctrl Pts',(121.991329280155,-22.0614466587275,30.8865205684525));
#72139=CARTESIAN_POINT('Ctrl Pts',(122.,-22.0348987466286,30.8519226558093));
#72140=CARTESIAN_POINT('Ctrl Pts',(122.,-22.0123424414419,30.8225267065724));
#72141=CARTESIAN_POINT('',(121.75,-22.2403124007256,31.1196229417564));
#72142=CARTESIAN_POINT('Origin',(113.,-24.5036446896497,29.3054840759098));
#72143=CARTESIAN_POINT('',(121.811388243054,-24.2656386875623,29.4881125046124));
#72144=CARTESIAN_POINT('Ctrl Pts',(121.5,-24.6960816898302,29.5356318566107));
#72145=CARTESIAN_POINT('Ctrl Pts',(121.5,-24.6801296971866,29.5489700413278));
#72146=CARTESIAN_POINT('Ctrl Pts',(121.502178291748,-24.6626361343801,29.5607352354493));
#72147=CARTESIAN_POINT('Ctrl Pts',(121.510716614322,-24.625911536016,29.5802270436011));
#72148=CARTESIAN_POINT('Ctrl Pts',(121.517077828304,-24.6066801452405,29.5879524700494));
#72149=CARTESIAN_POINT('Ctrl Pts',(121.541159186122,-24.5487264875151,29.6047939634926));
#72150=CARTESIAN_POINT('Ctrl Pts',(121.56412779323,-24.509633504542,29.6073422778058));
#72151=CARTESIAN_POINT('Ctrl Pts',(121.617288389766,-24.434656085119,29.6003545473749));
#72152=CARTESIAN_POINT('Ctrl Pts',(121.652509215907,-24.3945623020958,29.5877605876801));
#72153=CARTESIAN_POINT('Ctrl Pts',(121.726559498935,-24.3245682087703,29.5494817883985));
#72154=CARTESIAN_POINT('Ctrl Pts',(121.765406035132,-24.2947226776164,29.5237298740531));
#72155=CARTESIAN_POINT('Ctrl Pts',(121.804557793905,-24.2698451773449,29.4934979340675));
#72156=CARTESIAN_POINT('Ctrl Pts',(121.807962616873,-24.2677258316214,29.49083251536));
#72157=CARTESIAN_POINT('Ctrl Pts',(121.811388687965,-24.2656389582503,29.4881128573793));
#72158=CARTESIAN_POINT('',(113.,-24.2656386875623,29.4881125046124));
#72159=CARTESIAN_POINT('Origin',(113.,-24.0121032874578,29.1576987382828));
#72160=CARTESIAN_POINT('',(121.912131484566,-24.2042746349845,29.4081413143126));
#72161=CARTESIAN_POINT('',(121.75,-24.3030310854828,29.5368432263338));
#72162=CARTESIAN_POINT('Ctrl Pts',(122.,-24.0750611261991,29.2397469911497));
#72163=CARTESIAN_POINT('Ctrl Pts',(122.,-24.0976174313858,29.2691429403866));
#72164=CARTESIAN_POINT('Ctrl Pts',(121.991329280155,-24.1241653434847,29.3037408530298));
#72165=CARTESIAN_POINT('Ctrl Pts',(121.962987211232,-24.1658333240656,29.3580436225579));
#72166=CARTESIAN_POINT('Ctrl Pts',(121.938311286558,-24.1883284662027,29.3873598625566));
#72167=CARTESIAN_POINT('Ctrl Pts',(121.912131759621,-24.20427480233,29.4081415324016));
#72168=CARTESIAN_POINT('',(121.7,-23.2511515011969,28.1660070629188));
#72169=CARTESIAN_POINT('Origin',(121.7,-23.0685230724943,27.9280010608314));
#72170=CARTESIAN_POINT('',(103.5,-23.2511515011969,28.1660070629188));
#72171=CARTESIAN_POINT('Ctrl Pts',(121.375735931288,-29.4881125046124,24.2656386875623));
#72172=CARTESIAN_POINT('Ctrl Pts',(121.483824361121,-29.4022848693738,24.1997808267293));
#72173=CARTESIAN_POINT('Ctrl Pts',(121.591912387512,-29.3164569143438,24.1339227205117));
#72174=CARTESIAN_POINT('Ctrl Pts',(121.699999999997,-29.2306286312331,24.068064362549));
#72175=CARTESIAN_POINT('Ctrl Pts',(121.432344074477,-29.5329833529219,24.3000693004437));
#72176=CARTESIAN_POINT('Ctrl Pts',(121.540435642307,-29.4471580695557,24.2342130618665));
#72177=CARTESIAN_POINT('Ctrl Pts',(121.648526737398,-29.3613321441074,24.1683568810269));
#72178=CARTESIAN_POINT('Ctrl Pts',(121.756617543138,-29.2755062523583,24.1025001723947));
#72179=CARTESIAN_POINT('Ctrl Pts',(121.544995916356,-29.5810525234115,24.4223128317953));
#72180=CARTESIAN_POINT('Ctrl Pts',(121.653093466012,-29.4952268701867,24.3564659757563));
#72181=CARTESIAN_POINT('Ctrl Pts',(121.761190817463,-29.409401077777,24.2906189537558));
#72182=CARTESIAN_POINT('Ctrl Pts',(121.869287710261,-29.3235748067436,24.2247717885902));
#72183=CARTESIAN_POINT('Ctrl Pts',(121.589544531169,-29.518244332399,24.577280943507));
#72184=CARTESIAN_POINT('Ctrl Pts',(121.697637909658,-29.4324068897941,24.5114422368762));
#72185=CARTESIAN_POINT('Ctrl Pts',(121.805730586269,-29.3465688074239,24.4456032016902));
#72186=CARTESIAN_POINT('Ctrl Pts',(121.913823234176,-29.2607305411385,24.3797643238857));
#72187=CARTESIAN_POINT('Ctrl Pts',(121.587867965644,-29.4682231323184,24.6397181974285));
#72188=CARTESIAN_POINT('Ctrl Pts',(121.695956395477,-29.3823793561953,24.573879640517));
#72189=CARTESIAN_POINT('Ctrl Pts',(121.804044421868,-29.2965351197829,24.5080409992732));
#72190=CARTESIAN_POINT('Ctrl Pts',(121.912132034353,-29.2106904110617,24.4422022714329));
#72191=CARTESIAN_POINT('',(121.699999999997,-29.2306286312331,24.068064362549));
#72192=CARTESIAN_POINT('Origin',(121.699999999997,-29.0480002025305,24.3060703646364));
#72193=CARTESIAN_POINT('',(121.375735931288,-29.4881125046124,24.2656386875623));
#72194=CARTESIAN_POINT('Origin',(121.375735931288,-29.3054840759098,24.5036446896497));
#72195=CARTESIAN_POINT('Ctrl Pts',(121.375735931288,-29.4881125046124,24.2656386875623));
#72196=CARTESIAN_POINT('Ctrl Pts',(121.483824361121,-29.4022848693738,24.1997808267293));
#72197=CARTESIAN_POINT('Ctrl Pts',(121.591912387512,-29.3164569143438,24.1339227205117));
#72198=CARTESIAN_POINT('Ctrl Pts',(121.699999999997,-29.2306286312331,24.068064362549));
#72199=CARTESIAN_POINT('Origin',(121.375735931288,0.,0.));
#72200=CARTESIAN_POINT('',(121.375735931288,-29.5356318566107,24.6960816898302));
#72201=CARTESIAN_POINT('Origin',(121.375735931288,0.,0.));
#72202=CARTESIAN_POINT('Origin',(121.375735931288,-29.3054840759098,24.5036446896497));
#72203=CARTESIAN_POINT('Origin',(121.375735931288,-29.3054840759098,24.5036446896497));
#72204=CARTESIAN_POINT('Origin',(121.375735931288,-29.3054840759098,24.5036446896497));
#72205=CARTESIAN_POINT('Origin',(121.7,-3.61526888948732,4.79084925012077));
#72206=CARTESIAN_POINT('Origin',(121.7,-29.0480002025284,24.3060703646348));
#72207=CARTESIAN_POINT('',(121.7,-28.1660070629187,23.2511515011969));
#72208=CARTESIAN_POINT('',(121.7,-3.79789731818994,4.55284324803339));
#72209=CARTESIAN_POINT('Origin',(121.7,-27.7453726321287,23.3065290745817));
#72210=CARTESIAN_POINT('Origin',(121.7,-29.0480002025285,24.3060703646347));
#72211=CARTESIAN_POINT('Origin',(113.,-27.6125198053347,25.7740421742497));
#72212=CARTESIAN_POINT('',(104.3,-26.7286363288515,24.8901586977665));
#72213=CARTESIAN_POINT('',(103.5,-26.7286363288515,24.8901586977665));
#72214=CARTESIAN_POINT('Origin',(104.3,-26.5165042944955,24.6780266634105));
#72215=CARTESIAN_POINT('',(104.087868515434,-27.8357364161622,25.9972587850772));
#72216=CARTESIAN_POINT('Ctrl Pts',(104.087868240379,-27.8357366105424,25.9972589794574));
#72217=CARTESIAN_POINT('Ctrl Pts',(104.061688713442,-27.8172141452984,25.9787365142134));
#72218=CARTESIAN_POINT('Ctrl Pts',(104.037012788768,-27.7910849150434,25.9526072839584));
#72219=CARTESIAN_POINT('Ctrl Pts',(104.008670719845,-27.7426854760792,25.9042078449942));
#72220=CARTESIAN_POINT('Ctrl Pts',(104.,-27.7118487512525,25.8733711201675));
#72221=CARTESIAN_POINT('Ctrl Pts',(104.,-27.6856484770629,25.8471708459779));
#72222=CARTESIAN_POINT('',(104.25,-27.9504469620438,26.1119693309588));
#72223=CARTESIAN_POINT('Origin',(113.,-31.2535206487377,21.9649140007177));
#72224=CARTESIAN_POINT('',(121.811388243054,-31.0708922200351,22.2029200028051));
#72225=CARTESIAN_POINT('Ctrl Pts',(121.5,-31.4989671459791,22.1374133253307));
#72226=CARTESIAN_POINT('Ctrl Pts',(121.5,-31.4870108805358,22.1544257019283));
#72227=CARTESIAN_POINT('Ctrl Pts',(121.502178291748,-31.4731584527351,22.1703176740025));
#72228=CARTESIAN_POINT('Ctrl Pts',(121.510716614322,-31.4427300658883,22.1986503403779));
#72229=CARTESIAN_POINT('Ctrl Pts',(121.517077828304,-31.4261534563592,22.2110899794998));
#72230=CARTESIAN_POINT('Ctrl Pts',(121.541159186122,-31.3745334208853,22.2423571233226));
#72231=CARTESIAN_POINT('Ctrl Pts',(121.56412779323,-31.3374320512821,22.2549366144545));
#72232=CARTESIAN_POINT('Ctrl Pts',(121.617288389766,-31.2632008677554,22.2675925692634));
#72233=CARTESIAN_POINT('Ctrl Pts',(121.652509215907,-31.2212136906374,22.2658047729756));
#72234=CARTESIAN_POINT('Ctrl Pts',(121.726559498935,-31.1436973059289,22.2469460965475));
#72235=CARTESIAN_POINT('Ctrl Pts',(121.765406035132,-31.1082036507075,22.2297962492787));
#72236=CARTESIAN_POINT('Ctrl Pts',(121.804557793905,-31.0763492288632,22.2070332085326));
#72237=CARTESIAN_POINT('Ctrl Pts',(121.807962616873,-31.0736122369693,22.2050071388016));
#72238=CARTESIAN_POINT('Ctrl Pts',(121.811388687965,-31.0708925728024,22.2029202734926));
#72239=CARTESIAN_POINT('',(113.,-31.0708922200351,22.2029200028051));
#72240=CARTESIAN_POINT('Origin',(113.,-30.7404784537055,21.9493846027006));
#72241=CARTESIAN_POINT('',(121.912131484566,-30.9909210297353,22.1415559502273));
#72242=CARTESIAN_POINT('',(121.75,-31.1196229417564,22.2403124007256));
#72243=CARTESIAN_POINT('Ctrl Pts',(122.,-30.8225267065723,22.0123424414419));
#72244=CARTESIAN_POINT('Ctrl Pts',(122.,-30.8519226558093,22.0348987466286));
#72245=CARTESIAN_POINT('Ctrl Pts',(121.991329280155,-30.8865205684525,22.0614466587275));
#72246=CARTESIAN_POINT('Ctrl Pts',(121.962987211232,-30.9408233379805,22.1031146393084));
#72247=CARTESIAN_POINT('Ctrl Pts',(121.938311286558,-30.9701395779793,22.1256097814455));
#72248=CARTESIAN_POINT('Ctrl Pts',(121.912131759621,-30.9909212478242,22.1415561175728));
#72249=CARTESIAN_POINT('',(121.7,-29.7487867783414,21.1884328164397));
#72250=CARTESIAN_POINT('Origin',(121.7,-29.510780776254,21.0058043877371));
#72251=CARTESIAN_POINT('',(103.5,-29.7487867783414,21.1884328164397));
#72252=CARTESIAN_POINT('Origin',(104.3,-0.918719107418027,1.41027184575243));
#72253=CARTESIAN_POINT('',(104.3,-36.8889585127428,-8.5385076085815));
#72254=CARTESIAN_POINT('Origin',(104.3,-36.9666042262736,-8.24872986069479));
#72255=CARTESIAN_POINT('',(104.3,-35.5927574181843,-8.1911915720662));
#72256=CARTESIAN_POINT('Origin',(104.3,-35.3806253838283,-7.82376811064873));
#72257=CARTESIAN_POINT('',(104.3,-0.841073393887271,1.12049409786571));
#72258=CARTESIAN_POINT('Ctrl Pts',(104.300000000004,-36.8889585127466,-8.53850760858253));
#72259=CARTESIAN_POINT('Ctrl Pts',(104.40808761249,-36.9934564092991,-8.5665077355745));
#72260=CARTESIAN_POINT('Ctrl Pts',(104.516175638882,-37.0979539064058,-8.59450775553531));
#72261=CARTESIAN_POINT('Ctrl Pts',(104.624264068716,-37.2024510141591,-8.62250767116922));
#72262=CARTESIAN_POINT('Ctrl Pts',(104.243382456863,-36.94359804228,-8.55314822639582));
#72263=CARTESIAN_POINT('Ctrl Pts',(104.351473262604,-37.0480931745619,-8.58114746024185));
#72264=CARTESIAN_POINT('Ctrl Pts',(104.459564357696,-37.1525879086325,-8.60914704212312));
#72265=CARTESIAN_POINT('Ctrl Pts',(104.567655925526,-37.2570822976345,-8.63714607945793));
#72266=CARTESIAN_POINT('Ctrl Pts',(104.130708900332,-37.0698669867125,-8.51685469895554));
#72267=CARTESIAN_POINT('Ctrl Pts',(104.238805793131,-37.1743547785469,-8.54486004340248));
#72268=CARTESIAN_POINT('Ctrl Pts',(104.346903147053,-37.2788421636609,-8.57286509255766));
#72269=CARTESIAN_POINT('Ctrl Pts',(104.45500069671,-37.3833293341507,-8.60087013504839));
#72270=CARTESIAN_POINT('Ctrl Pts',(104.086176765825,-37.1545715999316,-8.37263814546983));
#72271=CARTESIAN_POINT('Ctrl Pts',(104.194269413734,-37.2590601192072,-8.40065805141574));
#72272=CARTESIAN_POINT('Ctrl Pts',(104.302362090345,-37.3635486513814,-8.42867771564422));
#72273=CARTESIAN_POINT('Ctrl Pts',(104.410455468834,-37.4680365334307,-8.45669707232437));
#72274=CARTESIAN_POINT('Ctrl Pts',(104.087867965648,-37.1736444530858,-8.29492882695157));
#72275=CARTESIAN_POINT('Ctrl Pts',(104.195955578134,-37.2781367752932,-8.32295393531793));
#72276=CARTESIAN_POINT('Ctrl Pts',(104.304043604526,-37.3826287412755,-8.35097872169309));
#72277=CARTESIAN_POINT('Ctrl Pts',(104.41213203436,-37.4871203601462,-8.37900319423444));
#72278=CARTESIAN_POINT('',(104.624264068716,-37.2024510141591,-8.62250767116922));
#72279=CARTESIAN_POINT('',(104.41213203436,-37.4871203601444,-8.37900319423404));
#72280=CARTESIAN_POINT('Origin',(104.624264068716,-37.2800967276899,-8.33272992328249));
#72281=CARTESIAN_POINT('',(104.087867965648,-37.1736444530839,-8.29492882695114));
#72282=CARTESIAN_POINT('Ctrl Pts',(104.41213203436,-37.4871203601462,-8.37900319423444));
#72283=CARTESIAN_POINT('Ctrl Pts',(104.304043604526,-37.3826287412755,-8.35097872169309));
#72284=CARTESIAN_POINT('Ctrl Pts',(104.195955578134,-37.2781367752932,-8.32295393531793));
#72285=CARTESIAN_POINT('Ctrl Pts',(104.087867965648,-37.1736444530858,-8.29492882695157));
#72286=CARTESIAN_POINT('Origin',(104.300000000004,-36.9666042262774,-8.24872986069581));
#72287=CARTESIAN_POINT('Ctrl Pts',(104.300000000004,-36.8889585127466,-8.53850760858253));
#72288=CARTESIAN_POINT('Ctrl Pts',(104.40808761249,-36.9934564092991,-8.5665077355745));
#72289=CARTESIAN_POINT('Ctrl Pts',(104.516175638882,-37.0979539064058,-8.59450775553531));
#72290=CARTESIAN_POINT('Ctrl Pts',(104.624264068716,-37.2024510141591,-8.62250767116922));
#72291=CARTESIAN_POINT('Origin',(104.3,-36.9666042262736,-8.24872986069479));
#72292=CARTESIAN_POINT('Origin',(104.3,-36.9666042262736,-8.24872986069479));
#72293=CARTESIAN_POINT('Origin',(113.,-37.2800967276863,-8.33272992328154));
#72294=CARTESIAN_POINT('',(121.811388243054,-37.2024510141556,-8.62250767116826));
#72295=CARTESIAN_POINT('',(121.5,-37.5728723564378,-8.39817021063716));
#72296=CARTESIAN_POINT('Ctrl Pts',(121.811388687965,-37.2024514436577,-8.62250778625266));
#72297=CARTESIAN_POINT('Ctrl Pts',(121.80796264376,-37.2057626685107,-8.62339502101782));
#72298=CARTESIAN_POINT('Ctrl Pts',(121.80455782351,-37.2090666597662,-8.62421946419965));
#72299=CARTESIAN_POINT('Ctrl Pts',(121.765406035132,-37.2472073755322,-8.63305961883979));
#72300=CARTESIAN_POINT('Ctrl Pts',(121.726559498935,-37.2865621995426,-8.63532117790981));
#72301=CARTESIAN_POINT('Ctrl Pts',(121.652509215907,-37.3653949038344,-8.62308008690721));
#72302=CARTESIAN_POINT('Ctrl Pts',(121.617288389766,-37.4048701574215,-8.60866399825097));
#72303=CARTESIAN_POINT('Ctrl Pts',(121.56412779323,-37.4686076043297,-8.56856437653813));
#72304=CARTESIAN_POINT('Ctrl Pts',(121.541159186122,-37.4980708374905,-8.5427443626867));
#72305=CARTESIAN_POINT('Ctrl Pts',(121.517077828304,-37.533796113814,-8.49410315611479));
#72306=CARTESIAN_POINT('Ctrl Pts',(121.510716614322,-37.5443504602798,-8.47626683430663));
#72307=CARTESIAN_POINT('Ctrl Pts',(121.502178291748,-37.5616201820783,-8.43844642422113));
#72308=CARTESIAN_POINT('Ctrl Pts',(121.5,-37.5683365621785,-8.4184630618731));
#72309=CARTESIAN_POINT('Ctrl Pts',(121.5,-37.5728723564378,-8.39817021063716));
#72310=CARTESIAN_POINT('',(104.624264068712,-37.5728723564378,-8.39817021063716));
#72311=CARTESIAN_POINT('',(113.,-37.5728723564378,-8.39817021063716));
#72312=CARTESIAN_POINT('Origin',(104.624264068712,-37.2800967276863,-8.33272992328154));
#72313=CARTESIAN_POINT('',(113.,-37.2024510141556,-8.62250767116826));
#72314=CARTESIAN_POINT('Origin',(104.624264068712,-37.2800967276863,-8.33272992328169));
#72315=CARTESIAN_POINT('Origin',(104.624264068712,-37.2800967276863,-8.33272992328169));
#72316=CARTESIAN_POINT('Origin',(104.3,0.,0.));
#72317=CARTESIAN_POINT('',(104.087867965649,-37.5183010937784,-6.56222288596765));
#72318=CARTESIAN_POINT('Origin',(104.087867965644,0.,2.22044604925031E-15));
#72319=CARTESIAN_POINT('Origin',(104.3,-37.3093412868425,-6.52567430068159));
#72320=CARTESIAN_POINT('Origin',(104.25,0.,0.));
#72321=CARTESIAN_POINT('',(104.412132034356,-37.8400889356902,-6.60451033490358));
#72322=CARTESIAN_POINT('Origin',(104.412132034356,-2.22044604925031E-15,
3.33066907387547E-15));
#72323=CARTESIAN_POINT('Ctrl Pts',(104.087867965649,-37.5183010937809,-6.56222288596809));
#72324=CARTESIAN_POINT('Ctrl Pts',(104.195955578133,-37.6255641562333,-6.5763185424699));
#72325=CARTESIAN_POINT('Ctrl Pts',(104.304043604524,-37.7328267663559,-6.59041436013136));
#72326=CARTESIAN_POINT('Ctrl Pts',(104.412132034356,-37.8400889356902,-6.60451033490358));
#72327=CARTESIAN_POINT('Origin',(104.624264068712,0.,0.));
#72328=CARTESIAN_POINT('',(104.624264068712,-37.9266483495649,-6.61961818902332));
#72329=CARTESIAN_POINT('Origin',(104.624264068712,0.,0.));
#72330=CARTESIAN_POINT('Origin',(104.624264068712,-37.6311160247631,-6.56803674858937));
#72331=CARTESIAN_POINT('Origin',(113.,0.,0.));
#72332=CARTESIAN_POINT('',(121.5,-37.9266483495649,-6.61961818902332));
#72333=CARTESIAN_POINT('Origin',(121.5,0.,0.));
#72334=CARTESIAN_POINT('',(113.,-37.9266483495649,-6.61961818902332));
#72335=CARTESIAN_POINT('Origin',(104.3,-1.83300524666248,0.972571887399195));
#72336=CARTESIAN_POINT('',(104.3,-35.4588694735005,-13.2804347819611));
#72337=CARTESIAN_POINT('Origin',(104.3,-35.57367450321,-13.0032709222077));
#72338=CARTESIAN_POINT('',(104.3,-34.2190913987366,-12.7669018890611));
#72339=CARTESIAN_POINT('Origin',(104.3,-34.0567325686927,-12.3749329995982));
#72340=CARTESIAN_POINT('',(104.3,-1.71820021695295,0.695408027645809));
#72341=CARTESIAN_POINT('Ctrl Pts',(104.300000000003,-35.4588694735034,-13.2804347819623));
#72342=CARTESIAN_POINT('Ctrl Pts',(104.408087612489,-35.5588186261068,-13.3218350765183));
#72343=CARTESIAN_POINT('Ctrl Pts',(104.516175638881,-35.6587673966521,-13.3632352128207));
#72344=CARTESIAN_POINT('Ctrl Pts',(104.624264068715,-35.7587157947924,-13.4046351948679));
#72345=CARTESIAN_POINT('Ctrl Pts',(104.243382456863,-35.5111305701923,-13.3020820369953));
#72346=CARTESIAN_POINT('Ctrl Pts',(104.351473262603,-35.6110770987527,-13.3434810852367));
#72347=CARTESIAN_POINT('Ctrl Pts',(104.459564357695,-35.7110231870809,-13.3848804265588));
#72348=CARTESIAN_POINT('Ctrl Pts',(104.567655925526,-35.8109690043703,-13.4262791829526));
#72349=CARTESIAN_POINT('Ctrl Pts',(104.130709407257,-35.6410563204708,-13.2825795738598));
#72350=CARTESIAN_POINT('Ctrl Pts',(104.238806300056,-35.7409947737889,-13.3239837223043));
#72351=CARTESIAN_POINT('Ctrl Pts',(104.346903653609,-35.840932862619,-13.3653875253347));
#72352=CARTESIAN_POINT('Ctrl Pts',(104.455001203266,-35.9408707393213,-13.4067912933046));
#72353=CARTESIAN_POINT('Ctrl Pts',(104.086176765824,-35.7438605133323,-13.1506538199745));
#72354=CARTESIAN_POINT('Ctrl Pts',(104.194269413733,-35.8437977872112,-13.1920725002925));
#72355=CARTESIAN_POINT('Ctrl Pts',(104.302362090344,-35.9437351054287,-13.2334909426446));
#72356=CARTESIAN_POINT('Ctrl Pts',(104.410455468834,-36.0436718192265,-13.2749089952212));
#72357=CARTESIAN_POINT('Ctrl Pts',(104.087867965647,-35.77291329703,-13.0760988223457));
#72358=CARTESIAN_POINT('Ctrl Pts',(104.195955578133,-35.8728536622539,-13.1175231569589));
#72359=CARTESIAN_POINT('Ctrl Pts',(104.304043604525,-35.9727937163286,-13.1589471258389));
#72360=CARTESIAN_POINT('Ctrl Pts',(104.412132034359,-36.0727334672248,-13.2003707382629));
#72361=CARTESIAN_POINT('',(104.624264068715,-35.7587157947924,-13.4046351948679));
#72362=CARTESIAN_POINT('',(104.412132034359,-36.0727334672234,-13.2003707382624));
#72363=CARTESIAN_POINT('Origin',(104.624264068715,-35.873520824502,-13.1274713351145));
#72364=CARTESIAN_POINT('',(104.087867965647,-35.7729132970285,-13.0760988223451));
#72365=CARTESIAN_POINT('Ctrl Pts',(104.412132034359,-36.0727334672248,-13.2003707382629));
#72366=CARTESIAN_POINT('Ctrl Pts',(104.304043604525,-35.9727937163286,-13.1589471258389));
#72367=CARTESIAN_POINT('Ctrl Pts',(104.195955578133,-35.8728536622539,-13.1175231569589));
#72368=CARTESIAN_POINT('Ctrl Pts',(104.087867965647,-35.77291329703,-13.0760988223457));
#72369=CARTESIAN_POINT('Origin',(104.300000000003,-35.573674503213,-13.0032709222089));
#72370=CARTESIAN_POINT('Ctrl Pts',(104.300000000003,-35.4588694735034,-13.2804347819623));
#72371=CARTESIAN_POINT('Ctrl Pts',(104.408087612489,-35.5588186261068,-13.3218350765183));
#72372=CARTESIAN_POINT('Ctrl Pts',(104.516175638881,-35.6587673966521,-13.3632352128207));
#72373=CARTESIAN_POINT('Ctrl Pts',(104.624264068715,-35.7587157947924,-13.4046351948679));
#72374=CARTESIAN_POINT('Origin',(104.3,-35.57367450321,-13.0032709222077));
#72375=CARTESIAN_POINT('Origin',(104.3,-35.57367450321,-13.0032709222077));
#72376=CARTESIAN_POINT('Origin',(113.,-35.8735208244992,-13.1274713351134));
#72377=CARTESIAN_POINT('',(121.811388243054,-35.7587157947897,-13.4046351948667));
#72378=CARTESIAN_POINT('',(121.5,-36.155250045634,-13.2305666597347));
#72379=CARTESIAN_POINT('Ctrl Pts',(121.811388687965,-35.7587162055958,-13.4046353650279));
#72380=CARTESIAN_POINT('Ctrl Pts',(121.80796264376,-35.7618832950857,-13.4059472109483));
#72381=CARTESIAN_POINT('Ctrl Pts',(121.80455782351,-35.7650514088087,-13.4071958583021));
#72382=CARTESIAN_POINT('Ctrl Pts',(121.765406035132,-35.8017119537402,-13.4209387465913));
#72383=CARTESIAN_POINT('Ctrl Pts',(121.726559498935,-35.8404348990817,-13.4283177930335));
#72384=CARTESIAN_POINT('Ctrl Pts',(121.652509215907,-35.9201909616573,-13.426471158975));
#72385=CARTESIAN_POINT('Ctrl Pts',(121.617288389766,-35.9612101761366,-13.4173309564933));
#72386=CARTESIAN_POINT('Ctrl Pts',(121.56412779323,-36.0296363912825,-13.3858937988498));
#72387=CARTESIAN_POINT('Ctrl Pts',(121.541159186122,-36.0622177504903,-13.3641404024312));
#72388=CARTESIAN_POINT('Ctrl Pts',(121.517077828304,-36.1039863436012,-13.320578412409));
#72389=CARTESIAN_POINT('Ctrl Pts',(121.510716614322,-36.1167785033387,-13.304272301462));
#72390=CARTESIAN_POINT('Ctrl Pts',(121.502178291748,-36.1388370343898,-13.2690296012548));
#72391=CARTESIAN_POINT('Ctrl Pts',(121.5,-36.1481043071223,-13.2500938628618));
#72392=CARTESIAN_POINT('Ctrl Pts',(121.5,-36.155250045634,-13.2305666597347));
#72393=CARTESIAN_POINT('',(104.624264068712,-36.155250045634,-13.2305666597347));
#72394=CARTESIAN_POINT('',(113.,-36.155250045634,-13.2305666597347));
#72395=CARTESIAN_POINT('Origin',(104.624264068712,-35.8735208244992,-13.1274713351134));
#72396=CARTESIAN_POINT('',(113.,-35.7587157947897,-13.4046351948667));
#72397=CARTESIAN_POINT('Origin',(104.624264068712,-35.8735208244991,-13.1274713351135));
#72398=CARTESIAN_POINT('Origin',(104.624264068712,-35.8735208244991,-13.1274713351135));
#72399=CARTESIAN_POINT('Origin',(104.3,0.,0.));
#72400=CARTESIAN_POINT('',(104.087867965648,-36.3407848610969,-11.4032031398184));
#72401=CARTESIAN_POINT('Origin',(104.087867965644,-2.22044604925031E-15,
2.22044604925031E-15));
#72402=CARTESIAN_POINT('Origin',(104.3,-36.1383832819455,-11.3396925048198));
#72403=CARTESIAN_POINT('Origin',(104.25,0.,0.));
#72404=CARTESIAN_POINT('',(104.412132034356,-36.6543001437251,-11.4871305554741));
#72405=CARTESIAN_POINT('Origin',(104.412132034356,-2.22044604925031E-15,
2.22044604925031E-15));
#72406=CARTESIAN_POINT('Ctrl Pts',(104.087867965648,-36.3407848610989,-11.403203139819));
#72407=CARTESIAN_POINT('Ctrl Pts',(104.195955578133,-36.4452904208128,-11.4311788451333));
#72408=CARTESIAN_POINT('Ctrl Pts',(104.304043604523,-36.5497955110311,-11.4591546511876));
#72409=CARTESIAN_POINT('Ctrl Pts',(104.412132034356,-36.6543001437251,-11.4871305554741));
#72410=CARTESIAN_POINT('Origin',(104.624264068712,0.,0.));
#72411=CARTESIAN_POINT('',(104.624264068712,-36.7381470591438,-11.5134074305014));
#72412=CARTESIAN_POINT('Origin',(104.624264068712,0.,0.));
#72413=CARTESIAN_POINT('Origin',(104.624264068712,-36.4518757833583,-11.4236925674066));
#72414=CARTESIAN_POINT('Origin',(113.,0.,0.));
#72415=CARTESIAN_POINT('',(121.5,-36.7381470591438,-11.5134074305014));
#72416=CARTESIAN_POINT('Origin',(121.5,0.,0.));
#72417=CARTESIAN_POINT('',(113.,-36.7381470591438,-11.5134074305014));
#72418=CARTESIAN_POINT('Origin',(121.7,-3.96688872314567,-0.0886884109160058));
#72419=CARTESIAN_POINT('',(121.7,-35.4588694735005,13.2804347819611));
#72420=CARTESIAN_POINT('Origin',(121.7,-35.57367450321,13.0032709222077));
#72421=CARTESIAN_POINT('',(121.7,-34.2190913987366,12.7669018890611));
#72422=CARTESIAN_POINT('Origin',(121.7,-34.0567325686927,12.3749329995982));
#72423=CARTESIAN_POINT('',(121.7,-3.85208369343614,0.188475448837378));
#72424=CARTESIAN_POINT('Ctrl Pts',(121.699999999997,-35.4588694735035,13.2804347819624));
#72425=CARTESIAN_POINT('Ctrl Pts',(121.591912387511,-35.5588186261068,13.3218350765184));
#72426=CARTESIAN_POINT('Ctrl Pts',(121.483824361119,-35.6587673966521,13.3632352128207));
#72427=CARTESIAN_POINT('Ctrl Pts',(121.375735931285,-35.7587157947924,13.4046351948679));
#72428=CARTESIAN_POINT('Ctrl Pts',(121.756617543137,-35.5111305701923,13.3020820369954));
#72429=CARTESIAN_POINT('Ctrl Pts',(121.648526737397,-35.6110770987527,13.3434810852367));
#72430=CARTESIAN_POINT('Ctrl Pts',(121.540435642305,-35.7110231870809,13.3848804265588));
#72431=CARTESIAN_POINT('Ctrl Pts',(121.432344074474,-35.8109690043703,13.4262791829526));
#72432=CARTESIAN_POINT('Ctrl Pts',(121.86928828501,-35.6410554019366,13.2825757663851));
#72433=CARTESIAN_POINT('Ctrl Pts',(121.761191392211,-35.7409938552546,13.3239799148296));
#72434=CARTESIAN_POINT('Ctrl Pts',(121.653094040341,-35.8409319450386,13.3653837198587));
#72435=CARTESIAN_POINT('Ctrl Pts',(121.544996490684,-35.9408698217409,13.4067874878285));
#72436=CARTESIAN_POINT('Ctrl Pts',(121.913823234176,-35.7438605133324,13.1506538199745));
#72437=CARTESIAN_POINT('Ctrl Pts',(121.805730586267,-35.8437977872112,13.1920725002925));
#72438=CARTESIAN_POINT('Ctrl Pts',(121.697637909656,-35.9437351054287,13.2334909426446));
#72439=CARTESIAN_POINT('Ctrl Pts',(121.589544531166,-36.0436718192265,13.2749089952212));
#72440=CARTESIAN_POINT('Ctrl Pts',(121.912132034353,-35.77291329703,13.0760988223457));
#72441=CARTESIAN_POINT('Ctrl Pts',(121.804044421867,-35.8728536622539,13.1175231569589));
#72442=CARTESIAN_POINT('Ctrl Pts',(121.695956395475,-35.9727937163286,13.1589471258389));
#72443=CARTESIAN_POINT('Ctrl Pts',(121.587867965641,-36.0727334672248,13.2003707382629));
#72444=CARTESIAN_POINT('',(121.375735931285,-35.7587157947924,13.4046351948679));
#72445=CARTESIAN_POINT('',(121.587867965641,-36.0727334672234,13.2003707382624));
#72446=CARTESIAN_POINT('Origin',(121.375735931285,-35.8735208245019,13.1274713351145));
#72447=CARTESIAN_POINT('',(121.912132034353,-35.7729132970285,13.0760988223452));
#72448=CARTESIAN_POINT('Ctrl Pts',(121.587867965641,-36.0727334672248,13.2003707382629));
#72449=CARTESIAN_POINT('Ctrl Pts',(121.695956395475,-35.9727937163286,13.1589471258389));
#72450=CARTESIAN_POINT('Ctrl Pts',(121.804044421867,-35.8728536622539,13.1175231569589));
#72451=CARTESIAN_POINT('Ctrl Pts',(121.912132034353,-35.77291329703,13.0760988223457));
#72452=CARTESIAN_POINT('Origin',(121.699999999997,-35.573674503213,13.003270922209));
#72453=CARTESIAN_POINT('Ctrl Pts',(121.699999999997,-35.4588694735035,13.2804347819624));
#72454=CARTESIAN_POINT('Ctrl Pts',(121.591912387511,-35.5588186261068,13.3218350765184));
#72455=CARTESIAN_POINT('Ctrl Pts',(121.483824361119,-35.6587673966521,13.3632352128207));
#72456=CARTESIAN_POINT('Ctrl Pts',(121.375735931285,-35.7587157947924,13.4046351948679));
#72457=CARTESIAN_POINT('Origin',(121.7,-35.57367450321,13.0032709222077));
#72458=CARTESIAN_POINT('Origin',(121.7,-35.57367450321,13.0032709222077));
#72459=CARTESIAN_POINT('Origin',(113.,-35.8735208244992,13.1274713351134));
#72460=CARTESIAN_POINT('',(104.188611756946,-35.7587157947897,13.4046351948668));
#72461=CARTESIAN_POINT('',(104.5,-36.155250045634,13.2305666597347));
#72462=CARTESIAN_POINT('Ctrl Pts',(104.188611312035,-35.7587162055958,13.4046353650279));
#72463=CARTESIAN_POINT('Ctrl Pts',(104.19203735624,-35.7618832950857,13.4059472109483));
#72464=CARTESIAN_POINT('Ctrl Pts',(104.19544217649,-35.7650514088087,13.4071958583021));
#72465=CARTESIAN_POINT('Ctrl Pts',(104.234593964868,-35.8017119537402,13.4209387465913));
#72466=CARTESIAN_POINT('Ctrl Pts',(104.273440501065,-35.8404348990817,13.4283177930335));
#72467=CARTESIAN_POINT('Ctrl Pts',(104.347490784093,-35.9201909616572,13.426471158975));
#72468=CARTESIAN_POINT('Ctrl Pts',(104.382711610234,-35.9612101761365,13.4173309564933));
#72469=CARTESIAN_POINT('Ctrl Pts',(104.43587220677,-36.0296363912825,13.3858937988499));
#72470=CARTESIAN_POINT('Ctrl Pts',(104.458840813878,-36.0622177504903,13.3641404024312));
#72471=CARTESIAN_POINT('Ctrl Pts',(104.482922171696,-36.1039863436012,13.320578412409));
#72472=CARTESIAN_POINT('Ctrl Pts',(104.489283385678,-36.1167785033386,13.3042723014621));
#72473=CARTESIAN_POINT('Ctrl Pts',(104.497821708252,-36.1388370343898,13.2690296012548));
#72474=CARTESIAN_POINT('Ctrl Pts',(104.5,-36.1481043071223,13.2500938628618));
#72475=CARTESIAN_POINT('Ctrl Pts',(104.5,-36.155250045634,13.2305666597347));
#72476=CARTESIAN_POINT('',(121.375735931288,-36.155250045634,13.2305666597347));
#72477=CARTESIAN_POINT('',(113.,-36.155250045634,13.2305666597347));
#72478=CARTESIAN_POINT('Origin',(121.375735931288,-35.8735208244992,13.1274713351134));
#72479=CARTESIAN_POINT('',(113.,-35.7587157947897,13.4046351948668));
#72480=CARTESIAN_POINT('Origin',(121.375735931288,-35.8735208244991,13.1274713351135));
#72481=CARTESIAN_POINT('Origin',(121.375735931288,-35.8735208244991,13.1274713351135));
#72482=CARTESIAN_POINT('Origin',(121.7,0.,0.));
#72483=CARTESIAN_POINT('',(121.912132034352,-36.3407848610969,11.4032031398184));
#72484=CARTESIAN_POINT('Origin',(121.912132034356,0.,-1.11022302462516E-15));
#72485=CARTESIAN_POINT('Origin',(121.7,-36.1383832819456,11.3396925048197));
#72486=CARTESIAN_POINT('Origin',(121.75,0.,0.));
#72487=CARTESIAN_POINT('',(121.587867965644,-36.6543001437251,11.4871305554742));
#72488=CARTESIAN_POINT('Origin',(121.587867965644,-2.22044604925031E-15,
-1.11022302462516E-15));
#72489=CARTESIAN_POINT('Ctrl Pts',(121.912132034352,-36.3407848610989,11.4032031398191));
#72490=CARTESIAN_POINT('Ctrl Pts',(121.804044421867,-36.4452904208128,11.4311788451333));
#72491=CARTESIAN_POINT('Ctrl Pts',(121.695956395477,-36.5497955110311,11.4591546511876));
#72492=CARTESIAN_POINT('Ctrl Pts',(121.587867965644,-36.6543001437251,11.4871305554742));
#72493=CARTESIAN_POINT('Origin',(104.3,-0.608418263094196,1.98384261663693));
#72494=CARTESIAN_POINT('',(104.3,-34.4638925493512,15.6825215664905));
#72495=CARTESIAN_POINT('Origin',(104.3,-34.3490875196417,15.9596854262438));
#72496=CARTESIAN_POINT('',(104.3,-33.2241144745873,15.1689886735905));
#72497=CARTESIAN_POINT('Origin',(104.3,-32.8321455851244,15.3313475036343));
#72498=CARTESIAN_POINT('',(104.3,-0.723223292803723,1.70667875688354));
#72499=CARTESIAN_POINT('Ctrl Pts',(104.300000000003,-34.4638925493543,15.6825215664917));
#72500=CARTESIAN_POINT('Ctrl Pts',(104.408087612489,-34.5638417019577,15.7239218610477));
#72501=CARTESIAN_POINT('Ctrl Pts',(104.516175638881,-34.663790472503,15.7653219973501));
#72502=CARTESIAN_POINT('Ctrl Pts',(104.624264068715,-34.7637388706433,15.8067219793973));
#72503=CARTESIAN_POINT('Ctrl Pts',(104.243382456863,-34.5161536460432,15.7041688215248));
#72504=CARTESIAN_POINT('Ctrl Pts',(104.351473262603,-34.6161000618904,15.7455681418798));
#72505=CARTESIAN_POINT('Ctrl Pts',(104.459564357695,-34.7160463736859,15.7869669437042));
#72506=CARTESIAN_POINT('Ctrl Pts',(104.567655925526,-34.8159920802212,15.828365967482));
#72507=CARTESIAN_POINT('Ctrl Pts',(104.130709646627,-34.5942343545562,15.8098307364183));
#72508=CARTESIAN_POINT('Ctrl Pts',(104.238806539425,-34.6941786667331,15.8512207403264));
#72509=CARTESIAN_POINT('Ctrl Pts',(104.346903892804,-34.7941224771499,15.8926107306706));
#72510=CARTESIAN_POINT('Ctrl Pts',(104.455001442461,-34.8940661125617,15.934000595886));
#72511=CARTESIAN_POINT('Ctrl Pts',(104.086176765824,-34.5736426479042,15.9758096616227));
#72512=CARTESIAN_POINT('Ctrl Pts',(104.194269413733,-34.6735964016779,16.017188555955));
#72513=CARTESIAN_POINT('Ctrl Pts',(104.302362090344,-34.7735500185365,16.0585676499069));
#72514=CARTESIAN_POINT('Ctrl Pts',(104.410455468834,-34.8735029323928,16.0999465920824));
#72515=CARTESIAN_POINT('Ctrl Pts',(104.087867965647,-34.5414677238745,16.0490714263823));
#72516=CARTESIAN_POINT('Ctrl Pts',(104.195955578133,-34.6414276617498,16.0904485084352));
#72517=CARTESIAN_POINT('Ctrl Pts',(104.304043604525,-34.7413871209968,16.1318256290849));
#72518=CARTESIAN_POINT('Ctrl Pts',(104.412132034359,-34.8413461138118,16.1732027874075));
#72519=CARTESIAN_POINT('',(104.624264068715,-34.7637388706433,15.8067219793973));
#72520=CARTESIAN_POINT('',(104.412132034359,-34.8413461138104,16.1732027874068));
#72521=CARTESIAN_POINT('Origin',(104.624264068715,-34.6489338409338,16.0838858391507));
#72522=CARTESIAN_POINT('',(104.087867965647,-34.541467723873,16.0490714263816));
#72523=CARTESIAN_POINT('Ctrl Pts',(104.412132034359,-34.8413461138118,16.1732027874075));
#72524=CARTESIAN_POINT('Ctrl Pts',(104.304043604525,-34.7413871209968,16.1318256290849));
#72525=CARTESIAN_POINT('Ctrl Pts',(104.195955578133,-34.6414276617498,16.0904485084352));
#72526=CARTESIAN_POINT('Ctrl Pts',(104.087867965647,-34.5414677238745,16.0490714263823));
#72527=CARTESIAN_POINT('Origin',(104.300000000003,-34.3490875196448,15.9596854262451));
#72528=CARTESIAN_POINT('Ctrl Pts',(104.300000000003,-34.4638925493543,15.6825215664917));
#72529=CARTESIAN_POINT('Ctrl Pts',(104.408087612489,-34.5638417019577,15.7239218610477));
#72530=CARTESIAN_POINT('Ctrl Pts',(104.516175638881,-34.663790472503,15.7653219973501));
#72531=CARTESIAN_POINT('Ctrl Pts',(104.624264068715,-34.7637388706433,15.8067219793973));
#72532=CARTESIAN_POINT('Origin',(104.3,-34.3490875196417,15.9596854262438));
#72533=CARTESIAN_POINT('Origin',(104.3,-34.3490875196417,15.9596854262438));
#72534=CARTESIAN_POINT('Origin',(113.,-34.6489338409309,16.0838858391495));
#72535=CARTESIAN_POINT('',(121.811388243054,-34.7637388706404,15.8067219793961));
#72536=CARTESIAN_POINT('',(121.5,-34.9210458868021,16.210199078724));
#72537=CARTESIAN_POINT('Ctrl Pts',(121.811388687965,-34.7637392814463,15.8067221495578));
#72538=CARTESIAN_POINT('Ctrl Pts',(121.80796264376,-34.7669063670474,15.8080340048666));
#72539=CARTESIAN_POINT('Ctrl Pts',(121.80455782351,-34.7700294887557,15.8093912725525));
#72540=CARTESIAN_POINT('Ctrl Pts',(121.765406035132,-34.8056700981812,15.8255965029732));
#72541=CARTESIAN_POINT('Ctrl Pts',(121.726559498935,-34.8382691291977,15.8477599864337));
#72542=CARTESIAN_POINT('Ctrl Pts',(121.652509215907,-34.8933594144204,15.9054618065867));
#72543=CARTESIAN_POINT('Ctrl Pts',(121.617288389766,-34.9159012799814,15.9409298704602));
#72544=CARTESIAN_POINT('Ctrl Pts',(121.56412779323,-34.9420564933711,16.0115439385518));
#72545=CARTESIAN_POINT('Ctrl Pts',(121.541159186122,-34.9497130192858,16.0499644127093));
#72546=CARTESIAN_POINT('Ctrl Pts',(121.517077828304,-34.9484448961684,16.1103022466854));
#72547=CARTESIAN_POINT('Ctrl Pts',(121.510716614322,-34.9459601574395,16.1308778312071));
#72548=CARTESIAN_POINT('Ctrl Pts',(121.502178291748,-34.9366375420249,16.1713959204003));
#72549=CARTESIAN_POINT('Ctrl Pts',(121.5,-34.9298009043927,16.191338460817));
#72550=CARTESIAN_POINT('Ctrl Pts',(121.5,-34.9210458868021,16.210199078724));
#72551=CARTESIAN_POINT('',(104.624264068712,-34.9210458868021,16.210199078724));
#72552=CARTESIAN_POINT('',(113.,-34.9210458868021,16.210199078724));
#72553=CARTESIAN_POINT('Origin',(104.624264068712,-34.6489338409309,16.0838858391495));
#72554=CARTESIAN_POINT('',(113.,-34.7637388706404,15.8067219793961));
#72555=CARTESIAN_POINT('Origin',(104.624264068712,-34.6489338409309,16.0838858391494));
#72556=CARTESIAN_POINT('Origin',(104.624264068712,-34.6489338409309,16.0838858391494));
#72557=CARTESIAN_POINT('Origin',(104.3,0.,0.));
#72558=CARTESIAN_POINT('',(104.087867965647,-33.7600976763358,17.6335331415094));
#72559=CARTESIAN_POINT('Origin',(104.087867965644,0.,-2.22044604925031E-15));
#72560=CARTESIAN_POINT('Origin',(104.3,-33.5720693465106,17.5353224130539));
#72561=CARTESIAN_POINT('Origin',(104.25,0.,0.));
#72562=CARTESIAN_POINT('',(104.412132034356,-34.041132103426,17.7958762791241));
#72563=CARTESIAN_POINT('Origin',(104.412132034356,-2.22044604925031E-15,
-1.11022302462516E-15));
#72564=CARTESIAN_POINT('Ctrl Pts',(104.087867965647,-33.7600976763371,17.63353314151));
#72565=CARTESIAN_POINT('Ctrl Pts',(104.195955578132,-33.8537760772191,17.6876479205195));
#72566=CARTESIAN_POINT('Ctrl Pts',(104.304043604523,-33.9474542173515,17.7417622963114));
#72567=CARTESIAN_POINT('Ctrl Pts',(104.412132034356,-34.041132103426,17.7958762791241));
#72568=CARTESIAN_POINT('Origin',(104.624264068712,0.,0.));
#72569=CARTESIAN_POINT('',(104.624264068712,-34.1190013824203,17.8365844450781));
#72570=CARTESIAN_POINT('Origin',(104.624264068712,0.,0.));
#72571=CARTESIAN_POINT('Origin',(104.624264068712,-33.8531390339859,17.6975980727788));
#72572=CARTESIAN_POINT('Origin',(113.,0.,0.));
#72573=CARTESIAN_POINT('',(121.5,-34.1190013824203,17.8365844450781));
#72574=CARTESIAN_POINT('Origin',(121.5,0.,0.));
#72575=CARTESIAN_POINT('',(113.,-34.1190013824203,17.8365844450781));
#72576=CARTESIAN_POINT('Ctrl Pts',(104.624264068712,-33.7031390339858,17.9574056939141));
#72577=CARTESIAN_POINT('Ctrl Pts',(104.516175638879,-33.6094494902624,17.9033140106251));
#72578=CARTESIAN_POINT('Ctrl Pts',(104.408087612488,-33.5157595974544,17.8492221257921));
#72579=CARTESIAN_POINT('Ctrl Pts',(104.300000000003,-33.4220693465131,17.7951300341907));
#72580=CARTESIAN_POINT('Ctrl Pts',(104.567655925523,-33.752120102763,17.9856849271578));
#72581=CARTESIAN_POINT('Ctrl Pts',(104.459564357693,-33.6584329578312,17.9315947959052));
#72582=CARTESIAN_POINT('Ctrl Pts',(104.351473262602,-33.5647456205277,17.8775040493509));
#72583=CARTESIAN_POINT('Ctrl Pts',(104.243382456862,-33.4710578085036,17.8234135359081));
#72584=CARTESIAN_POINT('Ctrl Pts',(104.455001570347,-33.8834541246487,17.9833187182834));
#72585=CARTESIAN_POINT('Ctrl Pts',(104.346904020691,-33.789775506513,17.9292246547841));
#72586=CARTESIAN_POINT('Ctrl Pts',(104.238806667407,-33.6960966825317,17.8751305285007));
#72587=CARTESIAN_POINT('Ctrl Pts',(104.130709774609,-33.6024175423752,17.8210360125183));
#72588=CARTESIAN_POINT('Ctrl Pts',(104.410455468831,-34.0025898869996,17.8659835447083));
#72589=CARTESIAN_POINT('Ctrl Pts',(104.302362090342,-33.908914286335,17.8118754705986));
#72590=CARTESIAN_POINT('Ctrl Pts',(104.194269413732,-33.8152381372974,17.7577669311554));
#72591=CARTESIAN_POINT('Ctrl Pts',(104.086176765824,-33.72156206328,17.7036581615694));
#72592=CARTESIAN_POINT('Ctrl Pts',(104.412132034356,-34.041132103426,17.7958762791241));
#72593=CARTESIAN_POINT('Ctrl Pts',(104.304043604523,-33.9474542173515,17.7417622963114));
#72594=CARTESIAN_POINT('Ctrl Pts',(104.195955578132,-33.8537760772191,17.6876479205195));
#72595=CARTESIAN_POINT('Ctrl Pts',(104.087867965647,-33.7600976763371,17.63353314151));
#72596=CARTESIAN_POINT('',(104.300000000003,-33.4220693465131,17.7951300341907));
#72597=CARTESIAN_POINT('Origin',(104.300000000003,-33.5720693465132,17.5353224130554));
#72598=CARTESIAN_POINT('',(104.624264068712,-33.7031390339859,17.9574056939141));
#72599=CARTESIAN_POINT('Origin',(104.624264068712,-33.8531390339858,17.6975980727788));
#72600=CARTESIAN_POINT('Ctrl Pts',(104.624264068712,-33.7031390339858,17.9574056939141));
#72601=CARTESIAN_POINT('Ctrl Pts',(104.516175638879,-33.6094494902624,17.9033140106251));
#72602=CARTESIAN_POINT('Ctrl Pts',(104.408087612488,-33.5157595974544,17.8492221257921));
#72603=CARTESIAN_POINT('Ctrl Pts',(104.300000000003,-33.4220693465131,17.7951300341907));
#72604=CARTESIAN_POINT('Origin',(104.3,-2.89622949643128,-0.175381982007262));
#72605=CARTESIAN_POINT('Origin',(104.3,-33.5720693465106,17.5353224130539));
#72606=CARTESIAN_POINT('',(104.3,-32.259927238132,17.1241669750802));
#72607=CARTESIAN_POINT('',(104.3,-2.74622949643128,0.0844256391280657));
#72608=CARTESIAN_POINT('Origin',(104.3,-32.1501196169967,16.7143593539449));
#72609=CARTESIAN_POINT('Origin',(104.3,-33.5720693465106,17.5353224130539));
#72610=CARTESIAN_POINT('Origin',(104.624264068712,-33.8531390339859,17.6975980727788));
#72611=CARTESIAN_POINT('Origin',(104.624264068712,-33.8531390339859,17.6975980727788));
#72612=CARTESIAN_POINT('Origin',(113.,-34.3789638902265,15.6473429640468));
#72613=CARTESIAN_POINT('',(121.7,-33.2241144745873,15.1689886735905));
#72614=CARTESIAN_POINT('',(103.5,-33.2241144745873,15.1689886735905));
#72615=CARTESIAN_POINT('Origin',(121.7,-32.946950614834,15.0541836438809));
#72616=CARTESIAN_POINT('',(121.912131484566,-34.670610447079,15.7681469233145));
#72617=CARTESIAN_POINT('Ctrl Pts',(121.912131759621,-34.6706107010489,15.7681470285123));
#72618=CARTESIAN_POINT('Ctrl Pts',(121.938311286558,-34.6464099339429,15.7581227425572));
#72619=CARTESIAN_POINT('Ctrl Pts',(121.962987211232,-34.612270449391,15.7439817050434));
#72620=CARTESIAN_POINT('Ctrl Pts',(121.991329280155,-34.5490335349196,15.7177881174267));
#72621=CARTESIAN_POINT('Ctrl Pts',(122.,-34.5087434123029,15.7010994022092));
#72622=CARTESIAN_POINT('Ctrl Pts',(122.,-34.4745111043772,15.686919915995));
#72623=CARTESIAN_POINT('',(121.75,-34.8204869980086,15.8302278233913));
#72624=CARTESIAN_POINT('Ctrl Pts',(121.375735931288,-36.529521496889,11.1339148195199));
#72625=CARTESIAN_POINT('Ctrl Pts',(121.483824361121,-36.4250243891369,11.1059149038863));
#72626=CARTESIAN_POINT('Ctrl Pts',(121.591912387511,-36.3205268920315,11.0779148839258));
#72627=CARTESIAN_POINT('Ctrl Pts',(121.699999999996,-36.2160289954803,11.0499147569342));
#72628=CARTESIAN_POINT('Ctrl Pts',(121.432344074477,-36.5841527803644,11.1485532278086));
#72629=CARTESIAN_POINT('Ctrl Pts',(121.540435642307,-36.4796584662696,11.1205539109213));
#72630=CARTESIAN_POINT('Ctrl Pts',(121.648526737397,-36.3751635810634,11.0925548930909));
#72631=CARTESIAN_POINT('Ctrl Pts',(121.756617543136,-36.2706685250137,11.0645553747475));
#72632=CARTESIAN_POINT('Ctrl Pts',(121.544996634179,-36.6753444250015,11.2430954833527));
#72633=CARTESIAN_POINT('Ctrl Pts',(121.653094183835,-36.5708533597438,11.2151049763392));
#72634=CARTESIAN_POINT('Ctrl Pts',(121.761191535808,-36.4663621029995,11.1871143689483));
#72635=CARTESIAN_POINT('Ctrl Pts',(121.869288428606,-36.3618703486634,11.1591238127642));
#72636=CARTESIAN_POINT('Ctrl Pts',(121.589544531169,-36.6766200040331,11.410303769972));
#72637=CARTESIAN_POINT('Ctrl Pts',(121.697637909657,-36.5721211654519,11.3823253036304));
#72638=CARTESIAN_POINT('Ctrl Pts',(121.805730586267,-36.4676216100719,11.354346778571));
#72639=CARTESIAN_POINT('Ctrl Pts',(121.913823234175,-36.3631219450038,11.3263684692944));
#72640=CARTESIAN_POINT('Ctrl Pts',(121.587867965644,-36.6543001437251,11.4871305554742));
#72641=CARTESIAN_POINT('Ctrl Pts',(121.695956395477,-36.5497955110311,11.4591546511876));
#72642=CARTESIAN_POINT('Ctrl Pts',(121.804044421867,-36.4452904208128,11.4311788451333));
#72643=CARTESIAN_POINT('Ctrl Pts',(121.912132034352,-36.3407848610989,11.4032031398191));
#72644=CARTESIAN_POINT('',(121.699999999996,-36.2160289954803,11.0499147569342));
#72645=CARTESIAN_POINT('Origin',(121.699999999996,-36.1383832819496,11.3396925048209));
#72646=CARTESIAN_POINT('',(121.375735931288,-36.529521496889,11.1339148195199));
#72647=CARTESIAN_POINT('Origin',(121.375735931288,-36.4518757833582,11.4236925674066));
#72648=CARTESIAN_POINT('Ctrl Pts',(121.375735931288,-36.529521496889,11.1339148195199));
#72649=CARTESIAN_POINT('Ctrl Pts',(121.483824361121,-36.4250243891369,11.1059149038863));
#72650=CARTESIAN_POINT('Ctrl Pts',(121.591912387511,-36.3205268920315,11.0779148839258));
#72651=CARTESIAN_POINT('Ctrl Pts',(121.699999999996,-36.2160289954803,11.0499147569342));
#72652=CARTESIAN_POINT('Origin',(121.375735931288,0.,0.));
#72653=CARTESIAN_POINT('',(121.375735931288,-36.7381470591438,11.5134074305014));
#72654=CARTESIAN_POINT('Origin',(121.375735931288,0.,0.));
#72655=CARTESIAN_POINT('Origin',(121.375735931288,-36.4518757833582,11.4236925674066));
#72656=CARTESIAN_POINT('Origin',(121.375735931288,-36.4518757833582,11.4236925674066));
#72657=CARTESIAN_POINT('Origin',(121.375735931288,-36.4518757833582,11.4236925674066));
#72658=CARTESIAN_POINT('Origin',(121.7,-2.42302991782051,2.30569079837259));
#72659=CARTESIAN_POINT('Origin',(121.7,-36.1383832819455,11.3396925048198));
#72660=CARTESIAN_POINT('',(121.7,-34.9198279009177,10.7025987204178));
#72661=CARTESIAN_POINT('',(121.7,-2.50067563135127,2.01591305048587));
#72662=CARTESIAN_POINT('Origin',(121.7,-34.5524044395002,10.9147307547738));
#72663=CARTESIAN_POINT('Origin',(121.7,-36.1383832819456,11.3396925048197));
#72664=CARTESIAN_POINT('Origin',(113.,-35.3739408143757,13.2452561795175));
#72665=CARTESIAN_POINT('',(104.3,-34.2190913987366,12.7669018890611));
#72666=CARTESIAN_POINT('',(103.5,-34.2190913987366,12.7669018890611));
#72667=CARTESIAN_POINT('Origin',(104.3,-33.9419275389832,12.6520968593516));
#72668=CARTESIAN_POINT('',(104.087868515434,-35.6655873712282,13.3660601387852));
#72669=CARTESIAN_POINT('Ctrl Pts',(104.087868240379,-35.6655876251981,13.366060243983));
#72670=CARTESIAN_POINT('Ctrl Pts',(104.061688713442,-35.6413868580921,13.3560359580278));
#72671=CARTESIAN_POINT('Ctrl Pts',(104.037012788768,-35.6072473735402,13.341894920514));
#72672=CARTESIAN_POINT('Ctrl Pts',(104.008670719845,-35.5440104590688,13.3157013328973));
#72673=CARTESIAN_POINT('Ctrl Pts',(104.,-35.5037203364521,13.2990126176798));
#72674=CARTESIAN_POINT('Ctrl Pts',(104.,-35.4694880285264,13.2848331314657));
#72675=CARTESIAN_POINT('',(104.25,-35.8154639221579,13.428141038862));
#72676=CARTESIAN_POINT('Origin',(104.3,-3.98978165593707,-1.04471127832747));
#72677=CARTESIAN_POINT('',(104.3,-30.8134083466537,-22.0053456777902));
#72678=CARTESIAN_POINT('Origin',(104.3,-30.9960367753563,-21.7673396757028));
#72679=CARTESIAN_POINT('',(104.3,-29.7487867783414,-21.1884328164397));
#72680=CARTESIAN_POINT('Origin',(104.3,-29.6934092049567,-20.7677983856497));
#72681=CARTESIAN_POINT('',(104.3,-3.80715322723445,-1.28271728041484));
#72682=CARTESIAN_POINT('Ctrl Pts',(104.300000000003,-30.8134083466557,-22.0053456777917));
#72683=CARTESIAN_POINT('Ctrl Pts',(104.408087612488,-30.899236629767,-22.0712040357549));
#72684=CARTESIAN_POINT('Ctrl Pts',(104.51617563888,-30.9850645847977,-22.137062141973));
#72685=CARTESIAN_POINT('Ctrl Pts',(104.624264068714,-31.0708922200369,-22.2029200028065));
#72686=CARTESIAN_POINT('Ctrl Pts',(104.243382456862,-30.8582859677809,-22.0397814876374));
#72687=CARTESIAN_POINT('Ctrl Pts',(104.351473262603,-30.9441120388314,-22.1056379626008));
#72688=CARTESIAN_POINT('Ctrl Pts',(104.459564357694,-31.0299376087953,-22.171494606718));
#72689=CARTESIAN_POINT('Ctrl Pts',(104.567655925525,-31.1157630683464,-22.2373506156879));
#72690=CARTESIAN_POINT('Ctrl Pts',(104.130710008275,-30.9888322399386,-22.0545697937069));
#72691=CARTESIAN_POINT('Ctrl Pts',(104.238806901074,-31.0746491908742,-22.1204291050618));
#72692=CARTESIAN_POINT('Ctrl Pts',(104.346904254189,-31.1604658792464,-22.1862879890029));
#72693=CARTESIAN_POINT('Ctrl Pts',(104.455001803846,-31.2462823716881,-22.2521467836083));
#72694=CARTESIAN_POINT('Ctrl Pts',(104.086176765824,-31.1222783369416,-21.9537480036383));
#72695=CARTESIAN_POINT('Ctrl Pts',(104.194269413732,-31.2080903875008,-22.0196210464437));
#72696=CARTESIAN_POINT('Ctrl Pts',(104.302362090344,-31.293902542478,-22.0854938708675));
#72697=CARTESIAN_POINT('Ctrl Pts',(104.410455468833,-31.3797142145118,-22.1513661623616));
#72698=CARTESIAN_POINT('Ctrl Pts',(104.087867965647,-31.1696374243347,-21.8892528196839));
#72699=CARTESIAN_POINT('Ctrl Pts',(104.195955578132,-31.2554509974646,-21.9551321242181));
#72700=CARTESIAN_POINT('Ctrl Pts',(104.304043604524,-31.3412643647062,-22.0210109949498));
#72701=CARTESIAN_POINT('Ctrl Pts',(104.412132034358,-31.4270775313574,-22.0868894429031));
#72702=CARTESIAN_POINT('',(104.624264068714,-31.0708922200369,-22.2029200028065));
#72703=CARTESIAN_POINT('',(104.412132034358,-31.4270775313565,-22.0868894429024));
#72704=CARTESIAN_POINT('Origin',(104.624264068714,-31.2535206487396,-21.9649140007191));
#72705=CARTESIAN_POINT('',(104.087867965647,-31.1696374243336,-21.8892528196832));
#72706=CARTESIAN_POINT('Ctrl Pts',(104.412132034358,-31.4270775313574,-22.0868894429031));
#72707=CARTESIAN_POINT('Ctrl Pts',(104.304043604524,-31.3412643647062,-22.0210109949498));
#72708=CARTESIAN_POINT('Ctrl Pts',(104.195955578132,-31.2554509974646,-21.9551321242181));
#72709=CARTESIAN_POINT('Ctrl Pts',(104.087867965647,-31.1696374243347,-21.8892528196839));
#72710=CARTESIAN_POINT('Origin',(104.300000000003,-30.9960367753583,-21.7673396757043));
#72711=CARTESIAN_POINT('Ctrl Pts',(104.300000000003,-30.8134083466557,-22.0053456777917));
#72712=CARTESIAN_POINT('Ctrl Pts',(104.408087612488,-30.899236629767,-22.0712040357549));
#72713=CARTESIAN_POINT('Ctrl Pts',(104.51617563888,-30.9850645847977,-22.137062141973));
#72714=CARTESIAN_POINT('Ctrl Pts',(104.624264068714,-31.0708922200369,-22.2029200028065));
#72715=CARTESIAN_POINT('Origin',(104.3,-30.9960367753563,-21.7673396757028));
#72716=CARTESIAN_POINT('Origin',(104.3,-30.9960367753563,-21.7673396757028));
#72717=CARTESIAN_POINT('Origin',(113.,-31.2535206487377,-21.9649140007177));
#72718=CARTESIAN_POINT('',(121.811388243054,-31.0708922200351,-22.2029200028051));
#72719=CARTESIAN_POINT('',(121.5,-31.4989671459791,-22.1374133253307));
#72720=CARTESIAN_POINT('Ctrl Pts',(121.811388687965,-31.0708925728024,-22.2029202734925));
#72721=CARTESIAN_POINT('Ctrl Pts',(121.80796264376,-31.0736122156265,-22.2050071224247));
#72722=CARTESIAN_POINT('Ctrl Pts',(121.80455782351,-31.0763492047763,-22.2070331913203));
#72723=CARTESIAN_POINT('Ctrl Pts',(121.765406035132,-31.1082036507076,-22.2297962492787));
#72724=CARTESIAN_POINT('Ctrl Pts',(121.726559498935,-31.1436973059289,-22.2469460965475));
#72725=CARTESIAN_POINT('Ctrl Pts',(121.652509215907,-31.2212136906375,-22.2658047729756));
#72726=CARTESIAN_POINT('Ctrl Pts',(121.617288389766,-31.2632008677555,-22.2675925692634));
#72727=CARTESIAN_POINT('Ctrl Pts',(121.56412779323,-31.3374320512821,-22.2549366144545));
#72728=CARTESIAN_POINT('Ctrl Pts',(121.541159186122,-31.3745334208854,-22.2423571233226));
#72729=CARTESIAN_POINT('Ctrl Pts',(121.517077828304,-31.4261534563593,-22.2110899794998));
#72730=CARTESIAN_POINT('Ctrl Pts',(121.510716614322,-31.4427300658883,-22.1986503403778));
#72731=CARTESIAN_POINT('Ctrl Pts',(121.502178291748,-31.4731584527351,-22.1703176740025));
#72732=CARTESIAN_POINT('Ctrl Pts',(121.5,-31.4870108805359,-22.1544257019282));
#72733=CARTESIAN_POINT('Ctrl Pts',(121.5,-31.4989671459791,-22.1374133253307));
#72734=CARTESIAN_POINT('',(104.624264068712,-31.4989671459791,-22.1374133253307));
#72735=CARTESIAN_POINT('',(113.,-31.4989671459791,-22.1374133253307));
#72736=CARTESIAN_POINT('Origin',(104.624264068712,-31.2535206487377,-21.9649140007177));
#72737=CARTESIAN_POINT('',(113.,-31.0708922200351,-22.2029200028051));
#72738=CARTESIAN_POINT('Origin',(104.624264068712,-31.2535206487377,-21.9649140007178));
#72739=CARTESIAN_POINT('Origin',(104.624264068712,-31.2535206487377,-21.9649140007178));
#72740=CARTESIAN_POINT('Origin',(104.3,0.,0.));
#72741=CARTESIAN_POINT('',(104.087867965647,-32.1511364971898,-20.4203356511962));
#72742=CARTESIAN_POINT('Origin',(104.087867965644,-2.22044604925031E-15,
2.22044604925031E-15));
#72743=CARTESIAN_POINT('Origin',(104.3,-31.9720693465106,-20.3066037051641));
#72744=CARTESIAN_POINT('Origin',(104.25,0.,0.));
#72745=CARTESIAN_POINT('',(104.412132034356,-32.4322469920394,-20.5825470355869));
#72746=CARTESIAN_POINT('Origin',(104.412132034356,-2.22044604925031E-15,
2.22044604925031E-15));
#72747=CARTESIAN_POINT('Ctrl Pts',(104.087867965647,-32.1511364971911,-20.4203356511969));
#72748=CARTESIAN_POINT('Ctrl Pts',(104.195955578132,-32.2448404709744,-20.4744061366419));
#72749=CARTESIAN_POINT('Ctrl Pts',(104.304043604523,-32.3385439651864,-20.5284765978799));
#72750=CARTESIAN_POINT('Ctrl Pts',(104.412132034356,-32.4322469920394,-20.5825470355869));
#72751=CARTESIAN_POINT('Origin',(104.624264068712,0.,0.));
#72752=CARTESIAN_POINT('',(104.624264068712,-32.5064359373941,-20.6296297263933));
#72753=CARTESIAN_POINT('Origin',(104.624264068712,0.,0.));
#72754=CARTESIAN_POINT('Origin',(104.624264068712,-32.2531390339859,-20.468879364889));
#72755=CARTESIAN_POINT('Origin',(113.,0.,0.));
#72756=CARTESIAN_POINT('',(121.5,-32.5064359373941,-20.6296297263933));
#72757=CARTESIAN_POINT('Origin',(121.5,0.,0.));
#72758=CARTESIAN_POINT('',(113.,-32.5064359373941,-20.6296297263933));
#72759=CARTESIAN_POINT('Origin',(121.7,-2.74230173957738,-2.86772609312011));
#72760=CARTESIAN_POINT('',(121.7,-34.4638925493513,-15.6825215664904));
#72761=CARTESIAN_POINT('Origin',(121.7,-34.3490875196417,-15.9596854262438));
#72762=CARTESIAN_POINT('',(121.7,-33.2241144745874,-15.1689886735904));
#72763=CARTESIAN_POINT('Origin',(121.7,-32.8321455851244,-15.3313475036343));
#72764=CARTESIAN_POINT('',(121.7,-2.8571067692869,-2.59056223336672));
#72765=CARTESIAN_POINT('Ctrl Pts',(121.699999999997,-34.4638925493544,-15.6825215664917));
#72766=CARTESIAN_POINT('Ctrl Pts',(121.591912387511,-34.5638417019577,-15.7239218610477));
#72767=CARTESIAN_POINT('Ctrl Pts',(121.483824361119,-34.663790472503,-15.7653219973501));
#72768=CARTESIAN_POINT('Ctrl Pts',(121.375735931285,-34.7637388706433,-15.8067219793973));
#72769=CARTESIAN_POINT('Ctrl Pts',(121.756617543137,-34.5161536460432,-15.7041688215248));
#72770=CARTESIAN_POINT('Ctrl Pts',(121.648526737397,-34.6161000618905,-15.7455681418798));
#72771=CARTESIAN_POINT('Ctrl Pts',(121.540435642305,-34.7160463736859,-15.7869669437042));
#72772=CARTESIAN_POINT('Ctrl Pts',(121.432344074474,-34.8159920802212,-15.828365967482));
#72773=CARTESIAN_POINT('Ctrl Pts',(121.869288077041,-34.5942310582327,-15.8098327514129));
#72774=CARTESIAN_POINT('Ctrl Pts',(121.761191184242,-34.6941753704096,-15.851222755321));
#72775=CARTESIAN_POINT('Ctrl Pts',(121.653093832523,-34.7941191828858,-15.8926127449365));
#72776=CARTESIAN_POINT('Ctrl Pts',(121.544996282866,-34.8940628182975,-15.9340026101519));
#72777=CARTESIAN_POINT('Ctrl Pts',(121.913823234176,-34.5736426479043,-15.9758096616227));
#72778=CARTESIAN_POINT('Ctrl Pts',(121.805730586267,-34.673596401678,-16.017188555955));
#72779=CARTESIAN_POINT('Ctrl Pts',(121.697637909656,-34.7735500185365,-16.0585676499069));
#72780=CARTESIAN_POINT('Ctrl Pts',(121.589544531166,-34.8735029323928,-16.0999465920823));
#72781=CARTESIAN_POINT('Ctrl Pts',(121.912132034353,-34.5414677238746,-16.0490714263823));
#72782=CARTESIAN_POINT('Ctrl Pts',(121.804044421867,-34.6414276617498,-16.0904485084352));
#72783=CARTESIAN_POINT('Ctrl Pts',(121.695956395475,-34.7413871209968,-16.1318256290849));
#72784=CARTESIAN_POINT('Ctrl Pts',(121.587867965641,-34.8413461138118,-16.1732027874074));
#72785=CARTESIAN_POINT('',(121.375735931285,-34.7637388706433,-15.8067219793973));
#72786=CARTESIAN_POINT('',(121.587867965641,-34.8413461138104,-16.1732027874068));
#72787=CARTESIAN_POINT('Origin',(121.375735931285,-34.6489338409338,-16.0838858391507));
#72788=CARTESIAN_POINT('',(121.912132034353,-34.5414677238731,-16.0490714263816));
#72789=CARTESIAN_POINT('Ctrl Pts',(121.587867965641,-34.8413461138118,-16.1732027874074));
#72790=CARTESIAN_POINT('Ctrl Pts',(121.695956395475,-34.7413871209968,-16.1318256290849));
#72791=CARTESIAN_POINT('Ctrl Pts',(121.804044421867,-34.6414276617498,-16.0904485084352));
#72792=CARTESIAN_POINT('Ctrl Pts',(121.912132034353,-34.5414677238746,-16.0490714263823));
#72793=CARTESIAN_POINT('Origin',(121.699999999997,-34.3490875196449,-15.9596854262451));
#72794=CARTESIAN_POINT('Ctrl Pts',(121.699999999997,-34.4638925493544,-15.6825215664917));
#72795=CARTESIAN_POINT('Ctrl Pts',(121.591912387511,-34.5638417019577,-15.7239218610477));
#72796=CARTESIAN_POINT('Ctrl Pts',(121.483824361119,-34.663790472503,-15.7653219973501));
#72797=CARTESIAN_POINT('Ctrl Pts',(121.375735931285,-34.7637388706433,-15.8067219793973));
#72798=CARTESIAN_POINT('Origin',(121.7,-34.3490875196417,-15.9596854262438));
#72799=CARTESIAN_POINT('Origin',(121.7,-34.3490875196417,-15.9596854262438));
#72800=CARTESIAN_POINT('Origin',(113.,-34.6489338409309,-16.0838858391495));
#72801=CARTESIAN_POINT('',(104.188611756946,-34.7637388706404,-15.8067219793961));
#72802=CARTESIAN_POINT('',(104.5,-34.9210458868021,-16.210199078724));
#72803=CARTESIAN_POINT('Ctrl Pts',(104.188611312035,-34.7637392814463,-15.8067221495578));
#72804=CARTESIAN_POINT('Ctrl Pts',(104.19203735624,-34.7669063670474,-15.8080340048666));
#72805=CARTESIAN_POINT('Ctrl Pts',(104.19544217649,-34.7700294887557,-15.8093912725525));
#72806=CARTESIAN_POINT('Ctrl Pts',(104.234593964868,-34.8056700981812,-15.8255965029732));
#72807=CARTESIAN_POINT('Ctrl Pts',(104.273440501065,-34.8382691291977,-15.8477599864337));
#72808=CARTESIAN_POINT('Ctrl Pts',(104.347490784093,-34.8933594144204,-15.9054618065867));
#72809=CARTESIAN_POINT('Ctrl Pts',(104.382711610234,-34.9159012799815,-15.9409298704602));
#72810=CARTESIAN_POINT('Ctrl Pts',(104.43587220677,-34.9420564933711,-16.0115439385517));
#72811=CARTESIAN_POINT('Ctrl Pts',(104.458840813878,-34.9497130192858,-16.0499644127093));
#72812=CARTESIAN_POINT('Ctrl Pts',(104.482922171696,-34.9484448961684,-16.1103022466853));
#72813=CARTESIAN_POINT('Ctrl Pts',(104.489283385678,-34.9459601574395,-16.1308778312071));
#72814=CARTESIAN_POINT('Ctrl Pts',(104.497821708252,-34.9366375420249,-16.1713959204003));
#72815=CARTESIAN_POINT('Ctrl Pts',(104.5,-34.9298009043927,-16.1913384608169));
#72816=CARTESIAN_POINT('Ctrl Pts',(104.5,-34.9210458868021,-16.210199078724));
#72817=CARTESIAN_POINT('',(121.375735931288,-34.9210458868021,-16.210199078724));
#72818=CARTESIAN_POINT('',(113.,-34.9210458868021,-16.210199078724));
#72819=CARTESIAN_POINT('Origin',(121.375735931288,-34.6489338409309,-16.0838858391495));
#72820=CARTESIAN_POINT('',(113.,-34.7637388706404,-15.8067219793961));
#72821=CARTESIAN_POINT('Origin',(121.375735931288,-34.648933840931,-16.0838858391494));
#72822=CARTESIAN_POINT('Origin',(121.375735931288,-34.648933840931,-16.0838858391494));
#72823=CARTESIAN_POINT('Origin',(121.7,0.,0.));
#72824=CARTESIAN_POINT('',(121.912132034353,-33.7600976763358,-17.6335331415093));
#72825=CARTESIAN_POINT('Origin',(121.912132034356,-2.22044604925031E-15,
1.11022302462516E-15));
#72826=CARTESIAN_POINT('Origin',(121.7,-33.5720693465106,-17.535322413054));
#72827=CARTESIAN_POINT('Origin',(121.75,0.,0.));
#72828=CARTESIAN_POINT('',(121.587867965644,-34.0411321034261,-17.7958762791241));
#72829=CARTESIAN_POINT('Origin',(121.587867965644,-2.22044604925031E-15,
2.22044604925031E-15));
#72830=CARTESIAN_POINT('Ctrl Pts',(121.912132034353,-33.7600976763372,-17.63353314151));
#72831=CARTESIAN_POINT('Ctrl Pts',(121.804044421868,-33.8537760772191,-17.6876479205194));
#72832=CARTESIAN_POINT('Ctrl Pts',(121.695956395477,-33.9474542173515,-17.7417622963114));
#72833=CARTESIAN_POINT('Ctrl Pts',(121.587867965644,-34.0411321034261,-17.7958762791241));
#72834=CARTESIAN_POINT('Ctrl Pts',(104.624264068712,-36.529521496889,-11.1339148195198));
#72835=CARTESIAN_POINT('Ctrl Pts',(104.516175638879,-36.4250243891369,-11.1059149038863));
#72836=CARTESIAN_POINT('Ctrl Pts',(104.408087612489,-36.3205268920315,-11.0779148839258));
#72837=CARTESIAN_POINT('Ctrl Pts',(104.300000000004,-36.2160289954803,-11.0499147569342));
#72838=CARTESIAN_POINT('Ctrl Pts',(104.567655925523,-36.5841527803644,-11.1485532278086));
#72839=CARTESIAN_POINT('Ctrl Pts',(104.459564357693,-36.4796584662696,-11.1205539109213));
#72840=CARTESIAN_POINT('Ctrl Pts',(104.351473262603,-36.3751635810634,-11.0925548930909));
#72841=CARTESIAN_POINT('Ctrl Pts',(104.243382456864,-36.2706685250137,-11.0645553747475));
#72842=CARTESIAN_POINT('Ctrl Pts',(104.455001016882,-36.6753475262196,-11.2430929770909));
#72843=CARTESIAN_POINT('Ctrl Pts',(104.346903467226,-36.5708564609618,-11.2151024700774));
#72844=CARTESIAN_POINT('Ctrl Pts',(104.238806113538,-36.4663652062277,-11.1871118616628));
#72845=CARTESIAN_POINT('Ctrl Pts',(104.130709220741,-36.3618734518916,-11.1591213054788));
#72846=CARTESIAN_POINT('Ctrl Pts',(104.410455468831,-36.6766200040331,-11.410303769972));
#72847=CARTESIAN_POINT('Ctrl Pts',(104.302362090343,-36.5721211654519,-11.3823253036304));
#72848=CARTESIAN_POINT('Ctrl Pts',(104.194269413733,-36.467621610072,-11.354346778571));
#72849=CARTESIAN_POINT('Ctrl Pts',(104.086176765825,-36.3631219450038,-11.3263684692943));
#72850=CARTESIAN_POINT('Ctrl Pts',(104.412132034356,-36.6543001437251,-11.4871305554741));
#72851=CARTESIAN_POINT('Ctrl Pts',(104.304043604523,-36.5497955110311,-11.4591546511876));
#72852=CARTESIAN_POINT('Ctrl Pts',(104.195955578133,-36.4452904208128,-11.4311788451333));
#72853=CARTESIAN_POINT('Ctrl Pts',(104.087867965648,-36.3407848610989,-11.403203139819));
#72854=CARTESIAN_POINT('',(104.300000000004,-36.2160289954803,-11.0499147569342));
#72855=CARTESIAN_POINT('Origin',(104.300000000004,-36.1383832819496,-11.3396925048209));
#72856=CARTESIAN_POINT('',(104.624264068712,-36.529521496889,-11.1339148195198));
#72857=CARTESIAN_POINT('Origin',(104.624264068712,-36.4518757833583,-11.4236925674066));
#72858=CARTESIAN_POINT('Ctrl Pts',(104.624264068712,-36.529521496889,-11.1339148195198));
#72859=CARTESIAN_POINT('Ctrl Pts',(104.516175638879,-36.4250243891369,-11.1059149038863));
#72860=CARTESIAN_POINT('Ctrl Pts',(104.408087612489,-36.3205268920315,-11.0779148839258));
#72861=CARTESIAN_POINT('Ctrl Pts',(104.300000000004,-36.2160289954803,-11.0499147569342));
#72862=CARTESIAN_POINT('Origin',(104.3,-0.0904981630899659,-1.68069079837259));
#72863=CARTESIAN_POINT('Origin',(104.3,-36.1383832819455,-11.3396925048198));
#72864=CARTESIAN_POINT('',(104.3,-34.9198279009177,-10.7025987204178));
#72865=CARTESIAN_POINT('',(104.3,-0.168143876620722,-1.39091305048587));
#72866=CARTESIAN_POINT('Origin',(104.3,-34.5524044395002,-10.9147307547737));
#72867=CARTESIAN_POINT('Origin',(104.3,-36.1383832819455,-11.3396925048198));
#72868=CARTESIAN_POINT('Origin',(104.624264068712,-36.4518757833583,-11.4236925674066));
#72869=CARTESIAN_POINT('Origin',(104.624264068712,-36.4518757833583,-11.4236925674066));
#72870=CARTESIAN_POINT('Origin',(113.,-35.3739408143757,-13.2452561795174));
#72871=CARTESIAN_POINT('',(121.7,-34.2190913987366,-12.7669018890611));
#72872=CARTESIAN_POINT('',(103.5,-34.2190913987366,-12.7669018890611));
#72873=CARTESIAN_POINT('Origin',(121.7,-33.9419275389832,-12.6520968593516));
#72874=CARTESIAN_POINT('',(121.912131484566,-35.6655873712282,-13.3660601387852));
#72875=CARTESIAN_POINT('Ctrl Pts',(121.912131759621,-35.6655876251981,-13.366060243983));
#72876=CARTESIAN_POINT('Ctrl Pts',(121.938311286558,-35.6413868580921,-13.3560359580278));
#72877=CARTESIAN_POINT('Ctrl Pts',(121.962987211232,-35.6072473735403,-13.341894920514));
#72878=CARTESIAN_POINT('Ctrl Pts',(121.991329280155,-35.5440104590688,-13.3157013328973));
#72879=CARTESIAN_POINT('Ctrl Pts',(122.,-35.5037203364522,-13.2990126176798));
#72880=CARTESIAN_POINT('Ctrl Pts',(122.,-35.4694880285265,-13.2848331314657));
#72881=CARTESIAN_POINT('',(121.75,-35.8154639221579,-13.4281410388619));
#72882=CARTESIAN_POINT('Ctrl Pts',(104.624264068712,-37.6702738824291,-6.27060329017722));
#72883=CARTESIAN_POINT('Ctrl Pts',(104.51617563888,-37.56301603955,-6.25648252727636));
#72884=CARTESIAN_POINT('Ctrl Pts',(104.408087612489,-37.4557577970312,-6.24236171176192));
#72885=CARTESIAN_POINT('Ctrl Pts',(104.300000000005,-37.3484991445136,-6.22824084227012));
#72886=CARTESIAN_POINT('Ctrl Pts',(104.567655925523,-37.7263484833951,-6.27798565144562));
#72887=CARTESIAN_POINT('Ctrl Pts',(104.459564357694,-37.6190934884253,-6.26386511752329));
#72888=CARTESIAN_POINT('Ctrl Pts',(104.351473262604,-37.5118379662647,-6.24974495464426));
#72889=CARTESIAN_POINT('Ctrl Pts',(104.243382456865,-37.4045822093923,-6.23562431783376));
#72890=CARTESIAN_POINT('Ctrl Pts',(104.455000447563,-37.8291036249763,-6.35981259677795));
#72891=CARTESIAN_POINT('Ctrl Pts',(104.346902897908,-37.7218530009686,-6.34570037330132));
#72892=CARTESIAN_POINT('Ctrl Pts',(104.238805543805,-37.6146021763207,-6.33158807371323));
#72893=CARTESIAN_POINT('Ctrl Pts',(104.130708651008,-37.5073508627117,-6.31747589142946));
#72894=CARTESIAN_POINT('Ctrl Pts',(104.410455468831,-37.852189938727,-6.52542748682474));
#72895=CARTESIAN_POINT('Ctrl Pts',(104.302362090343,-37.7449331795208,-6.51132821563267));
#72896=CARTESIAN_POINT('Ctrl Pts',(104.194269413733,-37.6376757019839,-6.49722897978621));
#72897=CARTESIAN_POINT('Ctrl Pts',(104.086176765826,-37.5304181438625,-6.48312997219362));
#72898=CARTESIAN_POINT('Ctrl Pts',(104.412132034356,-37.8400889356902,-6.60451033490358));
#72899=CARTESIAN_POINT('Ctrl Pts',(104.304043604524,-37.7328267663559,-6.59041436013136));
#72900=CARTESIAN_POINT('Ctrl Pts',(104.195955578133,-37.6255641562333,-6.5763185424699));
#72901=CARTESIAN_POINT('Ctrl Pts',(104.087867965649,-37.5183010937809,-6.56222288596809));
#72902=CARTESIAN_POINT('',(104.300000000005,-37.3484991445136,-6.22824084227012));
#72903=CARTESIAN_POINT('Origin',(104.300000000005,-37.3093412868476,-6.52567430068227));
#72904=CARTESIAN_POINT('',(104.624264068712,-37.6702738824291,-6.27060329017722));
#72905=CARTESIAN_POINT('Origin',(104.624264068712,-37.6311160247631,-6.56803674858937));
#72906=CARTESIAN_POINT('Ctrl Pts',(104.624264068712,-37.6702738824291,-6.27060329017722));
#72907=CARTESIAN_POINT('Ctrl Pts',(104.51617563888,-37.56301603955,-6.25648252727636));
#72908=CARTESIAN_POINT('Ctrl Pts',(104.408087612489,-37.4557577970312,-6.24236171176192));
#72909=CARTESIAN_POINT('Ctrl Pts',(104.300000000005,-37.3484991445136,-6.22824084227012));
#72910=CARTESIAN_POINT('Origin',(104.3,0.171615498867558,-1.59121272787762));
#72911=CARTESIAN_POINT('Origin',(104.3,-37.3093412868425,-6.52567430068159));
#72912=CARTESIAN_POINT('',(104.3,-36.018053390258,-6.05308433581783));
#72913=CARTESIAN_POINT('',(104.3,0.132457641201542,-1.29377926946548));
#72914=CARTESIAN_POINT('Origin',(104.3,-35.6814620741799,-6.31135993656395));
#72915=CARTESIAN_POINT('Origin',(104.3,-37.3093412868425,-6.52567430068159));
#72916=CARTESIAN_POINT('Origin',(104.624264068712,-37.6311160247631,-6.56803674858937));
#72917=CARTESIAN_POINT('Origin',(104.624264068712,-37.6311160247631,-6.56803674858937));
#72918=CARTESIAN_POINT('Origin',(113.,-36.8001647010456,-8.51471537844435));
#72919=CARTESIAN_POINT('',(121.7,-35.5927574181843,-8.1911915720662));
#72920=CARTESIAN_POINT('',(103.5,-35.5927574181843,-8.1911915720662));
#72921=CARTESIAN_POINT('Origin',(121.7,-35.3029796702975,-8.11354585853545));
#72922=CARTESIAN_POINT('',(121.912131484566,-37.1050842619827,-8.5964183285539));
#72923=CARTESIAN_POINT('Ctrl Pts',(121.912131759621,-37.105084527511,-8.59641839970199));
#72924=CARTESIAN_POINT('Ctrl Pts',(121.938311286558,-37.0797823694469,-8.58963870688197));
#72925=CARTESIAN_POINT('Ctrl Pts',(121.962987211232,-37.0440891771373,-8.58007474482732));
#72926=CARTESIAN_POINT('Ctrl Pts',(121.991329280155,-36.9779743139833,-8.5623593206375));
#72927=CARTESIAN_POINT('Ctrl Pts',(122.,-36.9358505645005,-8.55107229598142));
#72928=CARTESIAN_POINT('Ctrl Pts',(122.,-36.9000603243714,-8.54148233004191));
#72929=CARTESIAN_POINT('',(121.75,-37.261781781739,-8.63840530242856));
#72930=CARTESIAN_POINT('Origin',(104.3,0.125,1.6));
#72931=CARTESIAN_POINT('',(104.3,-37.8419261182179,1.3));
#72932=CARTESIAN_POINT('Origin',(104.3,-37.8419261182179,1.6));
#72933=CARTESIAN_POINT('',(104.3,-36.5,1.3));
#72934=CARTESIAN_POINT('Origin',(104.3,-36.2,1.6));
#72935=CARTESIAN_POINT('',(104.3,0.125,1.3));
#72936=CARTESIAN_POINT('Ctrl Pts',(104.300000000006,-37.8419261182243,1.3));
#72937=CARTESIAN_POINT('Ctrl Pts',(104.408087612492,-37.9501103014279,1.3));
#72938=CARTESIAN_POINT('Ctrl Pts',(104.516175638884,-38.0582940710949,1.3));
#72939=CARTESIAN_POINT('Ctrl Pts',(104.624264068718,-38.1664774376736,1.3));
#72940=CARTESIAN_POINT('Ctrl Pts',(104.243382456866,-37.8984931216591,1.3));
#72941=CARTESIAN_POINT('Ctrl Pts',(104.351473262606,-38.0066744036192,1.30000014726687));
#72942=CARTESIAN_POINT('Ctrl Pts',(104.459564357698,-38.1148553910149,1.29999985529285));
#72943=CARTESIAN_POINT('Ctrl Pts',(104.567655925529,-38.2230359041609,1.3));
#72944=CARTESIAN_POINT('Ctrl Pts',(104.130707929307,-38.0110670701893,1.36773633088588));
#72945=CARTESIAN_POINT('Ctrl Pts',(104.238804822106,-38.1192428433615,1.36772867591791));
#72946=CARTESIAN_POINT('Ctrl Pts',(104.346902176736,-38.2274181465522,1.36772120153623));
#72947=CARTESIAN_POINT('Ctrl Pts',(104.454999726393,-38.3355932413995,1.36771367741974));
#72948=CARTESIAN_POINT('Ctrl Pts',(104.086176765827,-38.0555584828822,1.5289633238052));
#72949=CARTESIAN_POINT('Ctrl Pts',(104.194269413736,-38.1637387275019,1.52894179178494));
#72950=CARTESIAN_POINT('Ctrl Pts',(104.302362090347,-38.2719189220196,1.52892049658419));
#72951=CARTESIAN_POINT('Ctrl Pts',(104.410455468836,-38.3800984089656,1.52889933018763));
#72952=CARTESIAN_POINT('Ctrl Pts',(104.08786796565,-38.0538687927104,1.60896117914607));
#72953=CARTESIAN_POINT('Ctrl Pts',(104.195955578136,-38.1620540571656,1.60893560624471));
#72954=CARTESIAN_POINT('Ctrl Pts',(104.304043604528,-38.2702388941964,1.60891025216514));
#72955=CARTESIAN_POINT('Ctrl Pts',(104.412132034362,-38.3784233147169,1.60888511138664));
#72956=CARTESIAN_POINT('',(104.624264068718,-38.1664774376736,1.3));
#72957=CARTESIAN_POINT('',(104.412132034362,-38.378423314714,1.60888511138652));
#72958=CARTESIAN_POINT('Origin',(104.624264068718,-38.1664774376736,1.6));
#72959=CARTESIAN_POINT('',(104.08786796565,-38.0538687927072,1.60896117914594));
#72960=CARTESIAN_POINT('Ctrl Pts',(104.412132034362,-38.3784233147169,1.60888511138664));
#72961=CARTESIAN_POINT('Ctrl Pts',(104.304043604528,-38.2702388941964,1.60891025216514));
#72962=CARTESIAN_POINT('Ctrl Pts',(104.195955578136,-38.1620540571656,1.60893560624471));
#72963=CARTESIAN_POINT('Ctrl Pts',(104.08786796565,-38.0538687927104,1.60896117914607));
#72964=CARTESIAN_POINT('Origin',(104.300000000006,-37.8419261182243,1.6));
#72965=CARTESIAN_POINT('Ctrl Pts',(104.300000000006,-37.8419261182243,1.3));
#72966=CARTESIAN_POINT('Ctrl Pts',(104.408087612492,-37.9501103014279,1.3));
#72967=CARTESIAN_POINT('Ctrl Pts',(104.516175638884,-38.0582940710949,1.3));
#72968=CARTESIAN_POINT('Ctrl Pts',(104.624264068718,-38.1664774376736,1.3));
#72969=CARTESIAN_POINT('Origin',(104.3,-37.8419261182179,1.6));
#72970=CARTESIAN_POINT('Origin',(104.3,-37.8419261182179,1.6));
#72971=CARTESIAN_POINT('Origin',(113.,-38.1664774376677,1.60000000000001));
#72972=CARTESIAN_POINT('',(121.811388243054,-38.1664774376677,1.3));
#72973=CARTESIAN_POINT('',(121.5,-38.4662141714714,1.61256544502619));
#72974=CARTESIAN_POINT('Ctrl Pts',(121.811388687965,-38.1664778823209,1.30000000000034));
#72975=CARTESIAN_POINT('Ctrl Pts',(121.80796264376,-38.1699059131779,1.30000000508129));
#72976=CARTESIAN_POINT('Ctrl Pts',(121.80455782351,-38.1733107052584,1.3000587899814));
#72977=CARTESIAN_POINT('Ctrl Pts',(121.765406035132,-38.2124398080324,1.30139139994019));
#72978=CARTESIAN_POINT('Ctrl Pts',(121.726559498935,-38.2510389834921,1.30939267959733));
#72979=CARTESIAN_POINT('Ctrl Pts',(121.652509215907,-38.3240173010395,1.34162007078636));
#72980=CARTESIAN_POINT('Ctrl Pts',(121.617288389766,-38.3584163096784,1.36576189057208));
#72981=CARTESIAN_POINT('Ctrl Pts',(121.56412779323,-38.4096034099481,1.420991615955));
#72982=CARTESIAN_POINT('Ctrl Pts',(121.541159186122,-38.4313799964546,1.45355748004154));
#72983=CARTESIAN_POINT('Ctrl Pts',(121.517077828304,-38.4532986928691,1.50978765959528));
#72984=CARTESIAN_POINT('Ctrl Pts',(121.510716614322,-38.4588770289215,1.52974788934973));
#72985=CARTESIAN_POINT('Ctrl Pts',(121.502178291748,-38.4657696567958,1.57074933311724));
#72986=CARTESIAN_POINT('Ctrl Pts',(121.5,-38.4670851070329,1.59179010598939));
#72987=CARTESIAN_POINT('Ctrl Pts',(121.5,-38.4662141714714,1.61256544502619));
#72988=CARTESIAN_POINT('',(104.624264068712,-38.4662141714714,1.61256544502619));
#72989=CARTESIAN_POINT('',(113.,-38.4662141714714,1.61256544502619));
#72990=CARTESIAN_POINT('Origin',(104.624264068712,-38.1664774376677,1.60000000000001));
#72991=CARTESIAN_POINT('',(113.,-38.1664774376677,1.3));
#72992=CARTESIAN_POINT('Origin',(104.624264068712,-38.1664774376677,1.59999999999976));
#72993=CARTESIAN_POINT('Origin',(104.624264068712,-38.1664774376677,1.59999999999976));
#72994=CARTESIAN_POINT('Origin',(104.3,0.,0.));
#72995=CARTESIAN_POINT('',(104.087867965649,-37.938324246066,3.37183029953926));
#72996=CARTESIAN_POINT('Origin',(104.087867965644,0.,-1.38777878078145E-15));
#72997=CARTESIAN_POINT('Origin',(104.3,-37.7270251019467,3.35305074428542));
#72998=CARTESIAN_POINT('Origin',(104.25,0.,0.));
#72999=CARTESIAN_POINT('',(104.412132034356,-38.2600922303079,3.41426858245338));
#73000=CARTESIAN_POINT('Origin',(104.412132034356,0.,-1.11022302462516E-15));
#73001=CARTESIAN_POINT('Ctrl Pts',(104.087867965649,-37.9383242460686,3.37183029953949));
#73002=CARTESIAN_POINT('Ctrl Pts',(104.195955578133,-38.0455806326541,3.38597666428458));
#73003=CARTESIAN_POINT('Ctrl Pts',(104.304043604524,-38.1528366240338,3.40012275628986));
#73004=CARTESIAN_POINT('Ctrl Pts',(104.412132034356,-38.2600922303079,3.41426858245338));
#73005=CARTESIAN_POINT('Origin',(104.624264068712,0.,0.));
#73006=CARTESIAN_POINT('',(104.624264068712,-38.3476124040547,3.42207874082298));
#73007=CARTESIAN_POINT('Origin',(104.624264068712,0.,0.));
#73008=CARTESIAN_POINT('Origin',(104.624264068712,-38.0487998398672,3.39541319219319));
#73009=CARTESIAN_POINT('Origin',(113.,0.,0.));
#73010=CARTESIAN_POINT('',(121.5,-38.3476124040547,3.42207874082298));
#73011=CARTESIAN_POINT('Origin',(121.5,0.,0.));
#73012=CARTESIAN_POINT('',(113.,-38.3476124040547,3.42207874082298));
#73013=CARTESIAN_POINT('Ctrl Pts',(104.624264068712,-37.2024510141555,8.62250767116828));
#73014=CARTESIAN_POINT('Ctrl Pts',(104.516175638879,-37.0979539064034,8.59450775553471));
#73015=CARTESIAN_POINT('Ctrl Pts',(104.408087612489,-36.9934564092979,8.56650773557423));
#73016=CARTESIAN_POINT('Ctrl Pts',(104.300000000004,-36.8889585127468,8.53850760858259));
#73017=CARTESIAN_POINT('Ctrl Pts',(104.567655925523,-37.257082297631,8.637146079457));
#73018=CARTESIAN_POINT('Ctrl Pts',(104.459564357693,-37.1525879086301,8.60914704212251));
#73019=CARTESIAN_POINT('Ctrl Pts',(104.351473262603,-37.0480931745608,8.58114746024158));
#73020=CARTESIAN_POINT('Ctrl Pts',(104.243382456864,-36.9435980422802,8.55314822639588));
#73021=CARTESIAN_POINT('Ctrl Pts',(104.455000696706,-37.3833293341471,8.60087013504746));
#73022=CARTESIAN_POINT('Ctrl Pts',(104.346903147051,-37.2788421636586,8.57286509255706));
#73023=CARTESIAN_POINT('Ctrl Pts',(104.23880579313,-37.1743547785458,8.54486004340221));
#73024=CARTESIAN_POINT('Ctrl Pts',(104.130708900332,-37.0698669867127,8.5168546989556));
#73025=CARTESIAN_POINT('Ctrl Pts',(104.410455468831,-37.4680365334272,8.45669707232344));
#73026=CARTESIAN_POINT('Ctrl Pts',(104.302362090343,-37.363548651379,8.42867771564362));
#73027=CARTESIAN_POINT('Ctrl Pts',(104.194269413732,-37.2590601192061,8.40065805141547));
#73028=CARTESIAN_POINT('Ctrl Pts',(104.086176765825,-37.1545715999318,8.3726381454699));
#73029=CARTESIAN_POINT('Ctrl Pts',(104.412132034356,-37.4871203601426,8.37900319423351));
#73030=CARTESIAN_POINT('Ctrl Pts',(104.304043604523,-37.3826287412732,8.35097872169248));
#73031=CARTESIAN_POINT('Ctrl Pts',(104.195955578133,-37.2781367752921,8.32295393531766));
#73032=CARTESIAN_POINT('Ctrl Pts',(104.087867965648,-37.173644453086,8.29492882695164));
#73033=CARTESIAN_POINT('',(104.300000000004,-36.8889585127468,8.53850760858259));
#73034=CARTESIAN_POINT('Origin',(104.300000000004,-36.9666042262775,8.24872986069587));
#73035=CARTESIAN_POINT('',(104.624264068712,-37.2024510141556,8.62250767116828));
#73036=CARTESIAN_POINT('Origin',(104.624264068712,-37.2800967276863,8.33272992328156));
#73037=CARTESIAN_POINT('Ctrl Pts',(104.624264068712,-37.2024510141555,8.62250767116828));
#73038=CARTESIAN_POINT('Ctrl Pts',(104.516175638879,-37.0979539064034,8.59450775553471));
#73039=CARTESIAN_POINT('Ctrl Pts',(104.408087612489,-36.9934564092979,8.56650773557423));
#73040=CARTESIAN_POINT('Ctrl Pts',(104.300000000004,-36.8889585127468,8.53850760858259));
#73041=CARTESIAN_POINT('Origin',(104.3,-0.918719107418034,-1.41027184575243));
#73042=CARTESIAN_POINT('Origin',(104.3,-36.9666042262736,8.24872986069481));
#73043=CARTESIAN_POINT('',(104.3,-35.5927574181843,8.19119157206623));
#73044=CARTESIAN_POINT('',(104.3,-0.841073393887278,-1.12049409786571));
#73045=CARTESIAN_POINT('Origin',(104.3,-35.3806253838283,7.82376811064875));
#73046=CARTESIAN_POINT('Origin',(104.3,-36.9666042262736,8.24872986069481));
#73047=CARTESIAN_POINT('Origin',(104.624264068712,-37.2800967276863,8.33272992328156));
#73048=CARTESIAN_POINT('Origin',(104.624264068712,-37.2800967276863,8.33272992328156));
#73049=CARTESIAN_POINT('Origin',(113.,-37.2800967276863,8.33272992328156));
#73050=CARTESIAN_POINT('',(121.811388243054,-37.2024510141556,8.62250767116829));
#73051=CARTESIAN_POINT('Ctrl Pts',(121.5,-37.5728723564378,8.39817021063717));
#73052=CARTESIAN_POINT('Ctrl Pts',(121.5,-37.5683365621785,8.41846306187311));
#73053=CARTESIAN_POINT('Ctrl Pts',(121.502178291748,-37.5616201820783,8.43844642422115));
#73054=CARTESIAN_POINT('Ctrl Pts',(121.510716614322,-37.5443504602797,8.47626683430666));
#73055=CARTESIAN_POINT('Ctrl Pts',(121.517077828304,-37.533796113814,8.49410315611481));
#73056=CARTESIAN_POINT('Ctrl Pts',(121.541159186122,-37.4980708374905,8.54274436268672));
#73057=CARTESIAN_POINT('Ctrl Pts',(121.56412779323,-37.4686076043297,8.56856437653814));
#73058=CARTESIAN_POINT('Ctrl Pts',(121.617288389766,-37.4048701574215,8.60866399825098));
#73059=CARTESIAN_POINT('Ctrl Pts',(121.652509215907,-37.3653949038344,8.62308008690722));
#73060=CARTESIAN_POINT('Ctrl Pts',(121.726559498935,-37.2865621995426,8.63532117790982));
#73061=CARTESIAN_POINT('Ctrl Pts',(121.765406035132,-37.2472073755322,8.63305961883981));
#73062=CARTESIAN_POINT('Ctrl Pts',(121.804557793905,-37.2090666886064,8.62421947088418));
#73063=CARTESIAN_POINT('Ctrl Pts',(121.807962616873,-37.2057626944961,8.62339502798055));
#73064=CARTESIAN_POINT('Ctrl Pts',(121.811388687965,-37.2024514436577,8.62250778625268));
#73065=CARTESIAN_POINT('',(113.,-37.2024510141556,8.62250767116829));
#73066=CARTESIAN_POINT('Origin',(113.,-36.8001647010456,8.51471537844438));
#73067=CARTESIAN_POINT('',(121.912131484566,-37.1050842619827,8.59641832855393));
#73068=CARTESIAN_POINT('',(121.75,-37.261781781739,8.63840530242858));
#73069=CARTESIAN_POINT('Ctrl Pts',(122.,-36.9000603243714,8.54148233004194));
#73070=CARTESIAN_POINT('Ctrl Pts',(122.,-36.9358505645005,8.55107229598144));
#73071=CARTESIAN_POINT('Ctrl Pts',(121.991329280155,-36.9779743139833,8.56235932063753));
#73072=CARTESIAN_POINT('Ctrl Pts',(121.962987211232,-37.0440891771373,8.58007474482734));
#73073=CARTESIAN_POINT('Ctrl Pts',(121.938311286558,-37.0797823694469,8.58963870688199));
#73074=CARTESIAN_POINT('Ctrl Pts',(121.912131759621,-37.105084527511,8.59641839970201));
#73075=CARTESIAN_POINT('',(121.7,-35.5927574181843,8.19119157206623));
#73076=CARTESIAN_POINT('Origin',(121.7,-35.3029796702975,8.11354585853547));
#73077=CARTESIAN_POINT('',(103.5,-35.5927574181843,8.19119157206623));
#73078=CARTESIAN_POINT('Ctrl Pts',(104.624264068712,-38.0096419822012,3.69284665060534));
#73079=CARTESIAN_POINT('Ctrl Pts',(104.51617563888,-37.9023841393222,3.67872588770448));
#73080=CARTESIAN_POINT('Ctrl Pts',(104.408087612489,-37.7951258968034,3.66460507219005));
#73081=CARTESIAN_POINT('Ctrl Pts',(104.300000000005,-37.6878672442858,3.65048420269825));
#73082=CARTESIAN_POINT('Ctrl Pts',(104.567655925523,-38.0657165831672,3.70022901187374));
#73083=CARTESIAN_POINT('Ctrl Pts',(104.459564357694,-37.9584615504213,3.68610876488974));
#73084=CARTESIAN_POINT('Ctrl Pts',(104.351473262604,-37.8512061044813,3.67198802305844));
#73085=CARTESIAN_POINT('Ctrl Pts',(104.243382456865,-37.7439503091645,3.65786767826189));
#73086=CARTESIAN_POINT('Ctrl Pts',(104.45500004306,-38.1861491282932,3.6477858428286));
#73087=CARTESIAN_POINT('Ctrl Pts',(104.346902493405,-38.078900468474,3.6336586998587));
#73088=CARTESIAN_POINT('Ctrl Pts',(104.238805139007,-37.9716515954047,3.61953157877267));
#73089=CARTESIAN_POINT('Ctrl Pts',(104.13070824621,-37.8644022801433,3.60540421753159));
#73090=CARTESIAN_POINT('Ctrl Pts',(104.410455468831,-38.2513127544414,3.49378871788));
#73091=CARTESIAN_POINT('Ctrl Pts',(104.302362090343,-38.1440615207735,3.47964747605772));
#73092=CARTESIAN_POINT('Ctrl Pts',(104.194269413733,-38.0368096023995,3.46550601417655));
#73093=CARTESIAN_POINT('Ctrl Pts',(104.086176765826,-37.9295576652633,3.45136431096227));
#73094=CARTESIAN_POINT('Ctrl Pts',(104.412132034356,-38.2600922303079,3.41426858245338));
#73095=CARTESIAN_POINT('Ctrl Pts',(104.304043604524,-38.1528366240338,3.40012275628986));
#73096=CARTESIAN_POINT('Ctrl Pts',(104.195955578133,-38.0455806326541,3.38597666428458));
#73097=CARTESIAN_POINT('Ctrl Pts',(104.087867965649,-37.9383242460686,3.37183029953949));
#73098=CARTESIAN_POINT('',(104.300000000005,-37.6878672442858,3.65048420269825));
#73099=CARTESIAN_POINT('Origin',(104.300000000005,-37.7270251019518,3.35305074428611));
#73100=CARTESIAN_POINT('',(104.624264068712,-38.0096419822012,3.69284665060534));
#73101=CARTESIAN_POINT('Origin',(104.624264068712,-38.0487998398672,3.3954131921932));
#73102=CARTESIAN_POINT('Ctrl Pts',(104.624264068712,-38.0096419822012,3.69284665060534));
#73103=CARTESIAN_POINT('Ctrl Pts',(104.51617563888,-37.9023841393222,3.67872588770448));
#73104=CARTESIAN_POINT('Ctrl Pts',(104.408087612489,-37.7951258968034,3.66460507219005));
#73105=CARTESIAN_POINT('Ctrl Pts',(104.300000000005,-37.6878672442858,3.65048420269825));
#73106=CARTESIAN_POINT('Origin',(104.3,-0.24606831623661,-1.58141082851857));
#73107=CARTESIAN_POINT('Origin',(104.3,-37.7270251019467,3.35305074428542));
#73108=CARTESIAN_POINT('',(104.3,-36.3574214900301,3.47532769624594));
#73109=CARTESIAN_POINT('',(104.3,-0.206910458570595,-1.28397737010643));
#73110=CARTESIAN_POINT('Origin',(104.3,-36.099145889284,3.13873638016779));
#73111=CARTESIAN_POINT('Origin',(104.3,-37.7270251019467,3.35305074428542));
#73112=CARTESIAN_POINT('Origin',(104.624264068712,-38.0487998398672,3.39541319219319));
#73113=CARTESIAN_POINT('Origin',(104.624264068712,-38.0487998398672,3.39541319219319));
#73114=CARTESIAN_POINT('Origin',(113.,-37.75,1.3));
#73115=CARTESIAN_POINT('',(121.7,-36.5,1.3));
#73116=CARTESIAN_POINT('',(103.5,-36.5,1.3));
#73117=CARTESIAN_POINT('Origin',(121.7,-36.2,1.3));
#73118=CARTESIAN_POINT('',(121.912131484566,-38.0656759583793,1.3));
#73119=CARTESIAN_POINT('Ctrl Pts',(121.912131759621,-38.0656762332744,1.3));
#73120=CARTESIAN_POINT('Ctrl Pts',(121.938311286558,-38.0394815117177,1.3));
#73121=CARTESIAN_POINT('Ctrl Pts',(121.962987211232,-38.0025291999168,1.3));
#73122=CARTESIAN_POINT('Ctrl Pts',(121.991329280155,-37.9340820569223,1.3));
#73123=CARTESIAN_POINT('Ctrl Pts',(122.,-37.8904723424532,1.3));
#73124=CARTESIAN_POINT('Ctrl Pts',(122.,-37.8534195593564,1.3));
#73125=CARTESIAN_POINT('',(121.75,-38.2279011681123,1.3));
#73126=CARTESIAN_POINT('Origin',(113.,-37.6311160247631,-6.56803674858937));
#73127=CARTESIAN_POINT('',(121.811388243054,-37.6702738824291,-6.27060329017722));
#73128=CARTESIAN_POINT('Ctrl Pts',(121.5,-37.9266483495649,-6.61961818902332));
#73129=CARTESIAN_POINT('Ctrl Pts',(121.5,-37.9302235600485,-6.59913426579449));
#73130=CARTESIAN_POINT('Ctrl Pts',(121.502178291748,-37.9316657356349,-6.57810179894056));
#73131=CARTESIAN_POINT('Ctrl Pts',(121.510716614322,-37.930183837478,-6.53655145973753));
#73132=CARTESIAN_POINT('Ctrl Pts',(121.517077828304,-37.9272585576496,-6.51603387355179));
#73133=CARTESIAN_POINT('Ctrl Pts',(121.541159186122,-37.9128668899463,-6.4574237869977));
#73134=CARTESIAN_POINT('Ctrl Pts',(121.56412779323,-37.8955273033918,-6.42229411347666));
#73135=CARTESIAN_POINT('Ctrl Pts',(121.617288389766,-37.8519870416124,-6.36085562876169));
#73136=CARTESIAN_POINT('Ctrl Pts',(121.652509215907,-37.8210334610709,-6.33243037397715));
#73137=CARTESIAN_POINT('Ctrl Pts',(121.726559498935,-37.7528860018039,-6.29095311068322));
#73138=CARTESIAN_POINT('Ctrl Pts',(121.765406035132,-37.7156614242077,-6.27798207968714));
#73139=CARTESIAN_POINT('Ctrl Pts',(121.804557793905,-37.6770410460388,-6.27155350246219));
#73140=CARTESIAN_POINT('Ctrl Pts',(121.807962616873,-37.6736730528646,-6.27105080457995));
#73141=CARTESIAN_POINT('Ctrl Pts',(121.811388687965,-37.6702743232782,-6.27060334821644));
#73142=CARTESIAN_POINT('',(113.,-37.6702738824291,-6.27060329017722));
#73143=CARTESIAN_POINT('Origin',(113.,-37.2573594669753,-6.21624207609289));
#73144=CARTESIAN_POINT('',(121.912131484566,-37.5703347737697,-6.25744605691555));
#73145=CARTESIAN_POINT('',(121.75,-37.7311721243448,-6.2786206958241));
#73146=CARTESIAN_POINT('Ctrl Pts',(122.,-37.3598942576648,-6.22974103737676));
#73147=CARTESIAN_POINT('Ctrl Pts',(122.,-37.3966300490657,-6.23457739606554));
#73148=CARTESIAN_POINT('Ctrl Pts',(121.991329280155,-37.4398666763821,-6.240269606039));
#73149=CARTESIAN_POINT('Ctrl Pts',(121.962987211232,-37.5077282445796,-6.2492037509824));
#73150=CARTESIAN_POINT('Ctrl Pts',(121.938311286558,-37.5443644242305,-6.25402699553551));
#73151=CARTESIAN_POINT('Ctrl Pts',(121.912131759621,-37.570335046313,-6.25744609279656));
#73152=CARTESIAN_POINT('',(121.7,-36.018053390258,-6.05308433581783));
#73153=CARTESIAN_POINT('Origin',(121.7,-35.7206199318459,-6.01392647815181));
#73154=CARTESIAN_POINT('',(103.5,-36.018053390258,-6.05308433581783));
#73155=CARTESIAN_POINT('Origin',(113.,-36.4518757833583,-11.4236925674066));
#73156=CARTESIAN_POINT('',(121.811388243054,-36.529521496889,-11.1339148195198));
#73157=CARTESIAN_POINT('Ctrl Pts',(121.5,-36.7381470591438,-11.5134074305014));
#73158=CARTESIAN_POINT('Ctrl Pts',(121.5,-36.7443653717069,-11.4935654086862));
#73159=CARTESIAN_POINT('Ctrl Pts',(121.502178291748,-36.7485404970926,-11.4729011191897));
#73160=CARTESIAN_POINT('Ctrl Pts',(121.510716614322,-36.7524946843416,-11.4315128223748));
#73161=CARTESIAN_POINT('Ctrl Pts',(121.517077828304,-36.7522725130859,-11.410788941346));
#73162=CARTESIAN_POINT('Ctrl Pts',(121.541159186122,-36.7456541195186,-11.3508017826222));
#73163=CARTESIAN_POINT('Ctrl Pts',(121.56412779323,-36.7330482180494,-11.3137093781204));
#73164=CARTESIAN_POINT('Ctrl Pts',(121.617288389766,-36.6978997807109,-11.2471133635808));
#73165=CARTESIAN_POINT('Ctrl Pts',(121.652509215907,-36.6709212526118,-11.2148910377878));
#73166=CARTESIAN_POINT('Ctrl Pts',(121.726559498935,-36.6087706735474,-11.1648735898636));
#73167=CARTESIAN_POINT('Ctrl Pts',(121.765406035132,-36.5735576166579,-11.1471547454652));
#73168=CARTESIAN_POINT('Ctrl Pts',(121.804557793905,-36.5361067388845,-11.1357401947051));
#73169=CARTESIAN_POINT('Ctrl Pts',(121.807962616873,-36.5328331745993,-11.1348021861485));
#73170=CARTESIAN_POINT('Ctrl Pts',(121.811388687965,-36.5295219263909,-11.1339149346049));
#73171=CARTESIAN_POINT('',(113.,-36.529521496889,-11.1339148195198));
#73172=CARTESIAN_POINT('Origin',(113.,-36.1272351837791,-11.0261225267959));
#73173=CARTESIAN_POINT('',(121.912131484566,-36.4321547447161,-11.1078254769055));
#73174=CARTESIAN_POINT('',(121.75,-36.5888522644724,-11.1498124507801));
#73175=CARTESIAN_POINT('Ctrl Pts',(122.,-36.2271308071049,-11.0528894783935));
#73176=CARTESIAN_POINT('Ctrl Pts',(122.,-36.262921047234,-11.062479444333));
#73177=CARTESIAN_POINT('Ctrl Pts',(121.991329280155,-36.3050447967168,-11.0737664689891));
#73178=CARTESIAN_POINT('Ctrl Pts',(121.962987211232,-36.3711596598708,-11.0914818931789));
#73179=CARTESIAN_POINT('Ctrl Pts',(121.938311286558,-36.4068528521804,-11.1010458552335));
#73180=CARTESIAN_POINT('Ctrl Pts',(121.912131759621,-36.4321550102444,-11.1078255480536));
#73181=CARTESIAN_POINT('',(121.7,-34.9198279009177,-10.7025987204178));
#73182=CARTESIAN_POINT('Origin',(121.7,-34.630050153031,-10.624953006887));
#73183=CARTESIAN_POINT('',(103.5,-34.9198279009177,-10.7025987204178));
#73184=CARTESIAN_POINT('Ctrl Pts',(121.375735931288,-33.7031390339859,-17.9574056939141));
#73185=CARTESIAN_POINT('Ctrl Pts',(121.483824361121,-33.6094494902625,-17.9033140106251));
#73186=CARTESIAN_POINT('Ctrl Pts',(121.591912387512,-33.5157595974544,-17.8492221257921));
#73187=CARTESIAN_POINT('Ctrl Pts',(121.699999999997,-33.4220693465132,-17.7951300341907));
#73188=CARTESIAN_POINT('Ctrl Pts',(121.432344074477,-33.752120102763,-17.9856849271578));
#73189=CARTESIAN_POINT('Ctrl Pts',(121.540435642307,-33.6584329578312,-17.9315947959052));
#73190=CARTESIAN_POINT('Ctrl Pts',(121.648526737398,-33.5647456205277,-17.8775040493508));
#73191=CARTESIAN_POINT('Ctrl Pts',(121.756617543138,-33.4710578085036,-17.823413535908));
#73192=CARTESIAN_POINT('Ctrl Pts',(121.544996182435,-33.8834537221696,-17.9833149249053));
#73193=CARTESIAN_POINT('Ctrl Pts',(121.653093732091,-33.7897751040339,-17.929220861406));
#73194=CARTESIAN_POINT('Ctrl Pts',(121.761191083735,-33.6960962793851,-17.8751267330704));
#73195=CARTESIAN_POINT('Ctrl Pts',(121.869287976533,-33.6024171392287,-17.8210322170879));
#73196=CARTESIAN_POINT('Ctrl Pts',(121.589544531169,-34.0025898869996,-17.8659835447083));
#73197=CARTESIAN_POINT('Ctrl Pts',(121.697637909658,-33.908914286335,-17.8118754705986));
#73198=CARTESIAN_POINT('Ctrl Pts',(121.805730586268,-33.8152381372974,-17.7577669311553));
#73199=CARTESIAN_POINT('Ctrl Pts',(121.913823234176,-33.72156206328,-17.7036581615694));
#73200=CARTESIAN_POINT('Ctrl Pts',(121.587867965644,-34.0411321034261,-17.7958762791241));
#73201=CARTESIAN_POINT('Ctrl Pts',(121.695956395477,-33.9474542173515,-17.7417622963114));
#73202=CARTESIAN_POINT('Ctrl Pts',(121.804044421868,-33.8537760772191,-17.6876479205194));
#73203=CARTESIAN_POINT('Ctrl Pts',(121.912132034353,-33.7600976763372,-17.63353314151));
#73204=CARTESIAN_POINT('',(121.699999999997,-33.4220693465132,-17.7951300341907));
#73205=CARTESIAN_POINT('Origin',(121.699999999997,-33.5720693465132,-17.5353224130553));
#73206=CARTESIAN_POINT('',(121.375735931288,-33.7031390339859,-17.9574056939141));
#73207=CARTESIAN_POINT('Origin',(121.375735931288,-33.8531390339859,-17.6975980727788));
#73208=CARTESIAN_POINT('Ctrl Pts',(121.375735931288,-33.7031390339859,-17.9574056939141));
#73209=CARTESIAN_POINT('Ctrl Pts',(121.483824361121,-33.6094494902625,-17.9033140106251));
#73210=CARTESIAN_POINT('Ctrl Pts',(121.591912387512,-33.5157595974544,-17.8492221257921));
#73211=CARTESIAN_POINT('Ctrl Pts',(121.699999999997,-33.4220693465132,-17.7951300341907));
#73212=CARTESIAN_POINT('Origin',(121.375735931288,0.,0.));
#73213=CARTESIAN_POINT('',(121.375735931288,-34.1190013824203,-17.8365844450781));
#73214=CARTESIAN_POINT('Origin',(121.375735931288,0.,0.));
#73215=CARTESIAN_POINT('Origin',(121.375735931288,-33.8531390339859,-17.6975980727788));
#73216=CARTESIAN_POINT('Origin',(121.375735931288,-33.8531390339859,-17.6975980727788));
#73217=CARTESIAN_POINT('Origin',(121.375735931288,-33.8531390339859,-17.6975980727788));
#73218=CARTESIAN_POINT('Origin',(121.7,-4.77122949643128,-0.907149772723275));
#73219=CARTESIAN_POINT('Origin',(121.7,-33.5720693465106,-17.5353224130539));
#73220=CARTESIAN_POINT('',(121.7,-32.259927238132,-17.1241669750802));
#73221=CARTESIAN_POINT('',(121.7,-4.62122949643128,-1.16695739385861));
#73222=CARTESIAN_POINT('Origin',(121.7,-32.1501196169967,-16.7143593539449));
#73223=CARTESIAN_POINT('Origin',(121.7,-33.5720693465106,-17.535322413054));
#73224=CARTESIAN_POINT('Origin',(113.,-34.3789638902265,-15.6473429640468));
#73225=CARTESIAN_POINT('',(104.3,-33.2241144745874,-15.1689886735904));
#73226=CARTESIAN_POINT('',(103.5,-33.2241144745874,-15.1689886735904));
#73227=CARTESIAN_POINT('Origin',(104.3,-32.946950614834,-15.0541836438809));
#73228=CARTESIAN_POINT('',(104.087868515434,-34.670610447079,-15.7681469233145));
#73229=CARTESIAN_POINT('Ctrl Pts',(104.087868240379,-34.6706107010489,-15.7681470285123));
#73230=CARTESIAN_POINT('Ctrl Pts',(104.061688713442,-34.6464099339429,-15.7581227425572));
#73231=CARTESIAN_POINT('Ctrl Pts',(104.037012788768,-34.612270449391,-15.7439817050433));
#73232=CARTESIAN_POINT('Ctrl Pts',(104.008670719845,-34.5490335349196,-15.7177881174266));
#73233=CARTESIAN_POINT('Ctrl Pts',(104.,-34.5087434123029,-15.7010994022091));
#73234=CARTESIAN_POINT('Ctrl Pts',(104.,-34.4745111043772,-15.686919915995));
#73235=CARTESIAN_POINT('',(104.25,-34.8204869980086,-15.8302278233913));
#73236=CARTESIAN_POINT('Ctrl Pts',(104.624264068712,-32.4031390339859,-20.2090717437536));
#73237=CARTESIAN_POINT('Ctrl Pts',(104.516175638879,-32.3094494902625,-20.1549800604647));
#73238=CARTESIAN_POINT('Ctrl Pts',(104.408087612488,-32.2157595974544,-20.1008881756316));
#73239=CARTESIAN_POINT('Ctrl Pts',(104.300000000003,-32.1220693465132,-20.0467960840302));
#73240=CARTESIAN_POINT('Ctrl Pts',(104.567655925523,-32.452120102763,-20.2373509769973));
#73241=CARTESIAN_POINT('Ctrl Pts',(104.459564357693,-32.3584331025383,-20.1832605951046));
#73242=CARTESIAN_POINT('Ctrl Pts',(104.351473262602,-32.2647454732609,-20.1291703542641));
#73243=CARTESIAN_POINT('Ctrl Pts',(104.243382456862,-32.1710578085036,-20.0750795857476));
#73244=CARTESIAN_POINT('Ctrl Pts',(104.455001730448,-32.5157376683244,-20.352272791064));
#73245=CARTESIAN_POINT('Ctrl Pts',(104.346904180792,-32.4220515260722,-20.2981917597167));
#73246=CARTESIAN_POINT('Ctrl Pts',(104.238806827625,-32.3283652263742,-20.2441105815259));
#73247=CARTESIAN_POINT('Ctrl Pts',(104.130709934827,-32.2346784312498,-20.1900293243369));
#73248=CARTESIAN_POINT('Ctrl Pts',(104.410455468831,-32.473690556812,-20.5141148642513));
#73249=CARTESIAN_POINT('Ctrl Pts',(104.302362090342,-32.3799937897508,-20.4600434514159));
#73250=CARTESIAN_POINT('Ctrl Pts',(104.194269413732,-32.2862963455125,-20.4059717963423));
#73251=CARTESIAN_POINT('Ctrl Pts',(104.086176765824,-32.1925987394748,-20.3519003213094));
#73252=CARTESIAN_POINT('Ctrl Pts',(104.412132034356,-32.4322469920394,-20.5825470355869));
#73253=CARTESIAN_POINT('Ctrl Pts',(104.304043604523,-32.3385439651864,-20.5284765978799));
#73254=CARTESIAN_POINT('Ctrl Pts',(104.195955578132,-32.2448404709744,-20.4744061366419));
#73255=CARTESIAN_POINT('Ctrl Pts',(104.087867965647,-32.1511364971911,-20.4203356511969));
#73256=CARTESIAN_POINT('',(104.300000000003,-32.1220693465132,-20.0467960840302));
#73257=CARTESIAN_POINT('Origin',(104.300000000003,-31.9720693465132,-20.3066037051655));
#73258=CARTESIAN_POINT('',(104.624264068712,-32.4031390339859,-20.2090717437536));
#73259=CARTESIAN_POINT('Origin',(104.624264068712,-32.2531390339859,-20.468879364889));
#73260=CARTESIAN_POINT('Ctrl Pts',(104.624264068712,-32.4031390339859,-20.2090717437536));
#73261=CARTESIAN_POINT('Ctrl Pts',(104.516175638879,-32.3094494902625,-20.1549800604647));
#73262=CARTESIAN_POINT('Ctrl Pts',(104.408087612488,-32.2157595974544,-20.1008881756316));
#73263=CARTESIAN_POINT('Ctrl Pts',(104.300000000003,-32.1220693465132,-20.0467960840302));
#73264=CARTESIAN_POINT('Origin',(104.3,-1.29622949643128,-2.59589931010293));
#73265=CARTESIAN_POINT('Origin',(104.3,-31.9720693465106,-20.3066037051641));
#73266=CARTESIAN_POINT('',(104.3,-30.959927238132,-19.3758330249198));
#73267=CARTESIAN_POINT('',(104.3,-1.44622949643128,-2.3360916889676));
#73268=CARTESIAN_POINT('Origin',(104.3,-30.5501196169967,-19.4856406460551));
#73269=CARTESIAN_POINT('Origin',(104.3,-31.9720693465106,-20.3066037051641));
#73270=CARTESIAN_POINT('Origin',(104.624264068712,-32.2531390339859,-20.468879364889));
#73271=CARTESIAN_POINT('Origin',(104.624264068712,-32.2531390339859,-20.468879364889));
#73272=CARTESIAN_POINT('Origin',(113.,-30.7404784537055,-21.9493846027006));
#73273=CARTESIAN_POINT('',(121.7,-29.7487867783414,-21.1884328164397));
#73274=CARTESIAN_POINT('',(103.5,-29.7487867783414,-21.1884328164397));
#73275=CARTESIAN_POINT('Origin',(121.7,-29.5107807762541,-21.0058043877371));
#73276=CARTESIAN_POINT('',(121.912131484566,-30.9909210297353,-22.1415559502272));
#73277=CARTESIAN_POINT('Ctrl Pts',(121.912131759621,-30.9909212478243,-22.1415561175728));
#73278=CARTESIAN_POINT('Ctrl Pts',(121.938311286558,-30.9701395779793,-22.1256097814455));
#73279=CARTESIAN_POINT('Ctrl Pts',(121.962987211232,-30.9408233379805,-22.1031146393084));
#73280=CARTESIAN_POINT('Ctrl Pts',(121.991329280155,-30.8865205684525,-22.0614466587275));
#73281=CARTESIAN_POINT('Ctrl Pts',(122.,-30.8519226558093,-22.0348987466286));
#73282=CARTESIAN_POINT('Ctrl Pts',(122.,-30.8225267065724,-22.0123424414419));
#73283=CARTESIAN_POINT('',(121.75,-31.1196229417564,-22.2403124007256));
#73284=CARTESIAN_POINT('Origin',(104.3,-3.72628900609773,-16.0458989224046));
#73285=CARTESIAN_POINT('',(104.3,-6.22824084226949,-37.3484991445085));
#73286=CARTESIAN_POINT('Origin',(104.3,-6.52567430068164,-37.3093412868425));
#73287=CARTESIAN_POINT('',(104.3,-6.05308433581787,-36.018053390258));
#73288=CARTESIAN_POINT('Origin',(104.3,-6.311359936564,-35.6814620741798));
#73289=CARTESIAN_POINT('',(104.3,-3.42885554768559,-16.0850567800706));
#73290=CARTESIAN_POINT('Ctrl Pts',(104.300000000005,-6.22824084227015,-37.3484991445135));
#73291=CARTESIAN_POINT('Ctrl Pts',(104.408087612491,-6.24236171176216,-37.4557577970327));
#73292=CARTESIAN_POINT('Ctrl Pts',(104.516175638883,-6.2564825272768,-37.5630160395531));
#73293=CARTESIAN_POINT('Ctrl Pts',(104.624264068717,-6.27060329017788,-37.6702738824337));
#73294=CARTESIAN_POINT('Ctrl Pts',(104.243382456865,-6.23562431783379,-37.4045822093922));
#73295=CARTESIAN_POINT('Ctrl Pts',(104.351473262605,-6.24974495464451,-37.5118379662662));
#73296=CARTESIAN_POINT('Ctrl Pts',(104.459564357697,-6.26386511752374,-37.6190934884283));
#73297=CARTESIAN_POINT('Ctrl Pts',(104.567655925527,-6.27798565144628,-37.7263484833998));
#73298=CARTESIAN_POINT('Ctrl Pts',(104.130708651008,-6.31747589142949,-37.5073508627116));
#73299=CARTESIAN_POINT('Ctrl Pts',(104.238805543807,-6.33158807371347,-37.6146021763222));
#73300=CARTESIAN_POINT('Ctrl Pts',(104.346902897911,-6.34570037330177,-37.7218530009716));
#73301=CARTESIAN_POINT('Ctrl Pts',(104.455000447568,-6.35981259677861,-37.829103624981));
#73302=CARTESIAN_POINT('Ctrl Pts',(104.086176765826,-6.48312997219364,-37.5304181438623));
#73303=CARTESIAN_POINT('Ctrl Pts',(104.194269413735,-6.49722897978645,-37.6376757019853));
#73304=CARTESIAN_POINT('Ctrl Pts',(104.302362090346,-6.51132821563312,-37.7449331795238));
#73305=CARTESIAN_POINT('Ctrl Pts',(104.410455468835,-6.52542748682539,-37.8521899387317));
#73306=CARTESIAN_POINT('Ctrl Pts',(104.087867965649,-6.56222288596812,-37.5183010937808));
#73307=CARTESIAN_POINT('Ctrl Pts',(104.195955578135,-6.57631854247014,-37.6255641562347));
#73308=CARTESIAN_POINT('Ctrl Pts',(104.304043604527,-6.59041436013181,-37.732826766359));
#73309=CARTESIAN_POINT('Ctrl Pts',(104.412132034361,-6.60451033490424,-37.8400889356949));
#73310=CARTESIAN_POINT('',(104.624264068717,-6.27060329017788,-37.6702738824337));
#73311=CARTESIAN_POINT('',(104.412132034361,-6.60451033490383,-37.8400889356926));
#73312=CARTESIAN_POINT('Origin',(104.624264068717,-6.56803674859002,-37.6311160247677));
#73313=CARTESIAN_POINT('',(104.087867965649,-6.56222288596768,-37.5183010937783));
#73314=CARTESIAN_POINT('Ctrl Pts',(104.412132034361,-6.60451033490424,-37.8400889356949));
#73315=CARTESIAN_POINT('Ctrl Pts',(104.304043604527,-6.59041436013181,-37.732826766359));
#73316=CARTESIAN_POINT('Ctrl Pts',(104.195955578135,-6.57631854247014,-37.6255641562347));
#73317=CARTESIAN_POINT('Ctrl Pts',(104.087867965649,-6.56222288596812,-37.5183010937808));
#73318=CARTESIAN_POINT('Origin',(104.300000000005,-6.5256743006823,-37.3093412868475));
#73319=CARTESIAN_POINT('Ctrl Pts',(104.300000000005,-6.22824084227015,-37.3484991445135));
#73320=CARTESIAN_POINT('Ctrl Pts',(104.408087612491,-6.24236171176216,-37.4557577970327));
#73321=CARTESIAN_POINT('Ctrl Pts',(104.516175638883,-6.2564825272768,-37.5630160395531));
#73322=CARTESIAN_POINT('Ctrl Pts',(104.624264068717,-6.27060329017788,-37.6702738824337));
#73323=CARTESIAN_POINT('Origin',(104.3,-6.52567430068164,-37.3093412868425));
#73324=CARTESIAN_POINT('Origin',(104.3,-6.52567430068164,-37.3093412868425));
#73325=CARTESIAN_POINT('Origin',(113.,-6.56803674858941,-37.6311160247631));
#73326=CARTESIAN_POINT('',(121.811388243054,-6.27060329017727,-37.6702738824291));
#73327=CARTESIAN_POINT('',(121.5,-6.61961818902336,-37.9266483495649));
#73328=CARTESIAN_POINT('Ctrl Pts',(121.811388687965,-6.27060334821648,-37.6702743232782));
#73329=CARTESIAN_POINT('Ctrl Pts',(121.80796264376,-6.27105080106853,-37.6736730261927));
#73330=CARTESIAN_POINT('Ctrl Pts',(121.80455782351,-6.27155349760124,-37.6770410168358));
#73331=CARTESIAN_POINT('Ctrl Pts',(121.765406035132,-6.27798207968718,-37.7156614242077));
#73332=CARTESIAN_POINT('Ctrl Pts',(121.726559498935,-6.29095311068325,-37.7528860018039));
#73333=CARTESIAN_POINT('Ctrl Pts',(121.652509215907,-6.33243037397719,-37.8210334610709));
#73334=CARTESIAN_POINT('Ctrl Pts',(121.617288389766,-6.36085562876173,-37.8519870416124));
#73335=CARTESIAN_POINT('Ctrl Pts',(121.56412779323,-6.42229411347671,-37.8955273033918));
#73336=CARTESIAN_POINT('Ctrl Pts',(121.541159186122,-6.45742378699774,-37.9128668899463));
#73337=CARTESIAN_POINT('Ctrl Pts',(121.517077828304,-6.51603387355183,-37.9272585576495));
#73338=CARTESIAN_POINT('Ctrl Pts',(121.510716614322,-6.53655145973757,-37.930183837478));
#73339=CARTESIAN_POINT('Ctrl Pts',(121.502178291748,-6.5781017989406,-37.9316657356349));
#73340=CARTESIAN_POINT('Ctrl Pts',(121.5,-6.59913426579454,-37.9302235600485));
#73341=CARTESIAN_POINT('Ctrl Pts',(121.5,-6.61961818902336,-37.9266483495649));
#73342=CARTESIAN_POINT('',(104.624264068712,-6.61961818902336,-37.9266483495649));
#73343=CARTESIAN_POINT('',(113.,-6.61961818902336,-37.9266483495649));
#73344=CARTESIAN_POINT('Origin',(104.624264068712,-6.56803674858941,-37.6311160247631));
#73345=CARTESIAN_POINT('',(113.,-6.27060329017727,-37.6702738824291));
#73346=CARTESIAN_POINT('Origin',(104.624264068712,-6.56803674858922,-37.6311160247631));
#73347=CARTESIAN_POINT('Origin',(104.624264068712,-6.56803674858922,-37.6311160247631));
#73348=CARTESIAN_POINT('Origin',(104.3,0.,0.));
#73349=CARTESIAN_POINT('',(104.087867965648,-8.29492882695121,-37.173644453084));
#73350=CARTESIAN_POINT('Origin',(104.087867965644,2.22044604925031E-15,
0.));
#73351=CARTESIAN_POINT('Origin',(104.3,-8.24872986069483,-36.9666042262736));
#73352=CARTESIAN_POINT('Origin',(104.25,0.,0.));
#73353=CARTESIAN_POINT('',(104.412132034356,-8.37900319423353,-37.4871203601426));
#73354=CARTESIAN_POINT('Origin',(104.412132034356,2.22044604925031E-15,
0.));
#73355=CARTESIAN_POINT('Ctrl Pts',(104.087867965648,-8.29492882695166,-37.173644453086));
#73356=CARTESIAN_POINT('Ctrl Pts',(104.195955578133,-8.32295393531767,-37.2781367752921));
#73357=CARTESIAN_POINT('Ctrl Pts',(104.304043604523,-8.35097872169251,-37.3826287412732));
#73358=CARTESIAN_POINT('Ctrl Pts',(104.412132034356,-8.37900319423354,-37.4871203601426));
#73359=CARTESIAN_POINT('Origin',(104.624264068712,0.,0.));
#73360=CARTESIAN_POINT('',(104.624264068712,-8.3981702106372,-37.5728723564378));
#73361=CARTESIAN_POINT('Origin',(104.624264068712,0.,0.));
#73362=CARTESIAN_POINT('Origin',(104.624264068712,-8.33272992328159,-37.2800967276863));
#73363=CARTESIAN_POINT('Origin',(113.,0.,0.));
#73364=CARTESIAN_POINT('',(121.5,-8.3981702106372,-37.5728723564378));
#73365=CARTESIAN_POINT('Origin',(121.5,0.,0.));
#73366=CARTESIAN_POINT('',(113.,-8.3981702106372,-37.5728723564378));
#73367=CARTESIAN_POINT('Ctrl Pts',(104.624264068712,-29.4881125046124,-24.2656386875623));
#73368=CARTESIAN_POINT('Ctrl Pts',(104.516175638879,-29.4022848693738,-24.1997808267293));
#73369=CARTESIAN_POINT('Ctrl Pts',(104.408087612488,-29.3164569143438,-24.1339227205117));
#73370=CARTESIAN_POINT('Ctrl Pts',(104.300000000003,-29.2306286312331,-24.068064362549));
#73371=CARTESIAN_POINT('Ctrl Pts',(104.567655925523,-29.5329833529219,-24.3000693004437));
#73372=CARTESIAN_POINT('Ctrl Pts',(104.459564357693,-29.4471580695557,-24.2342130618665));
#73373=CARTESIAN_POINT('Ctrl Pts',(104.351473262602,-29.3613321441074,-24.1683568810269));
#73374=CARTESIAN_POINT('Ctrl Pts',(104.243382456862,-29.2755062523583,-24.1025001723946));
#73375=CARTESIAN_POINT('Ctrl Pts',(104.455001885058,-29.5810561028804,-24.4223117753432));
#73376=CARTESIAN_POINT('Ctrl Pts',(104.346904335402,-29.4952304496556,-24.3564649193042));
#73377=CARTESIAN_POINT('Ctrl Pts',(104.238806982348,-29.4094046593508,-24.2906178971386));
#73378=CARTESIAN_POINT('Ctrl Pts',(104.130710089549,-29.3235783883173,-24.224770731973));
#73379=CARTESIAN_POINT('Ctrl Pts',(104.410455468831,-29.518244332399,-24.577280943507));
#73380=CARTESIAN_POINT('Ctrl Pts',(104.302362090342,-29.4324068897941,-24.5114422368762));
#73381=CARTESIAN_POINT('Ctrl Pts',(104.194269413731,-29.3465688074239,-24.4456032016902));
#73382=CARTESIAN_POINT('Ctrl Pts',(104.086176765824,-29.2607305411385,-24.3797643238856));
#73383=CARTESIAN_POINT('Ctrl Pts',(104.412132034356,-29.4682231323184,-24.6397181974285));
#73384=CARTESIAN_POINT('Ctrl Pts',(104.304043604523,-29.3823793561953,-24.5738796405169));
#73385=CARTESIAN_POINT('Ctrl Pts',(104.195955578132,-29.2965351197829,-24.5080409992732));
#73386=CARTESIAN_POINT('Ctrl Pts',(104.087867965647,-29.2106904110617,-24.4422022714329));
#73387=CARTESIAN_POINT('',(104.300000000003,-29.2306286312331,-24.068064362549));
#73388=CARTESIAN_POINT('Origin',(104.300000000003,-29.0480002025304,-24.3060703646363));
#73389=CARTESIAN_POINT('',(104.624264068712,-29.4881125046124,-24.2656386875623));
#73390=CARTESIAN_POINT('Origin',(104.624264068712,-29.3054840759098,-24.5036446896497));
#73391=CARTESIAN_POINT('Ctrl Pts',(104.624264068712,-29.4881125046124,-24.2656386875623));
#73392=CARTESIAN_POINT('Ctrl Pts',(104.516175638879,-29.4022848693738,-24.1997808267293));
#73393=CARTESIAN_POINT('Ctrl Pts',(104.408087612488,-29.3164569143438,-24.1339227205117));
#73394=CARTESIAN_POINT('Ctrl Pts',(104.300000000003,-29.2306286312331,-24.068064362549));
#73395=CARTESIAN_POINT('Origin',(104.3,-2.04174508310916,-3.58344196725942));
#73396=CARTESIAN_POINT('Origin',(104.3,-29.0480002025284,-24.3060703646347));
#73397=CARTESIAN_POINT('',(104.3,-28.1660070629188,-23.2511515011969));
#73398=CARTESIAN_POINT('',(104.3,-2.22437351181178,-3.34543596517205));
#73399=CARTESIAN_POINT('Origin',(104.3,-27.7453726321288,-23.3065290745816));
#73400=CARTESIAN_POINT('Origin',(104.3,-29.0480002025284,-24.3060703646347));
#73401=CARTESIAN_POINT('Origin',(104.624264068712,-29.3054840759098,-24.5036446896497));
#73402=CARTESIAN_POINT('Origin',(104.624264068712,-29.3054840759098,-24.5036446896497));
#73403=CARTESIAN_POINT('Origin',(113.,-29.3054840759098,-24.5036446896497));
#73404=CARTESIAN_POINT('',(121.811388243054,-29.4881125046124,-24.2656386875623));
#73405=CARTESIAN_POINT('Ctrl Pts',(121.5,-29.5356318566107,-24.6960816898302));
#73406=CARTESIAN_POINT('Ctrl Pts',(121.5,-29.5489700413278,-24.6801296971866));
#73407=CARTESIAN_POINT('Ctrl Pts',(121.502178291748,-29.5607352354493,-24.6626361343801));
#73408=CARTESIAN_POINT('Ctrl Pts',(121.510716614322,-29.5802270436011,-24.625911536016));
#73409=CARTESIAN_POINT('Ctrl Pts',(121.517077828304,-29.5879524700494,-24.6066801452405));
#73410=CARTESIAN_POINT('Ctrl Pts',(121.541159186122,-29.6047939634926,-24.5487264875151));
#73411=CARTESIAN_POINT('Ctrl Pts',(121.56412779323,-29.6073422778058,-24.509633504542));
#73412=CARTESIAN_POINT('Ctrl Pts',(121.617288389766,-29.6003545473749,-24.434656085119));
#73413=CARTESIAN_POINT('Ctrl Pts',(121.652509215907,-29.5877605876801,-24.3945623020958));
#73414=CARTESIAN_POINT('Ctrl Pts',(121.726559498935,-29.5494817883985,-24.3245682087703));
#73415=CARTESIAN_POINT('Ctrl Pts',(121.765406035132,-29.5237298740531,-24.2947226776164));
#73416=CARTESIAN_POINT('Ctrl Pts',(121.804557793905,-29.4934979340675,-24.2698451773449));
#73417=CARTESIAN_POINT('Ctrl Pts',(121.807962616873,-29.49083251536,-24.2677258316214));
#73418=CARTESIAN_POINT('Ctrl Pts',(121.811388687965,-29.4881128573793,-24.2656389582503));
#73419=CARTESIAN_POINT('',(113.,-29.4881125046124,-24.2656386875623));
#73420=CARTESIAN_POINT('Origin',(113.,-29.1576987382828,-24.0121032874578));
#73421=CARTESIAN_POINT('',(121.912131484566,-29.4081413143126,-24.2042746349845));
#73422=CARTESIAN_POINT('',(121.75,-29.5368432263338,-24.3030310854828));
#73423=CARTESIAN_POINT('Ctrl Pts',(122.,-29.2397469911497,-24.0750611261991));
#73424=CARTESIAN_POINT('Ctrl Pts',(122.,-29.2691429403866,-24.0976174313858));
#73425=CARTESIAN_POINT('Ctrl Pts',(121.991329280155,-29.3037408530298,-24.1241653434847));
#73426=CARTESIAN_POINT('Ctrl Pts',(121.962987211232,-29.3580436225579,-24.1658333240656));
#73427=CARTESIAN_POINT('Ctrl Pts',(121.938311286558,-29.3873598625566,-24.1883284662027));
#73428=CARTESIAN_POINT('Ctrl Pts',(121.912131759621,-29.4081415324016,-24.20427480233));
#73429=CARTESIAN_POINT('',(121.7,-28.1660070629188,-23.2511515011969));
#73430=CARTESIAN_POINT('Origin',(121.7,-27.9280010608314,-23.0685230724943));
#73431=CARTESIAN_POINT('',(103.5,-28.1660070629188,-23.2511515011969));
#73432=CARTESIAN_POINT('Origin',(104.3,4.61248681829539,-23.3959604433702));
#73433=CARTESIAN_POINT('',(104.3,8.5385076085815,-36.8889585127428));
#73434=CARTESIAN_POINT('Origin',(104.3,8.24872986069478,-36.9666042262736));
#73435=CARTESIAN_POINT('',(104.3,8.1911915720662,-35.5927574181843));
#73436=CARTESIAN_POINT('Origin',(104.3,7.82376811064873,-35.3806253838283));
#73437=CARTESIAN_POINT('',(104.3,4.90226456618211,-23.3183147298394));
#73438=CARTESIAN_POINT('Ctrl Pts',(104.300000000004,8.53850760858253,-36.8889585127467));
#73439=CARTESIAN_POINT('Ctrl Pts',(104.40808761249,8.5665077355745,-36.9934564092991));
#73440=CARTESIAN_POINT('Ctrl Pts',(104.516175638882,8.59450775553531,-37.0979539064057));
#73441=CARTESIAN_POINT('Ctrl Pts',(104.624264068716,8.62250767116921,-37.2024510141591));
#73442=CARTESIAN_POINT('Ctrl Pts',(104.243382456863,8.55314822639582,-36.9435980422801));
#73443=CARTESIAN_POINT('Ctrl Pts',(104.351473262604,8.58114746024185,-37.0480931745619));
#73444=CARTESIAN_POINT('Ctrl Pts',(104.459564357696,8.60914704212311,-37.1525879086325));
#73445=CARTESIAN_POINT('Ctrl Pts',(104.567655925526,8.63714607945793,-37.2570822976345));
#73446=CARTESIAN_POINT('Ctrl Pts',(104.130708900332,8.51685469895554,-37.0698669867126));
#73447=CARTESIAN_POINT('Ctrl Pts',(104.238805793131,8.54486004340248,-37.174354778547));
#73448=CARTESIAN_POINT('Ctrl Pts',(104.346903147053,8.57286509255765,-37.2788421636609));
#73449=CARTESIAN_POINT('Ctrl Pts',(104.45500069671,8.60087013504839,-37.3833293341507));
#73450=CARTESIAN_POINT('Ctrl Pts',(104.086176765825,8.37263814546984,-37.1545715999316));
#73451=CARTESIAN_POINT('Ctrl Pts',(104.194269413734,8.40065805141574,-37.2590601192072));
#73452=CARTESIAN_POINT('Ctrl Pts',(104.302362090345,8.42867771564422,-37.3635486513814));
#73453=CARTESIAN_POINT('Ctrl Pts',(104.410455468834,8.45669707232437,-37.4680365334307));
#73454=CARTESIAN_POINT('Ctrl Pts',(104.087867965648,8.29492882695158,-37.1736444530859));
#73455=CARTESIAN_POINT('Ctrl Pts',(104.195955578134,8.32295393531793,-37.2781367752932));
#73456=CARTESIAN_POINT('Ctrl Pts',(104.304043604526,8.35097872169308,-37.3826287412755));
#73457=CARTESIAN_POINT('Ctrl Pts',(104.41213203436,8.37900319423444,-37.4871203601462));
#73458=CARTESIAN_POINT('',(104.624264068716,8.62250767116921,-37.2024510141591));
#73459=CARTESIAN_POINT('',(104.41213203436,8.37900319423404,-37.4871203601444));
#73460=CARTESIAN_POINT('Origin',(104.624264068716,8.33272992328249,-37.2800967276899));
#73461=CARTESIAN_POINT('',(104.087867965648,8.29492882695115,-37.1736444530839));
#73462=CARTESIAN_POINT('Ctrl Pts',(104.41213203436,8.37900319423444,-37.4871203601462));
#73463=CARTESIAN_POINT('Ctrl Pts',(104.304043604526,8.35097872169308,-37.3826287412755));
#73464=CARTESIAN_POINT('Ctrl Pts',(104.195955578134,8.32295393531793,-37.2781367752932));
#73465=CARTESIAN_POINT('Ctrl Pts',(104.087867965648,8.29492882695158,-37.1736444530859));
#73466=CARTESIAN_POINT('Origin',(104.300000000004,8.24872986069581,-36.9666042262774));
#73467=CARTESIAN_POINT('Ctrl Pts',(104.300000000004,8.53850760858253,-36.8889585127467));
#73468=CARTESIAN_POINT('Ctrl Pts',(104.40808761249,8.5665077355745,-36.9934564092991));
#73469=CARTESIAN_POINT('Ctrl Pts',(104.516175638882,8.59450775553531,-37.0979539064057));
#73470=CARTESIAN_POINT('Ctrl Pts',(104.624264068716,8.62250767116921,-37.2024510141591));
#73471=CARTESIAN_POINT('Origin',(104.3,8.24872986069478,-36.9666042262736));
#73472=CARTESIAN_POINT('Origin',(104.3,8.24872986069478,-36.9666042262736));
#73473=CARTESIAN_POINT('Origin',(113.,8.33272992328154,-37.2800967276863));
#73474=CARTESIAN_POINT('',(121.811388243054,8.62250767116826,-37.2024510141556));
#73475=CARTESIAN_POINT('',(121.5,8.39817021063715,-37.5728723564378));
#73476=CARTESIAN_POINT('Ctrl Pts',(121.811388687965,8.62250778625266,-37.2024514436577));
#73477=CARTESIAN_POINT('Ctrl Pts',(121.80796264376,8.62339502101781,-37.2057626685107));
#73478=CARTESIAN_POINT('Ctrl Pts',(121.80455782351,8.62421946419965,-37.2090666597662));
#73479=CARTESIAN_POINT('Ctrl Pts',(121.765406035132,8.63305961883979,-37.2472073755322));
#73480=CARTESIAN_POINT('Ctrl Pts',(121.726559498935,8.6353211779098,-37.2865621995426));
#73481=CARTESIAN_POINT('Ctrl Pts',(121.652509215907,8.62308008690721,-37.3653949038344));
#73482=CARTESIAN_POINT('Ctrl Pts',(121.617288389766,8.60866399825096,-37.4048701574215));
#73483=CARTESIAN_POINT('Ctrl Pts',(121.56412779323,8.56856437653813,-37.4686076043297));
#73484=CARTESIAN_POINT('Ctrl Pts',(121.541159186122,8.5427443626867,-37.4980708374905));
#73485=CARTESIAN_POINT('Ctrl Pts',(121.517077828304,8.49410315611479,-37.533796113814));
#73486=CARTESIAN_POINT('Ctrl Pts',(121.510716614322,8.47626683430663,-37.5443504602798));
#73487=CARTESIAN_POINT('Ctrl Pts',(121.502178291748,8.43844642422112,-37.5616201820783));
#73488=CARTESIAN_POINT('Ctrl Pts',(121.5,8.4184630618731,-37.5683365621785));
#73489=CARTESIAN_POINT('Ctrl Pts',(121.5,8.39817021063715,-37.5728723564378));
#73490=CARTESIAN_POINT('',(104.624264068712,8.39817021063716,-37.5728723564378));
#73491=CARTESIAN_POINT('',(113.,8.39817021063716,-37.5728723564378));
#73492=CARTESIAN_POINT('Origin',(104.624264068712,8.33272992328154,-37.2800967276863));
#73493=CARTESIAN_POINT('',(113.,8.62250767116826,-37.2024510141556));
#73494=CARTESIAN_POINT('Origin',(104.624264068712,8.33272992328169,-37.2800967276863));
#73495=CARTESIAN_POINT('Origin',(104.624264068712,8.33272992328169,-37.2800967276863));
#73496=CARTESIAN_POINT('Origin',(104.3,0.,0.));
#73497=CARTESIAN_POINT('',(104.087867965649,6.56222288596764,-37.5183010937784));
#73498=CARTESIAN_POINT('Origin',(104.087867965644,2.22044604925031E-15,
0.));
#73499=CARTESIAN_POINT('Origin',(104.3,6.52567430068159,-37.3093412868425));
#73500=CARTESIAN_POINT('Origin',(104.25,0.,0.));
#73501=CARTESIAN_POINT('',(104.412132034356,6.60451033490358,-37.8400889356902));
#73502=CARTESIAN_POINT('Origin',(104.412132034356,1.66533453693773E-15,
0.));
#73503=CARTESIAN_POINT('Ctrl Pts',(104.087867965649,6.56222288596808,-37.5183010937809));
#73504=CARTESIAN_POINT('Ctrl Pts',(104.195955578133,6.57631854246989,-37.6255641562333));
#73505=CARTESIAN_POINT('Ctrl Pts',(104.304043604524,6.59041436013136,-37.7328267663559));
#73506=CARTESIAN_POINT('Ctrl Pts',(104.412132034356,6.60451033490358,-37.8400889356902));
#73507=CARTESIAN_POINT('Origin',(104.624264068712,0.,0.));
#73508=CARTESIAN_POINT('',(104.624264068712,6.61961818902331,-37.9266483495649));
#73509=CARTESIAN_POINT('Origin',(104.624264068712,0.,0.));
#73510=CARTESIAN_POINT('Origin',(104.624264068712,6.56803674858936,-37.6311160247631));
#73511=CARTESIAN_POINT('Origin',(113.,0.,0.));
#73512=CARTESIAN_POINT('',(121.5,6.61961818902331,-37.9266483495649));
#73513=CARTESIAN_POINT('Origin',(121.5,0.,0.));
#73514=CARTESIAN_POINT('',(113.,6.61961818902331,-37.9266483495649));
#73515=CARTESIAN_POINT('Origin',(104.3,8.52742811260079,-24.7680340892069));
#73516=CARTESIAN_POINT('',(104.3,13.2804347819611,-35.4588694735005));
#73517=CARTESIAN_POINT('Origin',(104.3,13.0032709222077,-35.57367450321));
#73518=CARTESIAN_POINT('',(104.3,12.7669018890611,-34.2190913987366));
#73519=CARTESIAN_POINT('Origin',(104.3,12.3749329995982,-34.0567325686927));
#73520=CARTESIAN_POINT('',(104.3,8.80459197235417,-24.6532290594974));
#73521=CARTESIAN_POINT('Ctrl Pts',(104.300000000003,13.2804347819623,-35.4588694735034));
#73522=CARTESIAN_POINT('Ctrl Pts',(104.408087612489,13.3218350765183,-35.5588186261068));
#73523=CARTESIAN_POINT('Ctrl Pts',(104.516175638881,13.3632352128207,-35.6587673966521));
#73524=CARTESIAN_POINT('Ctrl Pts',(104.624264068715,13.4046351948679,-35.7587157947924));
#73525=CARTESIAN_POINT('Ctrl Pts',(104.243382456863,13.3020820369953,-35.5111305701923));
#73526=CARTESIAN_POINT('Ctrl Pts',(104.351473262603,13.3434810852367,-35.6110770987527));
#73527=CARTESIAN_POINT('Ctrl Pts',(104.459564357695,13.3848804265587,-35.7110231870809));
#73528=CARTESIAN_POINT('Ctrl Pts',(104.567655925526,13.4262791829526,-35.8109690043703));
#73529=CARTESIAN_POINT('Ctrl Pts',(104.130709407257,13.2825795738598,-35.6410563204708));
#73530=CARTESIAN_POINT('Ctrl Pts',(104.238806300056,13.3239837223043,-35.7409947737889));
#73531=CARTESIAN_POINT('Ctrl Pts',(104.346903653609,13.3653875253347,-35.840932862619));
#73532=CARTESIAN_POINT('Ctrl Pts',(104.455001203266,13.4067912933046,-35.9408707393213));
#73533=CARTESIAN_POINT('Ctrl Pts',(104.086176765824,13.1506538199745,-35.7438605133323));
#73534=CARTESIAN_POINT('Ctrl Pts',(104.194269413733,13.1920725002925,-35.8437977872112));
#73535=CARTESIAN_POINT('Ctrl Pts',(104.302362090344,13.2334909426446,-35.9437351054287));
#73536=CARTESIAN_POINT('Ctrl Pts',(104.410455468834,13.2749089952212,-36.0436718192265));
#73537=CARTESIAN_POINT('Ctrl Pts',(104.087867965647,13.0760988223457,-35.77291329703));
#73538=CARTESIAN_POINT('Ctrl Pts',(104.195955578133,13.1175231569589,-35.8728536622539));
#73539=CARTESIAN_POINT('Ctrl Pts',(104.304043604525,13.1589471258389,-35.9727937163286));
#73540=CARTESIAN_POINT('Ctrl Pts',(104.412132034359,13.2003707382629,-36.0727334672248));
#73541=CARTESIAN_POINT('',(104.624264068715,13.4046351948679,-35.7587157947924));
#73542=CARTESIAN_POINT('',(104.412132034359,13.2003707382623,-36.0727334672234));
#73543=CARTESIAN_POINT('Origin',(104.624264068715,13.1274713351145,-35.873520824502));
#73544=CARTESIAN_POINT('',(104.087867965647,13.0760988223451,-35.7729132970285));
#73545=CARTESIAN_POINT('Ctrl Pts',(104.412132034359,13.2003707382629,-36.0727334672248));
#73546=CARTESIAN_POINT('Ctrl Pts',(104.304043604525,13.1589471258389,-35.9727937163286));
#73547=CARTESIAN_POINT('Ctrl Pts',(104.195955578133,13.1175231569589,-35.8728536622539));
#73548=CARTESIAN_POINT('Ctrl Pts',(104.087867965647,13.0760988223457,-35.77291329703));
#73549=CARTESIAN_POINT('Origin',(104.300000000003,13.0032709222089,-35.573674503213));
#73550=CARTESIAN_POINT('Ctrl Pts',(104.300000000003,13.2804347819623,-35.4588694735034));
#73551=CARTESIAN_POINT('Ctrl Pts',(104.408087612489,13.3218350765183,-35.5588186261068));
#73552=CARTESIAN_POINT('Ctrl Pts',(104.516175638881,13.3632352128207,-35.6587673966521));
#73553=CARTESIAN_POINT('Ctrl Pts',(104.624264068715,13.4046351948679,-35.7587157947924));
#73554=CARTESIAN_POINT('Origin',(104.3,13.0032709222077,-35.57367450321));
#73555=CARTESIAN_POINT('Origin',(104.3,13.0032709222077,-35.57367450321));
#73556=CARTESIAN_POINT('Origin',(113.,13.1274713351134,-35.8735208244992));
#73557=CARTESIAN_POINT('',(121.811388243054,13.4046351948667,-35.7587157947897));
#73558=CARTESIAN_POINT('',(121.5,13.2305666597347,-36.155250045634));
#73559=CARTESIAN_POINT('Ctrl Pts',(121.811388687965,13.4046353650279,-35.7587162055958));
#73560=CARTESIAN_POINT('Ctrl Pts',(121.80796264376,13.4059472109483,-35.7618832950857));
#73561=CARTESIAN_POINT('Ctrl Pts',(121.80455782351,13.4071958583021,-35.7650514088087));
#73562=CARTESIAN_POINT('Ctrl Pts',(121.765406035132,13.4209387465913,-35.8017119537402));
#73563=CARTESIAN_POINT('Ctrl Pts',(121.726559498935,13.4283177930335,-35.8404348990817));
#73564=CARTESIAN_POINT('Ctrl Pts',(121.652509215907,13.426471158975,-35.9201909616573));
#73565=CARTESIAN_POINT('Ctrl Pts',(121.617288389766,13.4173309564933,-35.9612101761366));
#73566=CARTESIAN_POINT('Ctrl Pts',(121.56412779323,13.3858937988498,-36.0296363912825));
#73567=CARTESIAN_POINT('Ctrl Pts',(121.541159186122,13.3641404024312,-36.0622177504903));
#73568=CARTESIAN_POINT('Ctrl Pts',(121.517077828304,13.320578412409,-36.1039863436012));
#73569=CARTESIAN_POINT('Ctrl Pts',(121.510716614322,13.304272301462,-36.1167785033387));
#73570=CARTESIAN_POINT('Ctrl Pts',(121.502178291748,13.2690296012548,-36.1388370343898));
#73571=CARTESIAN_POINT('Ctrl Pts',(121.5,13.2500938628618,-36.1481043071223));
#73572=CARTESIAN_POINT('Ctrl Pts',(121.5,13.2305666597347,-36.155250045634));
#73573=CARTESIAN_POINT('',(104.624264068712,13.2305666597347,-36.155250045634));
#73574=CARTESIAN_POINT('',(113.,13.2305666597347,-36.155250045634));
#73575=CARTESIAN_POINT('Origin',(104.624264068712,13.1274713351134,-35.8735208244992));
#73576=CARTESIAN_POINT('',(113.,13.4046351948667,-35.7587157947897));
#73577=CARTESIAN_POINT('Origin',(104.624264068712,13.1274713351135,-35.8735208244991));
#73578=CARTESIAN_POINT('Origin',(104.624264068712,13.1274713351135,-35.8735208244991));
#73579=CARTESIAN_POINT('Origin',(104.3,0.,0.));
#73580=CARTESIAN_POINT('',(104.087867965648,11.4032031398184,-36.3407848610969));
#73581=CARTESIAN_POINT('Origin',(104.087867965644,2.22044604925031E-15,
2.22044604925031E-15));
#73582=CARTESIAN_POINT('Origin',(104.3,11.3396925048198,-36.1383832819455));
#73583=CARTESIAN_POINT('Origin',(104.25,0.,0.));
#73584=CARTESIAN_POINT('',(104.412132034356,11.4871305554741,-36.6543001437251));
#73585=CARTESIAN_POINT('Origin',(104.412132034356,-2.22044604925031E-15,
-2.22044604925031E-15));
#73586=CARTESIAN_POINT('Ctrl Pts',(104.087867965648,11.403203139819,-36.3407848610989));
#73587=CARTESIAN_POINT('Ctrl Pts',(104.195955578133,11.4311788451333,-36.4452904208128));
#73588=CARTESIAN_POINT('Ctrl Pts',(104.304043604523,11.4591546511876,-36.5497955110311));
#73589=CARTESIAN_POINT('Ctrl Pts',(104.412132034356,11.4871305554741,-36.6543001437251));
#73590=CARTESIAN_POINT('Origin',(104.624264068712,0.,0.));
#73591=CARTESIAN_POINT('',(104.624264068712,11.5134074305014,-36.7381470591438));
#73592=CARTESIAN_POINT('Origin',(104.624264068712,0.,0.));
#73593=CARTESIAN_POINT('Origin',(104.624264068712,11.4236925674066,-36.4518757833583));
#73594=CARTESIAN_POINT('Origin',(113.,0.,0.));
#73595=CARTESIAN_POINT('',(121.5,11.5134074305014,-36.7381470591438));
#73596=CARTESIAN_POINT('Origin',(121.5,0.,0.));
#73597=CARTESIAN_POINT('',(113.,11.5134074305014,-36.7381470591438));
#73598=CARTESIAN_POINT('Ctrl Pts',(104.624264068712,-8.6225076711683,-37.2024510141555));
#73599=CARTESIAN_POINT('Ctrl Pts',(104.516175638879,-8.59450775553473,-37.0979539064034));
#73600=CARTESIAN_POINT('Ctrl Pts',(104.408087612489,-8.56650773557424,-36.9934564092979));
#73601=CARTESIAN_POINT('Ctrl Pts',(104.300000000004,-8.53850760858261,-36.8889585127468));
#73602=CARTESIAN_POINT('Ctrl Pts',(104.567655925523,-8.63714607945702,-37.257082297631));
#73603=CARTESIAN_POINT('Ctrl Pts',(104.459564357693,-8.60914704212253,-37.1525879086302));
#73604=CARTESIAN_POINT('Ctrl Pts',(104.351473262603,-8.58114746024159,-37.0480931745608));
#73605=CARTESIAN_POINT('Ctrl Pts',(104.243382456864,-8.5531482263959,-36.9435980422802));
#73606=CARTESIAN_POINT('Ctrl Pts',(104.455000696706,-8.60087013504747,-37.3833293341471));
#73607=CARTESIAN_POINT('Ctrl Pts',(104.346903147051,-8.57286509255708,-37.2788421636586));
#73608=CARTESIAN_POINT('Ctrl Pts',(104.238805793129,-8.54486004340222,-37.1743547785458));
#73609=CARTESIAN_POINT('Ctrl Pts',(104.130708900332,-8.51685469895562,-37.0698669867126));
#73610=CARTESIAN_POINT('Ctrl Pts',(104.410455468831,-8.45669707232346,-37.4680365334272));
#73611=CARTESIAN_POINT('Ctrl Pts',(104.302362090343,-8.42867771564364,-37.363548651379));
#73612=CARTESIAN_POINT('Ctrl Pts',(104.194269413732,-8.40065805141549,-37.2590601192061));
#73613=CARTESIAN_POINT('Ctrl Pts',(104.086176765825,-8.37263814546992,-37.1545715999318));
#73614=CARTESIAN_POINT('Ctrl Pts',(104.412132034356,-8.37900319423354,-37.4871203601426));
#73615=CARTESIAN_POINT('Ctrl Pts',(104.304043604523,-8.35097872169251,-37.3826287412732));
#73616=CARTESIAN_POINT('Ctrl Pts',(104.195955578133,-8.32295393531767,-37.2781367752921));
#73617=CARTESIAN_POINT('Ctrl Pts',(104.087867965648,-8.29492882695166,-37.173644453086));
#73618=CARTESIAN_POINT('',(104.300000000004,-8.53850760858261,-36.8889585127468));
#73619=CARTESIAN_POINT('Origin',(104.300000000004,-8.24872986069589,-36.9666042262775));
#73620=CARTESIAN_POINT('',(104.624264068712,-8.6225076711683,-37.2024510141556));
#73621=CARTESIAN_POINT('Origin',(104.624264068712,-8.33272992328158,-37.2800967276863));
#73622=CARTESIAN_POINT('Ctrl Pts',(104.624264068712,-8.6225076711683,-37.2024510141555));
#73623=CARTESIAN_POINT('Ctrl Pts',(104.516175638879,-8.59450775553473,-37.0979539064034));
#73624=CARTESIAN_POINT('Ctrl Pts',(104.408087612489,-8.56650773557424,-36.9934564092979));
#73625=CARTESIAN_POINT('Ctrl Pts',(104.300000000004,-8.53850760858261,-36.8889585127468));
#73626=CARTESIAN_POINT('Origin',(104.3,-2.06696949019975,-13.8959604433702));
#73627=CARTESIAN_POINT('Origin',(104.3,-8.24872986069483,-36.9666042262736));
#73628=CARTESIAN_POINT('',(104.3,-8.19119157206625,-35.5927574181843));
#73629=CARTESIAN_POINT('',(104.3,-2.35674723808646,-13.8183147298394));
#73630=CARTESIAN_POINT('Origin',(104.3,-7.82376811064877,-35.3806253838283));
#73631=CARTESIAN_POINT('Origin',(104.3,-8.24872986069483,-36.9666042262736));
#73632=CARTESIAN_POINT('Origin',(104.624264068712,-8.33272992328159,-37.2800967276863));
#73633=CARTESIAN_POINT('Origin',(104.624264068712,-8.33272992328159,-37.2800967276863));
#73634=CARTESIAN_POINT('Origin',(113.,-6.21624207609293,-37.2573594669753));
#73635=CARTESIAN_POINT('',(121.7,-6.05308433581787,-36.018053390258));
#73636=CARTESIAN_POINT('',(103.5,-6.05308433581787,-36.018053390258));
#73637=CARTESIAN_POINT('Origin',(121.7,-6.01392647815185,-35.7206199318459));
#73638=CARTESIAN_POINT('',(121.912131484566,-6.2574460569156,-37.5703347737697));
#73639=CARTESIAN_POINT('Ctrl Pts',(121.912131759621,-6.25744609279661,-37.570335046313));
#73640=CARTESIAN_POINT('Ctrl Pts',(121.938311286558,-6.25402699553555,-37.5443644242305));
#73641=CARTESIAN_POINT('Ctrl Pts',(121.962987211232,-6.24920375098245,-37.5077282445796));
#73642=CARTESIAN_POINT('Ctrl Pts',(121.991329280155,-6.24026960603904,-37.439866676382));
#73643=CARTESIAN_POINT('Ctrl Pts',(122.,-6.23457739606559,-37.3966300490657));
#73644=CARTESIAN_POINT('Ctrl Pts',(122.,-6.22974103737681,-37.3598942576648));
#73645=CARTESIAN_POINT('',(121.75,-6.27862069582415,-37.7311721243447));
#73646=CARTESIAN_POINT('Origin',(121.7,-3.32857347866203,-12.2168887231457));
#73647=CARTESIAN_POINT('',(121.7,-13.2804347819611,-35.4588694735005));
#73648=CARTESIAN_POINT('Origin',(121.7,-13.0032709222078,-35.57367450321));
#73649=CARTESIAN_POINT('',(121.7,-12.7669018890611,-34.2190913987366));
#73650=CARTESIAN_POINT('Origin',(121.7,-12.3749329995982,-34.0567325686927));
#73651=CARTESIAN_POINT('',(121.7,-3.60573733841542,-12.1020836934361));
#73652=CARTESIAN_POINT('Ctrl Pts',(121.699999999997,-13.2804347819624,-35.4588694735035));
#73653=CARTESIAN_POINT('Ctrl Pts',(121.591912387511,-13.3218350765184,-35.5588186261068));
#73654=CARTESIAN_POINT('Ctrl Pts',(121.483824361119,-13.3632352128208,-35.6587673966521));
#73655=CARTESIAN_POINT('Ctrl Pts',(121.375735931285,-13.4046351948679,-35.7587157947924));
#73656=CARTESIAN_POINT('Ctrl Pts',(121.756617543137,-13.3020820369954,-35.5111305701923));
#73657=CARTESIAN_POINT('Ctrl Pts',(121.648526737397,-13.3434810852367,-35.6110770987527));
#73658=CARTESIAN_POINT('Ctrl Pts',(121.540435642305,-13.3848804265588,-35.711023187081));
#73659=CARTESIAN_POINT('Ctrl Pts',(121.432344074474,-13.4262791829526,-35.8109690043703));
#73660=CARTESIAN_POINT('Ctrl Pts',(121.86928828501,-13.2825757663851,-35.6410554019366));
#73661=CARTESIAN_POINT('Ctrl Pts',(121.761191392211,-13.3239799148297,-35.7409938552546));
#73662=CARTESIAN_POINT('Ctrl Pts',(121.653094040341,-13.3653837198587,-35.8409319450387));
#73663=CARTESIAN_POINT('Ctrl Pts',(121.544996490684,-13.4067874878286,-35.9408698217409));
#73664=CARTESIAN_POINT('Ctrl Pts',(121.913823234176,-13.1506538199745,-35.7438605133323));
#73665=CARTESIAN_POINT('Ctrl Pts',(121.805730586267,-13.1920725002925,-35.8437977872112));
#73666=CARTESIAN_POINT('Ctrl Pts',(121.697637909656,-13.2334909426446,-35.9437351054287));
#73667=CARTESIAN_POINT('Ctrl Pts',(121.589544531166,-13.2749089952212,-36.0436718192265));
#73668=CARTESIAN_POINT('Ctrl Pts',(121.912132034353,-13.0760988223457,-35.77291329703));
#73669=CARTESIAN_POINT('Ctrl Pts',(121.804044421867,-13.117523156959,-35.8728536622539));
#73670=CARTESIAN_POINT('Ctrl Pts',(121.695956395475,-13.158947125839,-35.9727937163286));
#73671=CARTESIAN_POINT('Ctrl Pts',(121.587867965641,-13.2003707382629,-36.0727334672248));
#73672=CARTESIAN_POINT('',(121.375735931285,-13.4046351948679,-35.7587157947924));
#73673=CARTESIAN_POINT('',(121.587867965641,-13.2003707382624,-36.0727334672234));
#73674=CARTESIAN_POINT('Origin',(121.375735931285,-13.1274713351146,-35.8735208245019));
#73675=CARTESIAN_POINT('',(121.912132034353,-13.0760988223452,-35.7729132970285));
#73676=CARTESIAN_POINT('Ctrl Pts',(121.587867965641,-13.2003707382629,-36.0727334672248));
#73677=CARTESIAN_POINT('Ctrl Pts',(121.695956395475,-13.158947125839,-35.9727937163286));
#73678=CARTESIAN_POINT('Ctrl Pts',(121.804044421867,-13.117523156959,-35.8728536622539));
#73679=CARTESIAN_POINT('Ctrl Pts',(121.912132034353,-13.0760988223457,-35.77291329703));
#73680=CARTESIAN_POINT('Origin',(121.699999999997,-13.003270922209,-35.573674503213));
#73681=CARTESIAN_POINT('Ctrl Pts',(121.699999999997,-13.2804347819624,-35.4588694735035));
#73682=CARTESIAN_POINT('Ctrl Pts',(121.591912387511,-13.3218350765184,-35.5588186261068));
#73683=CARTESIAN_POINT('Ctrl Pts',(121.483824361119,-13.3632352128208,-35.6587673966521));
#73684=CARTESIAN_POINT('Ctrl Pts',(121.375735931285,-13.4046351948679,-35.7587157947924));
#73685=CARTESIAN_POINT('Origin',(121.7,-13.0032709222078,-35.57367450321));
#73686=CARTESIAN_POINT('Origin',(121.7,-13.0032709222078,-35.57367450321));
#73687=CARTESIAN_POINT('Origin',(113.,-13.1274713351134,-35.8735208244992));
#73688=CARTESIAN_POINT('',(104.188611756946,-13.4046351948668,-35.7587157947897));
#73689=CARTESIAN_POINT('',(104.5,-13.2305666597347,-36.155250045634));
#73690=CARTESIAN_POINT('Ctrl Pts',(104.188611312035,-13.4046353650279,-35.7587162055958));
#73691=CARTESIAN_POINT('Ctrl Pts',(104.19203735624,-13.4059472109483,-35.7618832950857));
#73692=CARTESIAN_POINT('Ctrl Pts',(104.19544217649,-13.4071958583021,-35.7650514088087));
#73693=CARTESIAN_POINT('Ctrl Pts',(104.234593964868,-13.4209387465913,-35.8017119537402));
#73694=CARTESIAN_POINT('Ctrl Pts',(104.273440501065,-13.4283177930336,-35.8404348990817));
#73695=CARTESIAN_POINT('Ctrl Pts',(104.347490784093,-13.426471158975,-35.9201909616572));
#73696=CARTESIAN_POINT('Ctrl Pts',(104.382711610234,-13.4173309564933,-35.9612101761365));
#73697=CARTESIAN_POINT('Ctrl Pts',(104.43587220677,-13.3858937988499,-36.0296363912825));
#73698=CARTESIAN_POINT('Ctrl Pts',(104.458840813878,-13.3641404024313,-36.0622177504903));
#73699=CARTESIAN_POINT('Ctrl Pts',(104.482922171696,-13.320578412409,-36.1039863436012));
#73700=CARTESIAN_POINT('Ctrl Pts',(104.489283385678,-13.3042723014621,-36.1167785033386));
#73701=CARTESIAN_POINT('Ctrl Pts',(104.497821708253,-13.2690296012548,-36.1388370343898));
#73702=CARTESIAN_POINT('Ctrl Pts',(104.5,-13.2500938628619,-36.1481043071223));
#73703=CARTESIAN_POINT('Ctrl Pts',(104.5,-13.2305666597347,-36.155250045634));
#73704=CARTESIAN_POINT('',(121.375735931288,-13.2305666597347,-36.155250045634));
#73705=CARTESIAN_POINT('',(113.,-13.2305666597347,-36.155250045634));
#73706=CARTESIAN_POINT('Origin',(121.375735931288,-13.1274713351134,-35.8735208244992));
#73707=CARTESIAN_POINT('',(113.,-13.4046351948668,-35.7587157947897));
#73708=CARTESIAN_POINT('Origin',(121.375735931288,-13.1274713351135,-35.8735208244991));
#73709=CARTESIAN_POINT('Origin',(121.375735931288,-13.1274713351135,-35.8735208244991));
#73710=CARTESIAN_POINT('Origin',(121.7,0.,0.));
#73711=CARTESIAN_POINT('',(121.912132034352,-11.4032031398185,-36.3407848610969));
#73712=CARTESIAN_POINT('Origin',(121.912132034356,1.11022302462516E-15,
0.));
#73713=CARTESIAN_POINT('Origin',(121.7,-11.3396925048197,-36.1383832819456));
#73714=CARTESIAN_POINT('Origin',(121.75,0.,0.));
#73715=CARTESIAN_POINT('',(121.587867965644,-11.4871305554742,-36.6543001437251));
#73716=CARTESIAN_POINT('Origin',(121.587867965644,2.22044604925031E-15,
-2.22044604925031E-15));
#73717=CARTESIAN_POINT('Ctrl Pts',(121.912132034352,-11.4032031398191,-36.3407848610989));
#73718=CARTESIAN_POINT('Ctrl Pts',(121.804044421867,-11.4311788451333,-36.4452904208128));
#73719=CARTESIAN_POINT('Ctrl Pts',(121.695956395477,-11.4591546511876,-36.5497955110311));
#73720=CARTESIAN_POINT('Ctrl Pts',(121.587867965644,-11.4871305554742,-36.6543001437251));
#73721=CARTESIAN_POINT('Origin',(104.3,-5.91887145918133,-10.1084182630942));
#73722=CARTESIAN_POINT('',(104.3,-15.6825215664905,-34.4638925493512));
#73723=CARTESIAN_POINT('Origin',(104.3,-15.9596854262439,-34.3490875196417));
#73724=CARTESIAN_POINT('',(104.3,-15.1689886735905,-33.2241144745873));
#73725=CARTESIAN_POINT('Origin',(104.3,-15.3313475036343,-32.8321455851244));
#73726=CARTESIAN_POINT('',(104.3,-5.64170759942795,-10.2232232928037));
#73727=CARTESIAN_POINT('Ctrl Pts',(104.300000000003,-15.6825215664917,-34.4638925493543));
#73728=CARTESIAN_POINT('Ctrl Pts',(104.408087612489,-15.7239218610478,-34.5638417019577));
#73729=CARTESIAN_POINT('Ctrl Pts',(104.516175638881,-15.7653219973501,-34.6637904725029));
#73730=CARTESIAN_POINT('Ctrl Pts',(104.624264068715,-15.8067219793973,-34.7637388706433));
#73731=CARTESIAN_POINT('Ctrl Pts',(104.243382456863,-15.7041688215248,-34.5161536460432));
#73732=CARTESIAN_POINT('Ctrl Pts',(104.351473262603,-15.7455681418798,-34.6161000618904));
#73733=CARTESIAN_POINT('Ctrl Pts',(104.459564357695,-15.7869669437042,-34.7160463736859));
#73734=CARTESIAN_POINT('Ctrl Pts',(104.567655925526,-15.828365967482,-34.8159920802212));
#73735=CARTESIAN_POINT('Ctrl Pts',(104.130709646627,-15.8098307364183,-34.5942343545562));
#73736=CARTESIAN_POINT('Ctrl Pts',(104.238806539425,-15.8512207403264,-34.6941786667331));
#73737=CARTESIAN_POINT('Ctrl Pts',(104.346903892804,-15.8926107306706,-34.7941224771499));
#73738=CARTESIAN_POINT('Ctrl Pts',(104.455001442461,-15.934000595886,-34.8940661125617));
#73739=CARTESIAN_POINT('Ctrl Pts',(104.086176765824,-15.9758096616227,-34.5736426479042));
#73740=CARTESIAN_POINT('Ctrl Pts',(104.194269413733,-16.017188555955,-34.6735964016779));
#73741=CARTESIAN_POINT('Ctrl Pts',(104.302362090344,-16.0585676499069,-34.7735500185365));
#73742=CARTESIAN_POINT('Ctrl Pts',(104.410455468834,-16.0999465920824,-34.8735029323928));
#73743=CARTESIAN_POINT('Ctrl Pts',(104.087867965647,-16.0490714263823,-34.5414677238745));
#73744=CARTESIAN_POINT('Ctrl Pts',(104.195955578133,-16.0904485084352,-34.6414276617497));
#73745=CARTESIAN_POINT('Ctrl Pts',(104.304043604525,-16.1318256290849,-34.7413871209968));
#73746=CARTESIAN_POINT('Ctrl Pts',(104.412132034359,-16.1732027874075,-34.8413461138118));
#73747=CARTESIAN_POINT('',(104.624264068715,-15.8067219793973,-34.7637388706433));
#73748=CARTESIAN_POINT('',(104.412132034359,-16.1732027874068,-34.8413461138104));
#73749=CARTESIAN_POINT('Origin',(104.624264068715,-16.0838858391507,-34.6489338409338));
#73750=CARTESIAN_POINT('',(104.087867965647,-16.0490714263816,-34.541467723873));
#73751=CARTESIAN_POINT('Ctrl Pts',(104.412132034359,-16.1732027874075,-34.8413461138118));
#73752=CARTESIAN_POINT('Ctrl Pts',(104.304043604525,-16.1318256290849,-34.7413871209968));
#73753=CARTESIAN_POINT('Ctrl Pts',(104.195955578133,-16.0904485084352,-34.6414276617497));
#73754=CARTESIAN_POINT('Ctrl Pts',(104.087867965647,-16.0490714263823,-34.5414677238745));
#73755=CARTESIAN_POINT('Origin',(104.300000000003,-15.9596854262451,-34.3490875196448));
#73756=CARTESIAN_POINT('Ctrl Pts',(104.300000000003,-15.6825215664917,-34.4638925493543));
#73757=CARTESIAN_POINT('Ctrl Pts',(104.408087612489,-15.7239218610478,-34.5638417019577));
#73758=CARTESIAN_POINT('Ctrl Pts',(104.516175638881,-15.7653219973501,-34.6637904725029));
#73759=CARTESIAN_POINT('Ctrl Pts',(104.624264068715,-15.8067219793973,-34.7637388706433));
#73760=CARTESIAN_POINT('Origin',(104.3,-15.9596854262439,-34.3490875196417));
#73761=CARTESIAN_POINT('Origin',(104.3,-15.9596854262439,-34.3490875196417));
#73762=CARTESIAN_POINT('Origin',(113.,-16.0838858391495,-34.6489338409309));
#73763=CARTESIAN_POINT('',(121.811388243054,-15.8067219793961,-34.7637388706404));
#73764=CARTESIAN_POINT('',(121.5,-16.210199078724,-34.9210458868021));
#73765=CARTESIAN_POINT('Ctrl Pts',(121.811388687965,-15.8067221495579,-34.7637392814463));
#73766=CARTESIAN_POINT('Ctrl Pts',(121.80796264376,-15.8080340048666,-34.7669063670474));
#73767=CARTESIAN_POINT('Ctrl Pts',(121.80455782351,-15.8093912725525,-34.7700294887557));
#73768=CARTESIAN_POINT('Ctrl Pts',(121.765406035132,-15.8255965029732,-34.8056700981812));
#73769=CARTESIAN_POINT('Ctrl Pts',(121.726559498935,-15.8477599864337,-34.8382691291976));
#73770=CARTESIAN_POINT('Ctrl Pts',(121.652509215907,-15.9054618065868,-34.8933594144204));
#73771=CARTESIAN_POINT('Ctrl Pts',(121.617288389766,-15.9409298704602,-34.9159012799814));
#73772=CARTESIAN_POINT('Ctrl Pts',(121.56412779323,-16.0115439385518,-34.9420564933711));
#73773=CARTESIAN_POINT('Ctrl Pts',(121.541159186122,-16.0499644127093,-34.9497130192858));
#73774=CARTESIAN_POINT('Ctrl Pts',(121.517077828304,-16.1103022466854,-34.9484448961684));
#73775=CARTESIAN_POINT('Ctrl Pts',(121.510716614322,-16.1308778312071,-34.9459601574394));
#73776=CARTESIAN_POINT('Ctrl Pts',(121.502178291748,-16.1713959204003,-34.9366375420249));
#73777=CARTESIAN_POINT('Ctrl Pts',(121.5,-16.191338460817,-34.9298009043927));
#73778=CARTESIAN_POINT('Ctrl Pts',(121.5,-16.210199078724,-34.9210458868021));
#73779=CARTESIAN_POINT('',(104.624264068712,-16.210199078724,-34.9210458868021));
#73780=CARTESIAN_POINT('',(113.,-16.210199078724,-34.9210458868021));
#73781=CARTESIAN_POINT('Origin',(104.624264068712,-16.0838858391495,-34.6489338409309));
#73782=CARTESIAN_POINT('',(113.,-15.8067219793961,-34.7637388706404));
#73783=CARTESIAN_POINT('Origin',(104.624264068712,-16.0838858391494,-34.6489338409309));
#73784=CARTESIAN_POINT('Origin',(104.624264068712,-16.0838858391494,-34.6489338409309));
#73785=CARTESIAN_POINT('Origin',(104.3,0.,0.));
#73786=CARTESIAN_POINT('',(104.087867965647,-17.6335331415094,-33.7600976763358));
#73787=CARTESIAN_POINT('Origin',(104.087867965644,-2.22044604925031E-15,
2.22044604925031E-15));
#73788=CARTESIAN_POINT('Origin',(104.3,-17.5353224130539,-33.5720693465106));
#73789=CARTESIAN_POINT('Origin',(104.25,0.,0.));
#73790=CARTESIAN_POINT('',(104.412132034356,-17.7958762791241,-34.041132103426));
#73791=CARTESIAN_POINT('Origin',(104.412132034356,-2.22044604925031E-15,
0.));
#73792=CARTESIAN_POINT('Ctrl Pts',(104.087867965647,-17.63353314151,-33.7600976763371));
#73793=CARTESIAN_POINT('Ctrl Pts',(104.195955578132,-17.6876479205195,-33.8537760772191));
#73794=CARTESIAN_POINT('Ctrl Pts',(104.304043604523,-17.7417622963114,-33.9474542173515));
#73795=CARTESIAN_POINT('Ctrl Pts',(104.412132034356,-17.7958762791241,-34.041132103426));
#73796=CARTESIAN_POINT('Origin',(104.624264068712,0.,0.));
#73797=CARTESIAN_POINT('',(104.624264068712,-17.8365844450781,-34.1190013824203));
#73798=CARTESIAN_POINT('Origin',(104.624264068712,0.,0.));
#73799=CARTESIAN_POINT('Origin',(104.624264068712,-17.6975980727788,-33.8531390339859));
#73800=CARTESIAN_POINT('Origin',(113.,0.,0.));
#73801=CARTESIAN_POINT('',(121.5,-17.8365844450781,-34.1190013824203));
#73802=CARTESIAN_POINT('Origin',(121.5,0.,0.));
#73803=CARTESIAN_POINT('',(113.,-17.8365844450781,-34.1190013824203));
#73804=CARTESIAN_POINT('Ctrl Pts',(104.624264068712,-22.2029200028051,-31.0708922200351));
#73805=CARTESIAN_POINT('Ctrl Pts',(104.516175638879,-22.1370621419721,-30.9850645847965));
#73806=CARTESIAN_POINT('Ctrl Pts',(104.408087612488,-22.0712040357546,-30.8992366297665));
#73807=CARTESIAN_POINT('Ctrl Pts',(104.300000000003,-22.0053456777918,-30.8134083466558));
#73808=CARTESIAN_POINT('Ctrl Pts',(104.567655925523,-22.2373506156865,-31.1157630683446));
#73809=CARTESIAN_POINT('Ctrl Pts',(104.459564357693,-22.1714946067171,-31.0299376087941));
#73810=CARTESIAN_POINT('Ctrl Pts',(104.351473262602,-22.1056379626004,-30.9441120388309));
#73811=CARTESIAN_POINT('Ctrl Pts',(104.243382456862,-22.0397814876375,-30.858285967781));
#73812=CARTESIAN_POINT('Ctrl Pts',(104.455001803843,-22.252146783607,-31.2462823716862));
#73813=CARTESIAN_POINT('Ctrl Pts',(104.346904254187,-22.186287989002,-31.1604658792452));
#73814=CARTESIAN_POINT('Ctrl Pts',(104.238806901073,-22.1204291050614,-31.0746491908737));
#73815=CARTESIAN_POINT('Ctrl Pts',(104.130710008275,-22.054569793707,-30.9888322399387));
#73816=CARTESIAN_POINT('Ctrl Pts',(104.410455468831,-22.1513661623602,-31.37971421451));
#73817=CARTESIAN_POINT('Ctrl Pts',(104.302362090342,-22.0854938708666,-31.2939025424768));
#73818=CARTESIAN_POINT('Ctrl Pts',(104.194269413732,-22.0196210464434,-31.2080903875002));
#73819=CARTESIAN_POINT('Ctrl Pts',(104.086176765824,-21.9537480036384,-31.1222783369417));
#73820=CARTESIAN_POINT('Ctrl Pts',(104.412132034356,-22.0868894429017,-31.4270775313556));
#73821=CARTESIAN_POINT('Ctrl Pts',(104.304043604523,-22.0210109949489,-31.341264364705));
#73822=CARTESIAN_POINT('Ctrl Pts',(104.195955578132,-21.9551321242178,-31.255450997464));
#73823=CARTESIAN_POINT('Ctrl Pts',(104.087867965647,-21.8892528196841,-31.1696374243348));
#73824=CARTESIAN_POINT('Origin',(104.300000000003,-21.7673396757045,-30.9960367753584));
#73825=CARTESIAN_POINT('Origin',(104.624264068712,-21.9649140007177,-31.2535206487377));
#73826=CARTESIAN_POINT('Origin',(104.3,-3.17978755654757,-6.77226723466486));
#73827=CARTESIAN_POINT('Origin',(104.3,-21.7673396757028,-30.9960367753563));
#73828=CARTESIAN_POINT('Origin',(104.3,-20.7677983856497,-29.6934092049567));
#73829=CARTESIAN_POINT('Origin',(104.3,-21.7673396757028,-30.9960367753563));
#73830=CARTESIAN_POINT('Origin',(104.624264068712,-21.9649140007177,-31.2535206487377));
#73831=CARTESIAN_POINT('Origin',(121.7,-3.96526964499761,-6.22801134479455));
#73832=CARTESIAN_POINT('',(121.7,-25.8390437558098,-27.6775213868947));
#73833=CARTESIAN_POINT('Origin',(121.7,-25.6269117214538,-27.8896534212507));
#73834=CARTESIAN_POINT('',(121.7,-24.8901586977665,-26.7286363288515));
#73835=CARTESIAN_POINT('Origin',(121.7,-24.4658946290546,-26.7286363288515));
#73836=CARTESIAN_POINT('',(121.7,-4.17740167935357,-6.01587931043859));
#73837=CARTESIAN_POINT('Ctrl Pts',(121.699999999998,-25.8390437558115,-27.6775213868965));
#73838=CARTESIAN_POINT('Ctrl Pts',(121.591912387512,-25.915541525372,-27.7540191564569));
#73839=CARTESIAN_POINT('Ctrl Pts',(121.48382436112,-25.9920390025178,-27.8305166336028));
#73840=CARTESIAN_POINT('Ctrl Pts',(121.375735931286,-26.0685361946373,-27.9070138257223));
#73841=CARTESIAN_POINT('Ctrl Pts',(121.756617543138,-25.8790426675316,-27.7175202986166));
#73842=CARTESIAN_POINT('Ctrl Pts',(121.648526737397,-25.9555382814697,-27.7940161208215));
#73843=CARTESIAN_POINT('Ctrl Pts',(121.540435642306,-26.0320339977095,-27.8705114241477));
#73844=CARTESIAN_POINT('Ctrl Pts',(121.432344074475,-26.108529069824,-27.947006700909));
#73845=CARTESIAN_POINT('Ctrl Pts',(121.869287690755,-25.9107403075881,-27.8450200746977));
#73846=CARTESIAN_POINT('Ctrl Pts',(121.761190797956,-25.9872375432381,-27.9215064845882));
#73847=CARTESIAN_POINT('Ctrl Pts',(121.653093446519,-26.0637343230645,-27.9979926900664));
#73848=CARTESIAN_POINT('Ctrl Pts',(121.544995896862,-26.1402309865405,-28.0744787128348));
#73849=CARTESIAN_POINT('Ctrl Pts',(121.913823234177,-25.8282031306363,-27.9904837995326));
#73850=CARTESIAN_POINT('Ctrl Pts',(121.805730586268,-25.9047133406349,-28.0669635586562));
#73851=CARTESIAN_POINT('Ctrl Pts',(121.697637909656,-25.9812233477494,-28.1434434498089));
#73852=CARTESIAN_POINT('Ctrl Pts',(121.589544531167,-26.0577327634568,-28.2199229317112));
#73853=CARTESIAN_POINT('Ctrl Pts',(121.912132034354,-25.7704413132658,-28.045856034146));
#73854=CARTESIAN_POINT('Ctrl Pts',(121.804044421868,-25.8469579301586,-28.1223364854948));
#73855=CARTESIAN_POINT('Ctrl Pts',(121.695956395476,-25.9234740900862,-28.1988167893393));
#73856=CARTESIAN_POINT('Ctrl Pts',(121.587867965642,-25.9999898046701,-28.2752969494932));
#73857=CARTESIAN_POINT('',(121.375735931286,-26.0685361946373,-27.9070138257223));
#73858=CARTESIAN_POINT('',(121.587867965642,-25.9999898046693,-28.2752969494924));
#73859=CARTESIAN_POINT('Origin',(121.375735931286,-25.8564041602813,-28.1191458600783));
#73860=CARTESIAN_POINT('',(121.912132034354,-25.770441313265,-28.0458560341451));
#73861=CARTESIAN_POINT('Ctrl Pts',(121.587867965642,-25.9999898046701,-28.2752969494932));
#73862=CARTESIAN_POINT('Ctrl Pts',(121.695956395476,-25.9234740900862,-28.1988167893393));
#73863=CARTESIAN_POINT('Ctrl Pts',(121.804044421868,-25.8469579301586,-28.1223364854948));
#73864=CARTESIAN_POINT('Ctrl Pts',(121.912132034354,-25.7704413132658,-28.045856034146));
#73865=CARTESIAN_POINT('Origin',(121.699999999998,-25.6269117214555,-27.8896534212524));
#73866=CARTESIAN_POINT('Ctrl Pts',(121.699999999998,-25.8390437558115,-27.6775213868965));
#73867=CARTESIAN_POINT('Ctrl Pts',(121.591912387512,-25.915541525372,-27.7540191564569));
#73868=CARTESIAN_POINT('Ctrl Pts',(121.48382436112,-25.9920390025178,-27.8305166336028));
#73869=CARTESIAN_POINT('Ctrl Pts',(121.375735931286,-26.0685361946373,-27.9070138257223));
#73870=CARTESIAN_POINT('Origin',(121.7,-25.6269117214538,-27.8896534212507));
#73871=CARTESIAN_POINT('Origin',(121.7,-25.6269117214538,-27.8896534212507));
#73872=CARTESIAN_POINT('Origin',(113.,-25.8564041602798,-28.1191458600767));
#73873=CARTESIAN_POINT('',(104.188611756946,-26.0685361946357,-27.9070138257207));
#73874=CARTESIAN_POINT('',(104.5,-26.0594649259364,-28.3399768485066));
#73875=CARTESIAN_POINT('Ctrl Pts',(104.188611312035,-26.0685365090528,-27.9070141401382));
#73876=CARTESIAN_POINT('Ctrl Pts',(104.19203735624,-26.0709604893251,-27.9094381275961));
#73877=CARTESIAN_POINT('Ctrl Pts',(104.19544217649,-26.0733264736922,-27.9118872463662));
#73878=CARTESIAN_POINT('Ctrl Pts',(104.234593964868,-26.100052630067,-27.940497997818));
#73879=CARTESIAN_POINT('Ctrl Pts',(104.273440501065,-26.121688609679,-27.9734494956375));
#73880=CARTESIAN_POINT('Ctrl Pts',(104.347490784093,-26.1505038660466,-28.0478411657046));
#73881=CARTESIAN_POINT('Ctrl Pts',(104.382711610234,-26.1577567938406,-28.0892357824599));
#73882=CARTESIAN_POINT('Ctrl Pts',(104.43587220677,-26.1548982262093,-28.1644838415112));
#73883=CARTESIAN_POINT('Ctrl Pts',(104.458840813878,-26.1472690548683,-28.2029097568318));
#73884=CARTESIAN_POINT('Ctrl Pts',(104.482922171696,-26.123007172468,-28.2581693569711));
#73885=CARTESIAN_POINT('Ctrl Pts',(104.489283385678,-26.1128376379049,-28.2762278500349));
#73886=CARTESIAN_POINT('Ctrl Pts',(104.497821708252,-26.0887190628886,-28.3100940728715));
#73887=CARTESIAN_POINT('Ctrl Pts',(104.5,-26.0747711534923,-28.3259023098338));
#73888=CARTESIAN_POINT('Ctrl Pts',(104.5,-26.0594649259364,-28.3399768485066));
#73889=CARTESIAN_POINT('',(121.375735931288,-26.0594649259364,-28.3399768485066));
#73890=CARTESIAN_POINT('',(113.,-26.0594649259364,-28.3399768485066));
#73891=CARTESIAN_POINT('Origin',(121.375735931288,-25.8564041602798,-28.1191458600767));
#73892=CARTESIAN_POINT('',(113.,-26.0685361946357,-27.9070138257207));
#73893=CARTESIAN_POINT('Origin',(121.375735931288,-25.8564041602798,-28.1191458600766));
#73894=CARTESIAN_POINT('Origin',(121.375735931288,-25.8564041602798,-28.1191458600766));
#73895=CARTESIAN_POINT('Origin',(121.7,0.,0.));
#73896=CARTESIAN_POINT('',(121.912132034353,-24.4422022714321,-29.2106904110607));
#73897=CARTESIAN_POINT('Origin',(121.912132034356,0.,2.22044604925031E-15));
#73898=CARTESIAN_POINT('Origin',(121.7,-24.3060703646347,-29.0480002025285));
#73899=CARTESIAN_POINT('Origin',(121.75,0.,0.));
#73900=CARTESIAN_POINT('',(121.587867965644,-24.6397181974285,-29.4682231323184));
#73901=CARTESIAN_POINT('Origin',(121.587867965644,2.22044604925031E-15,
-2.22044604925031E-15));
#73902=CARTESIAN_POINT('Ctrl Pts',(121.912132034353,-24.4422022714329,-29.2106904110617));
#73903=CARTESIAN_POINT('Ctrl Pts',(121.804044421868,-24.5080409992732,-29.2965351197829));
#73904=CARTESIAN_POINT('Ctrl Pts',(121.695956395477,-24.573879640517,-29.3823793561953));
#73905=CARTESIAN_POINT('Ctrl Pts',(121.587867965644,-24.6397181974285,-29.4682231323184));
#73906=CARTESIAN_POINT('Ctrl Pts',(121.375735931288,-24.2656386875623,-29.4881125046124));
#73907=CARTESIAN_POINT('Ctrl Pts',(121.483824361121,-24.1997808267293,-29.4022848693738));
#73908=CARTESIAN_POINT('Ctrl Pts',(121.591912387512,-24.1339227205117,-29.3164569143438));
#73909=CARTESIAN_POINT('Ctrl Pts',(121.699999999997,-24.068064362549,-29.2306286312331));
#73910=CARTESIAN_POINT('Ctrl Pts',(121.432344074477,-24.3000693004437,-29.5329833529219));
#73911=CARTESIAN_POINT('Ctrl Pts',(121.540435642307,-24.2342130618665,-29.4471580695557));
#73912=CARTESIAN_POINT('Ctrl Pts',(121.648526737398,-24.1683568810269,-29.3613321441074));
#73913=CARTESIAN_POINT('Ctrl Pts',(121.756617543138,-24.1025001723946,-29.2755062523583));
#73914=CARTESIAN_POINT('Ctrl Pts',(121.544995916356,-24.4223128317953,-29.5810525234115));
#73915=CARTESIAN_POINT('Ctrl Pts',(121.653093466012,-24.3564659757563,-29.4952268701867));
#73916=CARTESIAN_POINT('Ctrl Pts',(121.761190817463,-24.2906189537557,-29.409401077777));
#73917=CARTESIAN_POINT('Ctrl Pts',(121.869287710261,-24.2247717885901,-29.3235748067435));
#73918=CARTESIAN_POINT('Ctrl Pts',(121.589544531169,-24.577280943507,-29.518244332399));
#73919=CARTESIAN_POINT('Ctrl Pts',(121.697637909658,-24.5114422368762,-29.4324068897941));
#73920=CARTESIAN_POINT('Ctrl Pts',(121.805730586269,-24.4456032016902,-29.3465688074238));
#73921=CARTESIAN_POINT('Ctrl Pts',(121.913823234176,-24.3797643238856,-29.2607305411384));
#73922=CARTESIAN_POINT('Ctrl Pts',(121.587867965644,-24.6397181974285,-29.4682231323184));
#73923=CARTESIAN_POINT('Ctrl Pts',(121.695956395477,-24.573879640517,-29.3823793561953));
#73924=CARTESIAN_POINT('Ctrl Pts',(121.804044421868,-24.5080409992732,-29.2965351197829));
#73925=CARTESIAN_POINT('Ctrl Pts',(121.912132034353,-24.4422022714329,-29.2106904110617));
#73926=CARTESIAN_POINT('',(121.699999999997,-24.068064362549,-29.2306286312331));
#73927=CARTESIAN_POINT('Origin',(121.699999999997,-24.3060703646363,-29.0480002025304));
#73928=CARTESIAN_POINT('',(121.375735931288,-24.2656386875623,-29.4881125046124));
#73929=CARTESIAN_POINT('Origin',(121.375735931288,-24.5036446896497,-29.3054840759098));
#73930=CARTESIAN_POINT('Ctrl Pts',(121.375735931288,-24.2656386875623,-29.4881125046124));
#73931=CARTESIAN_POINT('Ctrl Pts',(121.483824361121,-24.1997808267293,-29.4022848693738));
#73932=CARTESIAN_POINT('Ctrl Pts',(121.591912387512,-24.1339227205117,-29.3164569143438));
#73933=CARTESIAN_POINT('Ctrl Pts',(121.699999999997,-24.068064362549,-29.2306286312331));
#73934=CARTESIAN_POINT('Origin',(121.375735931288,0.,0.));
#73935=CARTESIAN_POINT('',(121.375735931288,-24.6960816898302,-29.5356318566107));
#73936=CARTESIAN_POINT('Origin',(121.375735931288,0.,0.));
#73937=CARTESIAN_POINT('Origin',(121.375735931288,-24.5036446896497,-29.3054840759098));
#73938=CARTESIAN_POINT('Origin',(121.375735931288,-24.5036446896497,-29.3054840759098));
#73939=CARTESIAN_POINT('Origin',(121.375735931288,-24.5036446896497,-29.3054840759098));
#73940=CARTESIAN_POINT('Origin',(121.7,-6.64499443910137,-6.03163794469829));
#73941=CARTESIAN_POINT('Origin',(121.7,-24.3060703646348,-29.0480002025284));
#73942=CARTESIAN_POINT('',(121.7,-23.2511515011969,-28.1660070629187));
#73943=CARTESIAN_POINT('',(121.7,-6.406988437014,-6.21426637340091));
#73944=CARTESIAN_POINT('Origin',(121.7,-23.3065290745817,-27.7453726321288));
#73945=CARTESIAN_POINT('Origin',(121.7,-24.3060703646347,-29.0480002025285));
#73946=CARTESIAN_POINT('Origin',(113.,-25.7740421742497,-27.6125198053347));
#73947=CARTESIAN_POINT('',(104.3,-24.8901586977665,-26.7286363288515));
#73948=CARTESIAN_POINT('',(103.5,-24.8901586977665,-26.7286363288515));
#73949=CARTESIAN_POINT('Origin',(104.3,-24.6780266634105,-26.5165042944955));
#73950=CARTESIAN_POINT('',(104.087868515434,-25.9972587850772,-27.8357364161622));
#73951=CARTESIAN_POINT('Ctrl Pts',(104.087868240379,-25.9972589794574,-27.8357366105424));
#73952=CARTESIAN_POINT('Ctrl Pts',(104.061688713442,-25.9787365142134,-27.8172141452984));
#73953=CARTESIAN_POINT('Ctrl Pts',(104.037012788768,-25.9526072839584,-27.7910849150434));
#73954=CARTESIAN_POINT('Ctrl Pts',(104.008670719845,-25.9042078449942,-27.7426854760792));
#73955=CARTESIAN_POINT('Ctrl Pts',(104.,-25.8733711201675,-27.7118487512525));
#73956=CARTESIAN_POINT('Ctrl Pts',(104.,-25.8471708459779,-27.6856484770629));
#73957=CARTESIAN_POINT('',(104.25,-26.1119693309588,-27.9504469620438));
#73958=CARTESIAN_POINT('Ctrl Pts',(104.624264068712,-17.9574056939141,-33.7031390339859));
#73959=CARTESIAN_POINT('Ctrl Pts',(104.516175638879,-17.9033140106252,-33.6094494902625));
#73960=CARTESIAN_POINT('Ctrl Pts',(104.408087612488,-17.8492221257921,-33.5157595974544));
#73961=CARTESIAN_POINT('Ctrl Pts',(104.300000000003,-17.7951300341907,-33.4220693465131));
#73962=CARTESIAN_POINT('Ctrl Pts',(104.567655925523,-17.9856849271578,-33.752120102763));
#73963=CARTESIAN_POINT('Ctrl Pts',(104.459564357693,-17.9315947959052,-33.6584329578312));
#73964=CARTESIAN_POINT('Ctrl Pts',(104.351473262602,-17.8775040493509,-33.5647456205277));
#73965=CARTESIAN_POINT('Ctrl Pts',(104.243382456862,-17.8234135359081,-33.4710578085036));
#73966=CARTESIAN_POINT('Ctrl Pts',(104.455001570347,-17.9833187182834,-33.8834541246487));
#73967=CARTESIAN_POINT('Ctrl Pts',(104.346904020691,-17.9292246547841,-33.789775506513));
#73968=CARTESIAN_POINT('Ctrl Pts',(104.238806667407,-17.8751305285007,-33.6960966825317));
#73969=CARTESIAN_POINT('Ctrl Pts',(104.130709774609,-17.8210360125183,-33.6024175423752));
#73970=CARTESIAN_POINT('Ctrl Pts',(104.410455468831,-17.8659835447084,-34.0025898869996));
#73971=CARTESIAN_POINT('Ctrl Pts',(104.302362090342,-17.8118754705987,-33.908914286335));
#73972=CARTESIAN_POINT('Ctrl Pts',(104.194269413732,-17.7577669311554,-33.8152381372974));
#73973=CARTESIAN_POINT('Ctrl Pts',(104.086176765824,-17.7036581615694,-33.72156206328));
#73974=CARTESIAN_POINT('Ctrl Pts',(104.412132034356,-17.7958762791241,-34.041132103426));
#73975=CARTESIAN_POINT('Ctrl Pts',(104.304043604523,-17.7417622963114,-33.9474542173515));
#73976=CARTESIAN_POINT('Ctrl Pts',(104.195955578132,-17.6876479205195,-33.8537760772191));
#73977=CARTESIAN_POINT('Ctrl Pts',(104.087867965647,-17.63353314151,-33.7600976763371));
#73978=CARTESIAN_POINT('',(104.300000000003,-17.7951300341907,-33.4220693465131));
#73979=CARTESIAN_POINT('Origin',(104.300000000003,-17.5353224130554,-33.5720693465132));
#73980=CARTESIAN_POINT('',(104.624264068712,-17.9574056939141,-33.7031390339859));
#73981=CARTESIAN_POINT('Origin',(104.624264068712,-17.6975980727788,-33.8531390339859));
#73982=CARTESIAN_POINT('Ctrl Pts',(104.624264068712,-17.9574056939141,-33.7031390339859));
#73983=CARTESIAN_POINT('Ctrl Pts',(104.516175638879,-17.9033140106252,-33.6094494902625));
#73984=CARTESIAN_POINT('Ctrl Pts',(104.408087612488,-17.8492221257921,-33.5157595974544));
#73985=CARTESIAN_POINT('Ctrl Pts',(104.300000000003,-17.7951300341907,-33.4220693465131));
#73986=CARTESIAN_POINT('Origin',(104.3,-3.3018593539449,-8.9189881604791));
#73987=CARTESIAN_POINT('Origin',(104.3,-17.5353224130539,-33.5720693465106));
#73988=CARTESIAN_POINT('',(104.3,-17.1241669750802,-32.259927238132));
#73989=CARTESIAN_POINT('',(104.3,-3.56166697508023,-8.7689881604791));
#73990=CARTESIAN_POINT('Origin',(104.3,-16.7143593539449,-32.1501196169967));
#73991=CARTESIAN_POINT('Origin',(104.3,-17.5353224130539,-33.5720693465106));
#73992=CARTESIAN_POINT('Origin',(104.624264068712,-17.6975980727788,-33.8531390339859));
#73993=CARTESIAN_POINT('Origin',(104.624264068712,-17.6975980727788,-33.8531390339859));
#73994=CARTESIAN_POINT('Origin',(113.,-15.6473429640468,-34.3789638902265));
#73995=CARTESIAN_POINT('',(121.7,-15.1689886735905,-33.2241144745873));
#73996=CARTESIAN_POINT('',(103.5,-15.1689886735905,-33.2241144745873));
#73997=CARTESIAN_POINT('Origin',(121.7,-15.0541836438809,-32.946950614834));
#73998=CARTESIAN_POINT('',(121.912131484566,-15.7681469233145,-34.6706104470789));
#73999=CARTESIAN_POINT('Ctrl Pts',(121.912131759621,-15.7681470285124,-34.6706107010489));
#74000=CARTESIAN_POINT('Ctrl Pts',(121.938311286558,-15.7581227425572,-34.6464099339428));
#74001=CARTESIAN_POINT('Ctrl Pts',(121.962987211232,-15.7439817050434,-34.612270449391));
#74002=CARTESIAN_POINT('Ctrl Pts',(121.991329280155,-15.7177881174267,-34.5490335349196));
#74003=CARTESIAN_POINT('Ctrl Pts',(122.,-15.7010994022092,-34.5087434123029));
#74004=CARTESIAN_POINT('Ctrl Pts',(122.,-15.686919915995,-34.4745111043772));
#74005=CARTESIAN_POINT('',(121.75,-15.8302278233913,-34.8204869980086));
#74006=CARTESIAN_POINT('Ctrl Pts',(121.375735931288,-11.1339148195199,-36.529521496889));
#74007=CARTESIAN_POINT('Ctrl Pts',(121.483824361121,-11.1059149038863,-36.4250243891369));
#74008=CARTESIAN_POINT('Ctrl Pts',(121.591912387511,-11.0779148839259,-36.3205268920315));
#74009=CARTESIAN_POINT('Ctrl Pts',(121.699999999996,-11.0499147569342,-36.2160289954803));
#74010=CARTESIAN_POINT('Ctrl Pts',(121.432344074477,-11.1485532278086,-36.5841527803644));
#74011=CARTESIAN_POINT('Ctrl Pts',(121.540435642307,-11.1205539109214,-36.4796584662696));
#74012=CARTESIAN_POINT('Ctrl Pts',(121.648526737397,-11.0925548930909,-36.3751635810634));
#74013=CARTESIAN_POINT('Ctrl Pts',(121.756617543136,-11.0645553747475,-36.2706685250137));
#74014=CARTESIAN_POINT('Ctrl Pts',(121.544996634179,-11.2430954833528,-36.6753444250015));
#74015=CARTESIAN_POINT('Ctrl Pts',(121.653094183835,-11.2151049763392,-36.5708533597438));
#74016=CARTESIAN_POINT('Ctrl Pts',(121.761191535808,-11.1871143689483,-36.4663621029995));
#74017=CARTESIAN_POINT('Ctrl Pts',(121.869288428606,-11.1591238127642,-36.3618703486634));
#74018=CARTESIAN_POINT('Ctrl Pts',(121.589544531169,-11.410303769972,-36.6766200040331));
#74019=CARTESIAN_POINT('Ctrl Pts',(121.697637909657,-11.3823253036304,-36.5721211654519));
#74020=CARTESIAN_POINT('Ctrl Pts',(121.805730586267,-11.354346778571,-36.467621610072));
#74021=CARTESIAN_POINT('Ctrl Pts',(121.913823234175,-11.3263684692944,-36.3631219450038));
#74022=CARTESIAN_POINT('Ctrl Pts',(121.587867965644,-11.4871305554742,-36.6543001437251));
#74023=CARTESIAN_POINT('Ctrl Pts',(121.695956395477,-11.4591546511876,-36.5497955110311));
#74024=CARTESIAN_POINT('Ctrl Pts',(121.804044421867,-11.4311788451333,-36.4452904208128));
#74025=CARTESIAN_POINT('Ctrl Pts',(121.912132034352,-11.4032031398191,-36.3407848610989));
#74026=CARTESIAN_POINT('',(121.699999999996,-11.0499147569342,-36.2160289954803));
#74027=CARTESIAN_POINT('Origin',(121.699999999996,-11.3396925048209,-36.1383832819496));
#74028=CARTESIAN_POINT('',(121.375735931288,-11.1339148195199,-36.529521496889));
#74029=CARTESIAN_POINT('Origin',(121.375735931288,-11.4236925674066,-36.4518757833582));
#74030=CARTESIAN_POINT('Ctrl Pts',(121.375735931288,-11.1339148195199,-36.529521496889));
#74031=CARTESIAN_POINT('Ctrl Pts',(121.483824361121,-11.1059149038863,-36.4250243891369));
#74032=CARTESIAN_POINT('Ctrl Pts',(121.591912387511,-11.0779148839259,-36.3205268920315));
#74033=CARTESIAN_POINT('Ctrl Pts',(121.699999999996,-11.0499147569342,-36.2160289954803));
#74034=CARTESIAN_POINT('Origin',(121.375735931288,0.,0.));
#74035=CARTESIAN_POINT('',(121.375735931288,-11.5134074305014,-36.7381470591438));
#74036=CARTESIAN_POINT('Origin',(121.375735931288,0.,0.));
#74037=CARTESIAN_POINT('Origin',(121.375735931288,-11.4236925674066,-36.4518757833582));
#74038=CARTESIAN_POINT('Origin',(121.375735931288,-11.4236925674066,-36.4518757833582));
#74039=CARTESIAN_POINT('Origin',(121.375735931288,-11.4236925674066,-36.4518757833582));
#74040=CARTESIAN_POINT('Origin',(121.7,-5.32540037959422,-13.6927394990421));
#74041=CARTESIAN_POINT('Origin',(121.7,-11.3396925048199,-36.1383832819455));
#74042=CARTESIAN_POINT('',(121.7,-10.7025987204178,-34.9198279009177));
#74043=CARTESIAN_POINT('',(121.7,-5.0356226317075,-13.7703852125729));
#74044=CARTESIAN_POINT('Origin',(121.7,-10.9147307547738,-34.5524044395002));
#74045=CARTESIAN_POINT('Origin',(121.7,-11.3396925048197,-36.1383832819456));
#74046=CARTESIAN_POINT('Origin',(113.,-13.2452561795175,-35.3739408143757));
#74047=CARTESIAN_POINT('',(104.3,-12.7669018890611,-34.2190913987366));
#74048=CARTESIAN_POINT('',(103.5,-12.7669018890611,-34.2190913987366));
#74049=CARTESIAN_POINT('Origin',(104.3,-12.6520968593516,-33.9419275389832));
#74050=CARTESIAN_POINT('',(104.087868515434,-13.3660601387852,-35.6655873712282));
#74051=CARTESIAN_POINT('Ctrl Pts',(104.087868240379,-13.366060243983,-35.6655876251981));
#74052=CARTESIAN_POINT('Ctrl Pts',(104.061688713442,-13.3560359580278,-35.6413868580921));
#74053=CARTESIAN_POINT('Ctrl Pts',(104.037012788768,-13.341894920514,-35.6072473735402));
#74054=CARTESIAN_POINT('Ctrl Pts',(104.008670719845,-13.3157013328973,-35.5440104590688));
#74055=CARTESIAN_POINT('Ctrl Pts',(104.,-13.2990126176798,-35.5037203364521));
#74056=CARTESIAN_POINT('Ctrl Pts',(104.,-13.2848331314657,-35.4694880285264));
#74057=CARTESIAN_POINT('',(104.25,-13.428141038862,-35.8154639221579));
#74058=CARTESIAN_POINT('Origin',(113.,-8.33272992328159,-37.2800967276863));
#74059=CARTESIAN_POINT('',(121.811388243054,-8.62250767116831,-37.2024510141556));
#74060=CARTESIAN_POINT('Ctrl Pts',(121.5,-8.3981702106372,-37.5728723564378));
#74061=CARTESIAN_POINT('Ctrl Pts',(121.5,-8.41846306187314,-37.5683365621785));
#74062=CARTESIAN_POINT('Ctrl Pts',(121.502178291748,-8.43844642422117,-37.5616201820783));
#74063=CARTESIAN_POINT('Ctrl Pts',(121.510716614322,-8.47626683430668,-37.5443504602797));
#74064=CARTESIAN_POINT('Ctrl Pts',(121.517077828304,-8.49410315611484,-37.533796113814));
#74065=CARTESIAN_POINT('Ctrl Pts',(121.541159186122,-8.54274436268675,-37.4980708374905));
#74066=CARTESIAN_POINT('Ctrl Pts',(121.56412779323,-8.56856437653817,-37.4686076043297));
#74067=CARTESIAN_POINT('Ctrl Pts',(121.617288389766,-8.60866399825101,-37.4048701574215));
#74068=CARTESIAN_POINT('Ctrl Pts',(121.652509215907,-8.62308008690725,-37.3653949038344));
#74069=CARTESIAN_POINT('Ctrl Pts',(121.726559498935,-8.63532117790985,-37.2865621995426));
#74070=CARTESIAN_POINT('Ctrl Pts',(121.765406035132,-8.63305961883984,-37.2472073755322));
#74071=CARTESIAN_POINT('Ctrl Pts',(121.804557793905,-8.6242194708842,-37.2090666886064));
#74072=CARTESIAN_POINT('Ctrl Pts',(121.807962616873,-8.62339502798058,-37.2057626944961));
#74073=CARTESIAN_POINT('Ctrl Pts',(121.811388687965,-8.6225077862527,-37.2024514436577));
#74074=CARTESIAN_POINT('',(113.,-8.62250767116831,-37.2024510141556));
#74075=CARTESIAN_POINT('Origin',(113.,-8.5147153784444,-36.8001647010456));
#74076=CARTESIAN_POINT('',(121.912131484566,-8.59641832855394,-37.1050842619827));
#74077=CARTESIAN_POINT('',(121.75,-8.6384053024286,-37.261781781739));
#74078=CARTESIAN_POINT('Ctrl Pts',(122.,-8.54148233004195,-36.9000603243714));
#74079=CARTESIAN_POINT('Ctrl Pts',(122.,-8.55107229598146,-36.9358505645005));
#74080=CARTESIAN_POINT('Ctrl Pts',(121.991329280155,-8.56235932063755,-36.9779743139833));
#74081=CARTESIAN_POINT('Ctrl Pts',(121.962987211232,-8.58007474482737,-37.0440891771373));
#74082=CARTESIAN_POINT('Ctrl Pts',(121.938311286558,-8.58963870688201,-37.0797823694469));
#74083=CARTESIAN_POINT('Ctrl Pts',(121.912131759621,-8.59641839970203,-37.105084527511));
#74084=CARTESIAN_POINT('',(121.7,-8.19119157206625,-35.5927574181843));
#74085=CARTESIAN_POINT('Origin',(121.7,-8.11354585853549,-35.3029796702975));
#74086=CARTESIAN_POINT('',(103.5,-8.19119157206625,-35.5927574181843));
#74087=CARTESIAN_POINT('Ctrl Pts',(104.624264068712,11.1339148195198,-36.529521496889));
#74088=CARTESIAN_POINT('Ctrl Pts',(104.516175638879,11.1059149038863,-36.4250243891369));
#74089=CARTESIAN_POINT('Ctrl Pts',(104.408087612489,11.0779148839258,-36.3205268920315));
#74090=CARTESIAN_POINT('Ctrl Pts',(104.300000000004,11.0499147569342,-36.2160289954803));
#74091=CARTESIAN_POINT('Ctrl Pts',(104.567655925523,11.1485532278086,-36.5841527803644));
#74092=CARTESIAN_POINT('Ctrl Pts',(104.459564357693,11.1205539109213,-36.4796584662696));
#74093=CARTESIAN_POINT('Ctrl Pts',(104.351473262603,11.0925548930909,-36.3751635810634));
#74094=CARTESIAN_POINT('Ctrl Pts',(104.243382456864,11.0645553747475,-36.2706685250137));
#74095=CARTESIAN_POINT('Ctrl Pts',(104.455001016882,11.2430929770909,-36.6753475262196));
#74096=CARTESIAN_POINT('Ctrl Pts',(104.346903467226,11.2151024700773,-36.5708564609618));
#74097=CARTESIAN_POINT('Ctrl Pts',(104.238806113538,11.1871118616628,-36.4663652062277));
#74098=CARTESIAN_POINT('Ctrl Pts',(104.130709220741,11.1591213054787,-36.3618734518916));
#74099=CARTESIAN_POINT('Ctrl Pts',(104.410455468831,11.410303769972,-36.6766200040331));
#74100=CARTESIAN_POINT('Ctrl Pts',(104.302362090343,11.3823253036304,-36.5721211654519));
#74101=CARTESIAN_POINT('Ctrl Pts',(104.194269413733,11.354346778571,-36.4676216100719));
#74102=CARTESIAN_POINT('Ctrl Pts',(104.086176765825,11.3263684692943,-36.3631219450038));
#74103=CARTESIAN_POINT('Ctrl Pts',(104.412132034356,11.4871305554741,-36.6543001437251));
#74104=CARTESIAN_POINT('Ctrl Pts',(104.304043604523,11.4591546511876,-36.5497955110311));
#74105=CARTESIAN_POINT('Ctrl Pts',(104.195955578133,11.4311788451333,-36.4452904208128));
#74106=CARTESIAN_POINT('Ctrl Pts',(104.087867965648,11.403203139819,-36.3407848610989));
#74107=CARTESIAN_POINT('',(104.300000000004,11.0499147569342,-36.2160289954803));
#74108=CARTESIAN_POINT('Origin',(104.300000000004,11.3396925048209,-36.1383832819496));
#74109=CARTESIAN_POINT('',(104.624264068712,11.1339148195198,-36.529521496889));
#74110=CARTESIAN_POINT('Origin',(104.624264068712,11.4236925674066,-36.4518757833583));
#74111=CARTESIAN_POINT('Ctrl Pts',(104.624264068712,11.1339148195198,-36.529521496889));
#74112=CARTESIAN_POINT('Ctrl Pts',(104.516175638879,11.1059149038863,-36.4250243891369));
#74113=CARTESIAN_POINT('Ctrl Pts',(104.408087612489,11.0779148839258,-36.3205268920315));
#74114=CARTESIAN_POINT('Ctrl Pts',(104.300000000004,11.0499147569342,-36.2160289954803));
#74115=CARTESIAN_POINT('Origin',(104.3,7.70344946242041,-22.5677394990421));
#74116=CARTESIAN_POINT('Origin',(104.3,11.3396925048198,-36.1383832819455));
#74117=CARTESIAN_POINT('',(104.3,10.7025987204178,-34.9198279009177));
#74118=CARTESIAN_POINT('',(104.3,7.41367171453369,-22.6453852125729));
#74119=CARTESIAN_POINT('Origin',(104.3,10.9147307547737,-34.5524044395003));
#74120=CARTESIAN_POINT('Origin',(104.3,11.3396925048198,-36.1383832819455));
#74121=CARTESIAN_POINT('Origin',(104.624264068712,11.4236925674066,-36.4518757833583));
#74122=CARTESIAN_POINT('Origin',(104.624264068712,11.4236925674066,-36.4518757833583));
#74123=CARTESIAN_POINT('Origin',(113.,13.2452561795174,-35.3739408143757));
#74124=CARTESIAN_POINT('',(121.7,12.7669018890611,-34.2190913987366));
#74125=CARTESIAN_POINT('',(103.5,12.7669018890611,-34.2190913987366));
#74126=CARTESIAN_POINT('Origin',(121.7,12.6520968593516,-33.9419275389832));
#74127=CARTESIAN_POINT('',(121.912131484566,13.3660601387852,-35.6655873712282));
#74128=CARTESIAN_POINT('Ctrl Pts',(121.912131759621,13.366060243983,-35.6655876251982));
#74129=CARTESIAN_POINT('Ctrl Pts',(121.938311286558,13.3560359580278,-35.6413868580921));
#74130=CARTESIAN_POINT('Ctrl Pts',(121.962987211232,13.341894920514,-35.6072473735403));
#74131=CARTESIAN_POINT('Ctrl Pts',(121.991329280155,13.3157013328973,-35.5440104590688));
#74132=CARTESIAN_POINT('Ctrl Pts',(122.,13.2990126176798,-35.5037203364522));
#74133=CARTESIAN_POINT('Ctrl Pts',(122.,13.2848331314656,-35.4694880285265));
#74134=CARTESIAN_POINT('',(121.75,13.4281410388619,-35.8154639221579));
#74135=CARTESIAN_POINT('Ctrl Pts',(104.624264068712,6.27060329017722,-37.6702738824291));
#74136=CARTESIAN_POINT('Ctrl Pts',(104.51617563888,6.25648252727636,-37.56301603955));
#74137=CARTESIAN_POINT('Ctrl Pts',(104.408087612489,6.24236171176192,-37.4557577970312));
#74138=CARTESIAN_POINT('Ctrl Pts',(104.300000000005,6.22824084227012,-37.3484991445136));
#74139=CARTESIAN_POINT('Ctrl Pts',(104.567655925523,6.27798565144562,-37.7263484833951));
#74140=CARTESIAN_POINT('Ctrl Pts',(104.459564357694,6.26386511752329,-37.6190934884253));
#74141=CARTESIAN_POINT('Ctrl Pts',(104.351473262604,6.24974495464426,-37.5118379662647));
#74142=CARTESIAN_POINT('Ctrl Pts',(104.243382456865,6.23562431783375,-37.4045822093923));
#74143=CARTESIAN_POINT('Ctrl Pts',(104.455000447563,6.35981259677795,-37.8291036249763));
#74144=CARTESIAN_POINT('Ctrl Pts',(104.346902897908,6.34570037330132,-37.7218530009686));
#74145=CARTESIAN_POINT('Ctrl Pts',(104.238805543805,6.33158807371323,-37.6146021763207));
#74146=CARTESIAN_POINT('Ctrl Pts',(104.130708651008,6.31747589142946,-37.5073508627117));
#74147=CARTESIAN_POINT('Ctrl Pts',(104.410455468831,6.52542748682473,-37.8521899387271));
#74148=CARTESIAN_POINT('Ctrl Pts',(104.302362090343,6.51132821563267,-37.7449331795208));
#74149=CARTESIAN_POINT('Ctrl Pts',(104.194269413733,6.49722897978621,-37.6376757019839));
#74150=CARTESIAN_POINT('Ctrl Pts',(104.086176765826,6.48312997219361,-37.5304181438624));
#74151=CARTESIAN_POINT('Ctrl Pts',(104.412132034356,6.60451033490358,-37.8400889356902));
#74152=CARTESIAN_POINT('Ctrl Pts',(104.304043604524,6.59041436013136,-37.7328267663559));
#74153=CARTESIAN_POINT('Ctrl Pts',(104.195955578133,6.57631854246989,-37.6255641562333));
#74154=CARTESIAN_POINT('Ctrl Pts',(104.087867965649,6.56222288596808,-37.5183010937809));
#74155=CARTESIAN_POINT('',(104.300000000005,6.22824084227012,-37.3484991445136));
#74156=CARTESIAN_POINT('Origin',(104.300000000005,6.52567430068226,-37.3093412868476));
#74157=CARTESIAN_POINT('',(104.624264068712,6.27060329017722,-37.6702738824291));
#74158=CARTESIAN_POINT('Origin',(104.624264068712,6.56803674858936,-37.6311160247631));
#74159=CARTESIAN_POINT('Ctrl Pts',(104.624264068712,6.27060329017722,-37.6702738824291));
#74160=CARTESIAN_POINT('Ctrl Pts',(104.51617563888,6.25648252727636,-37.56301603955));
#74161=CARTESIAN_POINT('Ctrl Pts',(104.408087612489,6.24236171176192,-37.4557577970312));
#74162=CARTESIAN_POINT('Ctrl Pts',(104.300000000005,6.22824084227012,-37.3484991445136));
#74163=CARTESIAN_POINT('Origin',(104.3,4.37369830660541,-20.9634607793525));
#74164=CARTESIAN_POINT('Origin',(104.3,6.52567430068159,-37.3093412868425));
#74165=CARTESIAN_POINT('',(104.3,6.05308433581782,-36.018053390258));
#74166=CARTESIAN_POINT('',(104.3,4.07626484819327,-21.0026186370185));
#74167=CARTESIAN_POINT('Origin',(104.3,6.31135993656395,-35.6814620741799));
#74168=CARTESIAN_POINT('Origin',(104.3,6.52567430068159,-37.3093412868425));
#74169=CARTESIAN_POINT('Origin',(104.624264068712,6.56803674858936,-37.6311160247631));
#74170=CARTESIAN_POINT('Origin',(104.624264068712,6.56803674858936,-37.6311160247631));
#74171=CARTESIAN_POINT('Origin',(113.,8.51471537844435,-36.8001647010456));
#74172=CARTESIAN_POINT('',(121.7,8.1911915720662,-35.5927574181843));
#74173=CARTESIAN_POINT('',(103.5,8.1911915720662,-35.5927574181843));
#74174=CARTESIAN_POINT('Origin',(121.7,8.11354585853545,-35.3029796702976));
#74175=CARTESIAN_POINT('',(121.912131484566,8.5964183285539,-37.1050842619827));
#74176=CARTESIAN_POINT('Ctrl Pts',(121.912131759621,8.59641839970199,-37.105084527511));
#74177=CARTESIAN_POINT('Ctrl Pts',(121.938311286558,8.58963870688196,-37.0797823694469));
#74178=CARTESIAN_POINT('Ctrl Pts',(121.962987211232,8.58007474482732,-37.0440891771374));
#74179=CARTESIAN_POINT('Ctrl Pts',(121.991329280155,8.5623593206375,-36.9779743139833));
#74180=CARTESIAN_POINT('Ctrl Pts',(122.,8.55107229598141,-36.9358505645005));
#74181=CARTESIAN_POINT('Ctrl Pts',(122.,8.54148233004191,-36.9000603243714));
#74182=CARTESIAN_POINT('',(121.75,8.63840530242855,-37.261781781739));
#74183=CARTESIAN_POINT('Origin',(104.3,-1.6,-18.875));
#74184=CARTESIAN_POINT('',(104.3,-1.30000000000001,-37.8419261182179));
#74185=CARTESIAN_POINT('Origin',(104.3,-1.60000000000001,-37.8419261182179));
#74186=CARTESIAN_POINT('',(104.3,-1.30000000000001,-36.5));
#74187=CARTESIAN_POINT('Origin',(104.3,-1.60000000000001,-36.2));
#74188=CARTESIAN_POINT('',(104.3,-1.3,-18.875));
#74189=CARTESIAN_POINT('Ctrl Pts',(104.300000000006,-1.30000000000001,-37.8419261182243));
#74190=CARTESIAN_POINT('Ctrl Pts',(104.408087612492,-1.30000000000001,-37.9501103014279));
#74191=CARTESIAN_POINT('Ctrl Pts',(104.516175638884,-1.30000000000001,-38.0582940710949));
#74192=CARTESIAN_POINT('Ctrl Pts',(104.624264068718,-1.30000000000001,-38.1664774376737));
#74193=CARTESIAN_POINT('Ctrl Pts',(104.243382456866,-1.30000000000001,-37.8984931216591));
#74194=CARTESIAN_POINT('Ctrl Pts',(104.351473262606,-1.30000014726687,-38.0066744036192));
#74195=CARTESIAN_POINT('Ctrl Pts',(104.459564357698,-1.29999985529285,-38.1148553910149));
#74196=CARTESIAN_POINT('Ctrl Pts',(104.567655925529,-1.30000000000001,-38.223035904161));
#74197=CARTESIAN_POINT('Ctrl Pts',(104.130707929307,-1.36773633088589,-38.0110670701893));
#74198=CARTESIAN_POINT('Ctrl Pts',(104.238804822106,-1.36772867591792,-38.1192428433615));
#74199=CARTESIAN_POINT('Ctrl Pts',(104.346902176736,-1.36772120153624,-38.2274181465522));
#74200=CARTESIAN_POINT('Ctrl Pts',(104.454999726393,-1.36771367741974,-38.3355932413996));
#74201=CARTESIAN_POINT('Ctrl Pts',(104.086176765827,-1.52896332380521,-38.0555584828822));
#74202=CARTESIAN_POINT('Ctrl Pts',(104.194269413736,-1.52894179178495,-38.1637387275019));
#74203=CARTESIAN_POINT('Ctrl Pts',(104.302362090347,-1.5289204965842,-38.2719189220196));
#74204=CARTESIAN_POINT('Ctrl Pts',(104.410455468836,-1.52889933018763,-38.3800984089656));
#74205=CARTESIAN_POINT('Ctrl Pts',(104.08786796565,-1.60896117914608,-38.0538687927104));
#74206=CARTESIAN_POINT('Ctrl Pts',(104.195955578136,-1.60893560624471,-38.1620540571656));
#74207=CARTESIAN_POINT('Ctrl Pts',(104.304043604528,-1.60891025216514,-38.2702388941964));
#74208=CARTESIAN_POINT('Ctrl Pts',(104.412132034362,-1.60888511138664,-38.3784233147169));
#74209=CARTESIAN_POINT('',(104.624264068718,-1.30000000000001,-38.1664774376737));
#74210=CARTESIAN_POINT('',(104.412132034362,-1.60888511138652,-38.378423314714));
#74211=CARTESIAN_POINT('Origin',(104.624264068718,-1.60000000000001,-38.1664774376737));
#74212=CARTESIAN_POINT('',(104.08786796565,-1.60896117914594,-38.0538687927072));
#74213=CARTESIAN_POINT('Ctrl Pts',(104.412132034362,-1.60888511138664,-38.3784233147169));
#74214=CARTESIAN_POINT('Ctrl Pts',(104.304043604528,-1.60891025216514,-38.2702388941964));
#74215=CARTESIAN_POINT('Ctrl Pts',(104.195955578136,-1.60893560624471,-38.1620540571656));
#74216=CARTESIAN_POINT('Ctrl Pts',(104.08786796565,-1.60896117914608,-38.0538687927104));
#74217=CARTESIAN_POINT('Origin',(104.300000000006,-1.60000000000001,-37.8419261182243));
#74218=CARTESIAN_POINT('Ctrl Pts',(104.300000000006,-1.30000000000001,-37.8419261182243));
#74219=CARTESIAN_POINT('Ctrl Pts',(104.408087612492,-1.30000000000001,-37.9501103014279));
#74220=CARTESIAN_POINT('Ctrl Pts',(104.516175638884,-1.30000000000001,-38.0582940710949));
#74221=CARTESIAN_POINT('Ctrl Pts',(104.624264068718,-1.30000000000001,-38.1664774376737));
#74222=CARTESIAN_POINT('Origin',(104.3,-1.60000000000001,-37.8419261182179));
#74223=CARTESIAN_POINT('Origin',(104.3,-1.60000000000001,-37.8419261182179));
#74224=CARTESIAN_POINT('Origin',(113.,-1.60000000000001,-38.1664774376677));
#74225=CARTESIAN_POINT('',(121.811388243054,-1.30000000000001,-38.1664774376677));
#74226=CARTESIAN_POINT('',(121.5,-1.61256544502618,-38.4662141714714));
#74227=CARTESIAN_POINT('Ctrl Pts',(121.811388687965,-1.30000000000033,-38.1664778823209));
#74228=CARTESIAN_POINT('Ctrl Pts',(121.80796264376,-1.30000000508128,-38.1699059131779));
#74229=CARTESIAN_POINT('Ctrl Pts',(121.80455782351,-1.3000587899814,-38.1733107052584));
#74230=CARTESIAN_POINT('Ctrl Pts',(121.765406035132,-1.30139139994018,-38.2124398080324));
#74231=CARTESIAN_POINT('Ctrl Pts',(121.726559498935,-1.30939267959732,-38.2510389834921));
#74232=CARTESIAN_POINT('Ctrl Pts',(121.652509215907,-1.34162007078635,-38.3240173010395));
#74233=CARTESIAN_POINT('Ctrl Pts',(121.617288389766,-1.36576189057207,-38.3584163096784));
#74234=CARTESIAN_POINT('Ctrl Pts',(121.56412779323,-1.42099161595499,-38.4096034099481));
#74235=CARTESIAN_POINT('Ctrl Pts',(121.541159186122,-1.45355748004153,-38.4313799964546));
#74236=CARTESIAN_POINT('Ctrl Pts',(121.517077828304,-1.50978765959527,-38.4532986928691));
#74237=CARTESIAN_POINT('Ctrl Pts',(121.510716614322,-1.52974788934973,-38.4588770289215));
#74238=CARTESIAN_POINT('Ctrl Pts',(121.502178291748,-1.57074933311724,-38.4657696567958));
#74239=CARTESIAN_POINT('Ctrl Pts',(121.5,-1.59179010598938,-38.4670851070329));
#74240=CARTESIAN_POINT('Ctrl Pts',(121.5,-1.61256544502619,-38.4662141714714));
#74241=CARTESIAN_POINT('',(104.624264068712,-1.61256544502618,-38.4662141714714));
#74242=CARTESIAN_POINT('',(113.,-1.61256544502618,-38.4662141714714));
#74243=CARTESIAN_POINT('Origin',(104.624264068712,-1.60000000000001,-38.1664774376677));
#74244=CARTESIAN_POINT('',(113.,-1.30000000000001,-38.1664774376677));
#74245=CARTESIAN_POINT('Origin',(104.624264068712,-1.59999999999976,-38.1664774376677));
#74246=CARTESIAN_POINT('Origin',(104.624264068712,-1.59999999999976,-38.1664774376677));
#74247=CARTESIAN_POINT('Origin',(104.3,0.,0.));
#74248=CARTESIAN_POINT('',(104.087867965649,-3.37183029953928,-37.938324246066));
#74249=CARTESIAN_POINT('Origin',(104.087867965644,2.22044604925031E-15,
0.));
#74250=CARTESIAN_POINT('Origin',(104.3,-3.35305074428544,-37.7270251019467));
#74251=CARTESIAN_POINT('Origin',(104.25,0.,0.));
#74252=CARTESIAN_POINT('',(104.412132034356,-3.4142685824534,-38.2600922303079));
#74253=CARTESIAN_POINT('Origin',(104.412132034356,2.4980018054066E-15,0.));
#74254=CARTESIAN_POINT('Ctrl Pts',(104.087867965649,-3.37183029953951,-37.9383242460686));
#74255=CARTESIAN_POINT('Ctrl Pts',(104.195955578133,-3.3859766642846,-38.0455806326541));
#74256=CARTESIAN_POINT('Ctrl Pts',(104.304043604524,-3.40012275628988,-38.1528366240338));
#74257=CARTESIAN_POINT('Ctrl Pts',(104.412132034356,-3.4142685824534,-38.2600922303079));
#74258=CARTESIAN_POINT('Origin',(104.624264068712,0.,0.));
#74259=CARTESIAN_POINT('',(104.624264068712,-3.42207874082301,-38.3476124040547));
#74260=CARTESIAN_POINT('Origin',(104.624264068712,0.,0.));
#74261=CARTESIAN_POINT('Origin',(104.624264068712,-3.39541319219322,-38.0487998398672));
#74262=CARTESIAN_POINT('Origin',(113.,0.,0.));
#74263=CARTESIAN_POINT('',(121.5,-3.42207874082301,-38.3476124040547));
#74264=CARTESIAN_POINT('Origin',(121.5,0.,0.));
#74265=CARTESIAN_POINT('',(113.,-3.42207874082301,-38.3476124040547));
#74266=CARTESIAN_POINT('Ctrl Pts',(104.624264068712,-3.69284665060536,-38.0096419822012));
#74267=CARTESIAN_POINT('Ctrl Pts',(104.51617563888,-3.6787258877045,-37.9023841393222));
#74268=CARTESIAN_POINT('Ctrl Pts',(104.408087612489,-3.66460507219007,-37.7951258968034));
#74269=CARTESIAN_POINT('Ctrl Pts',(104.300000000005,-3.65048420269827,-37.6878672442858));
#74270=CARTESIAN_POINT('Ctrl Pts',(104.567655925523,-3.70022901187376,-38.0657165831673));
#74271=CARTESIAN_POINT('Ctrl Pts',(104.459564357694,-3.68610876488976,-37.9584615504213));
#74272=CARTESIAN_POINT('Ctrl Pts',(104.351473262604,-3.67198802305846,-37.8512061044813));
#74273=CARTESIAN_POINT('Ctrl Pts',(104.243382456865,-3.65786767826191,-37.7439503091645));
#74274=CARTESIAN_POINT('Ctrl Pts',(104.45500004306,-3.64778584282862,-38.1861491282933));
#74275=CARTESIAN_POINT('Ctrl Pts',(104.346902493405,-3.63365869985872,-38.078900468474));
#74276=CARTESIAN_POINT('Ctrl Pts',(104.238805139007,-3.61953157877269,-37.9716515954047));
#74277=CARTESIAN_POINT('Ctrl Pts',(104.13070824621,-3.60540421753161,-37.8644022801433));
#74278=CARTESIAN_POINT('Ctrl Pts',(104.410455468831,-3.49378871788002,-38.2513127544414));
#74279=CARTESIAN_POINT('Ctrl Pts',(104.302362090343,-3.47964747605774,-38.1440615207735));
#74280=CARTESIAN_POINT('Ctrl Pts',(104.194269413733,-3.46550601417657,-38.0368096023995));
#74281=CARTESIAN_POINT('Ctrl Pts',(104.086176765826,-3.45136431096229,-37.9295576652633));
#74282=CARTESIAN_POINT('Ctrl Pts',(104.412132034356,-3.4142685824534,-38.2600922303079));
#74283=CARTESIAN_POINT('Ctrl Pts',(104.304043604524,-3.40012275628988,-38.1528366240338));
#74284=CARTESIAN_POINT('Ctrl Pts',(104.195955578133,-3.3859766642846,-38.0455806326541));
#74285=CARTESIAN_POINT('Ctrl Pts',(104.087867965649,-3.37183029953951,-37.9383242460686));
#74286=CARTESIAN_POINT('',(104.300000000005,-3.65048420269827,-37.6878672442858));
#74287=CARTESIAN_POINT('Origin',(104.300000000005,-3.35305074428613,-37.7270251019518));
#74288=CARTESIAN_POINT('',(104.624264068712,-3.69284665060536,-38.0096419822012));
#74289=CARTESIAN_POINT('Origin',(104.624264068712,-3.39541319219322,-38.0487998398672));
#74290=CARTESIAN_POINT('Ctrl Pts',(104.624264068712,-3.69284665060536,-38.0096419822012));
#74291=CARTESIAN_POINT('Ctrl Pts',(104.51617563888,-3.6787258877045,-37.9023841393222));
#74292=CARTESIAN_POINT('Ctrl Pts',(104.408087612489,-3.66460507219007,-37.7951258968034));
#74293=CARTESIAN_POINT('Ctrl Pts',(104.300000000005,-3.65048420269827,-37.6878672442858));
#74294=CARTESIAN_POINT('Origin',(104.3,-0.553665449701535,-16.4635827375088));
#74295=CARTESIAN_POINT('Origin',(104.3,-3.35305074428544,-37.7270251019467));
#74296=CARTESIAN_POINT('',(104.3,-3.47532769624596,-36.3574214900301));
#74297=CARTESIAN_POINT('',(104.3,-0.851098908113681,-16.4244248798428));
#74298=CARTESIAN_POINT('Origin',(104.3,-3.1387363801678,-36.099145889284));
#74299=CARTESIAN_POINT('Origin',(104.3,-3.35305074428544,-37.7270251019467));
#74300=CARTESIAN_POINT('Origin',(104.624264068712,-3.39541319219322,-38.0487998398672));
#74301=CARTESIAN_POINT('Origin',(104.624264068712,-3.39541319219322,-38.0487998398672));
#74302=CARTESIAN_POINT('Origin',(113.,-1.30000000000001,-37.75));
#74303=CARTESIAN_POINT('',(121.7,-1.30000000000001,-36.5));
#74304=CARTESIAN_POINT('',(103.5,-1.30000000000001,-36.5));
#74305=CARTESIAN_POINT('Origin',(121.7,-1.30000000000001,-36.2));
#74306=CARTESIAN_POINT('',(121.912131484566,-1.30000000000001,-38.0656759583793));
#74307=CARTESIAN_POINT('Ctrl Pts',(121.912131759621,-1.30000000000001,-38.0656762332744));
#74308=CARTESIAN_POINT('Ctrl Pts',(121.938311286558,-1.30000000000001,-38.0394815117177));
#74309=CARTESIAN_POINT('Ctrl Pts',(121.962987211232,-1.30000000000001,-38.0025291999168));
#74310=CARTESIAN_POINT('Ctrl Pts',(121.991329280155,-1.30000000000001,-37.9340820569223));
#74311=CARTESIAN_POINT('Ctrl Pts',(122.,-1.30000000000001,-37.8904723424532));
#74312=CARTESIAN_POINT('Ctrl Pts',(122.,-1.30000000000001,-37.8534195593564));
#74313=CARTESIAN_POINT('',(121.75,-1.30000000000001,-38.2279011681123));
#74314=CARTESIAN_POINT('Origin',(113.,6.56803674858936,-37.6311160247631));
#74315=CARTESIAN_POINT('',(121.811388243054,6.27060329017722,-37.6702738824291));
#74316=CARTESIAN_POINT('Ctrl Pts',(121.5,6.61961818902331,-37.9266483495649));
#74317=CARTESIAN_POINT('Ctrl Pts',(121.5,6.59913426579449,-37.9302235600485));
#74318=CARTESIAN_POINT('Ctrl Pts',(121.502178291748,6.57810179894056,-37.9316657356349));
#74319=CARTESIAN_POINT('Ctrl Pts',(121.510716614322,6.53655145973753,-37.930183837478));
#74320=CARTESIAN_POINT('Ctrl Pts',(121.517077828304,6.5160338735518,-37.9272585576496));
#74321=CARTESIAN_POINT('Ctrl Pts',(121.541159186122,6.4574237869977,-37.9128668899463));
#74322=CARTESIAN_POINT('Ctrl Pts',(121.56412779323,6.42229411347666,-37.8955273033918));
#74323=CARTESIAN_POINT('Ctrl Pts',(121.617288389766,6.36085562876168,-37.8519870416124));
#74324=CARTESIAN_POINT('Ctrl Pts',(121.652509215907,6.33243037397715,-37.8210334610709));
#74325=CARTESIAN_POINT('Ctrl Pts',(121.726559498935,6.29095311068321,-37.7528860018039));
#74326=CARTESIAN_POINT('Ctrl Pts',(121.765406035132,6.27798207968713,-37.7156614242077));
#74327=CARTESIAN_POINT('Ctrl Pts',(121.804557793905,6.27155350246219,-37.6770410460388));
#74328=CARTESIAN_POINT('Ctrl Pts',(121.807962616873,6.27105080457995,-37.6736730528646));
#74329=CARTESIAN_POINT('Ctrl Pts',(121.811388687965,6.27060334821644,-37.6702743232782));
#74330=CARTESIAN_POINT('',(113.,6.27060329017722,-37.6702738824291));
#74331=CARTESIAN_POINT('Origin',(113.,6.21624207609289,-37.2573594669753));
#74332=CARTESIAN_POINT('',(121.912131484566,6.25744605691555,-37.5703347737697));
#74333=CARTESIAN_POINT('',(121.75,6.2786206958241,-37.7311721243448));
#74334=CARTESIAN_POINT('Ctrl Pts',(122.,6.22974103737676,-37.3598942576648));
#74335=CARTESIAN_POINT('Ctrl Pts',(122.,6.23457739606554,-37.3966300490657));
#74336=CARTESIAN_POINT('Ctrl Pts',(121.991329280155,6.240269606039,-37.4398666763821));
#74337=CARTESIAN_POINT('Ctrl Pts',(121.962987211232,6.2492037509824,-37.5077282445796));
#74338=CARTESIAN_POINT('Ctrl Pts',(121.938311286558,6.25402699553551,-37.5443644242305));
#74339=CARTESIAN_POINT('Ctrl Pts',(121.912131759621,6.25744609279656,-37.570335046313));
#74340=CARTESIAN_POINT('',(121.7,6.05308433581782,-36.018053390258));
#74341=CARTESIAN_POINT('Origin',(121.7,6.01392647815181,-35.7206199318459));
#74342=CARTESIAN_POINT('',(103.5,6.05308433581782,-36.018053390258));
#74343=CARTESIAN_POINT('Origin',(113.,11.4236925674066,-36.4518757833583));
#74344=CARTESIAN_POINT('',(121.811388243054,11.1339148195198,-36.529521496889));
#74345=CARTESIAN_POINT('Ctrl Pts',(121.5,11.5134074305014,-36.7381470591438));
#74346=CARTESIAN_POINT('Ctrl Pts',(121.5,11.4935654086862,-36.7443653717069));
#74347=CARTESIAN_POINT('Ctrl Pts',(121.502178291748,11.4729011191897,-36.7485404970926));
#74348=CARTESIAN_POINT('Ctrl Pts',(121.510716614322,11.4315128223748,-36.7524946843416));
#74349=CARTESIAN_POINT('Ctrl Pts',(121.517077828304,11.410788941346,-36.7522725130859));
#74350=CARTESIAN_POINT('Ctrl Pts',(121.541159186122,11.3508017826222,-36.7456541195186));
#74351=CARTESIAN_POINT('Ctrl Pts',(121.56412779323,11.3137093781204,-36.7330482180494));
#74352=CARTESIAN_POINT('Ctrl Pts',(121.617288389766,11.2471133635808,-36.6978997807109));
#74353=CARTESIAN_POINT('Ctrl Pts',(121.652509215907,11.2148910377878,-36.6709212526118));
#74354=CARTESIAN_POINT('Ctrl Pts',(121.726559498935,11.1648735898636,-36.6087706735474));
#74355=CARTESIAN_POINT('Ctrl Pts',(121.765406035132,11.1471547454652,-36.5735576166579));
#74356=CARTESIAN_POINT('Ctrl Pts',(121.804557793905,11.1357401947051,-36.5361067388845));
#74357=CARTESIAN_POINT('Ctrl Pts',(121.807962616873,11.1348021861485,-36.5328331745993));
#74358=CARTESIAN_POINT('Ctrl Pts',(121.811388687965,11.1339149346049,-36.5295219263909));
#74359=CARTESIAN_POINT('',(113.,11.1339148195198,-36.529521496889));
#74360=CARTESIAN_POINT('Origin',(113.,11.0261225267959,-36.1272351837791));
#74361=CARTESIAN_POINT('',(121.912131484566,11.1078254769055,-36.4321547447162));
#74362=CARTESIAN_POINT('',(121.75,11.1498124507801,-36.5888522644724));
#74363=CARTESIAN_POINT('Ctrl Pts',(122.,11.0528894783935,-36.2271308071049));
#74364=CARTESIAN_POINT('Ctrl Pts',(122.,11.062479444333,-36.262921047234));
#74365=CARTESIAN_POINT('Ctrl Pts',(121.991329280155,11.0737664689891,-36.3050447967168));
#74366=CARTESIAN_POINT('Ctrl Pts',(121.962987211232,11.0914818931789,-36.3711596598708));
#74367=CARTESIAN_POINT('Ctrl Pts',(121.938311286558,11.1010458552335,-36.4068528521804));
#74368=CARTESIAN_POINT('Ctrl Pts',(121.912131759621,11.1078255480536,-36.4321550102444));
#74369=CARTESIAN_POINT('',(121.7,10.7025987204178,-34.9198279009177));
#74370=CARTESIAN_POINT('Origin',(121.7,10.624953006887,-34.630050153031));
#74371=CARTESIAN_POINT('',(103.5,10.7025987204178,-34.9198279009177));
#74372=CARTESIAN_POINT('Origin',(104.3,29.7962294964313,-19.0503819820073));
#74373=CARTESIAN_POINT('',(104.3,32.1220693465106,-20.0467960840288));
#74374=CARTESIAN_POINT('Origin',(104.3,31.9720693465106,-20.3066037051641));
#74375=CARTESIAN_POINT('',(104.3,30.959927238132,-19.3758330249198));
#74376=CARTESIAN_POINT('Origin',(104.3,30.5501196169967,-19.4856406460551));
#74377=CARTESIAN_POINT('',(104.3,29.9462294964313,-18.7905743608719));
#74378=CARTESIAN_POINT('Ctrl Pts',(104.300000000003,32.1220693465131,-20.0467960840302));
#74379=CARTESIAN_POINT('Ctrl Pts',(104.408087612489,32.2157595974552,-20.100888175632));
#74380=CARTESIAN_POINT('Ctrl Pts',(104.51617563888,32.3094494902639,-20.1549800604655));
#74381=CARTESIAN_POINT('Ctrl Pts',(104.624264068715,32.4031390339881,-20.209071743755));
#74382=CARTESIAN_POINT('Ctrl Pts',(104.243382456862,32.1710578085035,-20.0750795857476));
#74383=CARTESIAN_POINT('Ctrl Pts',(104.351473262603,32.2647454732616,-20.1291703542645));
#74384=CARTESIAN_POINT('Ctrl Pts',(104.459564357695,32.3584331025398,-20.1832605951055));
#74385=CARTESIAN_POINT('Ctrl Pts',(104.567655925525,32.4521201027652,-20.2373509769986));
#74386=CARTESIAN_POINT('Ctrl Pts',(104.130709934827,32.2346784312497,-20.1900293243369));
#74387=CARTESIAN_POINT('Ctrl Pts',(104.238806827626,32.328365226375,-20.2441105815263));
#74388=CARTESIAN_POINT('Ctrl Pts',(104.346904180794,32.4220515260737,-20.2981917597176));
#74389=CARTESIAN_POINT('Ctrl Pts',(104.455001730451,32.5157376683266,-20.3522727910653));
#74390=CARTESIAN_POINT('Ctrl Pts',(104.086176765824,32.1925987394747,-20.3519003213093));
#74391=CARTESIAN_POINT('Ctrl Pts',(104.194269413733,32.2862963455132,-20.4059717963427));
#74392=CARTESIAN_POINT('Ctrl Pts',(104.302362090344,32.3799937897523,-20.4600434514168));
#74393=CARTESIAN_POINT('Ctrl Pts',(104.410455468833,32.4736905568142,-20.5141148642527));
#74394=CARTESIAN_POINT('Ctrl Pts',(104.087867965647,32.151136497191,-20.4203356511969));
#74395=CARTESIAN_POINT('Ctrl Pts',(104.195955578133,32.2448404709751,-20.4744061366423));
#74396=CARTESIAN_POINT('Ctrl Pts',(104.304043604525,32.3385439651879,-20.5284765978808));
#74397=CARTESIAN_POINT('Ctrl Pts',(104.412132034359,32.4322469920417,-20.5825470355882));
#74398=CARTESIAN_POINT('',(104.624264068715,32.4031390339881,-20.209071743755));
#74399=CARTESIAN_POINT('',(104.412132034359,32.4322469920406,-20.5825470355875));
#74400=CARTESIAN_POINT('Origin',(104.624264068715,32.2531390339881,-20.4688793648903));
#74401=CARTESIAN_POINT('',(104.087867965647,32.1511364971898,-20.4203356511962));
#74402=CARTESIAN_POINT('Ctrl Pts',(104.412132034359,32.4322469920417,-20.5825470355882));
#74403=CARTESIAN_POINT('Ctrl Pts',(104.304043604525,32.3385439651879,-20.5284765978808));
#74404=CARTESIAN_POINT('Ctrl Pts',(104.195955578133,32.2448404709751,-20.4744061366423));
#74405=CARTESIAN_POINT('Ctrl Pts',(104.087867965647,32.151136497191,-20.4203356511969));
#74406=CARTESIAN_POINT('Origin',(104.300000000003,31.9720693465131,-20.3066037051655));
#74407=CARTESIAN_POINT('Ctrl Pts',(104.300000000003,32.1220693465131,-20.0467960840302));
#74408=CARTESIAN_POINT('Ctrl Pts',(104.408087612489,32.2157595974552,-20.100888175632));
#74409=CARTESIAN_POINT('Ctrl Pts',(104.51617563888,32.3094494902639,-20.1549800604655));
#74410=CARTESIAN_POINT('Ctrl Pts',(104.624264068715,32.4031390339881,-20.209071743755));
#74411=CARTESIAN_POINT('Origin',(104.3,31.9720693465106,-20.3066037051641));
#74412=CARTESIAN_POINT('Origin',(104.3,31.9720693465106,-20.3066037051641));
#74413=CARTESIAN_POINT('Origin',(113.,32.2531390339859,-20.468879364889));
#74414=CARTESIAN_POINT('',(121.811388243054,32.4031390339859,-20.2090717437537));
#74415=CARTESIAN_POINT('',(121.5,32.5064359373941,-20.6296297263934));
#74416=CARTESIAN_POINT('Ctrl Pts',(121.811388687965,32.4031394190667,-20.2090719660805));
#74417=CARTESIAN_POINT('Ctrl Pts',(121.80796264376,32.4061081783332,-20.2107859859092));
#74418=CARTESIAN_POINT('Ctrl Pts',(121.80455782351,32.4090274223195,-20.2125392911664));
#74419=CARTESIAN_POINT('Ctrl Pts',(121.765406035132,32.4422479143698,-20.233257916631));
#74420=CARTESIAN_POINT('Ctrl Pts',(121.726559498935,32.4716751410544,-20.2594868158067));
#74421=CARTESIAN_POINT('Ctrl Pts',(121.652509215907,32.5187625223813,-20.3238857140478));
#74422=CARTESIAN_POINT('Ctrl Pts',(121.617288389766,32.5364820278348,-20.3619926475953));
#74423=CARTESIAN_POINT('Ctrl Pts',(121.56412779323,32.553196494323,-20.4354165429558));
#74424=CARTESIAN_POINT('Ctrl Pts',(121.541159186122,32.555772639402,-20.4745077018041));
#74425=CARTESIAN_POINT('Ctrl Pts',(121.517077828304,32.546639697538,-20.5341638139643));
#74426=CARTESIAN_POINT('Ctrl Pts',(121.510716614322,32.5414905633929,-20.5542390480232));
#74427=CARTESIAN_POINT('Ctrl Pts',(121.502178291748,32.5269590323472,-20.5931936538549));
#74428=CARTESIAN_POINT('Ctrl Pts',(121.5,32.5175778592339,-20.612073222796));
#74429=CARTESIAN_POINT('Ctrl Pts',(121.5,32.5064359373941,-20.6296297263934));
#74430=CARTESIAN_POINT('',(104.624264068712,32.5064359373941,-20.6296297263934));
#74431=CARTESIAN_POINT('',(113.,32.5064359373941,-20.6296297263934));
#74432=CARTESIAN_POINT('Origin',(104.624264068712,32.2531390339859,-20.468879364889));
#74433=CARTESIAN_POINT('',(113.,32.4031390339859,-20.2090717437537));
#74434=CARTESIAN_POINT('Origin',(104.624264068712,32.2531390339859,-20.4688793648889));
#74435=CARTESIAN_POINT('Origin',(104.624264068712,32.2531390339859,-20.4688793648889));
#74436=CARTESIAN_POINT('Origin',(104.3,0.,0.));
#74437=CARTESIAN_POINT('',(104.087867965647,31.1696374243337,-21.8892528196833));
#74438=CARTESIAN_POINT('Origin',(104.087867965644,-2.22044604925031E-15,
-2.22044604925031E-15));
#74439=CARTESIAN_POINT('Origin',(104.3,30.9960367753563,-21.7673396757028));
#74440=CARTESIAN_POINT('Origin',(104.25,0.,0.));
#74441=CARTESIAN_POINT('',(104.412132034356,31.4270775313556,-22.0868894429017));
#74442=CARTESIAN_POINT('Origin',(104.412132034356,0.,-2.22044604925031E-15));
#74443=CARTESIAN_POINT('Ctrl Pts',(104.087867965647,31.1696374243348,-21.889252819684));
#74444=CARTESIAN_POINT('Ctrl Pts',(104.195955578132,31.255450997464,-21.9551321242177));
#74445=CARTESIAN_POINT('Ctrl Pts',(104.304043604523,31.341264364705,-22.0210109949489));
#74446=CARTESIAN_POINT('Ctrl Pts',(104.412132034356,31.4270775313556,-22.0868894429017));
#74447=CARTESIAN_POINT('Origin',(104.624264068712,0.,0.));
#74448=CARTESIAN_POINT('',(104.624264068712,31.4989671459791,-22.1374133253307));
#74449=CARTESIAN_POINT('Origin',(104.624264068712,0.,0.));
#74450=CARTESIAN_POINT('Origin',(104.624264068712,31.2535206487377,-21.9649140007177));
#74451=CARTESIAN_POINT('Origin',(113.,0.,0.));
#74452=CARTESIAN_POINT('',(121.5,31.4989671459791,-22.1374133253307));
#74453=CARTESIAN_POINT('Origin',(121.5,0.,0.));
#74454=CARTESIAN_POINT('',(113.,31.4989671459791,-22.1374133253307));
#74455=CARTESIAN_POINT('Origin',(121.7,32.1341506127237,-11.578573478662));
#74456=CARTESIAN_POINT('',(121.7,35.4588694735005,-13.2804347819611));
#74457=CARTESIAN_POINT('Origin',(121.7,35.57367450321,-13.0032709222078));
#74458=CARTESIAN_POINT('',(121.7,34.2190913987366,-12.7669018890611));
#74459=CARTESIAN_POINT('Origin',(121.7,34.0567325686927,-12.3749329995982));
#74460=CARTESIAN_POINT('',(121.7,32.0193455830142,-11.8557373384154));
#74461=CARTESIAN_POINT('Ctrl Pts',(121.699999999997,35.4588694735035,-13.2804347819624));
#74462=CARTESIAN_POINT('Ctrl Pts',(121.591912387511,35.5588186261068,-13.3218350765184));
#74463=CARTESIAN_POINT('Ctrl Pts',(121.483824361119,35.6587673966521,-13.3632352128208));
#74464=CARTESIAN_POINT('Ctrl Pts',(121.375735931285,35.7587157947924,-13.4046351948679));
#74465=CARTESIAN_POINT('Ctrl Pts',(121.756617543137,35.5111305701923,-13.3020820369954));
#74466=CARTESIAN_POINT('Ctrl Pts',(121.648526737397,35.6110770987528,-13.3434810852367));
#74467=CARTESIAN_POINT('Ctrl Pts',(121.540435642305,35.711023187081,-13.3848804265588));
#74468=CARTESIAN_POINT('Ctrl Pts',(121.432344074474,35.8109690043703,-13.4262791829526));
#74469=CARTESIAN_POINT('Ctrl Pts',(121.86928828501,35.6410554019366,-13.2825757663851));
#74470=CARTESIAN_POINT('Ctrl Pts',(121.761191392211,35.7409938552547,-13.3239799148297));
#74471=CARTESIAN_POINT('Ctrl Pts',(121.653094040341,35.8409319450387,-13.3653837198587));
#74472=CARTESIAN_POINT('Ctrl Pts',(121.544996490684,35.940869821741,-13.4067874878286));
#74473=CARTESIAN_POINT('Ctrl Pts',(121.913823234176,35.7438605133323,-13.1506538199745));
#74474=CARTESIAN_POINT('Ctrl Pts',(121.805730586267,35.8437977872112,-13.1920725002925));
#74475=CARTESIAN_POINT('Ctrl Pts',(121.697637909656,35.9437351054288,-13.2334909426447));
#74476=CARTESIAN_POINT('Ctrl Pts',(121.589544531166,36.0436718192265,-13.2749089952212));
#74477=CARTESIAN_POINT('Ctrl Pts',(121.912132034353,35.77291329703,-13.0760988223457));
#74478=CARTESIAN_POINT('Ctrl Pts',(121.804044421867,35.8728536622539,-13.117523156959));
#74479=CARTESIAN_POINT('Ctrl Pts',(121.695956395475,35.9727937163286,-13.158947125839));
#74480=CARTESIAN_POINT('Ctrl Pts',(121.587867965641,36.0727334672248,-13.2003707382629));
#74481=CARTESIAN_POINT('',(121.375735931285,35.7587157947924,-13.4046351948679));
#74482=CARTESIAN_POINT('',(121.587867965641,36.0727334672234,-13.2003707382624));
#74483=CARTESIAN_POINT('Origin',(121.375735931285,35.873520824502,-13.1274713351146));
#74484=CARTESIAN_POINT('',(121.912132034353,35.7729132970285,-13.0760988223452));
#74485=CARTESIAN_POINT('Ctrl Pts',(121.587867965641,36.0727334672248,-13.2003707382629));
#74486=CARTESIAN_POINT('Ctrl Pts',(121.695956395475,35.9727937163286,-13.158947125839));
#74487=CARTESIAN_POINT('Ctrl Pts',(121.804044421867,35.8728536622539,-13.117523156959));
#74488=CARTESIAN_POINT('Ctrl Pts',(121.912132034353,35.77291329703,-13.0760988223457));
#74489=CARTESIAN_POINT('Origin',(121.699999999997,35.573674503213,-13.003270922209));
#74490=CARTESIAN_POINT('Ctrl Pts',(121.699999999997,35.4588694735035,-13.2804347819624));
#74491=CARTESIAN_POINT('Ctrl Pts',(121.591912387511,35.5588186261068,-13.3218350765184));
#74492=CARTESIAN_POINT('Ctrl Pts',(121.483824361119,35.6587673966521,-13.3632352128208));
#74493=CARTESIAN_POINT('Ctrl Pts',(121.375735931285,35.7587157947924,-13.4046351948679));
#74494=CARTESIAN_POINT('Origin',(121.7,35.57367450321,-13.0032709222078));
#74495=CARTESIAN_POINT('Origin',(121.7,35.57367450321,-13.0032709222078));
#74496=CARTESIAN_POINT('Origin',(113.,35.8735208244992,-13.1274713351134));
#74497=CARTESIAN_POINT('',(104.188611756946,35.7587157947896,-13.4046351948668));
#74498=CARTESIAN_POINT('',(104.5,36.155250045634,-13.2305666597347));
#74499=CARTESIAN_POINT('Ctrl Pts',(104.188611312035,35.7587162055958,-13.4046353650279));
#74500=CARTESIAN_POINT('Ctrl Pts',(104.19203735624,35.7618832950857,-13.4059472109483));
#74501=CARTESIAN_POINT('Ctrl Pts',(104.19544217649,35.7650514088087,-13.4071958583021));
#74502=CARTESIAN_POINT('Ctrl Pts',(104.234593964868,35.8017119537402,-13.4209387465913));
#74503=CARTESIAN_POINT('Ctrl Pts',(104.273440501065,35.8404348990817,-13.4283177930335));
#74504=CARTESIAN_POINT('Ctrl Pts',(104.347490784093,35.9201909616572,-13.426471158975));
#74505=CARTESIAN_POINT('Ctrl Pts',(104.382711610234,35.9612101761365,-13.4173309564933));
#74506=CARTESIAN_POINT('Ctrl Pts',(104.43587220677,36.0296363912825,-13.3858937988499));
#74507=CARTESIAN_POINT('Ctrl Pts',(104.458840813878,36.0622177504903,-13.3641404024313));
#74508=CARTESIAN_POINT('Ctrl Pts',(104.482922171696,36.1039863436012,-13.320578412409));
#74509=CARTESIAN_POINT('Ctrl Pts',(104.489283385678,36.1167785033386,-13.3042723014621));
#74510=CARTESIAN_POINT('Ctrl Pts',(104.497821708253,36.1388370343898,-13.2690296012548));
#74511=CARTESIAN_POINT('Ctrl Pts',(104.5,36.1481043071223,-13.2500938628619));
#74512=CARTESIAN_POINT('Ctrl Pts',(104.5,36.155250045634,-13.2305666597347));
#74513=CARTESIAN_POINT('',(121.375735931288,36.155250045634,-13.2305666597347));
#74514=CARTESIAN_POINT('',(113.,36.155250045634,-13.2305666597347));
#74515=CARTESIAN_POINT('Origin',(121.375735931288,35.8735208244992,-13.1274713351134));
#74516=CARTESIAN_POINT('',(113.,35.7587157947896,-13.4046351948668));
#74517=CARTESIAN_POINT('Origin',(121.375735931288,35.8735208244991,-13.1274713351135));
#74518=CARTESIAN_POINT('Origin',(121.375735931288,35.8735208244991,-13.1274713351135));
#74519=CARTESIAN_POINT('Origin',(121.7,0.,0.));
#74520=CARTESIAN_POINT('',(121.912132034352,36.3407848610969,-11.4032031398185));
#74521=CARTESIAN_POINT('Origin',(121.912132034356,0.,-2.22044604925031E-15));
#74522=CARTESIAN_POINT('Origin',(121.7,36.1383832819456,-11.3396925048197));
#74523=CARTESIAN_POINT('Origin',(121.75,0.,0.));
#74524=CARTESIAN_POINT('',(121.587867965644,36.6543001437251,-11.4871305554742));
#74525=CARTESIAN_POINT('Origin',(121.587867965644,-2.22044604925031E-15,
-3.33066907387547E-15));
#74526=CARTESIAN_POINT('Ctrl Pts',(121.912132034352,36.3407848610989,-11.4032031398191));
#74527=CARTESIAN_POINT('Ctrl Pts',(121.804044421867,36.4452904208128,-11.4311788451333));
#74528=CARTESIAN_POINT('Ctrl Pts',(121.695956395477,36.5497955110311,-11.4591546511876));
#74529=CARTESIAN_POINT('Ctrl Pts',(121.587867965644,36.6543001437251,-11.4871305554742));
#74530=CARTESIAN_POINT('Origin',(104.3,33.0434471056386,-15.4188714591814));
#74531=CARTESIAN_POINT('',(104.3,34.4638925493512,-15.6825215664905));
#74532=CARTESIAN_POINT('Origin',(104.3,34.3490875196417,-15.9596854262439));
#74533=CARTESIAN_POINT('',(104.3,33.2241144745873,-15.1689886735905));
#74534=CARTESIAN_POINT('Origin',(104.3,32.8321455851244,-15.3313475036343));
#74535=CARTESIAN_POINT('',(104.3,33.1582521353481,-15.141707599428));
#74536=CARTESIAN_POINT('Ctrl Pts',(104.300000000003,34.4638925493543,-15.6825215664918));
#74537=CARTESIAN_POINT('Ctrl Pts',(104.408087612489,34.5638417019576,-15.7239218610478));
#74538=CARTESIAN_POINT('Ctrl Pts',(104.516175638881,34.6637904725029,-15.7653219973501));
#74539=CARTESIAN_POINT('Ctrl Pts',(104.624264068715,34.7637388706433,-15.8067219793973));
#74540=CARTESIAN_POINT('Ctrl Pts',(104.243382456863,34.5161536460432,-15.7041688215248));
#74541=CARTESIAN_POINT('Ctrl Pts',(104.351473262603,34.6161000618904,-15.7455681418798));
#74542=CARTESIAN_POINT('Ctrl Pts',(104.459564357695,34.7160463736858,-15.7869669437042));
#74543=CARTESIAN_POINT('Ctrl Pts',(104.567655925526,34.8159920802211,-15.828365967482));
#74544=CARTESIAN_POINT('Ctrl Pts',(104.130709646627,34.5942343545562,-15.8098307364183));
#74545=CARTESIAN_POINT('Ctrl Pts',(104.238806539425,34.6941786667331,-15.8512207403264));
#74546=CARTESIAN_POINT('Ctrl Pts',(104.346903892804,34.7941224771499,-15.8926107306706));
#74547=CARTESIAN_POINT('Ctrl Pts',(104.455001442461,34.8940661125616,-15.934000595886));
#74548=CARTESIAN_POINT('Ctrl Pts',(104.086176765824,34.5736426479042,-15.9758096616227));
#74549=CARTESIAN_POINT('Ctrl Pts',(104.194269413733,34.6735964016779,-16.017188555955));
#74550=CARTESIAN_POINT('Ctrl Pts',(104.302362090344,34.7735500185364,-16.0585676499069));
#74551=CARTESIAN_POINT('Ctrl Pts',(104.410455468834,34.8735029323928,-16.0999465920824));
#74552=CARTESIAN_POINT('Ctrl Pts',(104.087867965647,34.5414677238745,-16.0490714263823));
#74553=CARTESIAN_POINT('Ctrl Pts',(104.195955578133,34.6414276617497,-16.0904485084352));
#74554=CARTESIAN_POINT('Ctrl Pts',(104.304043604525,34.7413871209968,-16.1318256290849));
#74555=CARTESIAN_POINT('Ctrl Pts',(104.412132034359,34.8413461138118,-16.1732027874075));
#74556=CARTESIAN_POINT('',(104.624264068715,34.7637388706433,-15.8067219793973));
#74557=CARTESIAN_POINT('',(104.412132034359,34.8413461138104,-16.1732027874068));
#74558=CARTESIAN_POINT('Origin',(104.624264068715,34.6489338409337,-16.0838858391507));
#74559=CARTESIAN_POINT('',(104.087867965647,34.541467723873,-16.0490714263816));
#74560=CARTESIAN_POINT('Ctrl Pts',(104.412132034359,34.8413461138118,-16.1732027874075));
#74561=CARTESIAN_POINT('Ctrl Pts',(104.304043604525,34.7413871209968,-16.1318256290849));
#74562=CARTESIAN_POINT('Ctrl Pts',(104.195955578133,34.6414276617497,-16.0904485084352));
#74563=CARTESIAN_POINT('Ctrl Pts',(104.087867965647,34.5414677238745,-16.0490714263823));
#74564=CARTESIAN_POINT('Origin',(104.300000000003,34.3490875196448,-15.9596854262451));
#74565=CARTESIAN_POINT('Ctrl Pts',(104.300000000003,34.4638925493543,-15.6825215664918));
#74566=CARTESIAN_POINT('Ctrl Pts',(104.408087612489,34.5638417019576,-15.7239218610478));
#74567=CARTESIAN_POINT('Ctrl Pts',(104.516175638881,34.6637904725029,-15.7653219973501));
#74568=CARTESIAN_POINT('Ctrl Pts',(104.624264068715,34.7637388706433,-15.8067219793973));
#74569=CARTESIAN_POINT('Origin',(104.3,34.3490875196417,-15.9596854262439));
#74570=CARTESIAN_POINT('Origin',(104.3,34.3490875196417,-15.9596854262439));
#74571=CARTESIAN_POINT('Origin',(113.,34.6489338409309,-16.0838858391495));
#74572=CARTESIAN_POINT('',(121.811388243054,34.7637388706404,-15.8067219793961));
#74573=CARTESIAN_POINT('',(121.5,34.9210458868021,-16.210199078724));
#74574=CARTESIAN_POINT('Ctrl Pts',(121.811388687965,34.7637392814463,-15.8067221495579));
#74575=CARTESIAN_POINT('Ctrl Pts',(121.80796264376,34.7669063670474,-15.8080340048666));
#74576=CARTESIAN_POINT('Ctrl Pts',(121.80455782351,34.7700294887557,-15.8093912725525));
#74577=CARTESIAN_POINT('Ctrl Pts',(121.765406035132,34.8056700981812,-15.8255965029732));
#74578=CARTESIAN_POINT('Ctrl Pts',(121.726559498935,34.8382691291976,-15.8477599864337));
#74579=CARTESIAN_POINT('Ctrl Pts',(121.652509215907,34.8933594144204,-15.9054618065868));
#74580=CARTESIAN_POINT('Ctrl Pts',(121.617288389766,34.9159012799814,-15.9409298704603));
#74581=CARTESIAN_POINT('Ctrl Pts',(121.56412779323,34.9420564933711,-16.0115439385518));
#74582=CARTESIAN_POINT('Ctrl Pts',(121.541159186122,34.9497130192858,-16.0499644127094));
#74583=CARTESIAN_POINT('Ctrl Pts',(121.517077828304,34.9484448961684,-16.1103022466854));
#74584=CARTESIAN_POINT('Ctrl Pts',(121.510716614322,34.9459601574394,-16.1308778312071));
#74585=CARTESIAN_POINT('Ctrl Pts',(121.502178291748,34.9366375420249,-16.1713959204003));
#74586=CARTESIAN_POINT('Ctrl Pts',(121.5,34.9298009043927,-16.191338460817));
#74587=CARTESIAN_POINT('Ctrl Pts',(121.5,34.9210458868021,-16.210199078724));
#74588=CARTESIAN_POINT('',(104.624264068712,34.9210458868021,-16.210199078724));
#74589=CARTESIAN_POINT('',(113.,34.9210458868021,-16.210199078724));
#74590=CARTESIAN_POINT('Origin',(104.624264068712,34.6489338409309,-16.0838858391495));
#74591=CARTESIAN_POINT('',(113.,34.7637388706404,-15.8067219793961));
#74592=CARTESIAN_POINT('Origin',(104.624264068712,34.6489338409309,-16.0838858391494));
#74593=CARTESIAN_POINT('Origin',(104.624264068712,34.6489338409309,-16.0838858391494));
#74594=CARTESIAN_POINT('Origin',(104.3,0.,0.));
#74595=CARTESIAN_POINT('',(104.087867965647,33.7600976763358,-17.6335331415094));
#74596=CARTESIAN_POINT('Origin',(104.087867965644,-2.22044604925031E-15,
-4.44089209850063E-15));
#74597=CARTESIAN_POINT('Origin',(104.3,33.5720693465106,-17.5353224130539));
#74598=CARTESIAN_POINT('Origin',(104.25,0.,0.));
#74599=CARTESIAN_POINT('',(104.412132034356,34.041132103426,-17.7958762791241));
#74600=CARTESIAN_POINT('Origin',(104.412132034356,-2.22044604925031E-15,
-3.33066907387547E-15));
#74601=CARTESIAN_POINT('Ctrl Pts',(104.087867965647,33.7600976763371,-17.63353314151));
#74602=CARTESIAN_POINT('Ctrl Pts',(104.195955578132,33.8537760772191,-17.6876479205194));
#74603=CARTESIAN_POINT('Ctrl Pts',(104.304043604523,33.9474542173515,-17.7417622963114));
#74604=CARTESIAN_POINT('Ctrl Pts',(104.412132034356,34.041132103426,-17.7958762791241));
#74605=CARTESIAN_POINT('Origin',(104.624264068712,0.,0.));
#74606=CARTESIAN_POINT('',(104.624264068712,34.1190013824203,-17.8365844450781));
#74607=CARTESIAN_POINT('Origin',(104.624264068712,0.,0.));
#74608=CARTESIAN_POINT('Origin',(104.624264068712,33.8531390339859,-17.6975980727788));
#74609=CARTESIAN_POINT('Origin',(113.,0.,0.));
#74610=CARTESIAN_POINT('',(121.5,34.1190013824203,-17.8365844450781));
#74611=CARTESIAN_POINT('Origin',(121.5,0.,0.));
#74612=CARTESIAN_POINT('',(113.,34.1190013824203,-17.8365844450781));
#74613=CARTESIAN_POINT('Origin',(104.3,17.2622256995996,-25.1248579341572));
#74614=CARTESIAN_POINT('',(104.3,22.0053456777902,-30.8134083466537));
#74615=CARTESIAN_POINT('Origin',(104.3,21.7673396757028,-30.9960367753563));
#74616=CARTESIAN_POINT('',(104.3,21.1884328164397,-29.7487867783414));
#74617=CARTESIAN_POINT('Origin',(104.3,20.7677983856497,-29.6934092049567));
#74618=CARTESIAN_POINT('',(104.3,17.500231701687,-24.9422295054546));
#74619=CARTESIAN_POINT('Ctrl Pts',(104.300000000003,22.0053456777917,-30.8134083466557));
#74620=CARTESIAN_POINT('Ctrl Pts',(104.408087612488,22.0712040357549,-30.899236629767));
#74621=CARTESIAN_POINT('Ctrl Pts',(104.51617563888,22.137062141973,-30.9850645847977));
#74622=CARTESIAN_POINT('Ctrl Pts',(104.624264068714,22.2029200028065,-31.070892220037));
#74623=CARTESIAN_POINT('Ctrl Pts',(104.243382456862,22.0397814876374,-30.8582859677809));
#74624=CARTESIAN_POINT('Ctrl Pts',(104.351473262603,22.1056379626008,-30.9441120388314));
#74625=CARTESIAN_POINT('Ctrl Pts',(104.459564357694,22.171494606718,-31.0299376087954));
#74626=CARTESIAN_POINT('Ctrl Pts',(104.567655925525,22.2373506156879,-31.1157630683464));
#74627=CARTESIAN_POINT('Ctrl Pts',(104.130710008275,22.0545697937069,-30.9888322399386));
#74628=CARTESIAN_POINT('Ctrl Pts',(104.238806901074,22.1204291050618,-31.0746491908742));
#74629=CARTESIAN_POINT('Ctrl Pts',(104.346904254189,22.1862879890029,-31.1604658792464));
#74630=CARTESIAN_POINT('Ctrl Pts',(104.455001803846,22.2521467836083,-31.2462823716881));
#74631=CARTESIAN_POINT('Ctrl Pts',(104.086176765824,21.9537480036383,-31.1222783369416));
#74632=CARTESIAN_POINT('Ctrl Pts',(104.194269413732,22.0196210464437,-31.2080903875008));
#74633=CARTESIAN_POINT('Ctrl Pts',(104.302362090344,22.0854938708675,-31.293902542478));
#74634=CARTESIAN_POINT('Ctrl Pts',(104.410455468833,22.1513661623616,-31.3797142145118));
#74635=CARTESIAN_POINT('Ctrl Pts',(104.087867965647,21.8892528196839,-31.1696374243347));
#74636=CARTESIAN_POINT('Ctrl Pts',(104.195955578132,21.9551321242181,-31.2554509974646));
#74637=CARTESIAN_POINT('Ctrl Pts',(104.304043604524,22.0210109949498,-31.3412643647062));
#74638=CARTESIAN_POINT('Ctrl Pts',(104.412132034358,22.086889442903,-31.4270775313575));
#74639=CARTESIAN_POINT('',(104.624264068714,22.2029200028065,-31.070892220037));
#74640=CARTESIAN_POINT('',(104.412132034358,22.0868894429024,-31.4270775313565));
#74641=CARTESIAN_POINT('Origin',(104.624264068714,21.9649140007191,-31.2535206487396));
#74642=CARTESIAN_POINT('',(104.087867965647,21.8892528196832,-31.1696374243336));
#74643=CARTESIAN_POINT('Ctrl Pts',(104.412132034358,22.086889442903,-31.4270775313575));
#74644=CARTESIAN_POINT('Ctrl Pts',(104.304043604524,22.0210109949498,-31.3412643647062));
#74645=CARTESIAN_POINT('Ctrl Pts',(104.195955578132,21.9551321242181,-31.2554509974646));
#74646=CARTESIAN_POINT('Ctrl Pts',(104.087867965647,21.8892528196839,-31.1696374243347));
#74647=CARTESIAN_POINT('Origin',(104.300000000003,21.7673396757043,-30.9960367753583));
#74648=CARTESIAN_POINT('Ctrl Pts',(104.300000000003,22.0053456777917,-30.8134083466557));
#74649=CARTESIAN_POINT('Ctrl Pts',(104.408087612488,22.0712040357549,-30.899236629767));
#74650=CARTESIAN_POINT('Ctrl Pts',(104.51617563888,22.137062141973,-30.9850645847977));
#74651=CARTESIAN_POINT('Ctrl Pts',(104.624264068714,22.2029200028065,-31.070892220037));
#74652=CARTESIAN_POINT('Origin',(104.3,21.7673396757028,-30.9960367753563));
#74653=CARTESIAN_POINT('Origin',(104.3,21.7673396757028,-30.9960367753563));
#74654=CARTESIAN_POINT('Origin',(113.,21.9649140007177,-31.2535206487377));
#74655=CARTESIAN_POINT('',(121.811388243054,22.2029200028051,-31.0708922200351));
#74656=CARTESIAN_POINT('',(121.5,22.1374133253307,-31.4989671459791));
#74657=CARTESIAN_POINT('Ctrl Pts',(121.811388687965,22.2029202734925,-31.0708925728024));
#74658=CARTESIAN_POINT('Ctrl Pts',(121.80796264376,22.2050071224247,-31.0736122156265));
#74659=CARTESIAN_POINT('Ctrl Pts',(121.80455782351,22.2070331913202,-31.0763492047763));
#74660=CARTESIAN_POINT('Ctrl Pts',(121.765406035132,22.2297962492787,-31.1082036507076));
#74661=CARTESIAN_POINT('Ctrl Pts',(121.726559498935,22.2469460965475,-31.1436973059289));
#74662=CARTESIAN_POINT('Ctrl Pts',(121.652509215907,22.2658047729756,-31.2212136906375));
#74663=CARTESIAN_POINT('Ctrl Pts',(121.617288389766,22.2675925692634,-31.2632008677555));
#74664=CARTESIAN_POINT('Ctrl Pts',(121.56412779323,22.2549366144545,-31.3374320512821));
#74665=CARTESIAN_POINT('Ctrl Pts',(121.541159186122,22.2423571233226,-31.3745334208854));
#74666=CARTESIAN_POINT('Ctrl Pts',(121.517077828304,22.2110899794998,-31.4261534563593));
#74667=CARTESIAN_POINT('Ctrl Pts',(121.510716614322,22.1986503403778,-31.4427300658883));
#74668=CARTESIAN_POINT('Ctrl Pts',(121.502178291748,22.1703176740025,-31.4731584527351));
#74669=CARTESIAN_POINT('Ctrl Pts',(121.5,22.1544257019282,-31.4870108805359));
#74670=CARTESIAN_POINT('Ctrl Pts',(121.5,22.1374133253307,-31.4989671459791));
#74671=CARTESIAN_POINT('',(104.624264068712,22.1374133253307,-31.4989671459791));
#74672=CARTESIAN_POINT('',(113.,22.1374133253307,-31.4989671459791));
#74673=CARTESIAN_POINT('Origin',(104.624264068712,21.9649140007177,-31.2535206487377));
#74674=CARTESIAN_POINT('',(113.,22.2029200028051,-31.0708922200351));
#74675=CARTESIAN_POINT('Origin',(104.624264068712,21.9649140007178,-31.2535206487377));
#74676=CARTESIAN_POINT('Origin',(104.624264068712,21.9649140007178,-31.2535206487377));
#74677=CARTESIAN_POINT('Origin',(104.3,0.,0.));
#74678=CARTESIAN_POINT('',(104.087867965647,20.4203356511961,-32.1511364971898));
#74679=CARTESIAN_POINT('Origin',(104.087867965644,2.22044604925031E-15,
2.22044604925031E-15));
#74680=CARTESIAN_POINT('Origin',(104.3,20.306603705164,-31.9720693465106));
#74681=CARTESIAN_POINT('Origin',(104.25,0.,0.));
#74682=CARTESIAN_POINT('',(104.412132034356,20.5825470355869,-32.4322469920394));
#74683=CARTESIAN_POINT('Origin',(104.412132034356,4.44089209850063E-15,
4.44089209850063E-15));
#74684=CARTESIAN_POINT('Ctrl Pts',(104.087867965647,20.4203356511969,-32.1511364971911));
#74685=CARTESIAN_POINT('Ctrl Pts',(104.195955578132,20.4744061366419,-32.2448404709744));
#74686=CARTESIAN_POINT('Ctrl Pts',(104.304043604523,20.5284765978799,-32.3385439651864));
#74687=CARTESIAN_POINT('Ctrl Pts',(104.412132034356,20.5825470355869,-32.4322469920394));
#74688=CARTESIAN_POINT('Origin',(104.624264068712,0.,0.));
#74689=CARTESIAN_POINT('',(104.624264068712,20.6296297263933,-32.5064359373941));
#74690=CARTESIAN_POINT('Origin',(104.624264068712,0.,0.));
#74691=CARTESIAN_POINT('Origin',(104.624264068712,20.468879364889,-32.2531390339859));
#74692=CARTESIAN_POINT('Origin',(113.,0.,0.));
#74693=CARTESIAN_POINT('',(121.5,20.6296297263933,-32.5064359373941));
#74694=CARTESIAN_POINT('Origin',(121.5,0.,0.));
#74695=CARTESIAN_POINT('',(113.,20.6296297263933,-32.5064359373941));
#74696=CARTESIAN_POINT('Origin',(121.7,11.1177260931201,-22.6595636291554));
#74697=CARTESIAN_POINT('',(121.7,15.6825215664904,-34.4638925493513));
#74698=CARTESIAN_POINT('Origin',(121.7,15.9596854262438,-34.3490875196417));
#74699=CARTESIAN_POINT('',(121.7,15.1689886735904,-33.2241144745874));
#74700=CARTESIAN_POINT('Origin',(121.7,15.3313475036343,-32.8321455851244));
#74701=CARTESIAN_POINT('',(121.7,10.8405622333667,-22.7743686588649));
#74702=CARTESIAN_POINT('Ctrl Pts',(121.699999999997,15.6825215664917,-34.4638925493543));
#74703=CARTESIAN_POINT('Ctrl Pts',(121.591912387511,15.7239218610477,-34.5638417019577));
#74704=CARTESIAN_POINT('Ctrl Pts',(121.483824361119,15.7653219973501,-34.663790472503));
#74705=CARTESIAN_POINT('Ctrl Pts',(121.375735931285,15.8067219793973,-34.7637388706433));
#74706=CARTESIAN_POINT('Ctrl Pts',(121.756617543137,15.7041688215247,-34.5161536460432));
#74707=CARTESIAN_POINT('Ctrl Pts',(121.648526737397,15.7455681418797,-34.6161000618904));
#74708=CARTESIAN_POINT('Ctrl Pts',(121.540435642305,15.7869669437042,-34.7160463736859));
#74709=CARTESIAN_POINT('Ctrl Pts',(121.432344074474,15.828365967482,-34.8159920802212));
#74710=CARTESIAN_POINT('Ctrl Pts',(121.869288077041,15.8098327514128,-34.5942310582327));
#74711=CARTESIAN_POINT('Ctrl Pts',(121.761191184242,15.8512227553209,-34.6941753704096));
#74712=CARTESIAN_POINT('Ctrl Pts',(121.653093832523,15.8926127449365,-34.7941191828858));
#74713=CARTESIAN_POINT('Ctrl Pts',(121.544996282866,15.9340026101519,-34.8940628182975));
#74714=CARTESIAN_POINT('Ctrl Pts',(121.913823234176,15.9758096616226,-34.5736426479042));
#74715=CARTESIAN_POINT('Ctrl Pts',(121.805730586267,16.017188555955,-34.6735964016779));
#74716=CARTESIAN_POINT('Ctrl Pts',(121.697637909656,16.0585676499069,-34.7735500185365));
#74717=CARTESIAN_POINT('Ctrl Pts',(121.589544531166,16.0999465920823,-34.8735029323928));
#74718=CARTESIAN_POINT('Ctrl Pts',(121.912132034353,16.0490714263823,-34.5414677238745));
#74719=CARTESIAN_POINT('Ctrl Pts',(121.804044421867,16.0904485084352,-34.6414276617498));
#74720=CARTESIAN_POINT('Ctrl Pts',(121.695956395475,16.1318256290849,-34.7413871209968));
#74721=CARTESIAN_POINT('Ctrl Pts',(121.587867965641,16.1732027874074,-34.8413461138118));
#74722=CARTESIAN_POINT('',(121.375735931285,15.8067219793973,-34.7637388706433));
#74723=CARTESIAN_POINT('',(121.587867965641,16.1732027874068,-34.8413461138104));
#74724=CARTESIAN_POINT('Origin',(121.375735931285,16.0838858391507,-34.6489338409338));
#74725=CARTESIAN_POINT('',(121.912132034353,16.0490714263816,-34.541467723873));
#74726=CARTESIAN_POINT('Ctrl Pts',(121.587867965641,16.1732027874074,-34.8413461138118));
#74727=CARTESIAN_POINT('Ctrl Pts',(121.695956395475,16.1318256290849,-34.7413871209968));
#74728=CARTESIAN_POINT('Ctrl Pts',(121.804044421867,16.0904485084352,-34.6414276617498));
#74729=CARTESIAN_POINT('Ctrl Pts',(121.912132034353,16.0490714263823,-34.5414677238745));
#74730=CARTESIAN_POINT('Origin',(121.699999999997,15.9596854262451,-34.3490875196448));
#74731=CARTESIAN_POINT('Ctrl Pts',(121.699999999997,15.6825215664917,-34.4638925493543));
#74732=CARTESIAN_POINT('Ctrl Pts',(121.591912387511,15.7239218610477,-34.5638417019577));
#74733=CARTESIAN_POINT('Ctrl Pts',(121.483824361119,15.7653219973501,-34.663790472503));
#74734=CARTESIAN_POINT('Ctrl Pts',(121.375735931285,15.8067219793973,-34.7637388706433));
#74735=CARTESIAN_POINT('Origin',(121.7,15.9596854262438,-34.3490875196417));
#74736=CARTESIAN_POINT('Origin',(121.7,15.9596854262438,-34.3490875196417));
#74737=CARTESIAN_POINT('Origin',(113.,16.0838858391495,-34.6489338409309));
#74738=CARTESIAN_POINT('',(104.188611756946,15.8067219793961,-34.7637388706404));
#74739=CARTESIAN_POINT('',(104.5,16.210199078724,-34.9210458868021));
#74740=CARTESIAN_POINT('Ctrl Pts',(104.188611312035,15.8067221495578,-34.7637392814463));
#74741=CARTESIAN_POINT('Ctrl Pts',(104.19203735624,15.8080340048666,-34.7669063670474));
#74742=CARTESIAN_POINT('Ctrl Pts',(104.19544217649,15.8093912725525,-34.7700294887557));
#74743=CARTESIAN_POINT('Ctrl Pts',(104.234593964868,15.8255965029732,-34.8056700981812));
#74744=CARTESIAN_POINT('Ctrl Pts',(104.273440501065,15.8477599864337,-34.8382691291977));
#74745=CARTESIAN_POINT('Ctrl Pts',(104.347490784093,15.9054618065867,-34.8933594144204));
#74746=CARTESIAN_POINT('Ctrl Pts',(104.382711610234,15.9409298704602,-34.9159012799815));
#74747=CARTESIAN_POINT('Ctrl Pts',(104.43587220677,16.0115439385517,-34.9420564933711));
#74748=CARTESIAN_POINT('Ctrl Pts',(104.458840813878,16.0499644127093,-34.9497130192858));
#74749=CARTESIAN_POINT('Ctrl Pts',(104.482922171696,16.1103022466853,-34.9484448961684));
#74750=CARTESIAN_POINT('Ctrl Pts',(104.489283385678,16.1308778312071,-34.9459601574395));
#74751=CARTESIAN_POINT('Ctrl Pts',(104.497821708252,16.1713959204003,-34.9366375420249));
#74752=CARTESIAN_POINT('Ctrl Pts',(104.5,16.1913384608169,-34.9298009043927));
#74753=CARTESIAN_POINT('Ctrl Pts',(104.5,16.210199078724,-34.9210458868021));
#74754=CARTESIAN_POINT('',(121.375735931288,16.210199078724,-34.9210458868021));
#74755=CARTESIAN_POINT('',(113.,16.210199078724,-34.9210458868021));
#74756=CARTESIAN_POINT('Origin',(121.375735931288,16.0838858391495,-34.6489338409309));
#74757=CARTESIAN_POINT('',(113.,15.8067219793961,-34.7637388706404));
#74758=CARTESIAN_POINT('Origin',(121.375735931288,16.0838858391494,-34.648933840931));
#74759=CARTESIAN_POINT('Origin',(121.375735931288,16.0838858391494,-34.648933840931));
#74760=CARTESIAN_POINT('Origin',(121.7,0.,0.));
#74761=CARTESIAN_POINT('',(121.912132034353,17.6335331415093,-33.7600976763359));
#74762=CARTESIAN_POINT('Origin',(121.912132034356,-1.11022302462516E-15,
0.));
#74763=CARTESIAN_POINT('Origin',(121.7,17.535322413054,-33.5720693465106));
#74764=CARTESIAN_POINT('Origin',(121.75,0.,0.));
#74765=CARTESIAN_POINT('',(121.587867965644,17.7958762791241,-34.0411321034261));
#74766=CARTESIAN_POINT('Origin',(121.587867965644,-1.11022302462516E-15,
0.));
#74767=CARTESIAN_POINT('Ctrl Pts',(121.912132034353,17.63353314151,-33.7600976763372));
#74768=CARTESIAN_POINT('Ctrl Pts',(121.804044421868,17.6876479205194,-33.8537760772191));
#74769=CARTESIAN_POINT('Ctrl Pts',(121.695956395477,17.7417622963114,-33.9474542173516));
#74770=CARTESIAN_POINT('Ctrl Pts',(121.587867965644,17.7958762791241,-34.0411321034261));
#74771=CARTESIAN_POINT('Ctrl Pts',(121.375735931288,17.9574056939141,-33.7031390339859));
#74772=CARTESIAN_POINT('Ctrl Pts',(121.483824361121,17.9033140106251,-33.6094494902625));
#74773=CARTESIAN_POINT('Ctrl Pts',(121.591912387512,17.849222125792,-33.5157595974545));
#74774=CARTESIAN_POINT('Ctrl Pts',(121.699999999997,17.7951300341907,-33.4220693465132));
#74775=CARTESIAN_POINT('Ctrl Pts',(121.432344074477,17.9856849271577,-33.752120102763));
#74776=CARTESIAN_POINT('Ctrl Pts',(121.540435642307,17.9315947959052,-33.6584329578312));
#74777=CARTESIAN_POINT('Ctrl Pts',(121.648526737398,17.8775040493508,-33.5647456205277));
#74778=CARTESIAN_POINT('Ctrl Pts',(121.756617543138,17.823413535908,-33.4710578085036));
#74779=CARTESIAN_POINT('Ctrl Pts',(121.544996182435,17.9833149249053,-33.8834537221696));
#74780=CARTESIAN_POINT('Ctrl Pts',(121.653093732091,17.929220861406,-33.7897751040339));
#74781=CARTESIAN_POINT('Ctrl Pts',(121.761191083735,17.8751267330703,-33.6960962793851));
#74782=CARTESIAN_POINT('Ctrl Pts',(121.869287976533,17.8210322170879,-33.6024171392287));
#74783=CARTESIAN_POINT('Ctrl Pts',(121.589544531169,17.8659835447083,-34.0025898869996));
#74784=CARTESIAN_POINT('Ctrl Pts',(121.697637909658,17.8118754705986,-33.908914286335));
#74785=CARTESIAN_POINT('Ctrl Pts',(121.805730586268,17.7577669311553,-33.8152381372974));
#74786=CARTESIAN_POINT('Ctrl Pts',(121.913823234176,17.7036581615694,-33.72156206328));
#74787=CARTESIAN_POINT('Ctrl Pts',(121.587867965644,17.7958762791241,-34.0411321034261));
#74788=CARTESIAN_POINT('Ctrl Pts',(121.695956395477,17.7417622963114,-33.9474542173516));
#74789=CARTESIAN_POINT('Ctrl Pts',(121.804044421868,17.6876479205194,-33.8537760772191));
#74790=CARTESIAN_POINT('Ctrl Pts',(121.912132034353,17.63353314151,-33.7600976763372));
#74791=CARTESIAN_POINT('',(121.699999999997,17.7951300341907,-33.4220693465132));
#74792=CARTESIAN_POINT('Origin',(121.699999999997,17.5353224130553,-33.5720693465132));
#74793=CARTESIAN_POINT('',(121.375735931288,17.9574056939141,-33.7031390339859));
#74794=CARTESIAN_POINT('Origin',(121.375735931288,17.6975980727787,-33.8531390339859));
#74795=CARTESIAN_POINT('Ctrl Pts',(121.375735931288,17.9574056939141,-33.7031390339859));
#74796=CARTESIAN_POINT('Ctrl Pts',(121.483824361121,17.9033140106251,-33.6094494902625));
#74797=CARTESIAN_POINT('Ctrl Pts',(121.591912387512,17.849222125792,-33.5157595974545));
#74798=CARTESIAN_POINT('Ctrl Pts',(121.699999999997,17.7951300341907,-33.4220693465132));
#74799=CARTESIAN_POINT('Origin',(121.375735931288,0.,0.));
#74800=CARTESIAN_POINT('',(121.375735931288,17.836584445078,-34.1190013824203));
#74801=CARTESIAN_POINT('Origin',(121.375735931288,0.,0.));
#74802=CARTESIAN_POINT('Origin',(121.375735931288,17.6975980727787,-33.8531390339859));
#74803=CARTESIAN_POINT('Origin',(121.375735931288,17.6975980727787,-33.8531390339859));
#74804=CARTESIAN_POINT('Origin',(121.375735931288,17.6975980727787,-33.8531390339859));
#74805=CARTESIAN_POINT('Origin',(121.7,12.1768593539449,-24.2909390776529));
#74806=CARTESIAN_POINT('Origin',(121.7,17.5353224130539,-33.5720693465106));
#74807=CARTESIAN_POINT('',(121.7,17.1241669750802,-32.259927238132));
#74808=CARTESIAN_POINT('',(121.7,12.4366669750802,-24.1409390776529));
#74809=CARTESIAN_POINT('Origin',(121.7,16.7143593539449,-32.1501196169967));
#74810=CARTESIAN_POINT('Origin',(121.7,17.535322413054,-33.5720693465106));
#74811=CARTESIAN_POINT('Origin',(113.,15.6473429640468,-34.3789638902265));
#74812=CARTESIAN_POINT('',(104.3,15.1689886735904,-33.2241144745874));
#74813=CARTESIAN_POINT('',(103.5,15.1689886735904,-33.2241144745874));
#74814=CARTESIAN_POINT('Origin',(104.3,15.0541836438809,-32.946950614834));
#74815=CARTESIAN_POINT('',(104.087868515434,15.7681469233145,-34.6706104470789));
#74816=CARTESIAN_POINT('Ctrl Pts',(104.087868240379,15.7681470285123,-34.6706107010489));
#74817=CARTESIAN_POINT('Ctrl Pts',(104.061688713442,15.7581227425572,-34.6464099339429));
#74818=CARTESIAN_POINT('Ctrl Pts',(104.037012788768,15.7439817050433,-34.612270449391));
#74819=CARTESIAN_POINT('Ctrl Pts',(104.008670719845,15.7177881174266,-34.5490335349196));
#74820=CARTESIAN_POINT('Ctrl Pts',(104.,15.7010994022091,-34.5087434123029));
#74821=CARTESIAN_POINT('Ctrl Pts',(104.,15.686919915995,-34.4745111043772));
#74822=CARTESIAN_POINT('',(104.25,15.8302278233913,-34.8204869980086));
#74823=CARTESIAN_POINT('Ctrl Pts',(104.624264068712,20.2090717437536,-32.4031390339859));
#74824=CARTESIAN_POINT('Ctrl Pts',(104.516175638879,20.1549800604646,-32.3094494902625));
#74825=CARTESIAN_POINT('Ctrl Pts',(104.408087612488,20.1008881756316,-32.2157595974544));
#74826=CARTESIAN_POINT('Ctrl Pts',(104.300000000003,20.0467960840302,-32.1220693465131));
#74827=CARTESIAN_POINT('Ctrl Pts',(104.567655925523,20.2373509769973,-32.452120102763));
#74828=CARTESIAN_POINT('Ctrl Pts',(104.459564357693,20.1832605951046,-32.3584331025383));
#74829=CARTESIAN_POINT('Ctrl Pts',(104.351473262602,20.129170354264,-32.2647454732609));
#74830=CARTESIAN_POINT('Ctrl Pts',(104.243382456862,20.0750795857476,-32.1710578085036));
#74831=CARTESIAN_POINT('Ctrl Pts',(104.455001730448,20.352272791064,-32.5157376683244));
#74832=CARTESIAN_POINT('Ctrl Pts',(104.346904180792,20.2981917597167,-32.4220515260722));
#74833=CARTESIAN_POINT('Ctrl Pts',(104.238806827625,20.2441105815258,-32.3283652263742));
#74834=CARTESIAN_POINT('Ctrl Pts',(104.130709934827,20.1900293243368,-32.2346784312498));
#74835=CARTESIAN_POINT('Ctrl Pts',(104.410455468831,20.5141148642513,-32.473690556812));
#74836=CARTESIAN_POINT('Ctrl Pts',(104.302362090342,20.4600434514158,-32.3799937897508));
#74837=CARTESIAN_POINT('Ctrl Pts',(104.194269413732,20.4059717963422,-32.2862963455125));
#74838=CARTESIAN_POINT('Ctrl Pts',(104.086176765824,20.3519003213093,-32.1925987394748));
#74839=CARTESIAN_POINT('Ctrl Pts',(104.412132034356,20.5825470355869,-32.4322469920394));
#74840=CARTESIAN_POINT('Ctrl Pts',(104.304043604523,20.5284765978799,-32.3385439651864));
#74841=CARTESIAN_POINT('Ctrl Pts',(104.195955578132,20.4744061366419,-32.2448404709744));
#74842=CARTESIAN_POINT('Ctrl Pts',(104.087867965647,20.4203356511969,-32.1511364971911));
#74843=CARTESIAN_POINT('',(104.300000000003,20.0467960840302,-32.1220693465131));
#74844=CARTESIAN_POINT('Origin',(104.300000000003,20.3066037051655,-31.9720693465131));
#74845=CARTESIAN_POINT('',(104.624264068712,20.2090717437536,-32.4031390339859));
#74846=CARTESIAN_POINT('Origin',(104.624264068712,20.4688793648889,-32.2531390339859));
#74847=CARTESIAN_POINT('Ctrl Pts',(104.624264068712,20.2090717437536,-32.4031390339859));
#74848=CARTESIAN_POINT('Ctrl Pts',(104.516175638879,20.1549800604646,-32.3094494902625));
#74849=CARTESIAN_POINT('Ctrl Pts',(104.408087612488,20.1008881756316,-32.2157595974544));
#74850=CARTESIAN_POINT('Ctrl Pts',(104.300000000003,20.0467960840302,-32.1220693465131));
#74851=CARTESIAN_POINT('Origin',(104.3,15.5731406460551,-23.7734708323834));
#74852=CARTESIAN_POINT('Origin',(104.3,20.3066037051641,-31.9720693465106));
#74853=CARTESIAN_POINT('',(104.3,19.3758330249197,-30.959927238132));
#74854=CARTESIAN_POINT('',(104.3,15.3133330249197,-23.9234708323834));
#74855=CARTESIAN_POINT('Origin',(104.3,19.4856406460551,-30.5501196169967));
#74856=CARTESIAN_POINT('Origin',(104.3,20.306603705164,-31.9720693465106));
#74857=CARTESIAN_POINT('Origin',(104.624264068712,20.4688793648889,-32.2531390339859));
#74858=CARTESIAN_POINT('Origin',(104.624264068712,20.4688793648889,-32.2531390339859));
#74859=CARTESIAN_POINT('Origin',(113.,21.9493846027006,-30.7404784537055));
#74860=CARTESIAN_POINT('',(121.7,21.1884328164397,-29.7487867783414));
#74861=CARTESIAN_POINT('',(103.5,21.1884328164397,-29.7487867783414));
#74862=CARTESIAN_POINT('Origin',(121.7,21.0058043877371,-29.5107807762541));
#74863=CARTESIAN_POINT('',(121.912131484566,22.1415559502272,-30.9909210297353));
#74864=CARTESIAN_POINT('Ctrl Pts',(121.912131759621,22.1415561175728,-30.9909212478243));
#74865=CARTESIAN_POINT('Ctrl Pts',(121.938311286558,22.1256097814454,-30.9701395779793));
#74866=CARTESIAN_POINT('Ctrl Pts',(121.962987211232,22.1031146393083,-30.9408233379805));
#74867=CARTESIAN_POINT('Ctrl Pts',(121.991329280155,22.0614466587275,-30.8865205684525));
#74868=CARTESIAN_POINT('Ctrl Pts',(122.,22.0348987466286,-30.8519226558093));
#74869=CARTESIAN_POINT('Ctrl Pts',(122.,22.0123424414418,-30.8225267065724));
#74870=CARTESIAN_POINT('',(121.75,22.2403124007255,-31.1196229417565));
#74871=CARTESIAN_POINT('Ctrl Pts',(104.624264068712,33.7031390339858,-17.9574056939141));
#74872=CARTESIAN_POINT('Ctrl Pts',(104.516175638879,33.6094494902624,-17.9033140106251));
#74873=CARTESIAN_POINT('Ctrl Pts',(104.408087612488,33.5157595974544,-17.8492221257921));
#74874=CARTESIAN_POINT('Ctrl Pts',(104.300000000003,33.4220693465131,-17.7951300341907));
#74875=CARTESIAN_POINT('Ctrl Pts',(104.567655925523,33.752120102763,-17.9856849271578));
#74876=CARTESIAN_POINT('Ctrl Pts',(104.459564357693,33.6584329578311,-17.9315947959052));
#74877=CARTESIAN_POINT('Ctrl Pts',(104.351473262602,33.5647456205277,-17.8775040493508));
#74878=CARTESIAN_POINT('Ctrl Pts',(104.243382456862,33.4710578085036,-17.8234135359081));
#74879=CARTESIAN_POINT('Ctrl Pts',(104.455001570347,33.8834541246487,-17.9833187182834));
#74880=CARTESIAN_POINT('Ctrl Pts',(104.346904020691,33.789775506513,-17.9292246547841));
#74881=CARTESIAN_POINT('Ctrl Pts',(104.238806667407,33.6960966825317,-17.8751305285007));
#74882=CARTESIAN_POINT('Ctrl Pts',(104.130709774609,33.6024175423752,-17.8210360125183));
#74883=CARTESIAN_POINT('Ctrl Pts',(104.410455468831,34.0025898869996,-17.8659835447084));
#74884=CARTESIAN_POINT('Ctrl Pts',(104.302362090342,33.908914286335,-17.8118754705986));
#74885=CARTESIAN_POINT('Ctrl Pts',(104.194269413732,33.8152381372974,-17.7577669311554));
#74886=CARTESIAN_POINT('Ctrl Pts',(104.086176765824,33.72156206328,-17.7036581615694));
#74887=CARTESIAN_POINT('Ctrl Pts',(104.412132034356,34.041132103426,-17.7958762791241));
#74888=CARTESIAN_POINT('Ctrl Pts',(104.304043604523,33.9474542173515,-17.7417622963114));
#74889=CARTESIAN_POINT('Ctrl Pts',(104.195955578132,33.8537760772191,-17.6876479205194));
#74890=CARTESIAN_POINT('Ctrl Pts',(104.087867965647,33.7600976763371,-17.63353314151));
#74891=CARTESIAN_POINT('',(104.300000000003,33.4220693465131,-17.7951300341907));
#74892=CARTESIAN_POINT('Origin',(104.300000000003,33.5720693465131,-17.5353224130554));
#74893=CARTESIAN_POINT('',(104.624264068712,33.7031390339858,-17.9574056939141));
#74894=CARTESIAN_POINT('Origin',(104.624264068712,33.8531390339858,-17.6975980727788));
#74895=CARTESIAN_POINT('Ctrl Pts',(104.624264068712,33.7031390339858,-17.9574056939141));
#74896=CARTESIAN_POINT('Ctrl Pts',(104.516175638879,33.6094494902624,-17.9033140106251));
#74897=CARTESIAN_POINT('Ctrl Pts',(104.408087612488,33.5157595974544,-17.8492221257921));
#74898=CARTESIAN_POINT('Ctrl Pts',(104.300000000003,33.4220693465131,-17.7951300341907));
#74899=CARTESIAN_POINT('Origin',(104.3,31.3962294964313,-16.2791006898971));
#74900=CARTESIAN_POINT('Origin',(104.3,33.5720693465106,-17.5353224130539));
#74901=CARTESIAN_POINT('',(104.3,32.259927238132,-17.1241669750802));
#74902=CARTESIAN_POINT('',(104.3,31.2462294964313,-16.5389083110324));
#74903=CARTESIAN_POINT('Origin',(104.3,32.1501196169967,-16.7143593539449));
#74904=CARTESIAN_POINT('Origin',(104.3,33.5720693465106,-17.5353224130539));
#74905=CARTESIAN_POINT('Origin',(104.624264068712,33.8531390339859,-17.6975980727788));
#74906=CARTESIAN_POINT('Origin',(104.624264068712,33.8531390339859,-17.6975980727788));
#74907=CARTESIAN_POINT('Origin',(113.,34.3789638902265,-15.6473429640468));
#74908=CARTESIAN_POINT('',(121.7,33.2241144745873,-15.1689886735905));
#74909=CARTESIAN_POINT('',(103.5,33.2241144745873,-15.1689886735905));
#74910=CARTESIAN_POINT('Origin',(121.7,32.946950614834,-15.0541836438809));
#74911=CARTESIAN_POINT('',(121.912131484566,34.6706104470789,-15.7681469233146));
#74912=CARTESIAN_POINT('Ctrl Pts',(121.912131759621,34.6706107010489,-15.7681470285124));
#74913=CARTESIAN_POINT('Ctrl Pts',(121.938311286558,34.6464099339429,-15.7581227425572));
#74914=CARTESIAN_POINT('Ctrl Pts',(121.962987211232,34.612270449391,-15.7439817050434));
#74915=CARTESIAN_POINT('Ctrl Pts',(121.991329280155,34.5490335349196,-15.7177881174267));
#74916=CARTESIAN_POINT('Ctrl Pts',(122.,34.5087434123029,-15.7010994022092));
#74917=CARTESIAN_POINT('Ctrl Pts',(122.,34.4745111043772,-15.686919915995));
#74918=CARTESIAN_POINT('',(121.75,34.8204869980086,-15.8302278233913));
#74919=CARTESIAN_POINT('Ctrl Pts',(121.375735931288,36.529521496889,-11.1339148195199));
#74920=CARTESIAN_POINT('Ctrl Pts',(121.483824361121,36.4250243891369,-11.1059149038863));
#74921=CARTESIAN_POINT('Ctrl Pts',(121.591912387511,36.3205268920315,-11.0779148839258));
#74922=CARTESIAN_POINT('Ctrl Pts',(121.699999999996,36.2160289954803,-11.0499147569342));
#74923=CARTESIAN_POINT('Ctrl Pts',(121.432344074477,36.5841527803644,-11.1485532278086));
#74924=CARTESIAN_POINT('Ctrl Pts',(121.540435642307,36.4796584662696,-11.1205539109214));
#74925=CARTESIAN_POINT('Ctrl Pts',(121.648526737397,36.3751635810634,-11.0925548930909));
#74926=CARTESIAN_POINT('Ctrl Pts',(121.756617543136,36.2706685250137,-11.0645553747475));
#74927=CARTESIAN_POINT('Ctrl Pts',(121.544996634179,36.6753444250015,-11.2430954833528));
#74928=CARTESIAN_POINT('Ctrl Pts',(121.653094183835,36.5708533597438,-11.2151049763393));
#74929=CARTESIAN_POINT('Ctrl Pts',(121.761191535808,36.4663621029995,-11.1871143689483));
#74930=CARTESIAN_POINT('Ctrl Pts',(121.869288428606,36.3618703486634,-11.1591238127642));
#74931=CARTESIAN_POINT('Ctrl Pts',(121.589544531169,36.6766200040331,-11.410303769972));
#74932=CARTESIAN_POINT('Ctrl Pts',(121.697637909657,36.5721211654519,-11.3823253036304));
#74933=CARTESIAN_POINT('Ctrl Pts',(121.805730586268,36.4676216100719,-11.354346778571));
#74934=CARTESIAN_POINT('Ctrl Pts',(121.913823234175,36.3631219450038,-11.3263684692944));
#74935=CARTESIAN_POINT('Ctrl Pts',(121.587867965644,36.6543001437251,-11.4871305554742));
#74936=CARTESIAN_POINT('Ctrl Pts',(121.695956395477,36.5497955110311,-11.4591546511876));
#74937=CARTESIAN_POINT('Ctrl Pts',(121.804044421867,36.4452904208128,-11.4311788451333));
#74938=CARTESIAN_POINT('Ctrl Pts',(121.912132034352,36.3407848610989,-11.4032031398191));
#74939=CARTESIAN_POINT('',(121.699999999996,36.2160289954803,-11.0499147569342));
#74940=CARTESIAN_POINT('Origin',(121.699999999996,36.1383832819496,-11.3396925048209));
#74941=CARTESIAN_POINT('',(121.375735931288,36.529521496889,-11.1339148195199));
#74942=CARTESIAN_POINT('Origin',(121.375735931288,36.4518757833582,-11.4236925674066));
#74943=CARTESIAN_POINT('Ctrl Pts',(121.375735931288,36.529521496889,-11.1339148195199));
#74944=CARTESIAN_POINT('Ctrl Pts',(121.483824361121,36.4250243891369,-11.1059149038863));
#74945=CARTESIAN_POINT('Ctrl Pts',(121.591912387511,36.3205268920315,-11.0779148839258));
#74946=CARTESIAN_POINT('Ctrl Pts',(121.699999999996,36.2160289954803,-11.0499147569342));
#74947=CARTESIAN_POINT('Origin',(121.375735931288,0.,0.));
#74948=CARTESIAN_POINT('',(121.375735931288,36.7381470591438,-11.5134074305014));
#74949=CARTESIAN_POINT('Origin',(121.375735931288,0.,0.));
#74950=CARTESIAN_POINT('Origin',(121.375735931288,36.4518757833582,-11.4236925674066));
#74951=CARTESIAN_POINT('Origin',(121.375735931288,36.4518757833582,-11.4236925674066));
#74952=CARTESIAN_POINT('Origin',(121.375735931288,36.4518757833582,-11.4236925674066));
#74953=CARTESIAN_POINT('Origin',(121.7,33.2124490802637,-10.5556907983726));
#74954=CARTESIAN_POINT('Origin',(121.7,36.1383832819455,-11.3396925048199));
#74955=CARTESIAN_POINT('',(121.7,34.9198279009177,-10.7025987204178));
#74956=CARTESIAN_POINT('',(121.7,33.2900947937945,-10.2659130504859));
#74957=CARTESIAN_POINT('Origin',(121.7,34.5524044395002,-10.9147307547738));
#74958=CARTESIAN_POINT('Origin',(121.7,36.1383832819456,-11.3396925048197));
#74959=CARTESIAN_POINT('Origin',(113.,35.3739408143757,-13.2452561795175));
#74960=CARTESIAN_POINT('',(104.3,34.2190913987366,-12.7669018890611));
#74961=CARTESIAN_POINT('',(103.5,34.2190913987366,-12.7669018890611));
#74962=CARTESIAN_POINT('Origin',(104.3,33.9419275389832,-12.6520968593516));
#74963=CARTESIAN_POINT('',(104.087868515434,35.6655873712282,-13.3660601387852));
#74964=CARTESIAN_POINT('Ctrl Pts',(104.087868240379,35.6655876251981,-13.366060243983));
#74965=CARTESIAN_POINT('Ctrl Pts',(104.061688713442,35.6413868580921,-13.3560359580279));
#74966=CARTESIAN_POINT('Ctrl Pts',(104.037012788768,35.6072473735402,-13.341894920514));
#74967=CARTESIAN_POINT('Ctrl Pts',(104.008670719845,35.5440104590688,-13.3157013328973));
#74968=CARTESIAN_POINT('Ctrl Pts',(104.,35.5037203364521,-13.2990126176798));
#74969=CARTESIAN_POINT('Ctrl Pts',(104.,35.4694880285264,-13.2848331314657));
#74970=CARTESIAN_POINT('',(104.25,35.8154639221579,-13.428141038862));
#74971=CARTESIAN_POINT('Origin',(113.,37.2800967276863,-8.33272992328159));
#74972=CARTESIAN_POINT('',(104.188611756946,37.2024510141556,-8.62250767116831));
#74973=CARTESIAN_POINT('',(104.5,37.5728723564378,-8.3981702106372));
#74974=CARTESIAN_POINT('Ctrl Pts',(104.188611312035,37.2024514436577,-8.6225077862527));
#74975=CARTESIAN_POINT('Ctrl Pts',(104.19203735624,37.2057626685107,-8.62339502101786));
#74976=CARTESIAN_POINT('Ctrl Pts',(104.19544217649,37.2090666597662,-8.62421946419969));
#74977=CARTESIAN_POINT('Ctrl Pts',(104.234593964868,37.2472073755322,-8.63305961883984));
#74978=CARTESIAN_POINT('Ctrl Pts',(104.273440501065,37.2865621995426,-8.63532117790985));
#74979=CARTESIAN_POINT('Ctrl Pts',(104.347490784093,37.3653949038344,-8.62308008690725));
#74980=CARTESIAN_POINT('Ctrl Pts',(104.382711610234,37.4048701574215,-8.60866399825101));
#74981=CARTESIAN_POINT('Ctrl Pts',(104.43587220677,37.4686076043297,-8.56856437653817));
#74982=CARTESIAN_POINT('Ctrl Pts',(104.458840813878,37.4980708374905,-8.54274436268675));
#74983=CARTESIAN_POINT('Ctrl Pts',(104.482922171696,37.533796113814,-8.49410315611483));
#74984=CARTESIAN_POINT('Ctrl Pts',(104.489283385678,37.5443504602797,-8.47626683430667));
#74985=CARTESIAN_POINT('Ctrl Pts',(104.497821708252,37.5616201820783,-8.43844642422117));
#74986=CARTESIAN_POINT('Ctrl Pts',(104.5,37.5683365621785,-8.41846306187314));
#74987=CARTESIAN_POINT('Ctrl Pts',(104.5,37.5728723564378,-8.3981702106372));
#74988=CARTESIAN_POINT('',(121.5,37.5728723564378,-8.3981702106372));
#74989=CARTESIAN_POINT('',(113.,37.5728723564378,-8.3981702106372));
#74990=CARTESIAN_POINT('',(121.811388243054,37.2024510141556,-8.62250767116831));
#74991=CARTESIAN_POINT('Ctrl Pts',(121.5,37.5728723564378,-8.3981702106372));
#74992=CARTESIAN_POINT('Ctrl Pts',(121.5,37.5683365621785,-8.41846306187314));
#74993=CARTESIAN_POINT('Ctrl Pts',(121.502178291748,37.5616201820783,-8.43844642422117));
#74994=CARTESIAN_POINT('Ctrl Pts',(121.510716614322,37.5443504602797,-8.47626683430668));
#74995=CARTESIAN_POINT('Ctrl Pts',(121.517077828304,37.533796113814,-8.49410315611484));
#74996=CARTESIAN_POINT('Ctrl Pts',(121.541159186122,37.4980708374905,-8.54274436268675));
#74997=CARTESIAN_POINT('Ctrl Pts',(121.56412779323,37.4686076043297,-8.56856437653817));
#74998=CARTESIAN_POINT('Ctrl Pts',(121.617288389766,37.4048701574215,-8.60866399825101));
#74999=CARTESIAN_POINT('Ctrl Pts',(121.652509215907,37.3653949038344,-8.62308008690725));
#75000=CARTESIAN_POINT('Ctrl Pts',(121.726559498935,37.2865621995426,-8.63532117790985));
#75001=CARTESIAN_POINT('Ctrl Pts',(121.765406035132,37.2472073755322,-8.63305961883984));
#75002=CARTESIAN_POINT('Ctrl Pts',(121.804557793905,37.2090666886064,-8.6242194708842));
#75003=CARTESIAN_POINT('Ctrl Pts',(121.807962616873,37.2057626944961,-8.62339502798057));
#75004=CARTESIAN_POINT('Ctrl Pts',(121.811388687965,37.2024514436577,-8.6225077862527));
#75005=CARTESIAN_POINT('',(113.,37.2024510141556,-8.62250767116831));
#75006=CARTESIAN_POINT('Origin',(104.25,0.,0.));
#75007=CARTESIAN_POINT('',(104.087868515434,37.1050842619827,-8.59641832855394));
#75008=CARTESIAN_POINT('',(104.25,37.261781781739,-8.6384053024286));
#75009=CARTESIAN_POINT('',(104.087868515434,37.5703347737696,-6.2574460569156));
#75010=CARTESIAN_POINT('Origin',(104.087867965644,0.,-2.77555756156289E-15));
#75011=CARTESIAN_POINT('',(104.188611756946,37.6702738824291,-6.27060329017727));
#75012=CARTESIAN_POINT('',(104.25,37.7311721243447,-6.27862069582415));
#75013=CARTESIAN_POINT('',(104.5,37.9266483495649,-6.61961818902336));
#75014=CARTESIAN_POINT('Ctrl Pts',(104.5,37.9266483495649,-6.61961818902336));
#75015=CARTESIAN_POINT('Ctrl Pts',(104.5,37.9302235600485,-6.59913426579454));
#75016=CARTESIAN_POINT('Ctrl Pts',(104.497821708252,37.9316657356348,-6.5781017989406));
#75017=CARTESIAN_POINT('Ctrl Pts',(104.489283385678,37.930183837478,-6.53655145973756));
#75018=CARTESIAN_POINT('Ctrl Pts',(104.482922171696,37.9272585576496,-6.51603387355182));
#75019=CARTESIAN_POINT('Ctrl Pts',(104.458840813878,37.9128668899463,-6.45742378699774));
#75020=CARTESIAN_POINT('Ctrl Pts',(104.43587220677,37.8955273033918,-6.42229411347671));
#75021=CARTESIAN_POINT('Ctrl Pts',(104.382711610234,37.8519870416124,-6.36085562876174));
#75022=CARTESIAN_POINT('Ctrl Pts',(104.347490784093,37.8210334610709,-6.33243037397719));
#75023=CARTESIAN_POINT('Ctrl Pts',(104.273440501065,37.7528860018039,-6.29095311068326));
#75024=CARTESIAN_POINT('Ctrl Pts',(104.234593964868,37.7156614242077,-6.27798207968718));
#75025=CARTESIAN_POINT('Ctrl Pts',(104.195442206095,37.6770410460387,-6.27155350246224));
#75026=CARTESIAN_POINT('Ctrl Pts',(104.192037383127,37.6736730528646,-6.27105080458));
#75027=CARTESIAN_POINT('Ctrl Pts',(104.188611312035,37.6702743232782,-6.27060334821649));
#75028=CARTESIAN_POINT('Origin',(104.5,0.,0.));
#75029=CARTESIAN_POINT('Origin',(113.,36.8001647010456,-8.5147153784444));
#75030=CARTESIAN_POINT('',(121.912131484566,37.1050842619827,-8.59641832855395));
#75031=CARTESIAN_POINT('',(121.75,37.261781781739,-8.6384053024286));
#75032=CARTESIAN_POINT('Ctrl Pts',(122.,36.9000603243714,-8.54148233004196));
#75033=CARTESIAN_POINT('Ctrl Pts',(122.,36.9358505645005,-8.55107229598146));
#75034=CARTESIAN_POINT('Ctrl Pts',(121.991329280155,36.9779743139833,-8.56235932063755));
#75035=CARTESIAN_POINT('Ctrl Pts',(121.962987211232,37.0440891771373,-8.58007474482737));
#75036=CARTESIAN_POINT('Ctrl Pts',(121.938311286558,37.0797823694469,-8.58963870688201));
#75037=CARTESIAN_POINT('Ctrl Pts',(121.912131759621,37.105084527511,-8.59641839970203));
#75038=CARTESIAN_POINT('',(121.7,35.5927574181843,-8.19119157206625));
#75039=CARTESIAN_POINT('Origin',(121.7,35.3029796702975,-8.11354585853549));
#75040=CARTESIAN_POINT('',(104.3,35.5927574181843,-8.19119157206625));
#75041=CARTESIAN_POINT('',(103.5,35.5927574181843,-8.19119157206625));
#75042=CARTESIAN_POINT('Origin',(104.3,35.3029796702975,-8.11354585853549));
#75043=CARTESIAN_POINT('Ctrl Pts',(104.087868240379,37.105084527511,-8.59641839970203));
#75044=CARTESIAN_POINT('Ctrl Pts',(104.061688713442,37.0797823694469,-8.589638706882));
#75045=CARTESIAN_POINT('Ctrl Pts',(104.037012788768,37.0440891771373,-8.58007474482736));
#75046=CARTESIAN_POINT('Ctrl Pts',(104.008670719845,36.9779743139833,-8.56235932063754));
#75047=CARTESIAN_POINT('Ctrl Pts',(104.,36.9358505645005,-8.55107229598145));
#75048=CARTESIAN_POINT('Ctrl Pts',(104.,36.9000603243714,-8.54148233004195));
#75049=CARTESIAN_POINT('Ctrl Pts',(104.624264068712,31.0708922200351,-22.2029200028051));
#75050=CARTESIAN_POINT('Ctrl Pts',(104.516175638879,30.9850645847965,-22.1370621419721));
#75051=CARTESIAN_POINT('Ctrl Pts',(104.408087612488,30.8992366297665,-22.0712040357545));
#75052=CARTESIAN_POINT('Ctrl Pts',(104.300000000003,30.8134083466558,-22.0053456777918));
#75053=CARTESIAN_POINT('Ctrl Pts',(104.567655925523,31.1157630683446,-22.2373506156865));
#75054=CARTESIAN_POINT('Ctrl Pts',(104.459564357693,31.0299376087941,-22.1714946067171));
#75055=CARTESIAN_POINT('Ctrl Pts',(104.351473262602,30.9441120388308,-22.1056379626004));
#75056=CARTESIAN_POINT('Ctrl Pts',(104.243382456862,30.858285967781,-22.0397814876375));
#75057=CARTESIAN_POINT('Ctrl Pts',(104.455001803843,31.2462823716862,-22.252146783607));
#75058=CARTESIAN_POINT('Ctrl Pts',(104.346904254187,31.1604658792452,-22.186287989002));
#75059=CARTESIAN_POINT('Ctrl Pts',(104.238806901073,31.0746491908736,-22.1204291050614));
#75060=CARTESIAN_POINT('Ctrl Pts',(104.130710008275,30.9888322399387,-22.054569793707));
#75061=CARTESIAN_POINT('Ctrl Pts',(104.410455468831,31.37971421451,-22.1513661623603));
#75062=CARTESIAN_POINT('Ctrl Pts',(104.302362090342,31.2939025424768,-22.0854938708666));
#75063=CARTESIAN_POINT('Ctrl Pts',(104.194269413731,31.2080903875002,-22.0196210464433));
#75064=CARTESIAN_POINT('Ctrl Pts',(104.086176765824,31.1222783369417,-21.9537480036384));
#75065=CARTESIAN_POINT('Ctrl Pts',(104.412132034356,31.4270775313556,-22.0868894429017));
#75066=CARTESIAN_POINT('Ctrl Pts',(104.304043604523,31.341264364705,-22.0210109949489));
#75067=CARTESIAN_POINT('Ctrl Pts',(104.195955578132,31.255450997464,-21.9551321242177));
#75068=CARTESIAN_POINT('Ctrl Pts',(104.087867965647,31.1696374243348,-21.889252819684));
#75069=CARTESIAN_POINT('',(104.300000000003,30.8134083466558,-22.0053456777918));
#75070=CARTESIAN_POINT('Origin',(104.300000000003,30.9960367753584,-21.7673396757045));
#75071=CARTESIAN_POINT('',(104.624264068712,31.0708922200351,-22.2029200028051));
#75072=CARTESIAN_POINT('Origin',(104.624264068712,31.2535206487377,-21.9649140007177));
#75073=CARTESIAN_POINT('Ctrl Pts',(104.624264068712,31.0708922200351,-22.2029200028051));
#75074=CARTESIAN_POINT('Ctrl Pts',(104.516175638879,30.9850645847965,-22.1370621419721));
#75075=CARTESIAN_POINT('Ctrl Pts',(104.408087612488,30.8992366297665,-22.0712040357545));
#75076=CARTESIAN_POINT('Ctrl Pts',(104.300000000003,30.8134083466558,-22.0053456777918));
#75077=CARTESIAN_POINT('Origin',(104.3,27.907343512885,-19.3973019778198));
#75078=CARTESIAN_POINT('Origin',(104.3,30.9960367753563,-21.7673396757028));
#75079=CARTESIAN_POINT('',(104.3,29.7487867783414,-21.1884328164397));
#75080=CARTESIAN_POINT('',(104.3,27.7247150841823,-19.6353079799072));
#75081=CARTESIAN_POINT('Origin',(104.3,29.6934092049567,-20.7677983856497));
#75082=CARTESIAN_POINT('Origin',(104.3,30.9960367753563,-21.7673396757028));
#75083=CARTESIAN_POINT('Origin',(104.624264068712,31.2535206487377,-21.9649140007177));
#75084=CARTESIAN_POINT('Origin',(104.624264068712,31.2535206487377,-21.9649140007177));
#75085=CARTESIAN_POINT('Origin',(113.,32.0424589928625,-20.0008330249198));
#75086=CARTESIAN_POINT('',(121.7,30.959927238132,-19.3758330249198));
#75087=CARTESIAN_POINT('',(103.5,30.959927238132,-19.3758330249198));
#75088=CARTESIAN_POINT('Origin',(121.7,30.7001196169967,-19.2258330249198));
#75089=CARTESIAN_POINT('',(121.912131484566,32.315842392183,-20.1586710041094));
#75090=CARTESIAN_POINT('Ctrl Pts',(121.912131759621,32.3158426302491,-20.158671141557));
#75091=CARTESIAN_POINT('Ctrl Pts',(121.938311286558,32.293157335936,-20.1455737807786));
#75092=CARTESIAN_POINT('Ctrl Pts',(121.962987211232,32.2611556951878,-20.1270976248782));
#75093=CARTESIAN_POINT('Ctrl Pts',(121.991329280155,32.2018787305382,-20.092874053381));
#75094=CARTESIAN_POINT('Ctrl Pts',(122.,32.1641116099562,-20.0710691961464));
#75095=CARTESIAN_POINT('Ctrl Pts',(122.,32.1320229585134,-20.052542804598));
#75096=CARTESIAN_POINT('',(121.75,32.456333544946,-20.2397836089759));
#75097=CARTESIAN_POINT('Origin',(121.7,22.7280113447945,-20.4652696449976));
#75098=CARTESIAN_POINT('',(121.7,27.6775213868948,-25.8390437558097));
#75099=CARTESIAN_POINT('Origin',(121.7,27.8896534212507,-25.6269117214538));
#75100=CARTESIAN_POINT('',(121.7,26.7286363288515,-24.8901586977665));
#75101=CARTESIAN_POINT('Origin',(121.7,26.7286363288515,-24.4658946290546));
#75102=CARTESIAN_POINT('',(121.7,22.5158793104386,-20.6774016793536));
#75103=CARTESIAN_POINT('Ctrl Pts',(121.699999999998,27.6775213868965,-25.8390437558114));
#75104=CARTESIAN_POINT('Ctrl Pts',(121.591912387512,27.7540191564569,-25.9155415253719));
#75105=CARTESIAN_POINT('Ctrl Pts',(121.48382436112,27.8305166336028,-25.9920390025178));
#75106=CARTESIAN_POINT('Ctrl Pts',(121.375735931286,27.9070138257223,-26.0685361946373));
#75107=CARTESIAN_POINT('Ctrl Pts',(121.756617543138,27.7175202986166,-25.8790426675316));
#75108=CARTESIAN_POINT('Ctrl Pts',(121.648526737397,27.7940161208215,-25.9555382814697));
#75109=CARTESIAN_POINT('Ctrl Pts',(121.540435642306,27.8705114241477,-26.0320339977095));
#75110=CARTESIAN_POINT('Ctrl Pts',(121.432344074475,27.947006700909,-26.108529069824));
#75111=CARTESIAN_POINT('Ctrl Pts',(121.869287690755,27.8450200746977,-25.910740307588));
#75112=CARTESIAN_POINT('Ctrl Pts',(121.761190797956,27.9215064845882,-25.9872375432381));
#75113=CARTESIAN_POINT('Ctrl Pts',(121.653093446519,27.9979926900665,-26.0637343230645));
#75114=CARTESIAN_POINT('Ctrl Pts',(121.544995896862,28.0744787128348,-26.1402309865405));
#75115=CARTESIAN_POINT('Ctrl Pts',(121.913823234177,27.9904837995326,-25.8282031306363));
#75116=CARTESIAN_POINT('Ctrl Pts',(121.805730586268,28.0669635586562,-25.9047133406349));
#75117=CARTESIAN_POINT('Ctrl Pts',(121.697637909656,28.1434434498089,-25.9812233477494));
#75118=CARTESIAN_POINT('Ctrl Pts',(121.589544531167,28.2199229317112,-26.0577327634568));
#75119=CARTESIAN_POINT('Ctrl Pts',(121.912132034354,28.045856034146,-25.7704413132658));
#75120=CARTESIAN_POINT('Ctrl Pts',(121.804044421868,28.1223364854948,-25.8469579301586));
#75121=CARTESIAN_POINT('Ctrl Pts',(121.695956395476,28.1988167893393,-25.9234740900862));
#75122=CARTESIAN_POINT('Ctrl Pts',(121.587867965642,28.2752969494932,-25.9999898046701));
#75123=CARTESIAN_POINT('',(121.375735931286,27.9070138257223,-26.0685361946373));
#75124=CARTESIAN_POINT('',(121.587867965642,28.2752969494924,-25.9999898046693));
#75125=CARTESIAN_POINT('Origin',(121.375735931286,28.1191458600783,-25.8564041602813));
#75126=CARTESIAN_POINT('',(121.912132034354,28.0458560341451,-25.770441313265));
#75127=CARTESIAN_POINT('Ctrl Pts',(121.587867965642,28.2752969494932,-25.9999898046701));
#75128=CARTESIAN_POINT('Ctrl Pts',(121.695956395476,28.1988167893393,-25.9234740900862));
#75129=CARTESIAN_POINT('Ctrl Pts',(121.804044421868,28.1223364854948,-25.8469579301586));
#75130=CARTESIAN_POINT('Ctrl Pts',(121.912132034354,28.045856034146,-25.7704413132658));
#75131=CARTESIAN_POINT('Origin',(121.699999999998,27.8896534212524,-25.6269117214555));
#75132=CARTESIAN_POINT('Ctrl Pts',(121.699999999998,27.6775213868965,-25.8390437558114));
#75133=CARTESIAN_POINT('Ctrl Pts',(121.591912387512,27.7540191564569,-25.9155415253719));
#75134=CARTESIAN_POINT('Ctrl Pts',(121.48382436112,27.8305166336028,-25.9920390025178));
#75135=CARTESIAN_POINT('Ctrl Pts',(121.375735931286,27.9070138257223,-26.0685361946373));
#75136=CARTESIAN_POINT('Origin',(121.7,27.8896534212507,-25.6269117214538));
#75137=CARTESIAN_POINT('Origin',(121.7,27.8896534212507,-25.6269117214538));
#75138=CARTESIAN_POINT('Origin',(113.,28.1191458600767,-25.8564041602798));
#75139=CARTESIAN_POINT('',(104.188611756946,27.9070138257207,-26.0685361946357));
#75140=CARTESIAN_POINT('',(104.5,28.3399768485066,-26.0594649259364));
#75141=CARTESIAN_POINT('Ctrl Pts',(104.188611312035,27.9070141401382,-26.0685365090528));
#75142=CARTESIAN_POINT('Ctrl Pts',(104.19203735624,27.9094381275961,-26.0709604893251));
#75143=CARTESIAN_POINT('Ctrl Pts',(104.19544217649,27.9118872463662,-26.0733264736922));
#75144=CARTESIAN_POINT('Ctrl Pts',(104.234593964868,27.9404979978181,-26.100052630067));
#75145=CARTESIAN_POINT('Ctrl Pts',(104.273440501065,27.9734494956375,-26.121688609679));
#75146=CARTESIAN_POINT('Ctrl Pts',(104.347490784093,28.0478411657046,-26.1505038660466));
#75147=CARTESIAN_POINT('Ctrl Pts',(104.382711610234,28.0892357824599,-26.1577567938406));
#75148=CARTESIAN_POINT('Ctrl Pts',(104.43587220677,28.1644838415113,-26.1548982262093));
#75149=CARTESIAN_POINT('Ctrl Pts',(104.458840813878,28.2029097568318,-26.1472690548683));
#75150=CARTESIAN_POINT('Ctrl Pts',(104.482922171696,28.2581693569711,-26.123007172468));
#75151=CARTESIAN_POINT('Ctrl Pts',(104.489283385678,28.2762278500349,-26.1128376379049));
#75152=CARTESIAN_POINT('Ctrl Pts',(104.497821708252,28.3100940728715,-26.0887190628886));
#75153=CARTESIAN_POINT('Ctrl Pts',(104.5,28.3259023098338,-26.0747711534923));
#75154=CARTESIAN_POINT('Ctrl Pts',(104.5,28.3399768485066,-26.0594649259364));
#75155=CARTESIAN_POINT('',(121.375735931288,28.3399768485066,-26.0594649259364));
#75156=CARTESIAN_POINT('',(113.,28.3399768485066,-26.0594649259364));
#75157=CARTESIAN_POINT('Origin',(121.375735931288,28.1191458600767,-25.8564041602798));
#75158=CARTESIAN_POINT('',(113.,27.9070138257207,-26.0685361946357));
#75159=CARTESIAN_POINT('Origin',(121.375735931288,28.1191458600766,-25.8564041602798));
#75160=CARTESIAN_POINT('Origin',(121.375735931288,28.1191458600766,-25.8564041602798));
#75161=CARTESIAN_POINT('Origin',(121.7,0.,0.));
#75162=CARTESIAN_POINT('',(121.912132034353,29.2106904110607,-24.4422022714321));
#75163=CARTESIAN_POINT('Origin',(121.912132034356,2.22044604925031E-15,
2.22044604925031E-15));
#75164=CARTESIAN_POINT('Origin',(121.7,29.0480002025285,-24.3060703646347));
#75165=CARTESIAN_POINT('Origin',(121.75,0.,0.));
#75166=CARTESIAN_POINT('',(121.587867965644,29.4682231323184,-24.6397181974285));
#75167=CARTESIAN_POINT('Origin',(121.587867965644,-2.22044604925031E-15,
-4.44089209850063E-15));
#75168=CARTESIAN_POINT('Ctrl Pts',(121.912132034353,29.2106904110617,-24.4422022714329));
#75169=CARTESIAN_POINT('Ctrl Pts',(121.804044421868,29.2965351197829,-24.5080409992732));
#75170=CARTESIAN_POINT('Ctrl Pts',(121.695956395477,29.3823793561953,-24.573879640517));
#75171=CARTESIAN_POINT('Ctrl Pts',(121.587867965644,29.4682231323184,-24.6397181974285));
#75172=CARTESIAN_POINT('Ctrl Pts',(104.624264068712,24.2656386875623,-29.4881125046124));
#75173=CARTESIAN_POINT('Ctrl Pts',(104.516175638879,24.1997808267293,-29.4022848693738));
#75174=CARTESIAN_POINT('Ctrl Pts',(104.408087612488,24.1339227205117,-29.3164569143438));
#75175=CARTESIAN_POINT('Ctrl Pts',(104.300000000003,24.068064362549,-29.2306286312331));
#75176=CARTESIAN_POINT('Ctrl Pts',(104.567655925523,24.3000693004436,-29.5329833529219));
#75177=CARTESIAN_POINT('Ctrl Pts',(104.459564357693,24.2342130618665,-29.4471580695557));
#75178=CARTESIAN_POINT('Ctrl Pts',(104.351473262602,24.1683568810269,-29.3613321441074));
#75179=CARTESIAN_POINT('Ctrl Pts',(104.243382456862,24.1025001723946,-29.2755062523583));
#75180=CARTESIAN_POINT('Ctrl Pts',(104.455001885058,24.4223117753432,-29.5810561028804));
#75181=CARTESIAN_POINT('Ctrl Pts',(104.346904335402,24.3564649193042,-29.4952304496556));
#75182=CARTESIAN_POINT('Ctrl Pts',(104.238806982348,24.2906178971386,-29.4094046593508));
#75183=CARTESIAN_POINT('Ctrl Pts',(104.13071008955,24.224770731973,-29.3235783883174));
#75184=CARTESIAN_POINT('Ctrl Pts',(104.410455468831,24.577280943507,-29.518244332399));
#75185=CARTESIAN_POINT('Ctrl Pts',(104.302362090342,24.5114422368762,-29.4324068897942));
#75186=CARTESIAN_POINT('Ctrl Pts',(104.194269413731,24.4456032016902,-29.3465688074239));
#75187=CARTESIAN_POINT('Ctrl Pts',(104.086176765824,24.3797643238856,-29.2607305411385));
#75188=CARTESIAN_POINT('Ctrl Pts',(104.412132034356,24.6397181974285,-29.4682231323184));
#75189=CARTESIAN_POINT('Ctrl Pts',(104.304043604523,24.573879640517,-29.3823793561953));
#75190=CARTESIAN_POINT('Ctrl Pts',(104.195955578132,24.5080409992732,-29.2965351197829));
#75191=CARTESIAN_POINT('Ctrl Pts',(104.087867965647,24.4422022714329,-29.2106904110617));
#75192=CARTESIAN_POINT('Origin',(104.300000000003,24.3060703646363,-29.0480002025305));
#75193=CARTESIAN_POINT('Origin',(104.624264068712,24.5036446896496,-29.3054840759098));
#75194=CARTESIAN_POINT('Origin',(104.3,19.8009563885316,-23.1768213613293));
#75195=CARTESIAN_POINT('Origin',(104.3,24.3060703646347,-29.0480002025284));
#75196=CARTESIAN_POINT('Origin',(104.3,23.3065290745816,-27.7453726321288));
#75197=CARTESIAN_POINT('Origin',(104.3,24.3060703646347,-29.0480002025284));
#75198=CARTESIAN_POINT('Origin',(104.624264068712,24.5036446896497,-29.3054840759098));
#75199=CARTESIAN_POINT('Ctrl Pts',(121.375735931288,29.4881125046124,-24.2656386875623));
#75200=CARTESIAN_POINT('Ctrl Pts',(121.483824361121,29.4022848693738,-24.1997808267293));
#75201=CARTESIAN_POINT('Ctrl Pts',(121.591912387512,29.3164569143438,-24.1339227205117));
#75202=CARTESIAN_POINT('Ctrl Pts',(121.699999999997,29.2306286312331,-24.068064362549));
#75203=CARTESIAN_POINT('Ctrl Pts',(121.432344074477,29.5329833529219,-24.3000693004437));
#75204=CARTESIAN_POINT('Ctrl Pts',(121.540435642307,29.4471580695557,-24.2342130618665));
#75205=CARTESIAN_POINT('Ctrl Pts',(121.648526737398,29.3613321441074,-24.1683568810269));
#75206=CARTESIAN_POINT('Ctrl Pts',(121.756617543138,29.2755062523583,-24.1025001723947));
#75207=CARTESIAN_POINT('Ctrl Pts',(121.544995916356,29.5810525234115,-24.4223128317953));
#75208=CARTESIAN_POINT('Ctrl Pts',(121.653093466012,29.4952268701867,-24.3564659757563));
#75209=CARTESIAN_POINT('Ctrl Pts',(121.761190817463,29.409401077777,-24.2906189537558));
#75210=CARTESIAN_POINT('Ctrl Pts',(121.869287710261,29.3235748067435,-24.2247717885901));
#75211=CARTESIAN_POINT('Ctrl Pts',(121.589544531169,29.518244332399,-24.577280943507));
#75212=CARTESIAN_POINT('Ctrl Pts',(121.697637909658,29.4324068897941,-24.5114422368762));
#75213=CARTESIAN_POINT('Ctrl Pts',(121.805730586269,29.3465688074239,-24.4456032016902));
#75214=CARTESIAN_POINT('Ctrl Pts',(121.913823234176,29.2607305411385,-24.3797643238857));
#75215=CARTESIAN_POINT('Ctrl Pts',(121.587867965644,29.4682231323184,-24.6397181974285));
#75216=CARTESIAN_POINT('Ctrl Pts',(121.695956395477,29.3823793561953,-24.573879640517));
#75217=CARTESIAN_POINT('Ctrl Pts',(121.804044421868,29.2965351197829,-24.5080409992732));
#75218=CARTESIAN_POINT('Ctrl Pts',(121.912132034353,29.2106904110617,-24.4422022714329));
#75219=CARTESIAN_POINT('',(121.699999999997,29.2306286312331,-24.068064362549));
#75220=CARTESIAN_POINT('Origin',(121.699999999997,29.0480002025305,-24.3060703646364));
#75221=CARTESIAN_POINT('',(121.375735931288,29.4881125046124,-24.2656386875623));
#75222=CARTESIAN_POINT('Origin',(121.375735931288,29.3054840759098,-24.5036446896497));
#75223=CARTESIAN_POINT('Ctrl Pts',(121.375735931288,29.4881125046124,-24.2656386875623));
#75224=CARTESIAN_POINT('Ctrl Pts',(121.483824361121,29.4022848693738,-24.1997808267293));
#75225=CARTESIAN_POINT('Ctrl Pts',(121.591912387512,29.3164569143438,-24.1339227205117));
#75226=CARTESIAN_POINT('Ctrl Pts',(121.699999999997,29.2306286312331,-24.068064362549));
#75227=CARTESIAN_POINT('Origin',(121.375735931288,0.,0.));
#75228=CARTESIAN_POINT('',(121.375735931288,29.5356318566107,-24.6960816898302));
#75229=CARTESIAN_POINT('Origin',(121.375735931288,0.,0.));
#75230=CARTESIAN_POINT('Origin',(121.375735931288,29.3054840759098,-24.5036446896497));
#75231=CARTESIAN_POINT('Origin',(121.375735931288,29.3054840759098,-24.5036446896497));
#75232=CARTESIAN_POINT('Origin',(121.375735931288,29.3054840759098,-24.5036446896497));
#75233=CARTESIAN_POINT('Origin',(121.7,24.3857831336789,-20.7286253838904));
#75234=CARTESIAN_POINT('Origin',(121.7,29.0480002025284,-24.3060703646348));
#75235=CARTESIAN_POINT('',(121.7,28.1660070629187,-23.2511515011969));
#75236=CARTESIAN_POINT('',(121.7,24.5684115623815,-20.490619381803));
#75237=CARTESIAN_POINT('Origin',(121.7,27.7453726321287,-23.3065290745817));
#75238=CARTESIAN_POINT('Origin',(121.7,29.0480002025285,-24.3060703646347));
#75239=CARTESIAN_POINT('Origin',(113.,27.6125198053347,-25.7740421742497));
#75240=CARTESIAN_POINT('',(104.3,26.7286363288515,-24.8901586977665));
#75241=CARTESIAN_POINT('',(103.5,26.7286363288515,-24.8901586977665));
#75242=CARTESIAN_POINT('Origin',(104.3,26.5165042944955,-24.6780266634105));
#75243=CARTESIAN_POINT('',(104.087868515434,27.8357364161622,-25.9972587850772));
#75244=CARTESIAN_POINT('Ctrl Pts',(104.087868240379,27.8357366105424,-25.9972589794574));
#75245=CARTESIAN_POINT('Ctrl Pts',(104.061688713442,27.8172141452984,-25.9787365142134));
#75246=CARTESIAN_POINT('Ctrl Pts',(104.037012788768,27.7910849150434,-25.9526072839584));
#75247=CARTESIAN_POINT('Ctrl Pts',(104.008670719845,27.7426854760792,-25.9042078449942));
#75248=CARTESIAN_POINT('Ctrl Pts',(104.,27.7118487512525,-25.8733711201675));
#75249=CARTESIAN_POINT('Ctrl Pts',(104.,27.6856484770629,-25.8471708459779));
#75250=CARTESIAN_POINT('',(104.25,27.9504469620438,-26.1119693309588));
#75251=CARTESIAN_POINT('Origin',(113.,31.2535206487377,-21.9649140007177));
#75252=CARTESIAN_POINT('',(121.811388243054,31.0708922200351,-22.2029200028051));
#75253=CARTESIAN_POINT('Ctrl Pts',(121.5,31.4989671459791,-22.1374133253307));
#75254=CARTESIAN_POINT('Ctrl Pts',(121.5,31.4870108805358,-22.1544257019283));
#75255=CARTESIAN_POINT('Ctrl Pts',(121.502178291748,31.4731584527351,-22.1703176740025));
#75256=CARTESIAN_POINT('Ctrl Pts',(121.510716614322,31.4427300658883,-22.1986503403779));
#75257=CARTESIAN_POINT('Ctrl Pts',(121.517077828304,31.4261534563592,-22.2110899794998));
#75258=CARTESIAN_POINT('Ctrl Pts',(121.541159186122,31.3745334208854,-22.2423571233226));
#75259=CARTESIAN_POINT('Ctrl Pts',(121.56412779323,31.3374320512821,-22.2549366144545));
#75260=CARTESIAN_POINT('Ctrl Pts',(121.617288389766,31.2632008677554,-22.2675925692634));
#75261=CARTESIAN_POINT('Ctrl Pts',(121.652509215907,31.2212136906374,-22.2658047729756));
#75262=CARTESIAN_POINT('Ctrl Pts',(121.726559498935,31.1436973059289,-22.2469460965475));
#75263=CARTESIAN_POINT('Ctrl Pts',(121.765406035132,31.1082036507075,-22.2297962492787));
#75264=CARTESIAN_POINT('Ctrl Pts',(121.804557793905,31.0763492288632,-22.2070332085326));
#75265=CARTESIAN_POINT('Ctrl Pts',(121.807962616873,31.0736122369693,-22.2050071388016));
#75266=CARTESIAN_POINT('Ctrl Pts',(121.811388687965,31.0708925728024,-22.2029202734926));
#75267=CARTESIAN_POINT('',(113.,31.0708922200351,-22.2029200028051));
#75268=CARTESIAN_POINT('Origin',(113.,30.7404784537055,-21.9493846027006));
#75269=CARTESIAN_POINT('',(121.912131484566,30.9909210297353,-22.1415559502273));
#75270=CARTESIAN_POINT('',(121.75,31.1196229417564,-22.2403124007256));
#75271=CARTESIAN_POINT('Ctrl Pts',(122.,30.8225267065723,-22.0123424414419));
#75272=CARTESIAN_POINT('Ctrl Pts',(122.,30.8519226558093,-22.0348987466286));
#75273=CARTESIAN_POINT('Ctrl Pts',(121.991329280155,30.8865205684525,-22.0614466587275));
#75274=CARTESIAN_POINT('Ctrl Pts',(121.962987211232,30.9408233379805,-22.1031146393084));
#75275=CARTESIAN_POINT('Ctrl Pts',(121.938311286558,30.9701395779793,-22.1256097814455));
#75276=CARTESIAN_POINT('Ctrl Pts',(121.912131759621,30.9909212478242,-22.1415561175728));
#75277=CARTESIAN_POINT('',(121.7,29.7487867783414,-21.1884328164397));
#75278=CARTESIAN_POINT('Origin',(121.7,29.510780776254,-21.0058043877371));
#75279=CARTESIAN_POINT('',(103.5,29.7487867783414,-21.1884328164397));
#75280=CARTESIAN_POINT('Origin',(121.7,0.,0.));
#75281=CARTESIAN_POINT('',(121.912131484566,38.0656759583793,-1.3));
#75282=CARTESIAN_POINT('Ctrl Pts',(121.912131759621,38.0656762332744,-1.3));
#75283=CARTESIAN_POINT('Ctrl Pts',(121.938311286558,38.0394815117177,-1.3));
#75284=CARTESIAN_POINT('Ctrl Pts',(121.962987211232,38.0025291999168,-1.3));
#75285=CARTESIAN_POINT('Ctrl Pts',(121.991329280155,37.9340820569223,-1.3));
#75286=CARTESIAN_POINT('Ctrl Pts',(122.,37.8904723424532,-1.3));
#75287=CARTESIAN_POINT('Ctrl Pts',(122.,37.8534195593564,-1.3));
#75288=CARTESIAN_POINT('',(121.912132034363,37.9383242460602,-3.37183029953825));
#75289=CARTESIAN_POINT('Origin',(121.7,37.7270251019467,-3.35305074428517));
#75290=CARTESIAN_POINT('Origin',(121.912132034356,0.,-3.60822483003176E-15));
#75291=CARTESIAN_POINT('Origin',(121.7,35.1412517328676,-3.01262722205121));
#75292=CARTESIAN_POINT('',(121.699999999992,37.6878672442969,-3.65048420269973));
#75293=CARTESIAN_POINT('Origin',(121.7,37.7270251019629,-3.35305074428758));
#75294=CARTESIAN_POINT('',(121.7,36.3574214900301,-3.47532769624597));
#75295=CARTESIAN_POINT('Origin',(121.7,36.099145889284,-3.13873638016781));
#75296=CARTESIAN_POINT('',(121.7,35.1020938752015,-3.31006068046335));
#75297=CARTESIAN_POINT('Origin',(121.699999999992,37.7270251019548,-3.35305074428652));
#75298=CARTESIAN_POINT('Origin',(121.699999999992,37.7270251019548,-3.35305074428652));
#75299=CARTESIAN_POINT('Ctrl Pts',(121.700000000005,37.6878672442757,-3.65048420269694));
#75300=CARTESIAN_POINT('Ctrl Pts',(121.591912387517,37.7951258967967,-3.66460507218919));
#75301=CARTESIAN_POINT('Ctrl Pts',(121.483824361124,37.9023841393188,-3.67872588770406));
#75302=CARTESIAN_POINT('Ctrl Pts',(121.375735931288,38.0096419822012,-3.69284665060537));
#75303=CARTESIAN_POINT('Ctrl Pts',(121.756617543145,37.7439503091544,-3.65786767826058));
#75304=CARTESIAN_POINT('Ctrl Pts',(121.648526737403,37.8512061044746,-3.67198802305758));
#75305=CARTESIAN_POINT('Ctrl Pts',(121.54043564231,37.9584615504179,-3.68610876488932));
#75306=CARTESIAN_POINT('Ctrl Pts',(121.432344074477,38.0657165831673,-3.70022901187376));
#75307=CARTESIAN_POINT('Ctrl Pts',(121.869289250818,37.8644002490085,-3.60540048647845));
#75308=CARTESIAN_POINT('Ctrl Pts',(121.761192358017,37.9716495642733,-3.61952784771998));
#75309=CARTESIAN_POINT('Ctrl Pts',(121.653095005441,38.0788984389064,-3.63365497063251));
#75310=CARTESIAN_POINT('Ctrl Pts',(121.544997455782,38.186147098729,-3.64778211360285));
#75311=CARTESIAN_POINT('Ctrl Pts',(121.913823234184,37.9295576652532,-3.45136431096096));
#75312=CARTESIAN_POINT('Ctrl Pts',(121.805730586274,38.0368096023928,-3.46550601417569));
#75313=CARTESIAN_POINT('Ctrl Pts',(121.69763790966,38.1440615207701,-3.4796474760573));
#75314=CARTESIAN_POINT('Ctrl Pts',(121.589544531169,38.2513127544414,-3.49378871788002));
#75315=CARTESIAN_POINT('Ctrl Pts',(121.912132034361,37.9383242460585,-3.37183029953818));
#75316=CARTESIAN_POINT('Ctrl Pts',(121.804044421873,38.0455806326474,-3.38597666428372));
#75317=CARTESIAN_POINT('Ctrl Pts',(121.69595639548,38.1528366240304,-3.40012275628943));
#75318=CARTESIAN_POINT('Ctrl Pts',(121.587867965644,38.2600922303079,-3.41426858245341));
#75319=CARTESIAN_POINT('',(121.375735931288,38.0096419822012,-3.69284665060536));
#75320=CARTESIAN_POINT('Ctrl Pts',(121.700000000005,37.6878672442757,-3.65048420269694));
#75321=CARTESIAN_POINT('Ctrl Pts',(121.591912387517,37.7951258967967,-3.66460507218919));
#75322=CARTESIAN_POINT('Ctrl Pts',(121.483824361124,37.9023841393188,-3.67872588770406));
#75323=CARTESIAN_POINT('Ctrl Pts',(121.375735931288,38.0096419822012,-3.69284665060537));
#75324=CARTESIAN_POINT('',(121.587867965644,38.2600922303079,-3.4142685824534));
#75325=CARTESIAN_POINT('Origin',(121.375735931288,38.0487998398672,-3.39541319219322));
#75326=CARTESIAN_POINT('Ctrl Pts',(121.587867965644,38.2600922303079,-3.41426858245341));
#75327=CARTESIAN_POINT('Ctrl Pts',(121.69595639548,38.1528366240304,-3.40012275628943));
#75328=CARTESIAN_POINT('Ctrl Pts',(121.804044421873,38.0455806326474,-3.38597666428372));
#75329=CARTESIAN_POINT('Ctrl Pts',(121.912132034361,37.9383242460585,-3.37183029953818));
#75330=CARTESIAN_POINT('Origin',(113.,37.5967275667474,-3.63848543652103));
#75331=CARTESIAN_POINT('',(104.3,36.3574214900301,-3.47532769624597));
#75332=CARTESIAN_POINT('',(103.5,36.3574214900301,-3.47532769624597));
#75333=CARTESIAN_POINT('',(104.300000000005,37.6878672442858,-3.65048420269827));
#75334=CARTESIAN_POINT('',(104.3,37.5595011580629,-3.6335844868415));
#75335=CARTESIAN_POINT('',(104.624264068712,38.0096419822012,-3.69284665060536));
#75336=CARTESIAN_POINT('Ctrl Pts',(104.624264068712,38.0096419822012,-3.69284665060536));
#75337=CARTESIAN_POINT('Ctrl Pts',(104.516175638879,37.9023841393221,-3.6787258877045));
#75338=CARTESIAN_POINT('Ctrl Pts',(104.408087612489,37.7951258968034,-3.66460507219007));
#75339=CARTESIAN_POINT('Ctrl Pts',(104.300000000005,37.6878672442858,-3.65048420269827));
#75340=CARTESIAN_POINT('',(113.,38.0096419822012,-3.69284665060536));
#75341=CARTESIAN_POINT('Origin',(121.7,0.,0.));
#75342=CARTESIAN_POINT('',(121.912131484566,37.5703347737697,-6.2574460569156));
#75343=CARTESIAN_POINT('Ctrl Pts',(121.912131759621,37.570335046313,-6.25744609279661));
#75344=CARTESIAN_POINT('Ctrl Pts',(121.938311286558,37.5443644242305,-6.25402699553556));
#75345=CARTESIAN_POINT('Ctrl Pts',(121.962987211232,37.5077282445796,-6.24920375098245));
#75346=CARTESIAN_POINT('Ctrl Pts',(121.991329280155,37.439866676382,-6.24026960603905));
#75347=CARTESIAN_POINT('Ctrl Pts',(122.,37.3966300490657,-6.23457739606559));
#75348=CARTESIAN_POINT('Ctrl Pts',(122.,37.3598942576648,-6.22974103737681));
#75349=CARTESIAN_POINT('Origin',(121.912132034356,0.,-2.77555756156289E-15));
#75350=CARTESIAN_POINT('Origin',(121.7,36.0718053304427,-5.24424943271127));
#75351=CARTESIAN_POINT('',(121.7,36.3615830783294,-5.32189514624203));
#75352=CARTESIAN_POINT('Origin',(103.5,35.256292659551,-9.44689514624204));
#75353=CARTESIAN_POINT('',(104.3,34.9198279009177,-10.7025987204178));
#75354=CARTESIAN_POINT('',(103.5,34.9198279009177,-10.7025987204178));
#75355=CARTESIAN_POINT('',(104.3,36.5290513235988,-4.69689514624202));
#75356=CARTESIAN_POINT('Origin',(113.,36.127235183779,-11.026122526796));
#75357=CARTESIAN_POINT('',(104.188611756946,36.529521496889,-11.1339148195199));
#75358=CARTESIAN_POINT('',(113.,36.529521496889,-11.1339148195199));
#75359=CARTESIAN_POINT('',(104.087868515434,36.4321547447161,-11.1078254769055));
#75360=CARTESIAN_POINT('',(104.25,36.5888522644724,-11.1498124507802));
#75361=CARTESIAN_POINT('Ctrl Pts',(104.,36.2271308071048,-11.0528894783935));
#75362=CARTESIAN_POINT('Ctrl Pts',(104.,36.2629210472339,-11.062479444333));
#75363=CARTESIAN_POINT('Ctrl Pts',(104.008670719845,36.3050447967167,-11.0737664689891));
#75364=CARTESIAN_POINT('Ctrl Pts',(104.037012788768,36.3711596598708,-11.0914818931789));
#75365=CARTESIAN_POINT('Ctrl Pts',(104.061688713442,36.4068528521804,-11.1010458552336));
#75366=CARTESIAN_POINT('Ctrl Pts',(104.087868240379,36.4321550102444,-11.1078255480536));
#75367=CARTESIAN_POINT('Origin',(104.3,34.630050153031,-10.6249530068871));
#75368=CARTESIAN_POINT('Origin',(113.,33.8531390339859,-17.6975980727788));
#75369=CARTESIAN_POINT('',(121.811388243054,33.7031390339859,-17.9574056939141));
#75370=CARTESIAN_POINT('Ctrl Pts',(121.5,34.1190013824203,-17.8365844450781));
#75371=CARTESIAN_POINT('Ctrl Pts',(121.5,34.1093679652232,-17.855011884237));
#75372=CARTESIAN_POINT('Ctrl Pts',(121.502178291748,34.0977083654644,-17.8725760029409));
#75373=CARTESIAN_POINT('Ctrl Pts',(121.510716614322,34.0712384527426,-17.9046379808983));
#75374=CARTESIAN_POINT('Ctrl Pts',(121.517077828304,34.0564273571332,-17.9191348789048));
#75375=CARTESIAN_POINT('Ctrl Pts',(121.541159186122,34.0093301194435,-17.9568722946504));
#75376=CARTESIAN_POINT('Ctrl Pts',(121.56412779323,33.974188110278,-17.9741868669924));
#75377=CARTESIAN_POINT('Ctrl Pts',(121.617288389766,33.9022439184069,-17.9964236620832));
#75378=CARTESIAN_POINT('Ctrl Pts',(121.652509215907,33.8603825931677,-18.0001315869917));
#75379=CARTESIAN_POINT('Ctrl Pts',(121.726559498935,33.7810678206517,-17.9915521676854));
#75380=CARTESIAN_POINT('Ctrl Pts',(121.765406035132,33.7436393143099,-17.9791818914014));
#75381=CARTESIAN_POINT('Ctrl Pts',(121.804557793905,33.7090862384283,-17.9607714280132));
#75382=CARTESIAN_POINT('Ctrl Pts',(121.807962616873,33.7061082067124,-17.9591199407196));
#75383=CARTESIAN_POINT('Ctrl Pts',(121.811388687965,33.703139419067,-17.9574059162404));
#75384=CARTESIAN_POINT('',(113.,33.7031390339859,-17.9574056939141));
#75385=CARTESIAN_POINT('Origin',(113.,33.3424589928625,-17.7491669750803));
#75386=CARTESIAN_POINT('',(121.912131484566,33.615842392183,-17.9070049542699));
#75387=CARTESIAN_POINT('',(121.75,33.756333544946,-17.9881175591364));
#75388=CARTESIAN_POINT('Ctrl Pts',(122.,33.4320229585134,-17.8008767547585));
#75389=CARTESIAN_POINT('Ctrl Pts',(122.,33.4641116099562,-17.8194031463069));
#75390=CARTESIAN_POINT('Ctrl Pts',(121.991329280155,33.5018787305382,-17.8412080035414));
#75391=CARTESIAN_POINT('Ctrl Pts',(121.962987211232,33.5611556951878,-17.8754315750386));
#75392=CARTESIAN_POINT('Ctrl Pts',(121.938311286558,33.593157335936,-17.8939077309391));
#75393=CARTESIAN_POINT('Ctrl Pts',(121.912131759621,33.6158426302491,-17.9070050917174));
#75394=CARTESIAN_POINT('',(121.7,32.259927238132,-17.1241669750802));
#75395=CARTESIAN_POINT('Origin',(121.7,32.0001196169967,-16.9741669750802));
#75396=CARTESIAN_POINT('',(103.5,32.259927238132,-17.1241669750802));
#75397=CARTESIAN_POINT('Origin',(121.7,0.,0.));
#75398=CARTESIAN_POINT('Origin',(121.912132034356,-2.22044604925031E-15,
-4.44089209850063E-15));
#75399=CARTESIAN_POINT('Origin',(121.7,35.4751196169967,-10.9552904187784));
#75400=CARTESIAN_POINT('',(121.7,35.734927238132,-11.1052904187784));
#75401=CARTESIAN_POINT('Origin',(103.5,31.609927238132,-18.25));
#75402=CARTESIAN_POINT('',(104.3,36.359927238132,-10.0227586640478));
#75403=CARTESIAN_POINT('Origin',(121.7,0.,0.));
#75404=CARTESIAN_POINT('Origin',(121.912132034356,-2.22044604925031E-15,
-2.22044604925031E-15));
#75405=CARTESIAN_POINT('Origin',(121.7,34.8341337964469,-14.0682756632309));
#75406=CARTESIAN_POINT('',(121.7,35.0721397985343,-14.2509040919335));
#75407=CARTESIAN_POINT('Origin',(103.5,28.9573969206301,-22.2197921588183));
#75408=CARTESIAN_POINT('',(104.3,28.1660070629187,-23.2511515011969));
#75409=CARTESIAN_POINT('',(103.5,28.1660070629187,-23.2511515011969));
#75410=CARTESIAN_POINT('',(104.3,35.9986159921561,-13.0434968090722));
#75411=CARTESIAN_POINT('Origin',(113.,29.1576987382828,-24.0121032874578));
#75412=CARTESIAN_POINT('',(104.188611756946,29.4881125046124,-24.2656386875623));
#75413=CARTESIAN_POINT('',(113.,29.4881125046124,-24.2656386875623));
#75414=CARTESIAN_POINT('',(104.087868515434,29.4081413143126,-24.2042746349845));
#75415=CARTESIAN_POINT('',(104.25,29.5368432263337,-24.3030310854828));
#75416=CARTESIAN_POINT('Ctrl Pts',(104.,29.2397469911496,-24.0750611261991));
#75417=CARTESIAN_POINT('Ctrl Pts',(104.,29.2691429403866,-24.0976174313858));
#75418=CARTESIAN_POINT('Ctrl Pts',(104.008670719845,29.3037408530298,-24.1241653434847));
#75419=CARTESIAN_POINT('Ctrl Pts',(104.037012788768,29.3580436225578,-24.1658333240656));
#75420=CARTESIAN_POINT('Ctrl Pts',(104.061688713442,29.3873598625566,-24.1883284662027));
#75421=CARTESIAN_POINT('Ctrl Pts',(104.087868240379,29.4081415324015,-24.20427480233));
#75422=CARTESIAN_POINT('Origin',(104.3,27.9280010608314,-23.0685230724943));
#75423=CARTESIAN_POINT('Origin',(121.7,0.,0.));
#75424=CARTESIAN_POINT('',(121.912131484566,25.9972587850772,-27.8357364161622));
#75425=CARTESIAN_POINT('Origin',(121.912132034356,4.44089209850063E-15,
4.44089209850063E-15));
#75426=CARTESIAN_POINT('Ctrl Pts',(121.912131759621,25.9972589794574,-27.8357366105424));
#75427=CARTESIAN_POINT('Ctrl Pts',(121.938311286558,25.9787365142134,-27.8172141452984));
#75428=CARTESIAN_POINT('Ctrl Pts',(121.962987211232,25.9526072839584,-27.7910849150435));
#75429=CARTESIAN_POINT('Ctrl Pts',(121.991329280155,25.9042078449942,-27.7426854760792));
#75430=CARTESIAN_POINT('Ctrl Pts',(122.,25.8733711201675,-27.7118487512525));
#75431=CARTESIAN_POINT('Ctrl Pts',(122.,25.8471708459779,-27.6856484770629));
#75432=CARTESIAN_POINT('Origin',(121.7,32.4224208522115,-20.7505028516579));
#75433=CARTESIAN_POINT('',(121.7,32.6050492809141,-20.9885088537453));
#75434=CARTESIAN_POINT('Origin',(103.5,22.2197921588183,-28.9573969206301));
#75435=CARTESIAN_POINT('',(104.3,34.1785730872922,-19.781101570884));
#75436=CARTESIAN_POINT('Origin',(113.,20.4688793648889,-32.2531390339859));
#75437=CARTESIAN_POINT('',(121.811388243054,20.2090717437536,-32.4031390339859));
#75438=CARTESIAN_POINT('Ctrl Pts',(121.5,20.6296297263933,-32.5064359373941));
#75439=CARTESIAN_POINT('Ctrl Pts',(121.5,20.612073222796,-32.5175778592339));
#75440=CARTESIAN_POINT('Ctrl Pts',(121.502178291748,20.5931936538549,-32.5269590323472));
#75441=CARTESIAN_POINT('Ctrl Pts',(121.510716614322,20.5542390480232,-32.541490563393));
#75442=CARTESIAN_POINT('Ctrl Pts',(121.517077828304,20.5341638139643,-32.546639697538));
#75443=CARTESIAN_POINT('Ctrl Pts',(121.541159186122,20.4745077018041,-32.555772639402));
#75444=CARTESIAN_POINT('Ctrl Pts',(121.56412779323,20.4354165429558,-32.553196494323));
#75445=CARTESIAN_POINT('Ctrl Pts',(121.617288389766,20.3619926475953,-32.5364820278348));
#75446=CARTESIAN_POINT('Ctrl Pts',(121.652509215907,20.3238857140478,-32.5187625223814));
#75447=CARTESIAN_POINT('Ctrl Pts',(121.726559498935,20.2594868158067,-32.4716751410544));
#75448=CARTESIAN_POINT('Ctrl Pts',(121.765406035132,20.233257916631,-32.4422479143698));
#75449=CARTESIAN_POINT('Ctrl Pts',(121.804557793905,20.2125393068328,-32.4090274474393));
#75450=CARTESIAN_POINT('Ctrl Pts',(121.807962616873,20.2107859993603,-32.4061082016311));
#75451=CARTESIAN_POINT('Ctrl Pts',(121.811388687965,20.2090719660805,-32.4031394190667));
#75452=CARTESIAN_POINT('',(113.,20.2090717437536,-32.4031390339859));
#75453=CARTESIAN_POINT('Origin',(113.,20.0008330249197,-32.0424589928626));
#75454=CARTESIAN_POINT('',(121.912131484566,20.1586710041094,-32.315842392183));
#75455=CARTESIAN_POINT('',(121.75,20.2397836089759,-32.4563335449461));
#75456=CARTESIAN_POINT('Ctrl Pts',(122.,20.052542804598,-32.1320229585134));
#75457=CARTESIAN_POINT('Ctrl Pts',(122.,20.0710691961464,-32.1641116099562));
#75458=CARTESIAN_POINT('Ctrl Pts',(121.991329280155,20.0928740533809,-32.2018787305382));
#75459=CARTESIAN_POINT('Ctrl Pts',(121.962987211232,20.1270976248781,-32.2611556951879));
#75460=CARTESIAN_POINT('Ctrl Pts',(121.938311286558,20.1455737807786,-32.293157335936));
#75461=CARTESIAN_POINT('Ctrl Pts',(121.912131759621,20.1586711415569,-32.3158426302492));
#75462=CARTESIAN_POINT('',(121.7,19.3758330249197,-30.959927238132));
#75463=CARTESIAN_POINT('Origin',(121.7,19.2258330249197,-30.7001196169967));
#75464=CARTESIAN_POINT('',(103.5,19.3758330249197,-30.959927238132));
#75465=CARTESIAN_POINT('Origin',(121.7,0.,0.));
#75466=CARTESIAN_POINT('Origin',(121.912132034356,-4.44089209850063E-15,
-2.22044604925031E-15));
#75467=CARTESIAN_POINT('Origin',(121.7,30.475,-24.2054100357751));
#75468=CARTESIAN_POINT('',(121.7,30.625,-24.4652176569104));
#75469=CARTESIAN_POINT('Origin',(103.5,18.25,-31.609927238132));
#75470=CARTESIAN_POINT('',(104.3,17.1241669750802,-32.259927238132));
#75471=CARTESIAN_POINT('',(103.5,17.1241669750802,-32.259927238132));
#75472=CARTESIAN_POINT('',(104.3,32.5,-23.3826859021799));
#75473=CARTESIAN_POINT('Origin',(113.,17.7491669750802,-33.3424589928626));
#75474=CARTESIAN_POINT('',(104.188611756946,17.9574056939141,-33.7031390339859));
#75475=CARTESIAN_POINT('',(113.,17.9574056939141,-33.7031390339859));
#75476=CARTESIAN_POINT('',(104.087868515434,17.9070049542698,-33.615842392183));
#75477=CARTESIAN_POINT('',(104.25,17.9881175591363,-33.7563335449461));
#75478=CARTESIAN_POINT('Ctrl Pts',(104.,17.8008767547584,-33.4320229585134));
#75479=CARTESIAN_POINT('Ctrl Pts',(104.,17.8194031463068,-33.4641116099562));
#75480=CARTESIAN_POINT('Ctrl Pts',(104.008670719845,17.8412080035414,-33.5018787305382));
#75481=CARTESIAN_POINT('Ctrl Pts',(104.037012788768,17.8754315750386,-33.5611556951879));
#75482=CARTESIAN_POINT('Ctrl Pts',(104.061688713442,17.893907730939,-33.593157335936));
#75483=CARTESIAN_POINT('Ctrl Pts',(104.087868240379,17.9070050917174,-33.6158426302492));
#75484=CARTESIAN_POINT('Origin',(104.3,16.9741669750802,-32.0001196169967));
#75485=CARTESIAN_POINT('Origin',(121.7,0.,0.));
#75486=CARTESIAN_POINT('Origin',(121.912132034356,2.22044604925031E-15,
0.));
#75487=CARTESIAN_POINT('Origin',(121.7,24.7639590139329,-30.8415149116643));
#75488=CARTESIAN_POINT('',(121.7,24.8416047274636,-31.131292659551));
#75489=CARTESIAN_POINT('Origin',(103.5,9.44689514624199,-35.256292659551));
#75490=CARTESIAN_POINT('',(104.3,27.1741364821942,-30.506292659551));
#75491=CARTESIAN_POINT('Origin',(121.7,0.,0.));
#75492=CARTESIAN_POINT('Origin',(121.912132034356,-2.22044604925031E-15,
0.));
#75493=CARTESIAN_POINT('Origin',(113.,-3.39541319219322,-38.0487998398672));
#75494=CARTESIAN_POINT('',(121.811388243054,-3.69284665060536,-38.0096419822012));
#75495=CARTESIAN_POINT('Ctrl Pts',(121.5,-3.42207874082301,-38.3476124040547));
#75496=CARTESIAN_POINT('Ctrl Pts',(121.5,-3.44279002385686,-38.3457641627452));
#75497=CARTESIAN_POINT('Ctrl Pts',(121.502178291748,-3.46347908928978,-38.3417135944028));
#75498=CARTESIAN_POINT('Ctrl Pts',(121.510716614322,-3.50323009155117,-38.329528171585));
#75499=CARTESIAN_POINT('Ctrl Pts',(121.517077828304,-3.52229143980923,-38.3213922261851));
#75500=CARTESIAN_POINT('Ctrl Pts',(121.541159186122,-3.57517959840048,-38.2923215360319));
#75501=CARTESIAN_POINT('Ctrl Pts',(121.56412779323,-3.60462444208904,-38.2664805530063));
#75502=CARTESIAN_POINT('Ctrl Pts',(121.617288389766,-3.65270041222603,-38.2085224397236));
#75503=CARTESIAN_POINT('Ctrl Pts',(121.652509215907,-3.67214572378301,-38.1712665795623));
#75504=CARTESIAN_POINT('Ctrl Pts',(121.726559498935,-3.69457182326876,-38.0947060829812));
#75505=CARTESIAN_POINT('Ctrl Pts',(121.765406035132,-3.69746644747368,-38.0553927522519));
#75506=CARTESIAN_POINT('Ctrl Pts',(121.804557793905,-3.69368028684236,-38.0164244933388));
#75507=CARTESIAN_POINT('Ctrl Pts',(121.807962616873,-3.69329415493239,-38.0130411539632));
#75508=CARTESIAN_POINT('Ctrl Pts',(121.811388687965,-3.69284670864392,-38.0096424230504));
#75509=CARTESIAN_POINT('',(113.,-3.69284665060536,-38.0096419822012));
#75510=CARTESIAN_POINT('Origin',(113.,-3.63848543652103,-37.5967275667474));
#75511=CARTESIAN_POINT('',(121.912131484566,-3.67968941734369,-37.9097028735418));
#75512=CARTESIAN_POINT('',(121.75,-3.70086405625224,-38.0705402241169));
#75513=CARTESIAN_POINT('Ctrl Pts',(122.,-3.6519843978049,-37.6992623574369));
#75514=CARTESIAN_POINT('Ctrl Pts',(122.,-3.65682075649368,-37.7359981488378));
#75515=CARTESIAN_POINT('Ctrl Pts',(121.991329280155,-3.66251296646713,-37.7792347761542));
#75516=CARTESIAN_POINT('Ctrl Pts',(121.962987211232,-3.67144711141054,-37.8470963443517));
#75517=CARTESIAN_POINT('Ctrl Pts',(121.938311286558,-3.67627035596364,-37.8837325240027));
#75518=CARTESIAN_POINT('Ctrl Pts',(121.912131759621,-3.6796894532247,-37.9097031460851));
#75519=CARTESIAN_POINT('',(121.7,-3.47532769624596,-36.3574214900301));
#75520=CARTESIAN_POINT('Origin',(121.7,-3.43616983857994,-36.059988031618));
#75521=CARTESIAN_POINT('',(103.5,-3.47532769624596,-36.3574214900301));
#75522=CARTESIAN_POINT('Ctrl Pts',(121.375735931288,3.69284665060532,-38.0096419822012));
#75523=CARTESIAN_POINT('Ctrl Pts',(121.48382436112,3.67872588770445,-37.9023841393222));
#75524=CARTESIAN_POINT('Ctrl Pts',(121.591912387511,3.66460507219002,-37.7951258968034));
#75525=CARTESIAN_POINT('Ctrl Pts',(121.699999999995,3.65048420269823,-37.6878672442858));
#75526=CARTESIAN_POINT('Ctrl Pts',(121.432344074477,3.70022901187371,-38.0657165831673));
#75527=CARTESIAN_POINT('Ctrl Pts',(121.540435642306,3.68610876488971,-37.9584615504213));
#75528=CARTESIAN_POINT('Ctrl Pts',(121.648526737396,3.67198802305841,-37.8512061044813));
#75529=CARTESIAN_POINT('Ctrl Pts',(121.756617543135,3.65786767826186,-37.7439503091645));
#75530=CARTESIAN_POINT('Ctrl Pts',(121.544997455782,3.6477821136028,-38.186147098729));
#75531=CARTESIAN_POINT('Ctrl Pts',(121.653095005438,3.63365497063291,-38.0788984389098));
#75532=CARTESIAN_POINT('Ctrl Pts',(121.761192358011,3.61952784772082,-37.97164956428));
#75533=CARTESIAN_POINT('Ctrl Pts',(121.869289250808,3.60540048647974,-37.8644002490187));
#75534=CARTESIAN_POINT('Ctrl Pts',(121.589544531169,3.49378871787998,-38.2513127544414));
#75535=CARTESIAN_POINT('Ctrl Pts',(121.697637909657,3.4796474760577,-38.1440615207735));
#75536=CARTESIAN_POINT('Ctrl Pts',(121.805730586267,3.46550601417653,-38.0368096023995));
#75537=CARTESIAN_POINT('Ctrl Pts',(121.913823234174,3.45136431096225,-37.9295576652634));
#75538=CARTESIAN_POINT('Ctrl Pts',(121.587867965644,3.41426858245336,-38.2600922303079));
#75539=CARTESIAN_POINT('Ctrl Pts',(121.695956395476,3.40012275628983,-38.1528366240338));
#75540=CARTESIAN_POINT('Ctrl Pts',(121.804044421867,3.38597666428456,-38.0455806326541));
#75541=CARTESIAN_POINT('Ctrl Pts',(121.912132034351,3.37183029953946,-37.9383242460686));
#75542=CARTESIAN_POINT('',(121.699999999995,3.65048420269823,-37.6878672442858));
#75543=CARTESIAN_POINT('Origin',(121.699999999995,3.35305074428608,-37.7270251019519));
#75544=CARTESIAN_POINT('',(121.375735931288,3.69284665060531,-38.0096419822012));
#75545=CARTESIAN_POINT('Origin',(121.375735931288,3.39541319219317,-38.0487998398672));
#75546=CARTESIAN_POINT('Ctrl Pts',(121.375735931288,3.69284665060532,-38.0096419822012));
#75547=CARTESIAN_POINT('Ctrl Pts',(121.48382436112,3.67872588770445,-37.9023841393222));
#75548=CARTESIAN_POINT('Ctrl Pts',(121.591912387511,3.66460507219002,-37.7951258968034));
#75549=CARTESIAN_POINT('Ctrl Pts',(121.699999999995,3.65048420269823,-37.6878672442858));
#75550=CARTESIAN_POINT('Origin',(121.375735931288,3.39541319219317,-38.0487998398672));
#75551=CARTESIAN_POINT('Origin',(121.375735931288,3.39541319219317,-38.0487998398672));
#75552=CARTESIAN_POINT('Origin',(121.7,1.15848203307056,-21.0576207880785));
#75553=CARTESIAN_POINT('Origin',(121.7,3.3530507442854,-37.7270251019467));
#75554=CARTESIAN_POINT('',(121.7,3.47532769624592,-36.3574214900301));
#75555=CARTESIAN_POINT('',(121.7,1.4559154914827,-21.0184629304125));
#75556=CARTESIAN_POINT('Origin',(121.7,3.13873638016776,-36.099145889284));
#75557=CARTESIAN_POINT('Origin',(121.7,3.35305074428562,-37.7270251019467));
#75558=CARTESIAN_POINT('Origin',(121.7,20.9439362252507,-33.7550468596362));
#75559=CARTESIAN_POINT('',(121.7,20.9830940829167,-34.0524803180483));
#75560=CARTESIAN_POINT('Origin',(103.5,4.76420601603187,-36.1877374401441));
#75561=CARTESIAN_POINT('',(103.5,3.47532769624592,-36.3574214900301));
#75562=CARTESIAN_POINT('',(104.3,23.440501365778,-33.7289565116701));
#75563=CARTESIAN_POINT('Origin',(113.,3.63848543652098,-37.5967275667474));
#75564=CARTESIAN_POINT('',(113.,3.69284665060531,-38.0096419822012));
#75565=CARTESIAN_POINT('Origin',(121.7,0.,0.));
#75566=CARTESIAN_POINT('Origin',(121.912132034356,2.22044604925031E-15,
0.));
#75567=CARTESIAN_POINT('Origin',(121.7,11.4938399085189,-38.0255611038277));
#75568=CARTESIAN_POINT('',(121.7,11.4546820508529,-38.3229945622399));
#75569=CARTESIAN_POINT('Origin',(103.5,-4.76420601603192,-36.1877374401441));
#75570=CARTESIAN_POINT('',(104.3,13.9120893337142,-38.646518368618));
#75571=CARTESIAN_POINT('Origin',(121.7,0.,0.));
#75572=CARTESIAN_POINT('Origin',(121.912132034356,2.22044604925031E-15,
0.));
#75573=CARTESIAN_POINT('Origin',(121.7,6.02546014851033,-39.0915149116643));
#75574=CARTESIAN_POINT('',(121.7,5.94781443497958,-39.381292659551));
#75575=CARTESIAN_POINT('Origin',(103.5,-9.44689514624203,-35.256292659551));
#75576=CARTESIAN_POINT('',(104.3,-10.7025987204178,-34.9198279009177));
#75577=CARTESIAN_POINT('',(103.5,-10.7025987204178,-34.9198279009177));
#75578=CARTESIAN_POINT('',(104.3,8.28034618971012,-40.006292659551));
#75579=CARTESIAN_POINT('Origin',(113.,-11.026122526796,-36.127235183779));
#75580=CARTESIAN_POINT('',(104.188611756946,-11.1339148195199,-36.529521496889));
#75581=CARTESIAN_POINT('',(113.,-11.1339148195199,-36.529521496889));
#75582=CARTESIAN_POINT('',(104.087868515434,-11.1078254769055,-36.4321547447161));
#75583=CARTESIAN_POINT('',(104.25,-11.1498124507802,-36.5888522644724));
#75584=CARTESIAN_POINT('Ctrl Pts',(104.,-11.0528894783935,-36.2271308071048));
#75585=CARTESIAN_POINT('Ctrl Pts',(104.,-11.062479444333,-36.2629210472339));
#75586=CARTESIAN_POINT('Ctrl Pts',(104.008670719845,-11.0737664689891,-36.3050447967167));
#75587=CARTESIAN_POINT('Ctrl Pts',(104.037012788768,-11.0914818931789,-36.3711596598708));
#75588=CARTESIAN_POINT('Ctrl Pts',(104.061688713442,-11.1010458552336,-36.4068528521804));
#75589=CARTESIAN_POINT('Ctrl Pts',(104.087868240379,-11.1078255480536,-36.4321550102444));
#75590=CARTESIAN_POINT('Origin',(104.3,-10.6249530068871,-34.630050153031));
#75591=CARTESIAN_POINT('Origin',(113.,-17.6975980727788,-33.8531390339859));
#75592=CARTESIAN_POINT('',(121.811388243054,-17.9574056939141,-33.7031390339859));
#75593=CARTESIAN_POINT('Ctrl Pts',(121.5,-17.8365844450781,-34.1190013824203));
#75594=CARTESIAN_POINT('Ctrl Pts',(121.5,-17.855011884237,-34.1093679652232));
#75595=CARTESIAN_POINT('Ctrl Pts',(121.502178291748,-17.8725760029409,-34.0977083654644));
#75596=CARTESIAN_POINT('Ctrl Pts',(121.510716614322,-17.9046379808983,-34.0712384527426));
#75597=CARTESIAN_POINT('Ctrl Pts',(121.517077828304,-17.9191348789048,-34.0564273571332));
#75598=CARTESIAN_POINT('Ctrl Pts',(121.541159186122,-17.9568722946504,-34.0093301194435));
#75599=CARTESIAN_POINT('Ctrl Pts',(121.56412779323,-17.9741868669924,-33.974188110278));
#75600=CARTESIAN_POINT('Ctrl Pts',(121.617288389766,-17.9964236620831,-33.9022439184069));
#75601=CARTESIAN_POINT('Ctrl Pts',(121.652509215907,-18.0001315869917,-33.8603825931677));
#75602=CARTESIAN_POINT('Ctrl Pts',(121.726559498935,-17.9915521676854,-33.7810678206517));
#75603=CARTESIAN_POINT('Ctrl Pts',(121.765406035132,-17.9791818914014,-33.7436393143099));
#75604=CARTESIAN_POINT('Ctrl Pts',(121.804557793905,-17.9607714280132,-33.7090862384283));
#75605=CARTESIAN_POINT('Ctrl Pts',(121.807962616873,-17.9591199407196,-33.7061082067124));
#75606=CARTESIAN_POINT('Ctrl Pts',(121.811388687965,-17.9574059162404,-33.703139419067));
#75607=CARTESIAN_POINT('',(113.,-17.9574056939141,-33.7031390339859));
#75608=CARTESIAN_POINT('Origin',(113.,-17.7491669750803,-33.3424589928625));
#75609=CARTESIAN_POINT('',(121.912131484566,-17.9070049542699,-33.615842392183));
#75610=CARTESIAN_POINT('',(121.75,-17.9881175591364,-33.756333544946));
#75611=CARTESIAN_POINT('Ctrl Pts',(122.,-17.8008767547585,-33.4320229585134));
#75612=CARTESIAN_POINT('Ctrl Pts',(122.,-17.8194031463069,-33.4641116099562));
#75613=CARTESIAN_POINT('Ctrl Pts',(121.991329280155,-17.8412080035414,-33.5018787305382));
#75614=CARTESIAN_POINT('Ctrl Pts',(121.962987211232,-17.8754315750386,-33.5611556951878));
#75615=CARTESIAN_POINT('Ctrl Pts',(121.938311286558,-17.8939077309391,-33.593157335936));
#75616=CARTESIAN_POINT('Ctrl Pts',(121.912131759621,-17.9070050917174,-33.6158426302491));
#75617=CARTESIAN_POINT('',(121.7,-17.1241669750802,-32.259927238132));
#75618=CARTESIAN_POINT('Origin',(121.7,-16.9741669750802,-32.0001196169967));
#75619=CARTESIAN_POINT('',(103.5,-17.1241669750802,-32.259927238132));
#75620=CARTESIAN_POINT('Origin',(121.7,0.,0.));
#75621=CARTESIAN_POINT('Origin',(121.912132034356,-2.22044604925031E-15,
0.));
#75622=CARTESIAN_POINT('Origin',(121.7,-5.72500000000002,-38.4948291982183));
#75623=CARTESIAN_POINT('',(121.7,-19.3758330249198,-30.959927238132));
#75624=CARTESIAN_POINT('Origin',(121.7,-19.2258330249198,-30.7001196169967));
#75625=CARTESIAN_POINT('',(121.7,-5.87500000000002,-38.7546368193536));
#75626=CARTESIAN_POINT('Origin',(103.5,-18.25,-31.609927238132));
#75627=CARTESIAN_POINT('',(103.5,-19.3758330249198,-30.959927238132));
#75628=CARTESIAN_POINT('',(104.3,-4.00000000000002,-39.8371685740842));
#75629=CARTESIAN_POINT('Origin',(121.7,0.,0.));
#75630=CARTESIAN_POINT('',(121.912131484566,-20.1586710041094,-32.315842392183));
#75631=CARTESIAN_POINT('Origin',(121.912132034356,-2.22044604925031E-15,
2.22044604925031E-15));
#75632=CARTESIAN_POINT('Ctrl Pts',(121.912131759621,-20.158671141557,-32.3158426302491));
#75633=CARTESIAN_POINT('Ctrl Pts',(121.938311286558,-20.1455737807786,-32.293157335936));
#75634=CARTESIAN_POINT('Ctrl Pts',(121.962987211232,-20.1270976248782,-32.2611556951878));
#75635=CARTESIAN_POINT('Ctrl Pts',(121.991329280155,-20.092874053381,-32.2018787305382));
#75636=CARTESIAN_POINT('Ctrl Pts',(122.,-20.0710691961464,-32.1641116099562));
#75637=CARTESIAN_POINT('Ctrl Pts',(122.,-20.052542804598,-32.1320229585134));
#75638=CARTESIAN_POINT('Origin',(121.7,-11.6519066080199,-36.6882789854275));
#75639=CARTESIAN_POINT('',(121.7,-11.8345350367225,-36.9262849875149));
#75640=CARTESIAN_POINT('Origin',(103.5,-22.2197921588183,-28.9573969206301));
#75641=CARTESIAN_POINT('',(104.3,-23.2511515011969,-28.1660070629187));
#75642=CARTESIAN_POINT('',(103.5,-23.2511515011969,-28.1660070629187));
#75643=CARTESIAN_POINT('',(104.3,-10.2610112303444,-38.1336922703762));
#75644=CARTESIAN_POINT('Origin',(113.,-24.0121032874578,-29.1576987382828));
#75645=CARTESIAN_POINT('',(104.188611756946,-24.2656386875623,-29.4881125046124));
#75646=CARTESIAN_POINT('',(113.,-24.2656386875623,-29.4881125046124));
#75647=CARTESIAN_POINT('',(104.087868515434,-24.2042746349845,-29.4081413143126));
#75648=CARTESIAN_POINT('',(104.25,-24.3030310854828,-29.5368432263338));
#75649=CARTESIAN_POINT('Ctrl Pts',(104.,-24.0750611261991,-29.2397469911496));
#75650=CARTESIAN_POINT('Ctrl Pts',(104.,-24.0976174313858,-29.2691429403866));
#75651=CARTESIAN_POINT('Ctrl Pts',(104.008670719845,-24.1241653434847,-29.3037408530298));
#75652=CARTESIAN_POINT('Ctrl Pts',(104.037012788768,-24.1658333240656,-29.3580436225578));
#75653=CARTESIAN_POINT('Ctrl Pts',(104.061688713442,-24.1883284662027,-29.3873598625566));
#75654=CARTESIAN_POINT('Ctrl Pts',(104.087868240379,-24.20427480233,-29.4081415324015));
#75655=CARTESIAN_POINT('Origin',(104.3,-23.0685230724943,-27.9280010608314));
#75656=CARTESIAN_POINT('Origin',(121.7,0.,0.));
#75657=CARTESIAN_POINT('',(121.912131484566,-27.8357364161622,-25.9972587850772));
#75658=CARTESIAN_POINT('Ctrl Pts',(121.912131759621,-27.8357366105424,-25.9972589794574));
#75659=CARTESIAN_POINT('Ctrl Pts',(121.938311286558,-27.8172141452984,-25.9787365142134));
#75660=CARTESIAN_POINT('Ctrl Pts',(121.962987211232,-27.7910849150435,-25.9526072839584));
#75661=CARTESIAN_POINT('Ctrl Pts',(121.991329280155,-27.7426854760792,-25.9042078449942));
#75662=CARTESIAN_POINT('Ctrl Pts',(122.,-27.7118487512525,-25.8733711201675));
#75663=CARTESIAN_POINT('Ctrl Pts',(122.,-27.685648477063,-25.8471708459779));
#75664=CARTESIAN_POINT('Origin',(121.912132034356,0.,0.));
#75665=CARTESIAN_POINT('Origin',(121.7,-22.6046480406385,-30.0060517970005));
#75666=CARTESIAN_POINT('',(121.7,-22.8426540427259,-30.1886802257031));
#75667=CARTESIAN_POINT('Origin',(103.5,-28.9573969206301,-22.2197921588183));
#75668=CARTESIAN_POINT('',(104.3,-21.916177849104,-31.3960875085644));
#75669=CARTESIAN_POINT('Origin',(113.,-32.2531390339859,-20.468879364889));
#75670=CARTESIAN_POINT('',(121.811388243054,-32.4031390339859,-20.2090717437536));
#75671=CARTESIAN_POINT('Ctrl Pts',(121.5,-32.5064359373941,-20.6296297263933));
#75672=CARTESIAN_POINT('Ctrl Pts',(121.5,-32.5175778592339,-20.612073222796));
#75673=CARTESIAN_POINT('Ctrl Pts',(121.502178291748,-32.5269590323472,-20.5931936538549));
#75674=CARTESIAN_POINT('Ctrl Pts',(121.510716614322,-32.541490563393,-20.5542390480232));
#75675=CARTESIAN_POINT('Ctrl Pts',(121.517077828304,-32.546639697538,-20.5341638139643));
#75676=CARTESIAN_POINT('Ctrl Pts',(121.541159186122,-32.555772639402,-20.4745077018041));
#75677=CARTESIAN_POINT('Ctrl Pts',(121.56412779323,-32.553196494323,-20.4354165429558));
#75678=CARTESIAN_POINT('Ctrl Pts',(121.617288389766,-32.5364820278348,-20.3619926475953));
#75679=CARTESIAN_POINT('Ctrl Pts',(121.652509215907,-32.5187625223814,-20.3238857140478));
#75680=CARTESIAN_POINT('Ctrl Pts',(121.726559498935,-32.4716751410544,-20.2594868158067));
#75681=CARTESIAN_POINT('Ctrl Pts',(121.765406035132,-32.4422479143698,-20.233257916631));
#75682=CARTESIAN_POINT('Ctrl Pts',(121.804557793905,-32.4090274474393,-20.2125393068328));
#75683=CARTESIAN_POINT('Ctrl Pts',(121.807962616873,-32.4061082016311,-20.2107859993603));
#75684=CARTESIAN_POINT('Ctrl Pts',(121.811388687965,-32.4031394190667,-20.2090719660805));
#75685=CARTESIAN_POINT('',(113.,-32.4031390339859,-20.2090717437536));
#75686=CARTESIAN_POINT('Origin',(113.,-32.0424589928626,-20.0008330249198));
#75687=CARTESIAN_POINT('',(121.912131484566,-32.315842392183,-20.1586710041094));
#75688=CARTESIAN_POINT('',(121.75,-32.4563335449461,-20.2397836089759));
#75689=CARTESIAN_POINT('Ctrl Pts',(122.,-32.1320229585134,-20.052542804598));
#75690=CARTESIAN_POINT('Ctrl Pts',(122.,-32.1641116099562,-20.0710691961464));
#75691=CARTESIAN_POINT('Ctrl Pts',(121.991329280155,-32.2018787305382,-20.0928740533809));
#75692=CARTESIAN_POINT('Ctrl Pts',(121.962987211232,-32.2611556951879,-20.1270976248782));
#75693=CARTESIAN_POINT('Ctrl Pts',(121.938311286558,-32.293157335936,-20.1455737807786));
#75694=CARTESIAN_POINT('Ctrl Pts',(121.912131759621,-32.3158426302492,-20.1586711415569));
#75695=CARTESIAN_POINT('',(121.7,-30.959927238132,-19.3758330249198));
#75696=CARTESIAN_POINT('Origin',(121.7,-30.7001196169967,-19.2258330249198));
#75697=CARTESIAN_POINT('',(103.5,-30.959927238132,-19.3758330249198));
#75698=CARTESIAN_POINT('Origin',(121.7,0.,0.));
#75699=CARTESIAN_POINT('Origin',(121.912132034356,-2.22044604925031E-15,
4.44089209850063E-15));
#75700=CARTESIAN_POINT('Origin',(121.7,-27.2251196169967,-25.2447095812216));
#75701=CARTESIAN_POINT('',(121.7,-27.484927238132,-25.3947095812216));
#75702=CARTESIAN_POINT('Origin',(103.5,-31.609927238132,-18.25));
#75703=CARTESIAN_POINT('',(104.3,-32.259927238132,-17.1241669750802));
#75704=CARTESIAN_POINT('',(103.5,-32.259927238132,-17.1241669750802));
#75705=CARTESIAN_POINT('',(104.3,-26.859927238132,-26.4772413359522));
#75706=CARTESIAN_POINT('Origin',(113.,-33.3424589928626,-17.7491669750802));
#75707=CARTESIAN_POINT('',(104.188611756946,-33.7031390339859,-17.9574056939141));
#75708=CARTESIAN_POINT('',(113.,-33.7031390339859,-17.9574056939141));
#75709=CARTESIAN_POINT('',(104.087868515434,-33.615842392183,-17.9070049542698));
#75710=CARTESIAN_POINT('',(104.25,-33.7563335449461,-17.9881175591364));
#75711=CARTESIAN_POINT('Ctrl Pts',(104.,-33.4320229585134,-17.8008767547584));
#75712=CARTESIAN_POINT('Ctrl Pts',(104.,-33.4641116099561,-17.8194031463068));
#75713=CARTESIAN_POINT('Ctrl Pts',(104.008670719845,-33.5018787305382,-17.8412080035414));
#75714=CARTESIAN_POINT('Ctrl Pts',(104.037012788768,-33.5611556951878,-17.8754315750386));
#75715=CARTESIAN_POINT('Ctrl Pts',(104.061688713442,-33.593157335936,-17.8939077309391));
#75716=CARTESIAN_POINT('Ctrl Pts',(104.087868240379,-33.6158426302492,-17.9070050917174));
#75717=CARTESIAN_POINT('Origin',(104.3,-32.0001196169967,-16.9741669750802));
#75718=CARTESIAN_POINT('Origin',(121.7,0.,0.));
#75719=CARTESIAN_POINT('Origin',(121.912132034356,-2.22044604925031E-15,
3.33066907387547E-15));
#75720=CARTESIAN_POINT('Origin',(121.7,-33.8612244928859,-13.4942494327112));
#75721=CARTESIAN_POINT('',(121.7,-34.1510022407726,-13.571895146242));
#75722=CARTESIAN_POINT('Origin',(103.5,-35.256292659551,-9.44689514624199));
#75723=CARTESIAN_POINT('',(104.3,-33.9835339955032,-14.196895146242));
#75724=CARTESIAN_POINT('Origin',(121.7,0.,0.));
#75725=CARTESIAN_POINT('Origin',(121.912132034356,0.,1.66533453693773E-15));
#75726=CARTESIAN_POINT('Origin',(113.,-38.0487998398672,3.39541319219319));
#75727=CARTESIAN_POINT('',(121.811388243054,-38.0096419822012,3.69284665060534));
#75728=CARTESIAN_POINT('Ctrl Pts',(121.5,-38.3476124040547,3.42207874082298));
#75729=CARTESIAN_POINT('Ctrl Pts',(121.5,-38.3457641627452,3.44279002385684));
#75730=CARTESIAN_POINT('Ctrl Pts',(121.502178291748,-38.3417135944028,3.46347908928975));
#75731=CARTESIAN_POINT('Ctrl Pts',(121.510716614322,-38.329528171585,3.50323009155113));
#75732=CARTESIAN_POINT('Ctrl Pts',(121.517077828304,-38.3213922261851,3.52229143980919));
#75733=CARTESIAN_POINT('Ctrl Pts',(121.541159186122,-38.2923215360319,3.57517959840044));
#75734=CARTESIAN_POINT('Ctrl Pts',(121.56412779323,-38.2664805530063,3.60462444208901));
#75735=CARTESIAN_POINT('Ctrl Pts',(121.617288389766,-38.2085224397236,3.652700412226));
#75736=CARTESIAN_POINT('Ctrl Pts',(121.652509215907,-38.1712665795624,3.67214572378298));
#75737=CARTESIAN_POINT('Ctrl Pts',(121.726559498935,-38.0947060829812,3.69457182326874));
#75738=CARTESIAN_POINT('Ctrl Pts',(121.765406035132,-38.0553927522519,3.69746644747365));
#75739=CARTESIAN_POINT('Ctrl Pts',(121.804557793905,-38.0164244933388,3.69368028684233));
#75740=CARTESIAN_POINT('Ctrl Pts',(121.807962616873,-38.0130411539632,3.69329415493236));
#75741=CARTESIAN_POINT('Ctrl Pts',(121.811388687965,-38.0096424230504,3.6928467086439));
#75742=CARTESIAN_POINT('',(113.,-38.0096419822012,3.69284665060534));
#75743=CARTESIAN_POINT('Origin',(113.,-37.5967275667474,3.63848543652101));
#75744=CARTESIAN_POINT('',(121.912131484566,-37.9097028735418,3.67968941734367));
#75745=CARTESIAN_POINT('',(121.75,-38.0705402241169,3.70086405625222));
#75746=CARTESIAN_POINT('Ctrl Pts',(122.,-37.6992623574369,3.65198439780488));
#75747=CARTESIAN_POINT('Ctrl Pts',(122.,-37.7359981488378,3.65682075649366));
#75748=CARTESIAN_POINT('Ctrl Pts',(121.991329280155,-37.7792347761542,3.66251296646712));
#75749=CARTESIAN_POINT('Ctrl Pts',(121.962987211232,-37.8470963443517,3.67144711141052));
#75750=CARTESIAN_POINT('Ctrl Pts',(121.938311286558,-37.8837325240027,3.67627035596363));
#75751=CARTESIAN_POINT('Ctrl Pts',(121.912131759621,-37.9097031460851,3.67968945322468));
#75752=CARTESIAN_POINT('',(121.7,-36.3574214900301,3.47532769624594));
#75753=CARTESIAN_POINT('Origin',(121.7,-36.059988031618,3.43616983857993));
#75754=CARTESIAN_POINT('',(103.5,-36.3574214900301,3.47532769624594));
#75755=CARTESIAN_POINT('Ctrl Pts',(121.375735931288,-38.0096419822012,-3.69284665060532));
#75756=CARTESIAN_POINT('Ctrl Pts',(121.48382436112,-37.9023841393222,-3.67872588770445));
#75757=CARTESIAN_POINT('Ctrl Pts',(121.591912387511,-37.7951258968034,-3.66460507219002));
#75758=CARTESIAN_POINT('Ctrl Pts',(121.699999999995,-37.6878672442858,-3.65048420269822));
#75759=CARTESIAN_POINT('Ctrl Pts',(121.432344074477,-38.0657165831673,-3.70022901187372));
#75760=CARTESIAN_POINT('Ctrl Pts',(121.540435642306,-37.9584615504213,-3.68610876488971));
#75761=CARTESIAN_POINT('Ctrl Pts',(121.648526737396,-37.8512061044813,-3.67198802305841));
#75762=CARTESIAN_POINT('Ctrl Pts',(121.756617543135,-37.7439503091645,-3.65786767826186));
#75763=CARTESIAN_POINT('Ctrl Pts',(121.544997455782,-38.186147098729,-3.64778211360281));
#75764=CARTESIAN_POINT('Ctrl Pts',(121.653095005438,-38.0788984389098,-3.63365497063291));
#75765=CARTESIAN_POINT('Ctrl Pts',(121.761192358011,-37.97164956428,-3.61952784772081));
#75766=CARTESIAN_POINT('Ctrl Pts',(121.869289250808,-37.8644002490186,-3.60540048647973));
#75767=CARTESIAN_POINT('Ctrl Pts',(121.589544531169,-38.2513127544414,-3.49378871787998));
#75768=CARTESIAN_POINT('Ctrl Pts',(121.697637909657,-38.1440615207735,-3.47964747605769));
#75769=CARTESIAN_POINT('Ctrl Pts',(121.805730586267,-38.0368096023995,-3.46550601417652));
#75770=CARTESIAN_POINT('Ctrl Pts',(121.913823234174,-37.9295576652633,-3.45136431096224));
#75771=CARTESIAN_POINT('Ctrl Pts',(121.587867965644,-38.2600922303079,-3.41426858245336));
#75772=CARTESIAN_POINT('Ctrl Pts',(121.695956395476,-38.1528366240338,-3.40012275628983));
#75773=CARTESIAN_POINT('Ctrl Pts',(121.804044421867,-38.0455806326541,-3.38597666428455));
#75774=CARTESIAN_POINT('Ctrl Pts',(121.912132034351,-37.9383242460686,-3.37183029953946));
#75775=CARTESIAN_POINT('',(121.699999999995,-37.6878672442858,-3.65048420269822));
#75776=CARTESIAN_POINT('Origin',(121.699999999995,-37.7270251019518,-3.35305074428608));
#75777=CARTESIAN_POINT('',(121.375735931288,-38.0096419822012,-3.69284665060532));
#75778=CARTESIAN_POINT('Origin',(121.375735931288,-38.0487998398673,-3.39541319219318));
#75779=CARTESIAN_POINT('Ctrl Pts',(121.375735931288,-38.0096419822012,-3.69284665060532));
#75780=CARTESIAN_POINT('Ctrl Pts',(121.48382436112,-37.9023841393222,-3.67872588770445));
#75781=CARTESIAN_POINT('Ctrl Pts',(121.591912387511,-37.7951258968034,-3.66460507219002));
#75782=CARTESIAN_POINT('Ctrl Pts',(121.699999999995,-37.6878672442858,-3.65048420269822));
#75783=CARTESIAN_POINT('Origin',(121.375735931288,-38.0487998398672,-3.39541319219318));
#75784=CARTESIAN_POINT('Origin',(121.375735931288,-38.0487998398672,-3.39541319219318));
#75785=CARTESIAN_POINT('Origin',(121.7,-2.70347559909794,1.25788702214042));
#75786=CARTESIAN_POINT('Origin',(121.7,-37.7270251019467,-3.3530507442854));
#75787=CARTESIAN_POINT('',(121.7,-36.3574214900301,-3.47532769624592));
#75788=CARTESIAN_POINT('',(121.7,-2.66431774143193,0.960453563728277));
#75789=CARTESIAN_POINT('Origin',(121.7,-36.099145889284,-3.13873638016776));
#75790=CARTESIAN_POINT('Origin',(121.7,-37.7270251019467,-3.35305074428562));
#75791=CARTESIAN_POINT('Origin',(121.7,-35.6091920486168,-6.86030528046165));
#75792=CARTESIAN_POINT('',(121.7,-35.9066255070289,-6.89946313812766));
#75793=CARTESIAN_POINT('Origin',(103.5,-36.1877374401441,-4.76420601603187));
#75794=CARTESIAN_POINT('',(103.5,-36.3574214900301,-3.47532769624592));
#75795=CARTESIAN_POINT('',(104.3,-35.8640327898902,-7.22298694450581));
#75796=CARTESIAN_POINT('Origin',(113.,-37.5967275667474,-3.63848543652098));
#75797=CARTESIAN_POINT('',(113.,-38.0096419822012,-3.69284665060532));
#75798=CARTESIAN_POINT('Origin',(121.7,0.,0.));
#75799=CARTESIAN_POINT('Origin',(121.912132034356,0.,-1.11022302462516E-15));
#75800=CARTESIAN_POINT('Origin',(121.7,-35.6091920486168,6.86030528046169));
#75801=CARTESIAN_POINT('',(121.7,-36.018053390258,6.05308433581785));
#75802=CARTESIAN_POINT('Origin',(121.7,-35.7206199318459,6.01392647815184));
#75803=CARTESIAN_POINT('',(121.7,-35.9066255070289,6.8994631381277));
#75804=CARTESIAN_POINT('Origin',(103.5,-36.1877374401441,4.7642060160319));
#75805=CARTESIAN_POINT('',(103.5,-36.018053390258,6.05308433581785));
#75806=CARTESIAN_POINT('',(104.3,-35.8640327898902,7.22298694450585));
#75807=CARTESIAN_POINT('Origin',(121.7,0.,0.));
#75808=CARTESIAN_POINT('',(121.912131484566,-37.5703347737697,6.25744605691558));
#75809=CARTESIAN_POINT('Ctrl Pts',(121.912131759621,-37.570335046313,6.25744609279659));
#75810=CARTESIAN_POINT('Ctrl Pts',(121.938311286558,-37.5443644242305,6.25402699553553));
#75811=CARTESIAN_POINT('Ctrl Pts',(121.962987211232,-37.5077282445796,6.24920375098243));
#75812=CARTESIAN_POINT('Ctrl Pts',(121.991329280155,-37.439866676382,6.24026960603902));
#75813=CARTESIAN_POINT('Ctrl Pts',(122.,-37.3966300490657,6.23457739606557));
#75814=CARTESIAN_POINT('Ctrl Pts',(122.,-37.3598942576648,6.22974103737679));
#75815=CARTESIAN_POINT('Origin',(121.912132034356,0.,-5.55111512312578E-16));
#75816=CARTESIAN_POINT('Origin',(121.7,-33.8612244928859,13.4942494327113));
#75817=CARTESIAN_POINT('',(121.7,-34.1510022407726,13.571895146242));
#75818=CARTESIAN_POINT('Origin',(103.5,-35.256292659551,9.44689514624202));
#75819=CARTESIAN_POINT('',(104.3,-34.9198279009177,10.7025987204178));
#75820=CARTESIAN_POINT('',(103.5,-34.9198279009177,10.7025987204178));
#75821=CARTESIAN_POINT('',(104.3,-33.9835339955032,14.196895146242));
#75822=CARTESIAN_POINT('Origin',(113.,-36.127235183779,11.026122526796));
#75823=CARTESIAN_POINT('',(104.188611756946,-36.529521496889,11.1339148195199));
#75824=CARTESIAN_POINT('',(113.,-36.529521496889,11.1339148195199));
#75825=CARTESIAN_POINT('',(104.087868515434,-36.4321547447161,11.1078254769055));
#75826=CARTESIAN_POINT('',(104.25,-36.5888522644724,11.1498124507802));
#75827=CARTESIAN_POINT('Ctrl Pts',(104.,-36.2271308071048,11.0528894783935));
#75828=CARTESIAN_POINT('Ctrl Pts',(104.,-36.2629210472339,11.062479444333));
#75829=CARTESIAN_POINT('Ctrl Pts',(104.008670719845,-36.3050447967167,11.0737664689891));
#75830=CARTESIAN_POINT('Ctrl Pts',(104.037012788768,-36.3711596598708,11.0914818931789));
#75831=CARTESIAN_POINT('Ctrl Pts',(104.061688713442,-36.4068528521804,11.1010458552336));
#75832=CARTESIAN_POINT('Ctrl Pts',(104.087868240379,-36.4321550102444,11.1078255480536));
#75833=CARTESIAN_POINT('Origin',(104.3,-34.630050153031,10.624953006887));
#75834=CARTESIAN_POINT('Origin',(113.,-33.8531390339859,17.6975980727788));
#75835=CARTESIAN_POINT('',(121.811388243054,-33.7031390339859,17.9574056939141));
#75836=CARTESIAN_POINT('Ctrl Pts',(121.5,-34.1190013824203,17.8365844450781));
#75837=CARTESIAN_POINT('Ctrl Pts',(121.5,-34.1093679652233,17.855011884237));
#75838=CARTESIAN_POINT('Ctrl Pts',(121.502178291748,-34.0977083654644,17.8725760029409));
#75839=CARTESIAN_POINT('Ctrl Pts',(121.510716614322,-34.0712384527426,17.9046379808983));
#75840=CARTESIAN_POINT('Ctrl Pts',(121.517077828304,-34.0564273571332,17.9191348789048));
#75841=CARTESIAN_POINT('Ctrl Pts',(121.541159186122,-34.0093301194435,17.9568722946504));
#75842=CARTESIAN_POINT('Ctrl Pts',(121.56412779323,-33.974188110278,17.9741868669924));
#75843=CARTESIAN_POINT('Ctrl Pts',(121.617288389766,-33.9022439184069,17.9964236620831));
#75844=CARTESIAN_POINT('Ctrl Pts',(121.652509215907,-33.8603825931677,18.0001315869917));
#75845=CARTESIAN_POINT('Ctrl Pts',(121.726559498935,-33.7810678206517,17.9915521676854));
#75846=CARTESIAN_POINT('Ctrl Pts',(121.765406035132,-33.7436393143099,17.9791818914014));
#75847=CARTESIAN_POINT('Ctrl Pts',(121.804557793905,-33.7090862384283,17.9607714280132));
#75848=CARTESIAN_POINT('Ctrl Pts',(121.807962616873,-33.7061082067124,17.9591199407196));
#75849=CARTESIAN_POINT('Ctrl Pts',(121.811388687965,-33.703139419067,17.9574059162404));
#75850=CARTESIAN_POINT('',(113.,-33.7031390339859,17.9574056939141));
#75851=CARTESIAN_POINT('Origin',(113.,-33.3424589928626,17.7491669750802));
#75852=CARTESIAN_POINT('',(121.912131484566,-33.615842392183,17.9070049542699));
#75853=CARTESIAN_POINT('',(121.75,-33.756333544946,17.9881175591364));
#75854=CARTESIAN_POINT('Ctrl Pts',(122.,-33.4320229585134,17.8008767547585));
#75855=CARTESIAN_POINT('Ctrl Pts',(122.,-33.4641116099562,17.8194031463069));
#75856=CARTESIAN_POINT('Ctrl Pts',(121.991329280155,-33.5018787305382,17.8412080035414));
#75857=CARTESIAN_POINT('Ctrl Pts',(121.962987211232,-33.5611556951879,17.8754315750386));
#75858=CARTESIAN_POINT('Ctrl Pts',(121.938311286558,-33.593157335936,17.8939077309391));
#75859=CARTESIAN_POINT('Ctrl Pts',(121.912131759621,-33.6158426302491,17.9070050917174));
#75860=CARTESIAN_POINT('',(121.7,-32.259927238132,17.1241669750802));
#75861=CARTESIAN_POINT('Origin',(121.7,-32.0001196169967,16.9741669750802));
#75862=CARTESIAN_POINT('',(103.5,-32.259927238132,17.1241669750802));
#75863=CARTESIAN_POINT('Origin',(121.7,0.,0.));
#75864=CARTESIAN_POINT('Origin',(121.912132034356,0.,-1.11022302462516E-15));
#75865=CARTESIAN_POINT('Origin',(121.7,-27.2251196169967,25.2447095812216));
#75866=CARTESIAN_POINT('',(121.7,-27.484927238132,25.3947095812216));
#75867=CARTESIAN_POINT('Origin',(103.5,-31.609927238132,18.25));
#75868=CARTESIAN_POINT('',(104.3,-26.859927238132,26.4772413359522));
#75869=CARTESIAN_POINT('Origin',(121.7,0.,0.));
#75870=CARTESIAN_POINT('Origin',(121.912132034356,0.,0.));
#75871=CARTESIAN_POINT('Origin',(121.7,-22.6046480406385,30.0060517970005));
#75872=CARTESIAN_POINT('',(121.7,-22.8426540427259,30.1886802257031));
#75873=CARTESIAN_POINT('Origin',(103.5,-28.9573969206301,22.2197921588183));
#75874=CARTESIAN_POINT('',(104.3,-28.1660070629187,23.2511515011969));
#75875=CARTESIAN_POINT('',(103.5,-28.1660070629187,23.2511515011969));
#75876=CARTESIAN_POINT('',(104.3,-21.916177849104,31.3960875085645));
#75877=CARTESIAN_POINT('Origin',(113.,-29.1576987382828,24.0121032874578));
#75878=CARTESIAN_POINT('',(104.188611756946,-29.4881125046124,24.2656386875623));
#75879=CARTESIAN_POINT('',(113.,-29.4881125046124,24.2656386875623));
#75880=CARTESIAN_POINT('',(104.087868515434,-29.4081413143126,24.2042746349845));
#75881=CARTESIAN_POINT('',(104.25,-29.5368432263338,24.3030310854828));
#75882=CARTESIAN_POINT('Ctrl Pts',(104.,-29.2397469911496,24.0750611261991));
#75883=CARTESIAN_POINT('Ctrl Pts',(104.,-29.2691429403866,24.0976174313858));
#75884=CARTESIAN_POINT('Ctrl Pts',(104.008670719845,-29.3037408530298,24.1241653434847));
#75885=CARTESIAN_POINT('Ctrl Pts',(104.037012788768,-29.3580436225578,24.1658333240656));
#75886=CARTESIAN_POINT('Ctrl Pts',(104.061688713442,-29.3873598625566,24.1883284662027));
#75887=CARTESIAN_POINT('Ctrl Pts',(104.087868240379,-29.4081415324016,24.20427480233));
#75888=CARTESIAN_POINT('Origin',(104.3,-27.9280010608314,23.0685230724943));
#75889=CARTESIAN_POINT('Origin',(121.7,0.,0.));
#75890=CARTESIAN_POINT('Origin',(121.912132034356,-2.22044604925031E-15,
-2.22044604925031E-15));
#75891=CARTESIAN_POINT('Origin',(121.7,-11.6519066080199,36.6882789854275));
#75892=CARTESIAN_POINT('',(121.7,-11.8345350367225,36.9262849875149));
#75893=CARTESIAN_POINT('Origin',(103.5,-22.2197921588183,28.9573969206301));
#75894=CARTESIAN_POINT('',(104.3,-10.2610112303443,38.1336922703762));
#75895=CARTESIAN_POINT('Origin',(113.,-20.468879364889,32.2531390339859));
#75896=CARTESIAN_POINT('',(121.811388243054,-20.2090717437536,32.4031390339859));
#75897=CARTESIAN_POINT('Ctrl Pts',(121.5,-20.6296297263933,32.5064359373941));
#75898=CARTESIAN_POINT('Ctrl Pts',(121.5,-20.612073222796,32.5175778592339));
#75899=CARTESIAN_POINT('Ctrl Pts',(121.502178291748,-20.5931936538549,32.5269590323472));
#75900=CARTESIAN_POINT('Ctrl Pts',(121.510716614322,-20.5542390480232,32.5414905633929));
#75901=CARTESIAN_POINT('Ctrl Pts',(121.517077828304,-20.5341638139643,32.546639697538));
#75902=CARTESIAN_POINT('Ctrl Pts',(121.541159186122,-20.4745077018041,32.555772639402));
#75903=CARTESIAN_POINT('Ctrl Pts',(121.56412779323,-20.4354165429558,32.553196494323));
#75904=CARTESIAN_POINT('Ctrl Pts',(121.617288389766,-20.3619926475953,32.5364820278348));
#75905=CARTESIAN_POINT('Ctrl Pts',(121.652509215907,-20.3238857140478,32.5187625223814));
#75906=CARTESIAN_POINT('Ctrl Pts',(121.726559498935,-20.2594868158067,32.4716751410544));
#75907=CARTESIAN_POINT('Ctrl Pts',(121.765406035132,-20.233257916631,32.4422479143698));
#75908=CARTESIAN_POINT('Ctrl Pts',(121.804557793905,-20.2125393068328,32.4090274474393));
#75909=CARTESIAN_POINT('Ctrl Pts',(121.807962616873,-20.2107859993603,32.4061082016311));
#75910=CARTESIAN_POINT('Ctrl Pts',(121.811388687965,-20.2090719660805,32.4031394190667));
#75911=CARTESIAN_POINT('',(113.,-20.2090717437536,32.4031390339859));
#75912=CARTESIAN_POINT('Origin',(113.,-20.0008330249198,32.0424589928626));
#75913=CARTESIAN_POINT('',(121.912131484566,-20.1586710041094,32.315842392183));
#75914=CARTESIAN_POINT('',(121.75,-20.2397836089759,32.4563335449461));
#75915=CARTESIAN_POINT('Ctrl Pts',(122.,-20.052542804598,32.1320229585134));
#75916=CARTESIAN_POINT('Ctrl Pts',(122.,-20.0710691961464,32.1641116099562));
#75917=CARTESIAN_POINT('Ctrl Pts',(121.991329280155,-20.0928740533809,32.2018787305382));
#75918=CARTESIAN_POINT('Ctrl Pts',(121.962987211232,-20.1270976248782,32.2611556951879));
#75919=CARTESIAN_POINT('Ctrl Pts',(121.938311286558,-20.1455737807786,32.293157335936));
#75920=CARTESIAN_POINT('Ctrl Pts',(121.912131759621,-20.158671141557,32.3158426302492));
#75921=CARTESIAN_POINT('',(121.7,-19.3758330249198,30.959927238132));
#75922=CARTESIAN_POINT('Origin',(121.7,-19.2258330249198,30.7001196169967));
#75923=CARTESIAN_POINT('',(103.5,-19.3758330249198,30.959927238132));
#75924=CARTESIAN_POINT('Origin',(121.7,0.,0.));
#75925=CARTESIAN_POINT('Origin',(121.912132034356,-2.22044604925031E-15,
-2.22044604925031E-15));
#75926=CARTESIAN_POINT('Origin',(121.7,-5.72499999999999,38.4948291982183));
#75927=CARTESIAN_POINT('',(121.7,-5.87499999999999,38.7546368193536));
#75928=CARTESIAN_POINT('Origin',(103.5,-18.25,31.609927238132));
#75929=CARTESIAN_POINT('',(104.3,-17.1241669750802,32.259927238132));
#75930=CARTESIAN_POINT('',(103.5,-17.1241669750802,32.259927238132));
#75931=CARTESIAN_POINT('',(104.3,-3.99999999999999,39.8371685740842));
#75932=CARTESIAN_POINT('Origin',(113.,-17.7491669750802,33.3424589928626));
#75933=CARTESIAN_POINT('',(104.188611756946,-17.9574056939141,33.7031390339859));
#75934=CARTESIAN_POINT('',(113.,-17.9574056939141,33.7031390339859));
#75935=CARTESIAN_POINT('',(104.087868515434,-17.9070049542699,33.615842392183));
#75936=CARTESIAN_POINT('',(104.25,-17.9881175591364,33.7563335449461));
#75937=CARTESIAN_POINT('Ctrl Pts',(104.,-17.8008767547584,33.4320229585134));
#75938=CARTESIAN_POINT('Ctrl Pts',(104.,-17.8194031463068,33.4641116099561));
#75939=CARTESIAN_POINT('Ctrl Pts',(104.008670719845,-17.8412080035414,33.5018787305382));
#75940=CARTESIAN_POINT('Ctrl Pts',(104.037012788768,-17.8754315750386,33.5611556951878));
#75941=CARTESIAN_POINT('Ctrl Pts',(104.061688713442,-17.8939077309391,33.593157335936));
#75942=CARTESIAN_POINT('Ctrl Pts',(104.087868240379,-17.9070050917174,33.6158426302491));
#75943=CARTESIAN_POINT('Origin',(104.3,-16.9741669750802,32.0001196169967));
#75944=CARTESIAN_POINT('Origin',(121.7,0.,0.));
#75945=CARTESIAN_POINT('Origin',(121.912132034356,0.,0.));
#75946=CARTESIAN_POINT('Origin',(121.7,6.02546014851037,39.0915149116643));
#75947=CARTESIAN_POINT('',(121.7,5.94781443497962,39.381292659551));
#75948=CARTESIAN_POINT('Origin',(103.5,-9.446895146242,35.256292659551));
#75949=CARTESIAN_POINT('',(104.3,8.28034618971017,40.006292659551));
#75950=CARTESIAN_POINT('Origin',(121.7,0.,0.));
#75951=CARTESIAN_POINT('Origin',(121.912132034356,-1.66533453693773E-15,
0.));
#75952=CARTESIAN_POINT('Origin',(113.,3.39541319219319,38.0487998398672));
#75953=CARTESIAN_POINT('',(121.811388243054,3.69284665060533,38.0096419822012));
#75954=CARTESIAN_POINT('Ctrl Pts',(121.5,3.42207874082298,38.3476124040547));
#75955=CARTESIAN_POINT('Ctrl Pts',(121.5,3.44279002385683,38.3457641627452));
#75956=CARTESIAN_POINT('Ctrl Pts',(121.502178291748,3.46347908928974,38.3417135944028));
#75957=CARTESIAN_POINT('Ctrl Pts',(121.510716614322,3.50323009155112,38.329528171585));
#75958=CARTESIAN_POINT('Ctrl Pts',(121.517077828304,3.52229143980918,38.3213922261851));
#75959=CARTESIAN_POINT('Ctrl Pts',(121.541159186122,3.57517959840044,38.2923215360319));
#75960=CARTESIAN_POINT('Ctrl Pts',(121.56412779323,3.60462444208901,38.2664805530063));
#75961=CARTESIAN_POINT('Ctrl Pts',(121.617288389766,3.652700412226,38.2085224397236));
#75962=CARTESIAN_POINT('Ctrl Pts',(121.652509215907,3.67214572378298,38.1712665795624));
#75963=CARTESIAN_POINT('Ctrl Pts',(121.726559498935,3.69457182326873,38.0947060829812));
#75964=CARTESIAN_POINT('Ctrl Pts',(121.765406035132,3.69746644747365,38.0553927522519));
#75965=CARTESIAN_POINT('Ctrl Pts',(121.804557793905,3.69368028684233,38.0164244933388));
#75966=CARTESIAN_POINT('Ctrl Pts',(121.807962616873,3.69329415493236,38.0130411539632));
#75967=CARTESIAN_POINT('Ctrl Pts',(121.811388687965,3.69284670864389,38.0096424230504));
#75968=CARTESIAN_POINT('',(113.,3.69284665060533,38.0096419822012));
#75969=CARTESIAN_POINT('Origin',(113.,3.638485436521,37.5967275667474));
#75970=CARTESIAN_POINT('',(121.912131484566,3.67968941734366,37.9097028735418));
#75971=CARTESIAN_POINT('',(121.75,3.70086405625221,38.0705402241169));
#75972=CARTESIAN_POINT('Ctrl Pts',(122.,3.65198439780487,37.6992623574369));
#75973=CARTESIAN_POINT('Ctrl Pts',(122.,3.65682075649365,37.7359981488378));
#75974=CARTESIAN_POINT('Ctrl Pts',(121.991329280155,3.66251296646711,37.7792347761542));
#75975=CARTESIAN_POINT('Ctrl Pts',(121.962987211232,3.67144711141051,37.8470963443518));
#75976=CARTESIAN_POINT('Ctrl Pts',(121.938311286558,3.67627035596362,37.8837325240027));
#75977=CARTESIAN_POINT('Ctrl Pts',(121.912131759621,3.67968945322467,37.9097031460851));
#75978=CARTESIAN_POINT('',(121.7,3.47532769624593,36.3574214900301));
#75979=CARTESIAN_POINT('Origin',(121.7,3.43616983857992,36.059988031618));
#75980=CARTESIAN_POINT('',(103.5,3.47532769624593,36.3574214900301));
#75981=CARTESIAN_POINT('Ctrl Pts',(121.375735931288,-3.69284665060532,38.0096419822012));
#75982=CARTESIAN_POINT('Ctrl Pts',(121.48382436112,-3.67872588770446,37.9023841393222));
#75983=CARTESIAN_POINT('Ctrl Pts',(121.591912387511,-3.66460507219003,37.7951258968034));
#75984=CARTESIAN_POINT('Ctrl Pts',(121.699999999995,-3.65048420269823,37.6878672442858));
#75985=CARTESIAN_POINT('Ctrl Pts',(121.432344074477,-3.70022901187372,38.0657165831673));
#75986=CARTESIAN_POINT('Ctrl Pts',(121.540435642306,-3.68610876488972,37.9584615504213));
#75987=CARTESIAN_POINT('Ctrl Pts',(121.648526737396,-3.67198802305842,37.8512061044813));
#75988=CARTESIAN_POINT('Ctrl Pts',(121.756617543135,-3.65786767826187,37.7439503091645));
#75989=CARTESIAN_POINT('Ctrl Pts',(121.544997455782,-3.64778211360281,38.186147098729));
#75990=CARTESIAN_POINT('Ctrl Pts',(121.653095005438,-3.63365497063291,38.0788984389098));
#75991=CARTESIAN_POINT('Ctrl Pts',(121.761192358011,-3.61952784772082,37.97164956428));
#75992=CARTESIAN_POINT('Ctrl Pts',(121.869289250808,-3.60540048647974,37.8644002490187));
#75993=CARTESIAN_POINT('Ctrl Pts',(121.589544531169,-3.49378871787998,38.2513127544414));
#75994=CARTESIAN_POINT('Ctrl Pts',(121.697637909657,-3.4796474760577,38.1440615207735));
#75995=CARTESIAN_POINT('Ctrl Pts',(121.805730586267,-3.46550601417653,38.0368096023995));
#75996=CARTESIAN_POINT('Ctrl Pts',(121.913823234174,-3.45136431096225,37.9295576652634));
#75997=CARTESIAN_POINT('Ctrl Pts',(121.587867965644,-3.41426858245336,38.2600922303079));
#75998=CARTESIAN_POINT('Ctrl Pts',(121.695956395476,-3.40012275628983,38.1528366240338));
#75999=CARTESIAN_POINT('Ctrl Pts',(121.804044421867,-3.38597666428456,38.0455806326541));
#76000=CARTESIAN_POINT('Ctrl Pts',(121.912132034351,-3.37183029953947,37.9383242460686));
#76001=CARTESIAN_POINT('',(121.699999999995,-3.65048420269823,37.6878672442858));
#76002=CARTESIAN_POINT('Origin',(121.699999999995,-3.35305074428609,37.7270251019519));
#76003=CARTESIAN_POINT('',(121.375735931288,-3.69284665060532,38.0096419822012));
#76004=CARTESIAN_POINT('Origin',(121.375735931288,-3.39541319219318,38.0487998398672));
#76005=CARTESIAN_POINT('Ctrl Pts',(121.375735931288,-3.69284665060532,38.0096419822012));
#76006=CARTESIAN_POINT('Ctrl Pts',(121.48382436112,-3.67872588770446,37.9023841393222));
#76007=CARTESIAN_POINT('Ctrl Pts',(121.591912387511,-3.66460507219003,37.7951258968034));
#76008=CARTESIAN_POINT('Ctrl Pts',(121.699999999995,-3.65048420269823,37.6878672442858));
#76009=CARTESIAN_POINT('Origin',(121.375735931288,-3.39541319219318,38.0487998398672));
#76010=CARTESIAN_POINT('Origin',(121.375735931288,-3.39541319219318,38.0487998398672));
#76011=CARTESIAN_POINT('Origin',(121.7,-0.596258166840185,16.787106543887));
#76012=CARTESIAN_POINT('Origin',(121.7,-3.3530507442854,37.7270251019467));
#76013=CARTESIAN_POINT('',(121.7,-3.47532769624592,36.3574214900301));
#76014=CARTESIAN_POINT('',(121.7,-0.893691625252331,16.7479486862209));
#76015=CARTESIAN_POINT('Origin',(121.7,-3.13873638016776,36.099145889284));
#76016=CARTESIAN_POINT('Origin',(121.7,-3.35305074428562,37.7270251019467));
#76017=CARTESIAN_POINT('Origin',(121.7,11.493839908519,38.0255611038277));
#76018=CARTESIAN_POINT('',(121.7,11.4546820508529,38.3229945622399));
#76019=CARTESIAN_POINT('Origin',(103.5,-4.76420601603188,36.1877374401441));
#76020=CARTESIAN_POINT('',(103.5,-3.47532769624592,36.3574214900301));
#76021=CARTESIAN_POINT('',(104.3,13.9120893337143,38.646518368618));
#76022=CARTESIAN_POINT('Origin',(113.,-3.63848543652099,37.5967275667474));
#76023=CARTESIAN_POINT('',(113.,-3.69284665060532,38.0096419822012));
#76024=CARTESIAN_POINT('Origin',(121.7,0.,0.));
#76025=CARTESIAN_POINT('Origin',(121.912132034356,-1.66533453693773E-15,
0.));
#76026=CARTESIAN_POINT('Origin',(121.7,20.9439362252507,33.7550468596361));
#76027=CARTESIAN_POINT('',(121.7,20.9830940829167,34.0524803180483));
#76028=CARTESIAN_POINT('Origin',(103.5,4.76420601603189,36.1877374401441));
#76029=CARTESIAN_POINT('',(104.3,23.440501365778,33.7289565116701));
#76030=CARTESIAN_POINT('Origin',(121.7,0.,0.));
#76031=CARTESIAN_POINT('Origin',(121.912132034356,-2.22044604925031E-15,
0.));
#76032=CARTESIAN_POINT('Origin',(113.,17.6975980727788,33.8531390339859));
#76033=CARTESIAN_POINT('',(121.811388243054,17.9574056939141,33.7031390339859));
#76034=CARTESIAN_POINT('Ctrl Pts',(121.5,17.8365844450781,34.1190013824203));
#76035=CARTESIAN_POINT('Ctrl Pts',(121.5,17.855011884237,34.1093679652233));
#76036=CARTESIAN_POINT('Ctrl Pts',(121.502178291748,17.8725760029409,34.0977083654644));
#76037=CARTESIAN_POINT('Ctrl Pts',(121.510716614322,17.9046379808983,34.0712384527427));
#76038=CARTESIAN_POINT('Ctrl Pts',(121.517077828304,17.9191348789048,34.0564273571332));
#76039=CARTESIAN_POINT('Ctrl Pts',(121.541159186122,17.9568722946504,34.0093301194435));
#76040=CARTESIAN_POINT('Ctrl Pts',(121.56412779323,17.9741868669924,33.974188110278));
#76041=CARTESIAN_POINT('Ctrl Pts',(121.617288389766,17.9964236620831,33.9022439184069));
#76042=CARTESIAN_POINT('Ctrl Pts',(121.652509215907,18.0001315869917,33.8603825931677));
#76043=CARTESIAN_POINT('Ctrl Pts',(121.726559498935,17.9915521676854,33.7810678206517));
#76044=CARTESIAN_POINT('Ctrl Pts',(121.765406035132,17.9791818914014,33.7436393143099));
#76045=CARTESIAN_POINT('Ctrl Pts',(121.804557793905,17.9607714280132,33.7090862384284));
#76046=CARTESIAN_POINT('Ctrl Pts',(121.807962616873,17.9591199407196,33.7061082067124));
#76047=CARTESIAN_POINT('Ctrl Pts',(121.811388687965,17.9574059162404,33.703139419067));
#76048=CARTESIAN_POINT('',(113.,17.9574056939141,33.7031390339859));
#76049=CARTESIAN_POINT('Origin',(113.,17.7491669750802,33.3424589928626));
#76050=CARTESIAN_POINT('',(121.912131484566,17.9070049542699,33.615842392183));
#76051=CARTESIAN_POINT('',(121.75,17.9881175591364,33.7563335449461));
#76052=CARTESIAN_POINT('Ctrl Pts',(122.,17.8008767547585,33.4320229585134));
#76053=CARTESIAN_POINT('Ctrl Pts',(122.,17.8194031463069,33.4641116099562));
#76054=CARTESIAN_POINT('Ctrl Pts',(121.991329280155,17.8412080035414,33.5018787305382));
#76055=CARTESIAN_POINT('Ctrl Pts',(121.962987211232,17.8754315750386,33.5611556951878));
#76056=CARTESIAN_POINT('Ctrl Pts',(121.938311286558,17.8939077309391,33.593157335936));
#76057=CARTESIAN_POINT('Ctrl Pts',(121.912131759621,17.9070050917174,33.6158426302491));
#76058=CARTESIAN_POINT('',(121.7,17.1241669750802,32.259927238132));
#76059=CARTESIAN_POINT('Origin',(121.7,16.9741669750802,32.0001196169967));
#76060=CARTESIAN_POINT('',(103.5,17.1241669750802,32.259927238132));
#76061=CARTESIAN_POINT('Ctrl Pts',(121.375735931288,11.1339148195199,36.529521496889));
#76062=CARTESIAN_POINT('Ctrl Pts',(121.483824361121,11.1059149038863,36.4250243891369));
#76063=CARTESIAN_POINT('Ctrl Pts',(121.591912387511,11.0779148839258,36.3205268920315));
#76064=CARTESIAN_POINT('Ctrl Pts',(121.699999999996,11.0499147569342,36.2160289954803));
#76065=CARTESIAN_POINT('Ctrl Pts',(121.432344074477,11.1485532278086,36.5841527803644));
#76066=CARTESIAN_POINT('Ctrl Pts',(121.540435642307,11.1205539109214,36.4796584662696));
#76067=CARTESIAN_POINT('Ctrl Pts',(121.648526737397,11.0925548930909,36.3751635810634));
#76068=CARTESIAN_POINT('Ctrl Pts',(121.756617543136,11.0645553747475,36.2706685250137));
#76069=CARTESIAN_POINT('Ctrl Pts',(121.544996634179,11.2430954833527,36.6753444250016));
#76070=CARTESIAN_POINT('Ctrl Pts',(121.653094183835,11.2151049763392,36.5708533597438));
#76071=CARTESIAN_POINT('Ctrl Pts',(121.761191535808,11.1871143689483,36.4663621029995));
#76072=CARTESIAN_POINT('Ctrl Pts',(121.869288428606,11.1591238127642,36.3618703486633));
#76073=CARTESIAN_POINT('Ctrl Pts',(121.589544531169,11.410303769972,36.6766200040331));
#76074=CARTESIAN_POINT('Ctrl Pts',(121.697637909657,11.3823253036304,36.5721211654519));
#76075=CARTESIAN_POINT('Ctrl Pts',(121.805730586268,11.354346778571,36.4676216100719));
#76076=CARTESIAN_POINT('Ctrl Pts',(121.913823234175,11.3263684692944,36.3631219450038));
#76077=CARTESIAN_POINT('Ctrl Pts',(121.587867965644,11.4871305554741,36.6543001437251));
#76078=CARTESIAN_POINT('Ctrl Pts',(121.695956395477,11.4591546511876,36.5497955110311));
#76079=CARTESIAN_POINT('Ctrl Pts',(121.804044421867,11.4311788451333,36.4452904208128));
#76080=CARTESIAN_POINT('Ctrl Pts',(121.912132034352,11.4032031398191,36.3407848610988));
#76081=CARTESIAN_POINT('',(121.699999999996,11.0499147569342,36.2160289954803));
#76082=CARTESIAN_POINT('Origin',(121.699999999996,11.3396925048209,36.1383832819495));
#76083=CARTESIAN_POINT('',(121.375735931288,11.1339148195199,36.529521496889));
#76084=CARTESIAN_POINT('Origin',(121.375735931288,11.4236925674066,36.4518757833583));
#76085=CARTESIAN_POINT('Ctrl Pts',(121.375735931288,11.1339148195199,36.529521496889));
#76086=CARTESIAN_POINT('Ctrl Pts',(121.483824361121,11.1059149038863,36.4250243891369));
#76087=CARTESIAN_POINT('Ctrl Pts',(121.591912387511,11.0779148839258,36.3205268920315));
#76088=CARTESIAN_POINT('Ctrl Pts',(121.699999999996,11.0499147569342,36.2160289954803));
#76089=CARTESIAN_POINT('Origin',(121.375735931288,0.,0.));
#76090=CARTESIAN_POINT('',(121.375735931288,11.5134074305014,36.7381470591438));
#76091=CARTESIAN_POINT('Origin',(121.375735931288,0.,0.));
#76092=CARTESIAN_POINT('Origin',(121.375735931288,11.4236925674066,36.4518757833582));
#76093=CARTESIAN_POINT('Origin',(121.375735931288,11.4236925674066,36.4518757833583));
#76094=CARTESIAN_POINT('Origin',(121.375735931288,11.4236925674066,36.4518757833583));
#76095=CARTESIAN_POINT('Origin',(121.7,7.53598121715098,21.9427394990421));
#76096=CARTESIAN_POINT('Origin',(121.7,11.3396925048198,36.1383832819455));
#76097=CARTESIAN_POINT('',(121.7,10.7025987204178,34.9198279009177));
#76098=CARTESIAN_POINT('',(121.7,7.24620346926425,22.0203852125729));
#76099=CARTESIAN_POINT('Origin',(121.7,10.9147307547738,34.5524044395002));
#76100=CARTESIAN_POINT('Origin',(121.7,24.7639590139329,30.8415149116643));
#76101=CARTESIAN_POINT('',(121.7,24.8416047274636,31.131292659551));
#76102=CARTESIAN_POINT('Origin',(121.7,11.3396925048197,36.1383832819456));
#76103=CARTESIAN_POINT('Origin',(113.,13.2452561795175,35.3739408143757));
#76104=CARTESIAN_POINT('',(104.3,12.7669018890611,34.2190913987366));
#76105=CARTESIAN_POINT('',(103.5,12.7669018890611,34.2190913987366));
#76106=CARTESIAN_POINT('Origin',(104.3,12.6520968593516,33.9419275389832));
#76107=CARTESIAN_POINT('',(104.087868515434,13.3660601387852,35.6655873712282));
#76108=CARTESIAN_POINT('Ctrl Pts',(104.087868240379,13.366060243983,35.6655876251981));
#76109=CARTESIAN_POINT('Ctrl Pts',(104.061688713442,13.3560359580278,35.6413868580921));
#76110=CARTESIAN_POINT('Ctrl Pts',(104.037012788768,13.341894920514,35.6072473735402));
#76111=CARTESIAN_POINT('Ctrl Pts',(104.008670719845,13.3157013328973,35.5440104590688));
#76112=CARTESIAN_POINT('Ctrl Pts',(104.,13.2990126176798,35.5037203364521));
#76113=CARTESIAN_POINT('Ctrl Pts',(104.,13.2848331314657,35.4694880285264));
#76114=CARTESIAN_POINT('',(104.25,13.428141038862,35.8154639221579));
#76115=CARTESIAN_POINT('Origin',(113.,11.026122526796,36.127235183779));
#76116=CARTESIAN_POINT('',(104.188611756946,11.1339148195199,36.529521496889));
#76117=CARTESIAN_POINT('',(113.,11.1339148195199,36.529521496889));
#76118=CARTESIAN_POINT('',(104.087868515434,11.1078254769055,36.4321547447161));
#76119=CARTESIAN_POINT('',(104.25,11.1498124507802,36.5888522644724));
#76120=CARTESIAN_POINT('Ctrl Pts',(104.,11.0528894783935,36.2271308071048));
#76121=CARTESIAN_POINT('Ctrl Pts',(104.,11.062479444333,36.2629210472339));
#76122=CARTESIAN_POINT('Ctrl Pts',(104.008670719845,11.0737664689891,36.3050447967167));
#76123=CARTESIAN_POINT('Ctrl Pts',(104.037012788768,11.0914818931789,36.3711596598708));
#76124=CARTESIAN_POINT('Ctrl Pts',(104.061688713442,11.1010458552336,36.4068528521804));
#76125=CARTESIAN_POINT('Ctrl Pts',(104.087868240379,11.1078255480536,36.4321550102444));
#76126=CARTESIAN_POINT('',(104.3,10.7025987204178,34.9198279009177));
#76127=CARTESIAN_POINT('Origin',(104.3,10.624953006887,34.630050153031));
#76128=CARTESIAN_POINT('',(103.5,10.7025987204178,34.9198279009177));
#76129=CARTESIAN_POINT('Origin',(121.7,0.,0.));
#76130=CARTESIAN_POINT('Origin',(121.912132034356,-4.44089209850063E-15,
2.22044604925031E-15));
#76131=CARTESIAN_POINT('Origin',(121.7,30.475,24.2054100357751));
#76132=CARTESIAN_POINT('',(121.7,30.625,24.4652176569104));
#76133=CARTESIAN_POINT('Origin',(103.5,18.25,31.609927238132));
#76134=CARTESIAN_POINT('',(104.3,32.5,23.3826859021798));
#76135=CARTESIAN_POINT('Origin',(121.7,0.,0.));
#76136=CARTESIAN_POINT('Origin',(121.912132034356,-2.22044604925031E-15,
2.22044604925031E-15));
#76137=CARTESIAN_POINT('Origin',(121.7,32.4224208522115,20.7505028516579));
#76138=CARTESIAN_POINT('',(121.7,32.6050492809141,20.9885088537453));
#76139=CARTESIAN_POINT('Origin',(103.5,22.2197921588183,28.9573969206301));
#76140=CARTESIAN_POINT('',(104.3,23.2511515011969,28.1660070629187));
#76141=CARTESIAN_POINT('',(103.5,23.2511515011969,28.1660070629187));
#76142=CARTESIAN_POINT('',(104.3,34.1785730872922,19.7811015708839));
#76143=CARTESIAN_POINT('Origin',(113.,24.0121032874578,29.1576987382828));
#76144=CARTESIAN_POINT('',(104.188611756946,24.2656386875623,29.4881125046124));
#76145=CARTESIAN_POINT('',(113.,24.2656386875623,29.4881125046124));
#76146=CARTESIAN_POINT('',(104.087868515434,24.2042746349845,29.4081413143126));
#76147=CARTESIAN_POINT('',(104.25,24.3030310854828,29.5368432263338));
#76148=CARTESIAN_POINT('Ctrl Pts',(104.,24.0750611261991,29.2397469911496));
#76149=CARTESIAN_POINT('Ctrl Pts',(104.,24.0976174313858,29.2691429403866));
#76150=CARTESIAN_POINT('Ctrl Pts',(104.008670719845,24.1241653434847,29.3037408530298));
#76151=CARTESIAN_POINT('Ctrl Pts',(104.037012788768,24.1658333240656,29.3580436225578));
#76152=CARTESIAN_POINT('Ctrl Pts',(104.061688713442,24.1883284662027,29.3873598625566));
#76153=CARTESIAN_POINT('Ctrl Pts',(104.087868240379,24.20427480233,29.4081415324016));
#76154=CARTESIAN_POINT('Origin',(104.3,23.0685230724943,27.9280010608314));
#76155=CARTESIAN_POINT('Origin',(121.7,0.,0.));
#76156=CARTESIAN_POINT('',(121.912131484566,27.8357364161622,25.9972587850772));
#76157=CARTESIAN_POINT('Ctrl Pts',(121.912131759621,27.8357366105424,25.9972589794574));
#76158=CARTESIAN_POINT('Ctrl Pts',(121.938311286558,27.8172141452984,25.9787365142134));
#76159=CARTESIAN_POINT('Ctrl Pts',(121.962987211232,27.7910849150435,25.9526072839584));
#76160=CARTESIAN_POINT('Ctrl Pts',(121.991329280155,27.7426854760792,25.9042078449942));
#76161=CARTESIAN_POINT('Ctrl Pts',(122.,27.7118487512525,25.8733711201675));
#76162=CARTESIAN_POINT('Ctrl Pts',(122.,27.6856484770629,25.8471708459779));
#76163=CARTESIAN_POINT('Origin',(121.912132034356,2.22044604925031E-15,
-2.22044604925031E-15));
#76164=CARTESIAN_POINT('Origin',(113.,32.2531390339859,20.468879364889));
#76165=CARTESIAN_POINT('',(121.811388243054,32.4031390339859,20.2090717437536));
#76166=CARTESIAN_POINT('Ctrl Pts',(121.5,32.5064359373941,20.6296297263933));
#76167=CARTESIAN_POINT('Ctrl Pts',(121.5,32.5175778592339,20.612073222796));
#76168=CARTESIAN_POINT('Ctrl Pts',(121.502178291748,32.5269590323472,20.5931936538549));
#76169=CARTESIAN_POINT('Ctrl Pts',(121.510716614322,32.5414905633929,20.5542390480232));
#76170=CARTESIAN_POINT('Ctrl Pts',(121.517077828304,32.546639697538,20.5341638139643));
#76171=CARTESIAN_POINT('Ctrl Pts',(121.541159186122,32.555772639402,20.4745077018041));
#76172=CARTESIAN_POINT('Ctrl Pts',(121.56412779323,32.553196494323,20.4354165429558));
#76173=CARTESIAN_POINT('Ctrl Pts',(121.617288389766,32.5364820278348,20.3619926475953));
#76174=CARTESIAN_POINT('Ctrl Pts',(121.652509215907,32.5187625223814,20.3238857140478));
#76175=CARTESIAN_POINT('Ctrl Pts',(121.726559498935,32.4716751410544,20.2594868158067));
#76176=CARTESIAN_POINT('Ctrl Pts',(121.765406035132,32.4422479143698,20.233257916631));
#76177=CARTESIAN_POINT('Ctrl Pts',(121.804557793905,32.4090274474393,20.2125393068328));
#76178=CARTESIAN_POINT('Ctrl Pts',(121.807962616873,32.4061082016311,20.2107859993603));
#76179=CARTESIAN_POINT('Ctrl Pts',(121.811388687965,32.4031394190667,20.2090719660805));
#76180=CARTESIAN_POINT('',(113.,32.4031390339859,20.2090717437536));
#76181=CARTESIAN_POINT('Origin',(113.,32.0424589928626,20.0008330249198));
#76182=CARTESIAN_POINT('',(121.912131484566,32.315842392183,20.1586710041094));
#76183=CARTESIAN_POINT('',(121.75,32.4563335449461,20.2397836089759));
#76184=CARTESIAN_POINT('Ctrl Pts',(122.,32.1320229585134,20.052542804598));
#76185=CARTESIAN_POINT('Ctrl Pts',(122.,32.1641116099562,20.0710691961464));
#76186=CARTESIAN_POINT('Ctrl Pts',(121.991329280155,32.2018787305382,20.0928740533809));
#76187=CARTESIAN_POINT('Ctrl Pts',(121.962987211232,32.2611556951879,20.1270976248782));
#76188=CARTESIAN_POINT('Ctrl Pts',(121.938311286558,32.293157335936,20.1455737807786));
#76189=CARTESIAN_POINT('Ctrl Pts',(121.912131759621,32.3158426302492,20.158671141557));
#76190=CARTESIAN_POINT('',(121.7,30.959927238132,19.3758330249198));
#76191=CARTESIAN_POINT('Origin',(121.7,30.7001196169967,19.2258330249198));
#76192=CARTESIAN_POINT('',(103.5,30.959927238132,19.3758330249198));
#76193=CARTESIAN_POINT('Origin',(121.7,34.8341337964469,14.0682756632309));
#76194=CARTESIAN_POINT('',(121.7,35.0721397985343,14.2509040919335));
#76195=CARTESIAN_POINT('Origin',(103.5,28.9573969206301,22.2197921588183));
#76196=CARTESIAN_POINT('',(104.3,35.9986159921561,13.0434968090721));
#76197=CARTESIAN_POINT('Origin',(121.7,0.,0.));
#76198=CARTESIAN_POINT('Origin',(121.912132034356,4.44089209850063E-15,
-4.44089209850063E-15));
#76199=CARTESIAN_POINT('Origin',(121.7,35.4751196169967,10.9552904187784));
#76200=CARTESIAN_POINT('',(121.7,35.734927238132,11.1052904187784));
#76201=CARTESIAN_POINT('Origin',(103.5,31.609927238132,18.25));
#76202=CARTESIAN_POINT('',(104.3,32.259927238132,17.1241669750802));
#76203=CARTESIAN_POINT('',(103.5,32.259927238132,17.1241669750802));
#76204=CARTESIAN_POINT('',(104.3,36.359927238132,10.0227586640478));
#76205=CARTESIAN_POINT('Origin',(113.,33.3424589928626,17.7491669750802));
#76206=CARTESIAN_POINT('',(104.188611756946,33.7031390339859,17.9574056939141));
#76207=CARTESIAN_POINT('',(113.,33.7031390339859,17.9574056939141));
#76208=CARTESIAN_POINT('',(104.087868515434,33.615842392183,17.9070049542699));
#76209=CARTESIAN_POINT('',(104.25,33.7563335449461,17.9881175591364));
#76210=CARTESIAN_POINT('Ctrl Pts',(104.,33.4320229585134,17.8008767547584));
#76211=CARTESIAN_POINT('Ctrl Pts',(104.,33.4641116099561,17.8194031463068));
#76212=CARTESIAN_POINT('Ctrl Pts',(104.008670719845,33.5018787305382,17.8412080035414));
#76213=CARTESIAN_POINT('Ctrl Pts',(104.037012788768,33.5611556951878,17.8754315750386));
#76214=CARTESIAN_POINT('Ctrl Pts',(104.061688713442,33.593157335936,17.8939077309391));
#76215=CARTESIAN_POINT('Ctrl Pts',(104.087868240379,33.6158426302491,17.9070050917174));
#76216=CARTESIAN_POINT('Origin',(104.3,32.0001196169967,16.9741669750802));
#76217=CARTESIAN_POINT('Origin',(104.3,37.875,-1.6));
#76218=CARTESIAN_POINT('',(104.3,37.8419261182179,-1.3));
#76219=CARTESIAN_POINT('Origin',(104.3,37.8419261182179,-1.6));
#76220=CARTESIAN_POINT('',(104.3,36.5,-1.3));
#76221=CARTESIAN_POINT('Origin',(104.3,36.2,-1.6));
#76222=CARTESIAN_POINT('',(104.3,37.875,-1.3));
#76223=CARTESIAN_POINT('Ctrl Pts',(104.300000000006,37.8419261182243,-1.3));
#76224=CARTESIAN_POINT('Ctrl Pts',(104.408087612492,37.9501103014279,-1.3));
#76225=CARTESIAN_POINT('Ctrl Pts',(104.516175638884,38.0582940710949,-1.3));
#76226=CARTESIAN_POINT('Ctrl Pts',(104.624264068718,38.1664774376737,-1.3));
#76227=CARTESIAN_POINT('Ctrl Pts',(104.243382456866,37.8984931216591,-1.3));
#76228=CARTESIAN_POINT('Ctrl Pts',(104.351473262606,38.0066744036192,-1.30000014726686));
#76229=CARTESIAN_POINT('Ctrl Pts',(104.459564357698,38.1148553910149,-1.29999985529285));
#76230=CARTESIAN_POINT('Ctrl Pts',(104.567655925529,38.223035904161,-1.3));
#76231=CARTESIAN_POINT('Ctrl Pts',(104.130707929307,38.0110670701893,-1.36773633088588));
#76232=CARTESIAN_POINT('Ctrl Pts',(104.238804822106,38.1192428433615,-1.36772867591791));
#76233=CARTESIAN_POINT('Ctrl Pts',(104.346902176736,38.2274181465522,-1.36772120153623));
#76234=CARTESIAN_POINT('Ctrl Pts',(104.454999726393,38.3355932413996,-1.36771367741973));
#76235=CARTESIAN_POINT('Ctrl Pts',(104.086176765827,38.0555584828822,-1.5289633238052));
#76236=CARTESIAN_POINT('Ctrl Pts',(104.194269413736,38.1637387275019,-1.52894179178494));
#76237=CARTESIAN_POINT('Ctrl Pts',(104.302362090347,38.2719189220196,-1.52892049658419));
#76238=CARTESIAN_POINT('Ctrl Pts',(104.410455468836,38.3800984089656,-1.52889933018762));
#76239=CARTESIAN_POINT('Ctrl Pts',(104.08786796565,38.0538687927104,-1.60896117914607));
#76240=CARTESIAN_POINT('Ctrl Pts',(104.195955578136,38.1620540571656,-1.60893560624471));
#76241=CARTESIAN_POINT('Ctrl Pts',(104.304043604528,38.2702388941964,-1.60891025216514));
#76242=CARTESIAN_POINT('Ctrl Pts',(104.412132034362,38.3784233147169,-1.60888511138664));
#76243=CARTESIAN_POINT('',(104.624264068718,38.1664774376737,-1.3));
#76244=CARTESIAN_POINT('',(104.412132034362,38.378423314714,-1.60888511138651));
#76245=CARTESIAN_POINT('Origin',(104.624264068718,38.1664774376737,-1.6));
#76246=CARTESIAN_POINT('',(104.08786796565,38.0538687927072,-1.60896117914593));
#76247=CARTESIAN_POINT('Ctrl Pts',(104.412132034362,38.3784233147169,-1.60888511138664));
#76248=CARTESIAN_POINT('Ctrl Pts',(104.304043604528,38.2702388941964,-1.60891025216514));
#76249=CARTESIAN_POINT('Ctrl Pts',(104.195955578136,38.1620540571656,-1.60893560624471));
#76250=CARTESIAN_POINT('Ctrl Pts',(104.08786796565,38.0538687927104,-1.60896117914607));
#76251=CARTESIAN_POINT('Origin',(104.300000000006,37.8419261182243,-1.6));
#76252=CARTESIAN_POINT('Ctrl Pts',(104.300000000006,37.8419261182243,-1.3));
#76253=CARTESIAN_POINT('Ctrl Pts',(104.408087612492,37.9501103014279,-1.3));
#76254=CARTESIAN_POINT('Ctrl Pts',(104.516175638884,38.0582940710949,-1.3));
#76255=CARTESIAN_POINT('Ctrl Pts',(104.624264068718,38.1664774376737,-1.3));
#76256=CARTESIAN_POINT('Origin',(104.3,37.8419261182179,-1.6));
#76257=CARTESIAN_POINT('Origin',(104.3,37.8419261182179,-1.6));
#76258=CARTESIAN_POINT('Origin',(113.,38.1664774376677,-1.6));
#76259=CARTESIAN_POINT('',(121.375735931288,38.4662141714714,-1.61256544502618));
#76260=CARTESIAN_POINT('',(104.624264068712,38.4662141714714,-1.61256544502618));
#76261=CARTESIAN_POINT('',(113.,38.4662141714714,-1.61256544502618));
#76262=CARTESIAN_POINT('Origin',(104.624264068712,38.1664774376677,-1.6));
#76263=CARTESIAN_POINT('',(121.811388243054,38.1664774376677,-1.3));
#76264=CARTESIAN_POINT('',(113.,38.1664774376677,-1.3));
#76265=CARTESIAN_POINT('',(121.587867965644,38.386744539812,-1.39632770509237));
#76266=CARTESIAN_POINT('Ctrl Pts',(121.811388687965,38.1664778823209,-1.30000000000033));
#76267=CARTESIAN_POINT('Ctrl Pts',(121.807962616872,38.1699059400815,-1.30000000508132));
#76268=CARTESIAN_POINT('Ctrl Pts',(121.804557793907,38.1733107348444,-1.30005879098899));
#76269=CARTESIAN_POINT('Ctrl Pts',(121.765406035132,38.2124398080324,-1.30139139994017));
#76270=CARTESIAN_POINT('Ctrl Pts',(121.726559498935,38.2510389834921,-1.30939267959732));
#76271=CARTESIAN_POINT('Ctrl Pts',(121.652509215907,38.3240173010395,-1.34162007078635));
#76272=CARTESIAN_POINT('Ctrl Pts',(121.617288389766,38.3584163096784,-1.36576189057207));
#76273=CARTESIAN_POINT('Ctrl Pts',(121.588030796123,38.3865877651743,-1.39615825493878));
#76274=CARTESIAN_POINT('Ctrl Pts',(121.587949375966,38.3866661590711,-1.39624293804697));
#76275=CARTESIAN_POINT('Ctrl Pts',(121.587867965644,38.386744539812,-1.39632770509232));
#76276=CARTESIAN_POINT('Ctrl Pts',(121.587867965644,38.386744539812,-1.39632770509233));
#76277=CARTESIAN_POINT('Ctrl Pts',(121.558616909181,38.4149070554612,-1.42678484563743));
#76278=CARTESIAN_POINT('Ctrl Pts',(121.523684543772,38.436448254986,-1.46272037967019));
#76279=CARTESIAN_POINT('Ctrl Pts',(121.45044439244,38.4622264673224,-1.53733192330205));
#76280=CARTESIAN_POINT('Ctrl Pts',(121.414182867144,38.4675247911798,-1.57398889128641));
#76281=CARTESIAN_POINT('Ctrl Pts',(121.377368866524,38.4662794783954,-1.61092740818357));
#76282=CARTESIAN_POINT('Ctrl Pts',(121.376552397245,38.4662485030193,-1.61174649862233));
#76283=CARTESIAN_POINT('Ctrl Pts',(121.375735931288,38.4662141714714,-1.61256544502618));
#76284=CARTESIAN_POINT('Origin',(121.375735931288,0.,0.));
#76285=CARTESIAN_POINT('Origin',(121.587867965644,0.,-3.46944695195361E-15));
#76286=CARTESIAN_POINT('',(121.375735931288,38.3476124040547,-3.42207874082301));
#76287=CARTESIAN_POINT('Origin',(121.375735931288,38.0487998398672,-3.39541319219322));
#76288=CARTESIAN_POINT('Origin',(121.375735931288,0.,0.));
#76289=CARTESIAN_POINT('Origin',(104.624264068712,38.1664774376677,-1.59999999999975));
#76290=CARTESIAN_POINT('Origin',(104.624264068712,38.1664774376677,-1.59999999999975));
#76291=CARTESIAN_POINT('Origin',(121.375735931288,38.0487998398672,-3.39541319219322));
#76292=CARTESIAN_POINT('Origin',(121.375735931288,38.0487998398672,-3.39541319219322));
#76293=CARTESIAN_POINT('Origin',(104.3,0.,0.));
#76294=CARTESIAN_POINT('',(104.087867965649,37.938324246066,-3.37183029953928));
#76295=CARTESIAN_POINT('Origin',(104.087867965644,0.,-3.33066907387547E-15));
#76296=CARTESIAN_POINT('Origin',(104.3,37.7270251019466,-3.35305074428545));
#76297=CARTESIAN_POINT('Origin',(104.25,0.,0.));
#76298=CARTESIAN_POINT('',(104.412132034356,38.2600922303079,-3.4142685824534));
#76299=CARTESIAN_POINT('Origin',(104.412132034356,0.,-3.46944695195361E-15));
#76300=CARTESIAN_POINT('Ctrl Pts',(104.087867965649,37.9383242460686,-3.37183029953951));
#76301=CARTESIAN_POINT('Ctrl Pts',(104.195955578133,38.0455806326541,-3.3859766642846));
#76302=CARTESIAN_POINT('Ctrl Pts',(104.304043604524,38.1528366240337,-3.40012275628987));
#76303=CARTESIAN_POINT('Ctrl Pts',(104.412132034356,38.2600922303079,-3.4142685824534));
#76304=CARTESIAN_POINT('Origin',(104.624264068712,0.,0.));
#76305=CARTESIAN_POINT('',(104.624264068712,38.3476124040547,-3.42207874082301));
#76306=CARTESIAN_POINT('Origin',(104.624264068712,0.,0.));
#76307=CARTESIAN_POINT('Origin',(104.624264068712,38.0487998398672,-3.39541319219322));
#76308=CARTESIAN_POINT('Origin',(113.,0.,0.));
#76309=CARTESIAN_POINT('',(113.,38.3476124040547,-3.42207874082301));
#76310=CARTESIAN_POINT('Origin',(113.,38.0487998398672,-3.39541319219322));
#76311=CARTESIAN_POINT('Origin',(104.624264068712,38.0487998398672,-3.39541319219322));
#76312=CARTESIAN_POINT('Origin',(104.3,37.5986590157289,3.33615102842932));
#76313=CARTESIAN_POINT('',(104.3,37.6878672442806,3.65048420269755));
#76314=CARTESIAN_POINT('Origin',(104.3,37.7270251019467,3.35305074428541));
#76315=CARTESIAN_POINT('',(104.3,36.3574214900301,3.47532769624593));
#76316=CARTESIAN_POINT('Origin',(104.3,36.099145889284,3.13873638016777));
#76317=CARTESIAN_POINT('',(104.3,37.5595011580629,3.63358448684147));
#76318=CARTESIAN_POINT('Origin',(121.7,35.375,1.6));
#76319=CARTESIAN_POINT('',(121.7,37.841926118218,1.3));
#76320=CARTESIAN_POINT('Origin',(121.7,37.841926118218,1.6));
#76321=CARTESIAN_POINT('',(121.7,36.5,1.3));
#76322=CARTESIAN_POINT('Origin',(121.7,36.2,1.6));
#76323=CARTESIAN_POINT('',(121.7,35.375,1.3));
#76324=CARTESIAN_POINT('Ctrl Pts',(121.699999999994,37.8419261182243,1.3));
#76325=CARTESIAN_POINT('Ctrl Pts',(121.591912387508,37.950110301428,1.3));
#76326=CARTESIAN_POINT('Ctrl Pts',(121.483824361116,38.0582940710949,1.3));
#76327=CARTESIAN_POINT('Ctrl Pts',(121.375735931282,38.1664774376736,1.3));
#76328=CARTESIAN_POINT('Ctrl Pts',(121.756617543134,37.8984931216591,1.3));
#76329=CARTESIAN_POINT('Ctrl Pts',(121.648526737394,38.0066744036192,1.30000014726686));
#76330=CARTESIAN_POINT('Ctrl Pts',(121.540435642302,38.1148553910149,1.29999985529285));
#76331=CARTESIAN_POINT('Ctrl Pts',(121.432344074471,38.223035904161,1.3));
#76332=CARTESIAN_POINT('Ctrl Pts',(121.869289488093,38.0110644898949,1.36773987413571));
#76333=CARTESIAN_POINT('Ctrl Pts',(121.761192595294,38.1192402630671,1.36773221916774));
#76334=CARTESIAN_POINT('Ctrl Pts',(121.653095242547,38.2274155681001,1.36772474312819));
#76335=CARTESIAN_POINT('Ctrl Pts',(121.54499769289,38.3355906629474,1.3677172190117));
#76336=CARTESIAN_POINT('Ctrl Pts',(121.913823234173,38.0555584828822,1.5289633238052));
#76337=CARTESIAN_POINT('Ctrl Pts',(121.805730586264,38.1637387275019,1.52894179178494));
#76338=CARTESIAN_POINT('Ctrl Pts',(121.697637909653,38.2719189220196,1.52892049658419));
#76339=CARTESIAN_POINT('Ctrl Pts',(121.589544531164,38.3800984089656,1.52889933018762));
#76340=CARTESIAN_POINT('Ctrl Pts',(121.91213203435,38.0538687927104,1.60896117914607));
#76341=CARTESIAN_POINT('Ctrl Pts',(121.804044421864,38.1620540571656,1.60893560624471));
#76342=CARTESIAN_POINT('Ctrl Pts',(121.695956395472,38.2702388941964,1.60891025216514));
#76343=CARTESIAN_POINT('Ctrl Pts',(121.587867965638,38.3784233147169,1.60888511138664));
#76344=CARTESIAN_POINT('',(121.375735931282,38.1664774376736,1.3));
#76345=CARTESIAN_POINT('',(121.587867965638,38.378423314714,1.60888511138651));
#76346=CARTESIAN_POINT('Origin',(121.375735931282,38.1664774376736,1.6));
#76347=CARTESIAN_POINT('',(121.91213203435,38.0538687927072,1.60896117914593));
#76348=CARTESIAN_POINT('Ctrl Pts',(121.587867965638,38.3784233147169,1.60888511138664));
#76349=CARTESIAN_POINT('Ctrl Pts',(121.695956395472,38.2702388941964,1.60891025216514));
#76350=CARTESIAN_POINT('Ctrl Pts',(121.804044421864,38.1620540571656,1.60893560624471));
#76351=CARTESIAN_POINT('Ctrl Pts',(121.91213203435,38.0538687927104,1.60896117914607));
#76352=CARTESIAN_POINT('Origin',(121.699999999994,37.8419261182243,1.6));
#76353=CARTESIAN_POINT('Ctrl Pts',(121.699999999994,37.8419261182243,1.3));
#76354=CARTESIAN_POINT('Ctrl Pts',(121.591912387508,37.950110301428,1.3));
#76355=CARTESIAN_POINT('Ctrl Pts',(121.483824361116,38.0582940710949,1.3));
#76356=CARTESIAN_POINT('Ctrl Pts',(121.375735931282,38.1664774376736,1.3));
#76357=CARTESIAN_POINT('Origin',(121.7,37.841926118218,1.6));
#76358=CARTESIAN_POINT('Origin',(121.7,37.841926118218,1.6));
#76359=CARTESIAN_POINT('Origin',(104.624264068712,0.,0.));
#76360=CARTESIAN_POINT('',(104.412132034356,38.386744539812,1.39632770509237));
#76361=CARTESIAN_POINT('',(104.412132034356,38.2600922303079,3.41426858245337));
#76362=CARTESIAN_POINT('Origin',(104.412132034356,0.,-3.33066907387547E-15));
#76363=CARTESIAN_POINT('',(104.624264068712,38.3476124040547,3.42207874082297));
#76364=CARTESIAN_POINT('Origin',(104.624264068712,38.0487998398672,3.39541319219318));
#76365=CARTESIAN_POINT('',(104.624264068712,38.4662141714714,1.61256544502618));
#76366=CARTESIAN_POINT('Origin',(104.624264068712,0.,0.));
#76367=CARTESIAN_POINT('Ctrl Pts',(104.624264068712,38.4662141714714,1.61256544502617));
#76368=CARTESIAN_POINT('Ctrl Pts',(104.623447602755,38.4662485030193,1.61174649862234));
#76369=CARTESIAN_POINT('Ctrl Pts',(104.622631133476,38.4662794783954,1.61092740818295));
#76370=CARTESIAN_POINT('Ctrl Pts',(104.585817132852,38.4675247911796,1.57398889128992));
#76371=CARTESIAN_POINT('Ctrl Pts',(104.54955560756,38.4622264673224,1.53733192330198));
#76372=CARTESIAN_POINT('Ctrl Pts',(104.476315456228,38.436448254986,1.46272037967007));
#76373=CARTESIAN_POINT('Ctrl Pts',(104.441383090818,38.4149070554612,1.42678484563735));
#76374=CARTESIAN_POINT('Ctrl Pts',(104.412132034356,38.386744539812,1.39632770509233));
#76375=CARTESIAN_POINT('Origin',(113.,38.1664774376677,1.6));
#76376=CARTESIAN_POINT('',(121.375735931288,38.4662141714714,1.61256544502618));
#76377=CARTESIAN_POINT('',(113.,38.4662141714714,1.61256544502618));
#76378=CARTESIAN_POINT('Origin',(121.375735931288,38.1664774376677,1.6));
#76379=CARTESIAN_POINT('',(104.188611756946,38.1664774376677,1.3));
#76380=CARTESIAN_POINT('',(113.,38.1664774376677,1.3));
#76381=CARTESIAN_POINT('Ctrl Pts',(104.188611312035,38.1664778823209,1.30000000000033));
#76382=CARTESIAN_POINT('Ctrl Pts',(104.192037383128,38.1699059400815,1.30000000508132));
#76383=CARTESIAN_POINT('Ctrl Pts',(104.195442206093,38.1733107348444,1.30005879098899));
#76384=CARTESIAN_POINT('Ctrl Pts',(104.234593964868,38.2124398080324,1.30139139994017));
#76385=CARTESIAN_POINT('Ctrl Pts',(104.273440501065,38.2510389834921,1.30939267959732));
#76386=CARTESIAN_POINT('Ctrl Pts',(104.347490784093,38.3240173010395,1.34162007078635));
#76387=CARTESIAN_POINT('Ctrl Pts',(104.382711610234,38.3584163096784,1.36576189057207));
#76388=CARTESIAN_POINT('Ctrl Pts',(104.411969203877,38.3865877651743,1.39615825493878));
#76389=CARTESIAN_POINT('Ctrl Pts',(104.412050624034,38.3866661590711,1.39624293804698));
#76390=CARTESIAN_POINT('Ctrl Pts',(104.412132034356,38.386744539812,1.39632770509232));
#76391=CARTESIAN_POINT('Origin',(121.375735931288,38.1664774376677,1.59999999999975));
#76392=CARTESIAN_POINT('Origin',(121.375735931288,38.1664774376677,1.59999999999975));
#76393=CARTESIAN_POINT('Ctrl Pts',(104.300000000005,37.6878672442858,3.65048420269823));
#76394=CARTESIAN_POINT('Ctrl Pts',(104.408087612489,37.7951258968034,3.66460507219003));
#76395=CARTESIAN_POINT('Ctrl Pts',(104.51617563888,37.9023841393222,3.67872588770446));
#76396=CARTESIAN_POINT('Ctrl Pts',(104.624264068712,38.0096419822012,3.69284665060533));
#76397=CARTESIAN_POINT('Ctrl Pts',(104.243382456865,37.7439503091645,3.65786767826187));
#76398=CARTESIAN_POINT('Ctrl Pts',(104.351473262604,37.8512061044813,3.67198802305842));
#76399=CARTESIAN_POINT('Ctrl Pts',(104.459564357694,37.9584615504213,3.68610876488972));
#76400=CARTESIAN_POINT('Ctrl Pts',(104.567655925523,38.0657165831673,3.70022901187373));
#76401=CARTESIAN_POINT('Ctrl Pts',(104.13070824621,37.8644022801433,3.60540421753157));
#76402=CARTESIAN_POINT('Ctrl Pts',(104.238805139007,37.9716515954047,3.61953157877266));
#76403=CARTESIAN_POINT('Ctrl Pts',(104.346902493405,38.078900468474,3.63365869985868));
#76404=CARTESIAN_POINT('Ctrl Pts',(104.45500004306,38.1861491282933,3.64778584282858));
#76405=CARTESIAN_POINT('Ctrl Pts',(104.086176765826,37.9295576652633,3.45136431096226));
#76406=CARTESIAN_POINT('Ctrl Pts',(104.194269413733,38.0368096023995,3.46550601417654));
#76407=CARTESIAN_POINT('Ctrl Pts',(104.302362090343,38.1440615207735,3.4796474760577));
#76408=CARTESIAN_POINT('Ctrl Pts',(104.410455468831,38.2513127544414,3.49378871787999));
#76409=CARTESIAN_POINT('Ctrl Pts',(104.087867965649,37.9383242460686,3.37183029953947));
#76410=CARTESIAN_POINT('Ctrl Pts',(104.195955578133,38.0455806326541,3.38597666428457));
#76411=CARTESIAN_POINT('Ctrl Pts',(104.304043604524,38.1528366240338,3.40012275628984));
#76412=CARTESIAN_POINT('Ctrl Pts',(104.412132034356,38.2600922303079,3.41426858245337));
#76413=CARTESIAN_POINT('',(104.624264068712,38.0096419822012,3.69284665060533));
#76414=CARTESIAN_POINT('Origin',(104.624264068712,38.0487998398672,3.39541319219319));
#76415=CARTESIAN_POINT('',(104.087867965649,37.938324246066,3.37183029953924));
#76416=CARTESIAN_POINT('Ctrl Pts',(104.412132034356,38.2600922303079,3.41426858245337));
#76417=CARTESIAN_POINT('Ctrl Pts',(104.304043604524,38.1528366240338,3.40012275628984));
#76418=CARTESIAN_POINT('Ctrl Pts',(104.195955578133,38.0455806326541,3.38597666428457));
#76419=CARTESIAN_POINT('Ctrl Pts',(104.087867965649,37.9383242460686,3.37183029953947));
#76420=CARTESIAN_POINT('Origin',(104.300000000005,37.7270251019518,3.35305074428609));
#76421=CARTESIAN_POINT('Ctrl Pts',(104.300000000005,37.6878672442858,3.65048420269823));
#76422=CARTESIAN_POINT('Ctrl Pts',(104.408087612489,37.7951258968034,3.66460507219003));
#76423=CARTESIAN_POINT('Ctrl Pts',(104.51617563888,37.9023841393222,3.67872588770446));
#76424=CARTESIAN_POINT('Ctrl Pts',(104.624264068712,38.0096419822012,3.69284665060533));
#76425=CARTESIAN_POINT('Origin',(104.624264068712,38.0487998398672,3.39541319219318));
#76426=CARTESIAN_POINT('Origin',(104.624264068712,38.0487998398672,3.39541319219318));
#76427=CARTESIAN_POINT('Origin',(104.3,37.7270251019466,3.35305074428563));
#76428=CARTESIAN_POINT('Origin',(104.3,37.7270251019466,3.35305074428563));
#76429=CARTESIAN_POINT('Origin',(113.,0.,0.));
#76430=CARTESIAN_POINT('',(121.375735931288,38.3476124040547,3.42207874082297));
#76431=CARTESIAN_POINT('',(113.,38.3476124040547,3.42207874082297));
#76432=CARTESIAN_POINT('Origin',(121.375735931288,0.,0.));
#76433=CARTESIAN_POINT('Origin',(113.,38.0487998398672,3.39541319219318));
#76434=CARTESIAN_POINT('',(121.375735931288,38.0096419822012,3.69284665060533));
#76435=CARTESIAN_POINT('',(113.,38.0096419822012,3.69284665060533));
#76436=CARTESIAN_POINT('Origin',(121.375735931288,38.0487998398672,3.39541319219318));
#76437=CARTESIAN_POINT('Origin',(113.,37.5967275667474,3.63848543652099));
#76438=CARTESIAN_POINT('',(121.7,36.3574214900301,3.47532769624593));
#76439=CARTESIAN_POINT('',(103.5,36.3574214900301,3.47532769624593));
#76440=CARTESIAN_POINT('Origin',(121.7,36.059988031618,3.43616983857991));
#76441=CARTESIAN_POINT('Ctrl Pts',(121.375735931288,38.0096419822012,3.69284665060533));
#76442=CARTESIAN_POINT('Ctrl Pts',(121.583825474459,37.8031514673445,3.66566165859633));
#76443=CARTESIAN_POINT('Ctrl Pts',(121.79191352265,37.5966594715985,3.63847647162457));
#76444=CARTESIAN_POINT('Ctrl Pts',(122.,37.3901659198623,3.6112910798028));
#76445=CARTESIAN_POINT('Origin',(104.3,0.,0.));
#76446=CARTESIAN_POINT('',(104.087868515434,38.0656759583793,1.3));
#76447=CARTESIAN_POINT('Origin',(104.087867965644,0.,-3.19189119579733E-15));
#76448=CARTESIAN_POINT('Ctrl Pts',(104.087868240379,38.0656762332744,1.3));
#76449=CARTESIAN_POINT('Ctrl Pts',(104.061688713442,38.0394815117177,1.3));
#76450=CARTESIAN_POINT('Ctrl Pts',(104.037012788768,38.0025291999168,1.3));
#76451=CARTESIAN_POINT('Ctrl Pts',(104.008670719845,37.9340820569223,1.3));
#76452=CARTESIAN_POINT('Ctrl Pts',(104.,37.8904723424532,1.3));
#76453=CARTESIAN_POINT('Ctrl Pts',(104.,37.8534195593564,1.3));
#76454=CARTESIAN_POINT('Origin',(104.25,0.,0.));
#76455=CARTESIAN_POINT('',(104.25,38.2279011681123,1.3));
#76456=CARTESIAN_POINT('Origin',(121.7,0.,0.));
#76457=CARTESIAN_POINT('',(121.912132034356,37.9383242460634,3.37183029953879));
#76458=CARTESIAN_POINT('Origin',(121.912132034356,0.,-3.33066907387547E-15));
#76459=CARTESIAN_POINT('Ctrl Pts',(121.912132034356,37.9383242460634,3.37183029953879));
#76460=CARTESIAN_POINT('Ctrl Pts',(121.912644761788,37.9377510612696,3.37248779876803));
#76461=CARTESIAN_POINT('Ctrl Pts',(121.913155626955,37.9371760091143,3.37314512705079));
#76462=CARTESIAN_POINT('Ctrl Pts',(121.940508718519,37.9061731758521,3.40845981939242));
#76463=CARTESIAN_POINT('Ctrl Pts',(121.962380614807,37.8703180968885,3.44290792623732));
#76464=CARTESIAN_POINT('Ctrl Pts',(121.991615201992,37.7932167467436,3.50530359020698));
#76465=CARTESIAN_POINT('Ctrl Pts',(122.,37.7517487643871,3.53404539859927));
#76466=CARTESIAN_POINT('Ctrl Pts',(122.,37.7082051239441,3.55846015394631));
#76467=CARTESIAN_POINT('Ctrl Pts',(121.375735931288,38.0096419822012,3.69284665060533));
#76468=CARTESIAN_POINT('Ctrl Pts',(121.583825474459,37.8031514673445,3.66566165859633));
#76469=CARTESIAN_POINT('Ctrl Pts',(121.79191352265,37.5966594715985,3.63847647162457));
#76470=CARTESIAN_POINT('Ctrl Pts',(122.,37.3901659198623,3.6112910798028));
#76471=CARTESIAN_POINT('Ctrl Pts',(121.432344074477,38.0657165831673,3.70022901187372));
#76472=CARTESIAN_POINT('Ctrl Pts',(121.640439658852,37.8592314783189,3.67304501309689));
#76473=CARTESIAN_POINT('Ctrl Pts',(121.848533661831,37.6527449072731,3.64585996863109));
#76474=CARTESIAN_POINT('Ctrl Pts',(122.056626387712,37.4462569420324,3.61867560296373));
#76475=CARTESIAN_POINT('Ctrl Pts',(121.544997455782,38.186147098729,3.64778211360282));
#76476=CARTESIAN_POINT('Ctrl Pts',(121.753104556242,37.9796742629036,3.62058483882079));
#76477=CARTESIAN_POINT('Ctrl Pts',(121.961210702025,37.773200439291,3.59338741284848));
#76478=CARTESIAN_POINT('Ctrl Pts',(122.169315338809,37.5667251447857,3.56618931926667));
#76479=CARTESIAN_POINT('Ctrl Pts',(121.589544531169,38.2513127544414,3.49378871787999));
#76480=CARTESIAN_POINT('Ctrl Pts',(121.797643601385,38.0448349634972,3.46656430028762));
#76481=CARTESIAN_POINT('Ctrl Pts',(122.005740672884,37.8383552309336,3.43933905383214));
#76482=CARTESIAN_POINT('Ctrl Pts',(122.21383700281,37.6318748010017,3.41211290549725));
#76483=CARTESIAN_POINT('Ctrl Pts',(121.587867965644,38.2600922303079,3.41426858245337));
#76484=CARTESIAN_POINT('Ctrl Pts',(121.795957508814,38.0536060213154,3.38703533918487));
#76485=CARTESIAN_POINT('Ctrl Pts',(122.004045557006,37.8471183852976,3.35980111082395));
#76486=CARTESIAN_POINT('Ctrl Pts',(122.212132034356,37.640629249017,3.33256584736066));
#76487=CARTESIAN_POINT('',(121.587867965644,38.2600922303079,3.41426858245337));
#76488=CARTESIAN_POINT('Ctrl Pts',(121.912132034434,37.9383242461395,3.37183029959021));
#76489=CARTESIAN_POINT('Ctrl Pts',(121.804044421952,38.0455806327306,3.38597666433816));
#76490=CARTESIAN_POINT('Ctrl Pts',(121.695956395478,38.152836624032,3.40012275628961));
#76491=CARTESIAN_POINT('Ctrl Pts',(121.587867965644,38.2600922303079,3.41426858245337));
#76492=CARTESIAN_POINT('Origin',(121.375735931288,38.0487998398672,3.39541319219318));
#76493=CARTESIAN_POINT('Origin',(121.375735931288,0.,0.));
#76494=CARTESIAN_POINT('Origin',(121.375735931288,38.0487998398672,3.39541319219318));
#76495=CARTESIAN_POINT('Origin',(121.587867965644,0.,-3.33066907387547E-15));
#76496=CARTESIAN_POINT('Origin',(121.375735931288,38.0487998398672,3.39541319219318));
#76497=CARTESIAN_POINT('Origin',(121.75,0.,0.));
#76498=CARTESIAN_POINT('Origin',(113.,37.75,1.3));
#76499=CARTESIAN_POINT('',(104.3,36.5,1.3));
#76500=CARTESIAN_POINT('',(103.5,36.5,1.3));
#76501=CARTESIAN_POINT('Origin',(104.3,36.2,1.3));
#76502=CARTESIAN_POINT('Ctrl Pts',(104.624264068712,38.0096419822012,-3.69284665060536));
#76503=CARTESIAN_POINT('Ctrl Pts',(104.516175638879,37.9023841393221,-3.6787258877045));
#76504=CARTESIAN_POINT('Ctrl Pts',(104.408087612489,37.7951258968034,-3.66460507219007));
#76505=CARTESIAN_POINT('Ctrl Pts',(104.300000000005,37.6878672442858,-3.65048420269827));
#76506=CARTESIAN_POINT('Ctrl Pts',(104.567655925523,38.0657165831672,-3.70022901187376));
#76507=CARTESIAN_POINT('Ctrl Pts',(104.459564357694,37.9584615504212,-3.68610876488976));
#76508=CARTESIAN_POINT('Ctrl Pts',(104.351473262604,37.8512061044813,-3.67198802305846));
#76509=CARTESIAN_POINT('Ctrl Pts',(104.243382456865,37.7439503091645,-3.65786767826191));
#76510=CARTESIAN_POINT('Ctrl Pts',(104.45500004306,38.1861491282932,-3.64778584282862));
#76511=CARTESIAN_POINT('Ctrl Pts',(104.346902493405,38.078900468474,-3.63365869985872));
#76512=CARTESIAN_POINT('Ctrl Pts',(104.238805139007,37.9716515954047,-3.6195315787727));
#76513=CARTESIAN_POINT('Ctrl Pts',(104.13070824621,37.8644022801433,-3.60540421753161));
#76514=CARTESIAN_POINT('Ctrl Pts',(104.410455468831,38.2513127544414,-3.49378871788002));
#76515=CARTESIAN_POINT('Ctrl Pts',(104.302362090343,38.1440615207734,-3.47964747605774));
#76516=CARTESIAN_POINT('Ctrl Pts',(104.194269413733,38.0368096023995,-3.46550601417657));
#76517=CARTESIAN_POINT('Ctrl Pts',(104.086176765826,37.9295576652633,-3.4513643109623));
#76518=CARTESIAN_POINT('Ctrl Pts',(104.412132034356,38.2600922303079,-3.4142685824534));
#76519=CARTESIAN_POINT('Ctrl Pts',(104.304043604524,38.1528366240337,-3.40012275628987));
#76520=CARTESIAN_POINT('Ctrl Pts',(104.195955578133,38.0455806326541,-3.3859766642846));
#76521=CARTESIAN_POINT('Ctrl Pts',(104.087867965649,37.9383242460686,-3.37183029953951));
#76522=CARTESIAN_POINT('Origin',(104.300000000005,37.7270251019518,-3.35305074428613));
#76523=CARTESIAN_POINT('Origin',(104.624264068712,38.0487998398672,-3.39541319219322));
#76524=CARTESIAN_POINT('Origin',(104.3,37.5986590157289,-3.33615102842936));
#76525=CARTESIAN_POINT('Origin',(104.3,37.7270251019467,-3.35305074428545));
#76526=CARTESIAN_POINT('Origin',(104.3,36.099145889284,-3.13873638016781));
#76527=CARTESIAN_POINT('Origin',(104.3,37.7270251019466,-3.35305074428545));
#76528=CARTESIAN_POINT('Origin',(104.624264068712,38.0487998398672,-3.39541319219322));
#76529=CARTESIAN_POINT('Origin',(121.7,0.,0.));
#76530=CARTESIAN_POINT('',(121.7,-4.04133443718627E-15,33.));
#76531=CARTESIAN_POINT('',(121.7,-33.,-4.04133443718627E-15));
#76532=CARTESIAN_POINT('Origin',(121.7,0.,0.));
#76533=CARTESIAN_POINT('Origin',(121.7,0.,0.));
#76534=CARTESIAN_POINT('Origin',(121.7,-4.07807384116069E-15,33.3));
#76535=CARTESIAN_POINT('Origin',(113.,0.,0.));
#76536=CARTESIAN_POINT('',(104.3,-33.,-4.04133443718627E-15));
#76537=CARTESIAN_POINT('',(113.,-33.,-4.04133443718627E-15));
#76538=CARTESIAN_POINT('',(104.3,-4.04133443718627E-15,33.));
#76539=CARTESIAN_POINT('Origin',(104.3,0.,0.));
#76540=CARTESIAN_POINT('Origin',(104.3,0.,0.));
#76541=CARTESIAN_POINT('Origin',(121.7,0.,0.));
#76542=CARTESIAN_POINT('',(121.912132034356,37.173644453082,8.29492882695057));
#76543=CARTESIAN_POINT('Origin',(121.912132034356,0.,5.55111512312578E-16));
#76544=CARTESIAN_POINT('Ctrl Pts',(121.912132034356,37.173644453082,8.29492882695057));
#76545=CARTESIAN_POINT('Ctrl Pts',(121.912644761788,37.1729903510924,8.29550588555455));
#76546=CARTESIAN_POINT('Ctrl Pts',(121.913155626955,37.172334420031,8.2960825309338));
#76547=CARTESIAN_POINT('Ctrl Pts',(121.940508718518,37.1369873279846,8.32704841941382));
#76548=CARTESIAN_POINT('Ctrl Pts',(121.962380614807,37.0969426139758,8.35652179100008));
#76549=CARTESIAN_POINT('Ctrl Pts',(121.991615201992,37.0123566081405,8.40831990576543));
#76550=CARTESIAN_POINT('Ctrl Pts',(122.,36.9674918313147,8.4314031661665));
#76551=CARTESIAN_POINT('Ctrl Pts',(122.,36.9211339477026,8.44992546431459));
#76552=CARTESIAN_POINT('Ctrl Pts',(121.375735931288,37.2024510141556,8.62250767116828));
#76553=CARTESIAN_POINT('Ctrl Pts',(121.583825474459,37.0012754077709,8.56860282990067));
#76554=CARTESIAN_POINT('Ctrl Pts',(121.79191352265,36.800098358614,8.51469760204339));
#76555=CARTESIAN_POINT('Ctrl Pts',(122.,36.5989197935167,8.46079196799113));
#76556=CARTESIAN_POINT('Ctrl Pts',(121.432344074477,37.257082297631,8.63714607945699));
#76557=CARTESIAN_POINT('Ctrl Pts',(121.640439658852,37.0559119253285,8.58324292907209));
#76558=CARTESIAN_POINT('Ctrl Pts',(121.848533661831,36.8547402358619,8.52933855056707));
#76559=CARTESIAN_POINT('Ctrl Pts',(122.056626387712,36.653567075527,8.47543466307433));
#76560=CARTESIAN_POINT('Ctrl Pts',(121.544996913559,37.3833278766636,8.60086634932545));
#76561=CARTESIAN_POINT('Ctrl Pts',(121.753104014018,37.1821714012872,8.54695163794227));
#76562=CARTESIAN_POINT('Ctrl Pts',(121.961210159033,36.981013965758,8.49303664688276));
#76563=CARTESIAN_POINT('Ctrl Pts',(122.169314795818,36.779855159611,8.43912080278263));
#76564=CARTESIAN_POINT('Ctrl Pts',(121.589544531169,37.4680365334272,8.45669707232343));
#76565=CARTESIAN_POINT('Ctrl Pts',(121.797643601385,37.2668786881714,8.40275480356762));
#76566=CARTESIAN_POINT('Ctrl Pts',(122.005740672884,37.0657190260955,8.34881145960757));
#76567=CARTESIAN_POINT('Ctrl Pts',(122.21383700281,36.8645587903363,8.29486713045898));
#76568=CARTESIAN_POINT('Ctrl Pts',(121.587867965644,37.4871203601426,8.37900319423351));
#76569=CARTESIAN_POINT('Ctrl Pts',(121.795957508814,37.285955320838,8.32505107653065));
#76570=CARTESIAN_POINT('Ctrl Pts',(122.004045557006,37.084788995297,8.27109779589882));
#76571=CARTESIAN_POINT('Ctrl Pts',(122.212132034356,36.8836213174361,8.21714329319647));
#76572=CARTESIAN_POINT('',(121.587867965644,37.4871203601426,8.37900319423351));
#76573=CARTESIAN_POINT('Ctrl Pts',(121.912132034434,37.1736444531508,8.2949288270115));
#76574=CARTESIAN_POINT('Ctrl Pts',(121.804044421952,37.2781367753618,8.32295393538098));
#76575=CARTESIAN_POINT('Ctrl Pts',(121.695956395478,37.3826287412719,8.35097872169212));
#76576=CARTESIAN_POINT('Ctrl Pts',(121.587867965644,37.4871203601426,8.37900319423351));
#76577=CARTESIAN_POINT('Origin',(121.375735931288,37.2800967276863,8.33272992328156));
#76578=CARTESIAN_POINT('Origin',(121.375735931288,0.,0.));
#76579=CARTESIAN_POINT('Origin',(121.375735931288,37.2800967276863,8.33272992328155));
#76580=CARTESIAN_POINT('Origin',(121.587867965644,0.,1.11022302462516E-15));
#76581=CARTESIAN_POINT('Origin',(121.375735931288,37.2800967276863,8.33272992328155));
#76582=CARTESIAN_POINT('Origin',(121.7,0.,0.));
#76583=CARTESIAN_POINT('',(121.912132034356,35.7729132970271,13.0760988223445));
#76584=CARTESIAN_POINT('Origin',(121.912132034356,2.22044604925031E-15,
-3.33066907387547E-15));
#76585=CARTESIAN_POINT('Ctrl Pts',(121.912132034356,35.7729132970271,13.0760988223445));
#76586=CARTESIAN_POINT('Ctrl Pts',(121.912644761788,35.7721894697088,13.0765855666898));
#76587=CARTESIAN_POINT('Ctrl Pts',(121.913155626953,35.7714638829032,13.0770716626056));
#76588=CARTESIAN_POINT('Ctrl Pts',(121.940508718538,35.732377330599,13.1031589122749));
#76589=CARTESIAN_POINT('Ctrl Pts',(121.962380614808,35.68882815772,13.1271532510543));
#76590=CARTESIAN_POINT('Ctrl Pts',(121.991615201992,35.5982047862083,13.1674675365095));
#76591=CARTESIAN_POINT('Ctrl Pts',(122.,35.5507108636835,13.184497287934));
#76592=CARTESIAN_POINT('Ctrl Pts',(122.,35.5023319331436,13.1968102072265));
#76593=CARTESIAN_POINT('Ctrl Pts',(121.375735931288,35.7587157947897,13.4046351948668));
#76594=CARTESIAN_POINT('Ctrl Pts',(121.583825474459,35.5662972672787,13.3249328311199));
#76595=CARTESIAN_POINT('Ctrl Pts',(121.79191352265,35.3738773597987,13.2452298957711));
#76596=CARTESIAN_POINT('Ctrl Pts',(122.,35.1814560023665,13.1655263598324));
#76597=CARTESIAN_POINT('Ctrl Pts',(121.432344074477,35.8109690043675,13.4262791829515));
#76598=CARTESIAN_POINT('Ctrl Pts',(121.640439658852,35.618555445456,13.3465791788063));
#76599=CARTESIAN_POINT('Ctrl Pts',(121.848533661831,35.4261407409506,13.2668777851234));
#76600=CARTESIAN_POINT('Ctrl Pts',(122.056626387712,35.2337245140706,13.1871766862653));
#76601=CARTESIAN_POINT('Ctrl Pts',(121.544996490687,35.9408698217382,13.4067874878274));
#76602=CARTESIAN_POINT('Ctrl Pts',(121.753103591146,35.7484715498757,13.3270778355028));
#76603=CARTESIAN_POINT('Ctrl Pts',(121.961209735563,35.5560723622402,13.2473677798582));
#76604=CARTESIAN_POINT('Ctrl Pts',(122.169314372347,35.3636719273963,13.1676567002806));
#76605=CARTESIAN_POINT('Ctrl Pts',(121.589544531169,36.0436718192237,13.2749089952201));
#76606=CARTESIAN_POINT('Ctrl Pts',(121.797643601385,35.8512757861603,13.1951718424748));
#76607=CARTESIAN_POINT('Ctrl Pts',(122.005740672884,35.6588780921622,13.1154333865813));
#76608=CARTESIAN_POINT('Ctrl Pts',(122.21383700281,35.4664799579815,13.0356938790469));
#76609=CARTESIAN_POINT('Ctrl Pts',(121.587867965644,36.072733467222,13.2003707382617));
#76610=CARTESIAN_POINT('Ctrl Pts',(121.795957508814,35.8803315872014,13.1206228818168));
#76611=CARTESIAN_POINT('Ctrl Pts',(122.004045557006,35.6879285837409,13.0408737045043));
#76612=CARTESIAN_POINT('Ctrl Pts',(122.212132034356,35.495524399042,12.9611231390632));
#76613=CARTESIAN_POINT('',(121.587867965644,36.072733467222,13.2003707382617));
#76614=CARTESIAN_POINT('Ctrl Pts',(121.912132034434,35.7729132970873,13.0760988224139));
#76615=CARTESIAN_POINT('Ctrl Pts',(121.804044421952,35.8728536623143,13.1175231570306));
#76616=CARTESIAN_POINT('Ctrl Pts',(121.695956395478,35.9727937163258,13.1589471258378));
#76617=CARTESIAN_POINT('Ctrl Pts',(121.587867965644,36.072733467222,13.2003707382617));
#76618=CARTESIAN_POINT('Origin',(121.375735931288,35.8735208244992,13.1274713351134));
#76619=CARTESIAN_POINT('Origin',(121.375735931288,0.,0.));
#76620=CARTESIAN_POINT('Origin',(121.375735931288,35.8735208244992,13.1274713351134));
#76621=CARTESIAN_POINT('Origin',(121.587867965644,-2.22044604925031E-15,
2.22044604925031E-15));
#76622=CARTESIAN_POINT('Origin',(121.375735931288,35.8735208244992,13.1274713351134));
#76623=CARTESIAN_POINT('Origin',(121.75,0.,0.));
#76624=CARTESIAN_POINT('Origin',(121.7,36.0718053304427,5.24424943271125));
#76625=CARTESIAN_POINT('',(121.7,36.3615830783294,5.32189514624201));
#76626=CARTESIAN_POINT('Origin',(103.5,35.256292659551,9.44689514624201));
#76627=CARTESIAN_POINT('',(104.3,34.9198279009177,10.7025987204178));
#76628=CARTESIAN_POINT('',(104.3,36.5290513235988,4.69689514624201));
#76629=CARTESIAN_POINT('',(103.5,34.9198279009177,10.7025987204178));
#76630=CARTESIAN_POINT('Origin',(121.75,0.,0.));
#76631=CARTESIAN_POINT('Origin',(121.7,36.1714159148471,2.58979103627007));
#76632=CARTESIAN_POINT('',(121.7,36.4688493732593,2.62894889393609));
#76633=CARTESIAN_POINT('Origin',(103.5,36.1877374401441,4.76420601603188));
#76634=CARTESIAN_POINT('',(104.3,36.018053390258,6.05308433581784));
#76635=CARTESIAN_POINT('',(104.3,36.5114420903979,2.30542508755794));
#76636=CARTESIAN_POINT('',(103.5,36.018053390258,6.05308433581784));
#76637=CARTESIAN_POINT('Origin',(104.3,0.,0.));
#76638=CARTESIAN_POINT('Origin',(104.3,-4.07807384116069E-15,33.3));
#76639=CARTESIAN_POINT('Origin',(121.7,36.2,0.));
#76640=CARTESIAN_POINT('',(121.7,36.5,-1.3));
#76641=CARTESIAN_POINT('Origin',(121.7,36.2,-1.3));
#76642=CARTESIAN_POINT('',(121.7,36.5,0.));
#76643=CARTESIAN_POINT('Origin',(103.5,36.5,0.));
#76644=CARTESIAN_POINT('',(103.5,36.5,-1.3));
#76645=CARTESIAN_POINT('',(104.3,36.5,0.));
#76646=CARTESIAN_POINT('Origin',(104.3,36.2,0.));
#76647=CARTESIAN_POINT('Origin',(104.3,36.2140086319858,2.26626722989192));
#76648=CARTESIAN_POINT('Origin',(104.3,35.7206199318459,6.01392647815182));
#76649=CARTESIAN_POINT('Origin',(104.3,36.2392735757121,4.61924943271125));
#76650=CARTESIAN_POINT('Origin',(104.3,34.630050153031,10.624953006887));
#76651=CARTESIAN_POINT('Origin',(113.,33.8531390339859,17.6975980727788));
#76652=CARTESIAN_POINT('',(104.5,34.1190013824203,17.8365844450781));
#76653=CARTESIAN_POINT('',(113.,34.1190013824203,17.8365844450781));
#76654=CARTESIAN_POINT('Ctrl Pts',(104.5,34.1190013824203,17.8365844450781));
#76655=CARTESIAN_POINT('Ctrl Pts',(104.5,34.1093679652233,17.8550118842369));
#76656=CARTESIAN_POINT('Ctrl Pts',(104.497821708252,34.0977083654644,17.8725760029409));
#76657=CARTESIAN_POINT('Ctrl Pts',(104.489283385678,34.0712384527427,17.9046379808983));
#76658=CARTESIAN_POINT('Ctrl Pts',(104.482922171696,34.0564273571332,17.9191348789048));
#76659=CARTESIAN_POINT('Ctrl Pts',(104.458840813878,34.0093301194435,17.9568722946504));
#76660=CARTESIAN_POINT('Ctrl Pts',(104.43587220677,33.974188110278,17.9741868669923));
#76661=CARTESIAN_POINT('Ctrl Pts',(104.382711610234,33.9022439184069,17.9964236620831));
#76662=CARTESIAN_POINT('Ctrl Pts',(104.347490784093,33.8603825931677,18.0001315869917));
#76663=CARTESIAN_POINT('Ctrl Pts',(104.273440501065,33.7810678206517,17.9915521676854));
#76664=CARTESIAN_POINT('Ctrl Pts',(104.234593964868,33.7436393143099,17.9791818914014));
#76665=CARTESIAN_POINT('Ctrl Pts',(104.195442206095,33.7090862384284,17.9607714280132));
#76666=CARTESIAN_POINT('Ctrl Pts',(104.192037383127,33.7061082067124,17.9591199407196));
#76667=CARTESIAN_POINT('Ctrl Pts',(104.188611312035,33.703139419067,17.9574059162404));
#76668=CARTESIAN_POINT('Origin',(121.7,35.8608081321196,8.01950930682723));
#76669=CARTESIAN_POINT('',(121.7,36.1379719918729,8.13431433653676));
#76670=CARTESIAN_POINT('Origin',(103.5,33.721602936662,13.9679452813258));
#76671=CARTESIAN_POINT('',(104.3,36.5040885153898,7.25043086005358));
#76672=CARTESIAN_POINT('Origin',(104.3,36.2269246556364,7.13562583034405));
#76673=CARTESIAN_POINT('Origin',(104.3,0.,0.));
#76674=CARTESIAN_POINT('Origin',(104.087867965644,2.22044604925031E-15,
-3.33066907387547E-15));
#76675=CARTESIAN_POINT('Origin',(104.3,36.1001196169967,9.87275866404783));
#76676=CARTESIAN_POINT('Origin',(104.3,35.7606099900688,12.8608683803695));
#76677=CARTESIAN_POINT('Origin',(113.,27.6125198053347,25.7740421742497));
#76678=CARTESIAN_POINT('',(121.7,26.7286363288515,24.8901586977665));
#76679=CARTESIAN_POINT('',(103.5,26.7286363288515,24.8901586977665));
#76680=CARTESIAN_POINT('Origin',(121.7,26.5165042944955,24.6780266634105));
#76681=CARTESIAN_POINT('',(121.75,27.9504469620439,26.1119693309588));
#76682=CARTESIAN_POINT('Origin',(113.,24.5036446896497,29.3054840759098));
#76683=CARTESIAN_POINT('',(104.5,24.6960816898302,29.5356318566107));
#76684=CARTESIAN_POINT('',(113.,24.6960816898302,29.5356318566107));
#76685=CARTESIAN_POINT('Ctrl Pts',(104.5,24.6960816898302,29.5356318566107));
#76686=CARTESIAN_POINT('Ctrl Pts',(104.5,24.6801296971867,29.5489700413278));
#76687=CARTESIAN_POINT('Ctrl Pts',(104.497821708253,24.6626361343801,29.5607352354492));
#76688=CARTESIAN_POINT('Ctrl Pts',(104.489283385678,24.625911536016,29.5802270436011));
#76689=CARTESIAN_POINT('Ctrl Pts',(104.482922171696,24.6066801452406,29.5879524700494));
#76690=CARTESIAN_POINT('Ctrl Pts',(104.458840813878,24.5487264875151,29.6047939634926));
#76691=CARTESIAN_POINT('Ctrl Pts',(104.43587220677,24.509633504542,29.6073422778058));
#76692=CARTESIAN_POINT('Ctrl Pts',(104.382711610234,24.4346560851191,29.6003545473749));
#76693=CARTESIAN_POINT('Ctrl Pts',(104.347490784093,24.3945623020958,29.5877605876801));
#76694=CARTESIAN_POINT('Ctrl Pts',(104.273440501065,24.3245682087703,29.5494817883985));
#76695=CARTESIAN_POINT('Ctrl Pts',(104.234593964868,24.2947226776164,29.5237298740531));
#76696=CARTESIAN_POINT('Ctrl Pts',(104.195442206095,24.2698451773449,29.4934979340675));
#76697=CARTESIAN_POINT('Ctrl Pts',(104.192037383127,24.2677258316214,29.49083251536));
#76698=CARTESIAN_POINT('Ctrl Pts',(104.188611312035,24.2656389582503,29.4881128573793));
#76699=CARTESIAN_POINT('Origin',(121.7,33.847265478953,17.347265478953));
#76700=CARTESIAN_POINT('',(121.7,34.059397513309,17.559397513309));
#76701=CARTESIAN_POINT('Origin',(103.5,25.809397513309,25.809397513309));
#76702=CARTESIAN_POINT('',(104.3,35.309397513309,16.309397513309));
#76703=CARTESIAN_POINT('Origin',(104.3,35.097265478953,16.097265478953));
#76704=CARTESIAN_POINT('Origin',(104.3,0.,0.));
#76705=CARTESIAN_POINT('Origin',(104.087867965644,2.22044604925031E-15,
-2.22044604925031E-15));
#76706=CARTESIAN_POINT('Origin',(104.3,33.9959446585896,19.5430955687966));
#76707=CARTESIAN_POINT('Origin',(104.3,32.35,23.1228782810445));
#76708=CARTESIAN_POINT('Origin',(113.,11.4236925674066,36.4518757833583));
#76709=CARTESIAN_POINT('',(104.5,11.5134074305014,36.7381470591438));
#76710=CARTESIAN_POINT('',(113.,11.5134074305014,36.7381470591438));
#76711=CARTESIAN_POINT('Ctrl Pts',(104.5,11.5134074305014,36.7381470591438));
#76712=CARTESIAN_POINT('Ctrl Pts',(104.5,11.4935654086862,36.7443653717069));
#76713=CARTESIAN_POINT('Ctrl Pts',(104.497821708252,11.4729011191897,36.7485404970926));
#76714=CARTESIAN_POINT('Ctrl Pts',(104.489283385678,11.4315128223748,36.7524946843416));
#76715=CARTESIAN_POINT('Ctrl Pts',(104.482922171696,11.410788941346,36.7522725130859));
#76716=CARTESIAN_POINT('Ctrl Pts',(104.458840813878,11.3508017826223,36.7456541195186));
#76717=CARTESIAN_POINT('Ctrl Pts',(104.43587220677,11.3137093781205,36.7330482180494));
#76718=CARTESIAN_POINT('Ctrl Pts',(104.382711610234,11.2471133635809,36.6978997807109));
#76719=CARTESIAN_POINT('Ctrl Pts',(104.347490784093,11.2148910377878,36.6709212526118));
#76720=CARTESIAN_POINT('Ctrl Pts',(104.273440501065,11.1648735898636,36.6087706735473));
#76721=CARTESIAN_POINT('Ctrl Pts',(104.234593964868,11.1471547454652,36.5735576166579));
#76722=CARTESIAN_POINT('Ctrl Pts',(104.195442206095,11.1357401947051,36.5361067388845));
#76723=CARTESIAN_POINT('Ctrl Pts',(104.192037383127,11.1348021861485,36.5328331745993));
#76724=CARTESIAN_POINT('Ctrl Pts',(104.188611312035,11.1339149346049,36.5295219263909));
#76725=CARTESIAN_POINT('Origin',(121.7,27.9367711964053,27.6108081321196));
#76726=CARTESIAN_POINT('',(121.7,28.0515762261148,27.8879719918729));
#76727=CARTESIAN_POINT('Origin',(103.5,13.9679452813258,33.721602936662));
#76728=CARTESIAN_POINT('',(104.3,30.185459702598,27.0040885153898));
#76729=CARTESIAN_POINT('Origin',(104.3,30.0706546728884,26.7269246556364));
#76730=CARTESIAN_POINT('Origin',(104.3,0.,0.));
#76731=CARTESIAN_POINT('Origin',(104.087867965644,-1.11022302462516E-15,
0.));
#76732=CARTESIAN_POINT('Origin',(104.3,27.0964907686634,30.2165149116643));
#76733=CARTESIAN_POINT('',(104.3,27.1741364821942,30.506292659551));
#76734=CARTESIAN_POINT('Origin',(103.5,9.44689514624202,35.256292659551));
#76735=CARTESIAN_POINT('Origin',(104.3,23.401343508112,33.431523053258));
#76736=CARTESIAN_POINT('Origin',(113.,-3.39541319219318,38.0487998398672));
#76737=CARTESIAN_POINT('Origin',(121.7,16.5,36.2));
#76738=CARTESIAN_POINT('',(121.7,16.5,36.5));
#76739=CARTESIAN_POINT('Origin',(103.5,2.23498040844392E-15,36.5));
#76740=CARTESIAN_POINT('',(104.3,19.,36.5));
#76741=CARTESIAN_POINT('Origin',(104.3,19.,36.2));
#76742=CARTESIAN_POINT('Origin',(104.3,0.,0.));
#76743=CARTESIAN_POINT('Origin',(104.087867965644,-1.94289029309402E-15,
0.));
#76744=CARTESIAN_POINT('Origin',(104.3,13.9512471913803,38.3490849102059));
#76745=CARTESIAN_POINT('Origin',(104.3,8.35799190324092,39.7165149116643));
#76746=CARTESIAN_POINT('Origin',(113.,-17.6975980727787,33.8531390339859));
#76747=CARTESIAN_POINT('',(104.5,-17.8365844450781,34.1190013824203));
#76748=CARTESIAN_POINT('',(113.,-17.8365844450781,34.1190013824203));
#76749=CARTESIAN_POINT('Ctrl Pts',(104.5,-17.8365844450781,34.1190013824203));
#76750=CARTESIAN_POINT('Ctrl Pts',(104.5,-17.8550118842369,34.1093679652233));
#76751=CARTESIAN_POINT('Ctrl Pts',(104.497821708252,-17.8725760029409,34.0977083654644));
#76752=CARTESIAN_POINT('Ctrl Pts',(104.489283385678,-17.9046379808982,34.0712384527427));
#76753=CARTESIAN_POINT('Ctrl Pts',(104.482922171696,-17.9191348789048,34.0564273571332));
#76754=CARTESIAN_POINT('Ctrl Pts',(104.458840813878,-17.9568722946504,34.0093301194435));
#76755=CARTESIAN_POINT('Ctrl Pts',(104.43587220677,-17.9741868669923,33.974188110278));
#76756=CARTESIAN_POINT('Ctrl Pts',(104.382711610234,-17.9964236620831,33.9022439184069));
#76757=CARTESIAN_POINT('Ctrl Pts',(104.347490784093,-18.0001315869917,33.8603825931677));
#76758=CARTESIAN_POINT('Ctrl Pts',(104.273440501065,-17.9915521676854,33.7810678206517));
#76759=CARTESIAN_POINT('Ctrl Pts',(104.234593964868,-17.9791818914014,33.7436393143099));
#76760=CARTESIAN_POINT('Ctrl Pts',(104.195442206095,-17.9607714280132,33.7090862384284));
#76761=CARTESIAN_POINT('Ctrl Pts',(104.192037383127,-17.9591199407196,33.7061082067124));
#76762=CARTESIAN_POINT('Ctrl Pts',(104.188611312035,-17.9574059162404,33.703139419067));
#76763=CARTESIAN_POINT('Origin',(121.7,0.23049069317278,39.2780700216976));
#76764=CARTESIAN_POINT('',(121.7,0.115685663463252,39.555233881451));
#76765=CARTESIAN_POINT('Origin',(103.5,-13.9679452813258,33.721602936662));
#76766=CARTESIAN_POINT('',(104.3,2.24956913994644,40.4391173579342));
#76767=CARTESIAN_POINT('Origin',(104.3,2.36437416965597,40.1619534981808));
#76768=CARTESIAN_POINT('Origin',(104.3,0.,0.));
#76769=CARTESIAN_POINT('Origin',(104.087867965644,-1.11022302462516E-15,
0.));
#76770=CARTESIAN_POINT('Origin',(104.3,-3.84999999999999,39.5773609529488));
#76771=CARTESIAN_POINT('Origin',(104.3,-10.0783828016417,37.8956862682889));
#76772=CARTESIAN_POINT('Origin',(113.,-29.3054840759098,24.5036446896497));
#76773=CARTESIAN_POINT('',(104.5,-29.5356318566107,24.6960816898302));
#76774=CARTESIAN_POINT('',(113.,-29.5356318566107,24.6960816898302));
#76775=CARTESIAN_POINT('Ctrl Pts',(104.5,-29.5356318566107,24.6960816898302));
#76776=CARTESIAN_POINT('Ctrl Pts',(104.5,-29.5489700413278,24.6801296971867));
#76777=CARTESIAN_POINT('Ctrl Pts',(104.497821708252,-29.5607352354492,24.6626361343801));
#76778=CARTESIAN_POINT('Ctrl Pts',(104.489283385678,-29.5802270436011,24.625911536016));
#76779=CARTESIAN_POINT('Ctrl Pts',(104.482922171696,-29.5879524700494,24.6066801452406));
#76780=CARTESIAN_POINT('Ctrl Pts',(104.458840813878,-29.6047939634926,24.5487264875151));
#76781=CARTESIAN_POINT('Ctrl Pts',(104.43587220677,-29.6073422778058,24.509633504542));
#76782=CARTESIAN_POINT('Ctrl Pts',(104.382711610234,-29.6003545473749,24.4346560851191));
#76783=CARTESIAN_POINT('Ctrl Pts',(104.347490784093,-29.5877605876801,24.3945623020958));
#76784=CARTESIAN_POINT('Ctrl Pts',(104.273440501065,-29.5494817883985,24.3245682087704));
#76785=CARTESIAN_POINT('Ctrl Pts',(104.234593964868,-29.5237298740531,24.2947226776164));
#76786=CARTESIAN_POINT('Ctrl Pts',(104.195442206095,-29.4934979340675,24.2698451773449));
#76787=CARTESIAN_POINT('Ctrl Pts',(104.192037383127,-29.49083251536,24.2677258316214));
#76788=CARTESIAN_POINT('Ctrl Pts',(104.188611312035,-29.4881128573793,24.2656389582503));
#76789=CARTESIAN_POINT('Origin',(121.7,-17.347265478953,33.847265478953));
#76790=CARTESIAN_POINT('',(121.7,-17.559397513309,34.059397513309));
#76791=CARTESIAN_POINT('Origin',(103.5,-25.809397513309,25.809397513309));
#76792=CARTESIAN_POINT('',(104.3,-16.309397513309,35.309397513309));
#76793=CARTESIAN_POINT('Origin',(104.3,-16.097265478953,35.097265478953));
#76794=CARTESIAN_POINT('Origin',(104.3,0.,0.));
#76795=CARTESIAN_POINT('Origin',(104.087867965644,0.,-2.22044604925031E-15));
#76796=CARTESIAN_POINT('Origin',(104.3,-21.6781718470166,31.2134590798618));
#76797=CARTESIAN_POINT('Origin',(104.3,-26.6001196169967,26.3272413359522));
#76798=CARTESIAN_POINT('Origin',(113.,-36.4518757833582,11.4236925674066));
#76799=CARTESIAN_POINT('',(104.5,-36.7381470591438,11.5134074305014));
#76800=CARTESIAN_POINT('',(113.,-36.7381470591438,11.5134074305014));
#76801=CARTESIAN_POINT('Ctrl Pts',(104.5,-36.7381470591438,11.5134074305014));
#76802=CARTESIAN_POINT('Ctrl Pts',(104.5,-36.7443653717069,11.4935654086862));
#76803=CARTESIAN_POINT('Ctrl Pts',(104.497821708252,-36.7485404970926,11.4729011191897));
#76804=CARTESIAN_POINT('Ctrl Pts',(104.489283385678,-36.7524946843416,11.4315128223748));
#76805=CARTESIAN_POINT('Ctrl Pts',(104.482922171696,-36.7522725130859,11.410788941346));
#76806=CARTESIAN_POINT('Ctrl Pts',(104.458840813878,-36.7456541195186,11.3508017826223));
#76807=CARTESIAN_POINT('Ctrl Pts',(104.43587220677,-36.7330482180494,11.3137093781205));
#76808=CARTESIAN_POINT('Ctrl Pts',(104.382711610234,-36.6978997807109,11.2471133635809));
#76809=CARTESIAN_POINT('Ctrl Pts',(104.347490784093,-36.6709212526118,11.2148910377878));
#76810=CARTESIAN_POINT('Ctrl Pts',(104.273440501065,-36.6087706735473,11.1648735898636));
#76811=CARTESIAN_POINT('Ctrl Pts',(104.234593964868,-36.5735576166579,11.1471547454652));
#76812=CARTESIAN_POINT('Ctrl Pts',(104.195442206095,-36.5361067388845,11.1357401947051));
#76813=CARTESIAN_POINT('Ctrl Pts',(104.192037383127,-36.5328331745993,11.1348021861485));
#76814=CARTESIAN_POINT('Ctrl Pts',(104.188611312035,-36.5295219263909,11.1339149346049));
#76815=CARTESIAN_POINT('Origin',(121.7,-31.0280700216976,19.6867711964053));
#76816=CARTESIAN_POINT('',(121.7,-31.305233881451,19.8015762261148));
#76817=CARTESIAN_POINT('Origin',(103.5,-33.721602936662,13.9679452813258));
#76818=CARTESIAN_POINT('',(104.3,-30.9391173579342,20.685459702598));
#76819=CARTESIAN_POINT('Origin',(104.3,-30.6619534981808,20.5706546728885));
#76820=CARTESIAN_POINT('Origin',(104.3,0.,0.));
#76821=CARTESIAN_POINT('Origin',(104.087867965644,-2.22044604925031E-15,
-1.11022302462516E-15));
#76822=CARTESIAN_POINT('Origin',(104.3,-33.6937562476164,14.1192494327113));
#76823=CARTESIAN_POINT('Origin',(113.,-37.2573594669753,6.21624207609292));
#76824=CARTESIAN_POINT('',(121.75,-37.7311721243447,6.27862069582413));
#76825=CARTESIAN_POINT('Origin',(104.3,-35.5665993314781,7.18382908683984));
#76826=CARTESIAN_POINT('Origin',(113.,-38.0487998398672,-3.39541319219318));
#76827=CARTESIAN_POINT('Origin',(121.7,-36.2,6.45388863150655E-15));
#76828=CARTESIAN_POINT('',(121.7,-36.5,6.49062803548097E-15));
#76829=CARTESIAN_POINT('Origin',(103.5,-36.5,4.46996081688784E-15));
#76830=CARTESIAN_POINT('',(104.3,-36.5,6.79678973526781E-15));
#76831=CARTESIAN_POINT('Origin',(104.3,-36.2,6.76005033129339E-15));
#76832=CARTESIAN_POINT('Origin',(104.3,0.,0.));
#76833=CARTESIAN_POINT('Origin',(104.087867965644,0.,2.77555756156289E-15));
#76834=CARTESIAN_POINT('Origin',(104.3,-35.5665993314781,-7.1838290868398));
#76835=CARTESIAN_POINT('Origin',(104.3,-33.6937562476164,-14.1192494327112));
#76836=CARTESIAN_POINT('Origin',(113.,-33.8531390339859,-17.6975980727788));
#76837=CARTESIAN_POINT('',(104.5,-34.1190013824203,-17.8365844450781));
#76838=CARTESIAN_POINT('',(113.,-34.1190013824203,-17.8365844450781));
#76839=CARTESIAN_POINT('Ctrl Pts',(104.5,-34.1190013824203,-17.8365844450781));
#76840=CARTESIAN_POINT('Ctrl Pts',(104.5,-34.1093679652233,-17.8550118842369));
#76841=CARTESIAN_POINT('Ctrl Pts',(104.497821708252,-34.0977083654644,-17.8725760029409));
#76842=CARTESIAN_POINT('Ctrl Pts',(104.489283385678,-34.0712384527427,-17.9046379808983));
#76843=CARTESIAN_POINT('Ctrl Pts',(104.482922171696,-34.0564273571332,-17.9191348789048));
#76844=CARTESIAN_POINT('Ctrl Pts',(104.458840813878,-34.0093301194435,-17.9568722946504));
#76845=CARTESIAN_POINT('Ctrl Pts',(104.43587220677,-33.974188110278,-17.9741868669923));
#76846=CARTESIAN_POINT('Ctrl Pts',(104.382711610234,-33.9022439184069,-17.9964236620831));
#76847=CARTESIAN_POINT('Ctrl Pts',(104.347490784093,-33.8603825931677,-18.0001315869917));
#76848=CARTESIAN_POINT('Ctrl Pts',(104.273440501065,-33.7810678206517,-17.9915521676854));
#76849=CARTESIAN_POINT('Ctrl Pts',(104.234593964868,-33.7436393143099,-17.9791818914014));
#76850=CARTESIAN_POINT('Ctrl Pts',(104.195442206095,-33.7090862384284,-17.9607714280132));
#76851=CARTESIAN_POINT('Ctrl Pts',(104.192037383127,-33.7061082067124,-17.9591199407196));
#76852=CARTESIAN_POINT('Ctrl Pts',(104.188611312035,-33.703139419067,-17.9574059162404));
#76853=CARTESIAN_POINT('Origin',(121.7,-31.0280700216976,-19.6867711964052));
#76854=CARTESIAN_POINT('',(121.7,-31.305233881451,-19.8015762261148));
#76855=CARTESIAN_POINT('Origin',(103.5,-33.721602936662,-13.9679452813258));
#76856=CARTESIAN_POINT('',(104.3,-30.9391173579342,-20.6854597025979));
#76857=CARTESIAN_POINT('Origin',(104.3,-30.6619534981808,-20.5706546728884));
#76858=CARTESIAN_POINT('Origin',(104.3,0.,0.));
#76859=CARTESIAN_POINT('Origin',(104.087867965644,2.22044604925031E-15,
-4.44089209850063E-15));
#76860=CARTESIAN_POINT('Origin',(104.3,-26.6001196169967,-26.3272413359522));
#76861=CARTESIAN_POINT('Origin',(104.3,-21.6781718470167,-31.2134590798618));
#76862=CARTESIAN_POINT('Origin',(113.,-27.6125198053347,-25.7740421742496));
#76863=CARTESIAN_POINT('',(121.7,-26.7286363288515,-24.8901586977665));
#76864=CARTESIAN_POINT('',(103.5,-26.7286363288515,-24.8901586977665));
#76865=CARTESIAN_POINT('Origin',(121.7,-26.5165042944955,-24.6780266634105));
#76866=CARTESIAN_POINT('',(121.75,-27.9504469620439,-26.1119693309588));
#76867=CARTESIAN_POINT('Origin',(113.,-24.5036446896497,-29.3054840759098));
#76868=CARTESIAN_POINT('',(104.5,-24.6960816898302,-29.5356318566107));
#76869=CARTESIAN_POINT('',(113.,-24.6960816898302,-29.5356318566107));
#76870=CARTESIAN_POINT('Ctrl Pts',(104.5,-24.6960816898302,-29.5356318566107));
#76871=CARTESIAN_POINT('Ctrl Pts',(104.5,-24.6801296971867,-29.5489700413278));
#76872=CARTESIAN_POINT('Ctrl Pts',(104.497821708252,-24.6626361343801,-29.5607352354492));
#76873=CARTESIAN_POINT('Ctrl Pts',(104.489283385678,-24.625911536016,-29.5802270436011));
#76874=CARTESIAN_POINT('Ctrl Pts',(104.482922171696,-24.6066801452406,-29.5879524700494));
#76875=CARTESIAN_POINT('Ctrl Pts',(104.458840813878,-24.5487264875151,-29.6047939634926));
#76876=CARTESIAN_POINT('Ctrl Pts',(104.43587220677,-24.509633504542,-29.6073422778058));
#76877=CARTESIAN_POINT('Ctrl Pts',(104.382711610234,-24.4346560851191,-29.6003545473748));
#76878=CARTESIAN_POINT('Ctrl Pts',(104.347490784093,-24.3945623020959,-29.5877605876801));
#76879=CARTESIAN_POINT('Ctrl Pts',(104.273440501065,-24.3245682087704,-29.5494817883985));
#76880=CARTESIAN_POINT('Ctrl Pts',(104.234593964868,-24.2947226776164,-29.5237298740531));
#76881=CARTESIAN_POINT('Ctrl Pts',(104.195442206095,-24.2698451773449,-29.4934979340675));
#76882=CARTESIAN_POINT('Ctrl Pts',(104.192037383127,-24.2677258316214,-29.49083251536));
#76883=CARTESIAN_POINT('Ctrl Pts',(104.188611312035,-24.2656389582503,-29.4881128573793));
#76884=CARTESIAN_POINT('Origin',(121.7,-17.347265478953,-33.847265478953));
#76885=CARTESIAN_POINT('',(121.7,-17.559397513309,-34.059397513309));
#76886=CARTESIAN_POINT('Origin',(103.5,-25.809397513309,-25.809397513309));
#76887=CARTESIAN_POINT('',(104.3,-16.309397513309,-35.309397513309));
#76888=CARTESIAN_POINT('Origin',(104.3,-16.097265478953,-35.097265478953));
#76889=CARTESIAN_POINT('Origin',(104.3,0.,0.));
#76890=CARTESIAN_POINT('Origin',(104.087867965644,-2.22044604925031E-15,
2.22044604925031E-15));
#76891=CARTESIAN_POINT('Origin',(104.3,-10.0783828016418,-37.8956862682889));
#76892=CARTESIAN_POINT('Origin',(113.,-20.0008330249198,-32.0424589928625));
#76893=CARTESIAN_POINT('',(121.75,-20.2397836089759,-32.456333544946));
#76894=CARTESIAN_POINT('Origin',(104.3,-3.85000000000002,-39.5773609529488));
#76895=CARTESIAN_POINT('Origin',(113.,-11.4236925674066,-36.4518757833582));
#76896=CARTESIAN_POINT('',(104.5,-11.5134074305014,-36.7381470591438));
#76897=CARTESIAN_POINT('',(113.,-11.5134074305014,-36.7381470591438));
#76898=CARTESIAN_POINT('Ctrl Pts',(104.5,-11.5134074305014,-36.7381470591438));
#76899=CARTESIAN_POINT('Ctrl Pts',(104.5,-11.4935654086862,-36.7443653717069));
#76900=CARTESIAN_POINT('Ctrl Pts',(104.497821708253,-11.4729011191897,-36.7485404970926));
#76901=CARTESIAN_POINT('Ctrl Pts',(104.489283385678,-11.4315128223748,-36.7524946843416));
#76902=CARTESIAN_POINT('Ctrl Pts',(104.482922171696,-11.410788941346,-36.7522725130859));
#76903=CARTESIAN_POINT('Ctrl Pts',(104.458840813878,-11.3508017826223,-36.7456541195186));
#76904=CARTESIAN_POINT('Ctrl Pts',(104.43587220677,-11.3137093781205,-36.7330482180494));
#76905=CARTESIAN_POINT('Ctrl Pts',(104.382711610234,-11.2471133635809,-36.6978997807109));
#76906=CARTESIAN_POINT('Ctrl Pts',(104.347490784093,-11.2148910377879,-36.6709212526118));
#76907=CARTESIAN_POINT('Ctrl Pts',(104.273440501065,-11.1648735898636,-36.6087706735473));
#76908=CARTESIAN_POINT('Ctrl Pts',(104.234593964868,-11.1471547454652,-36.5735576166579));
#76909=CARTESIAN_POINT('Ctrl Pts',(104.195442206095,-11.1357401947051,-36.5361067388845));
#76910=CARTESIAN_POINT('Ctrl Pts',(104.192037383127,-11.1348021861485,-36.5328331745992));
#76911=CARTESIAN_POINT('Ctrl Pts',(104.188611312035,-11.1339149346049,-36.5295219263909));
#76912=CARTESIAN_POINT('Origin',(121.7,0.230490693172739,-39.2780700216976));
#76913=CARTESIAN_POINT('',(121.7,0.11568566346321,-39.555233881451));
#76914=CARTESIAN_POINT('Origin',(103.5,-13.9679452813258,-33.721602936662));
#76915=CARTESIAN_POINT('',(104.3,2.24956913994639,-40.4391173579342));
#76916=CARTESIAN_POINT('Origin',(104.3,2.36437416965592,-40.1619534981808));
#76917=CARTESIAN_POINT('Origin',(104.3,0.,0.));
#76918=CARTESIAN_POINT('Origin',(104.087867965644,-2.22044604925031E-15,
2.22044604925031E-15));
#76919=CARTESIAN_POINT('Origin',(104.3,8.35799190324088,-39.7165149116643));
#76920=CARTESIAN_POINT('Origin',(104.3,13.9512471913802,-38.3490849102059));
#76921=CARTESIAN_POINT('Origin',(113.,3.39541319219317,-38.0487998398672));
#76922=CARTESIAN_POINT('Origin',(121.7,16.5,-36.2));
#76923=CARTESIAN_POINT('',(121.7,16.5,-36.5));
#76924=CARTESIAN_POINT('Origin',(103.5,-6.70494122533176E-15,-36.5));
#76925=CARTESIAN_POINT('',(104.3,19.,-36.5));
#76926=CARTESIAN_POINT('Origin',(104.3,19.,-36.2));
#76927=CARTESIAN_POINT('Origin',(104.3,0.,0.));
#76928=CARTESIAN_POINT('Origin',(104.087867965644,2.4980018054066E-15,0.));
#76929=CARTESIAN_POINT('Origin',(104.3,23.401343508112,-33.431523053258));
#76930=CARTESIAN_POINT('Origin',(104.3,27.0964907686634,-30.2165149116643));
#76931=CARTESIAN_POINT('Origin',(113.,17.6975980727787,-33.8531390339859));
#76932=CARTESIAN_POINT('',(104.5,17.836584445078,-34.1190013824203));
#76933=CARTESIAN_POINT('',(113.,17.836584445078,-34.1190013824203));
#76934=CARTESIAN_POINT('Ctrl Pts',(104.5,17.836584445078,-34.1190013824203));
#76935=CARTESIAN_POINT('Ctrl Pts',(104.5,17.8550118842369,-34.1093679652233));
#76936=CARTESIAN_POINT('Ctrl Pts',(104.497821708252,17.8725760029409,-34.0977083654644));
#76937=CARTESIAN_POINT('Ctrl Pts',(104.489283385678,17.9046379808982,-34.0712384527427));
#76938=CARTESIAN_POINT('Ctrl Pts',(104.482922171696,17.9191348789048,-34.0564273571332));
#76939=CARTESIAN_POINT('Ctrl Pts',(104.458840813878,17.9568722946504,-34.0093301194435));
#76940=CARTESIAN_POINT('Ctrl Pts',(104.43587220677,17.9741868669923,-33.974188110278));
#76941=CARTESIAN_POINT('Ctrl Pts',(104.382711610234,17.9964236620831,-33.9022439184069));
#76942=CARTESIAN_POINT('Ctrl Pts',(104.347490784093,18.0001315869917,-33.8603825931677));
#76943=CARTESIAN_POINT('Ctrl Pts',(104.273440501065,17.9915521676854,-33.7810678206517));
#76944=CARTESIAN_POINT('Ctrl Pts',(104.234593964868,17.9791818914014,-33.7436393143099));
#76945=CARTESIAN_POINT('Ctrl Pts',(104.195442206095,17.9607714280132,-33.7090862384284));
#76946=CARTESIAN_POINT('Ctrl Pts',(104.192037383127,17.9591199407196,-33.7061082067124));
#76947=CARTESIAN_POINT('Ctrl Pts',(104.188611312035,17.9574059162404,-33.703139419067));
#76948=CARTESIAN_POINT('Origin',(121.7,27.9367711964053,-27.6108081321196));
#76949=CARTESIAN_POINT('',(121.7,28.0515762261148,-27.887971991873));
#76950=CARTESIAN_POINT('Origin',(103.5,13.9679452813258,-33.721602936662));
#76951=CARTESIAN_POINT('',(104.3,30.185459702598,-27.0040885153898));
#76952=CARTESIAN_POINT('Origin',(104.3,30.0706546728884,-26.7269246556364));
#76953=CARTESIAN_POINT('Origin',(104.3,0.,0.));
#76954=CARTESIAN_POINT('Origin',(104.087867965644,-2.22044604925031E-15,
-2.22044604925031E-15));
#76955=CARTESIAN_POINT('Origin',(104.3,32.35,-23.1228782810445));
#76956=CARTESIAN_POINT('Origin',(104.3,33.9959446585896,-19.5430955687966));
#76957=CARTESIAN_POINT('Origin',(113.,25.7740421742496,-27.6125198053347));
#76958=CARTESIAN_POINT('',(121.7,24.8901586977665,-26.7286363288515));
#76959=CARTESIAN_POINT('',(103.5,24.8901586977665,-26.7286363288515));
#76960=CARTESIAN_POINT('Origin',(121.7,24.6780266634105,-26.5165042944955));
#76961=CARTESIAN_POINT('',(121.75,26.1119693309588,-27.9504469620439));
#76962=CARTESIAN_POINT('Origin',(113.,29.3054840759098,-24.5036446896497));
#76963=CARTESIAN_POINT('',(104.5,29.5356318566107,-24.6960816898302));
#76964=CARTESIAN_POINT('',(113.,29.5356318566107,-24.6960816898302));
#76965=CARTESIAN_POINT('Ctrl Pts',(104.5,29.5356318566107,-24.6960816898302));
#76966=CARTESIAN_POINT('Ctrl Pts',(104.5,29.5489700413278,-24.6801296971867));
#76967=CARTESIAN_POINT('Ctrl Pts',(104.497821708252,29.5607352354492,-24.6626361343801));
#76968=CARTESIAN_POINT('Ctrl Pts',(104.489283385678,29.5802270436011,-24.625911536016));
#76969=CARTESIAN_POINT('Ctrl Pts',(104.482922171696,29.5879524700494,-24.6066801452406));
#76970=CARTESIAN_POINT('Ctrl Pts',(104.458840813878,29.6047939634926,-24.5487264875151));
#76971=CARTESIAN_POINT('Ctrl Pts',(104.43587220677,29.6073422778058,-24.509633504542));
#76972=CARTESIAN_POINT('Ctrl Pts',(104.382711610234,29.6003545473748,-24.4346560851191));
#76973=CARTESIAN_POINT('Ctrl Pts',(104.347490784093,29.5877605876801,-24.3945623020959));
#76974=CARTESIAN_POINT('Ctrl Pts',(104.273440501065,29.5494817883985,-24.3245682087704));
#76975=CARTESIAN_POINT('Ctrl Pts',(104.234593964868,29.5237298740531,-24.2947226776164));
#76976=CARTESIAN_POINT('Ctrl Pts',(104.195442206095,29.4934979340675,-24.2698451773449));
#76977=CARTESIAN_POINT('Ctrl Pts',(104.192037383127,29.49083251536,-24.2677258316214));
#76978=CARTESIAN_POINT('Ctrl Pts',(104.188611312035,29.4881128573793,-24.2656389582503));
#76979=CARTESIAN_POINT('Origin',(121.7,33.847265478953,-17.347265478953));
#76980=CARTESIAN_POINT('',(121.7,34.059397513309,-17.559397513309));
#76981=CARTESIAN_POINT('Origin',(103.5,25.809397513309,-25.809397513309));
#76982=CARTESIAN_POINT('',(104.3,35.309397513309,-16.309397513309));
#76983=CARTESIAN_POINT('Origin',(104.3,35.097265478953,-16.097265478953));
#76984=CARTESIAN_POINT('Origin',(104.3,0.,0.));
#76985=CARTESIAN_POINT('Origin',(104.087867965644,-2.22044604925031E-15,
-2.22044604925031E-15));
#76986=CARTESIAN_POINT('Origin',(104.3,35.7606099900688,-12.8608683803695));
#76987=CARTESIAN_POINT('Origin',(104.3,36.1001196169967,-9.87275866404784));
#76988=CARTESIAN_POINT('Origin',(113.,36.4518757833582,-11.4236925674066));
#76989=CARTESIAN_POINT('',(104.5,36.7381470591438,-11.5134074305014));
#76990=CARTESIAN_POINT('',(113.,36.7381470591438,-11.5134074305014));
#76991=CARTESIAN_POINT('Ctrl Pts',(104.5,36.7381470591438,-11.5134074305014));
#76992=CARTESIAN_POINT('Ctrl Pts',(104.5,36.7443653717069,-11.4935654086862));
#76993=CARTESIAN_POINT('Ctrl Pts',(104.497821708253,36.7485404970926,-11.4729011191897));
#76994=CARTESIAN_POINT('Ctrl Pts',(104.489283385678,36.7524946843416,-11.4315128223748));
#76995=CARTESIAN_POINT('Ctrl Pts',(104.482922171696,36.7522725130859,-11.410788941346));
#76996=CARTESIAN_POINT('Ctrl Pts',(104.458840813878,36.7456541195185,-11.3508017826223));
#76997=CARTESIAN_POINT('Ctrl Pts',(104.43587220677,36.7330482180494,-11.3137093781205));
#76998=CARTESIAN_POINT('Ctrl Pts',(104.382711610234,36.6978997807109,-11.2471133635809));
#76999=CARTESIAN_POINT('Ctrl Pts',(104.347490784093,36.6709212526118,-11.2148910377879));
#77000=CARTESIAN_POINT('Ctrl Pts',(104.273440501065,36.6087706735473,-11.1648735898636));
#77001=CARTESIAN_POINT('Ctrl Pts',(104.234593964868,36.5735576166579,-11.1471547454652));
#77002=CARTESIAN_POINT('Ctrl Pts',(104.195442206095,36.5361067388845,-11.1357401947051));
#77003=CARTESIAN_POINT('Ctrl Pts',(104.192037383127,36.5328331745992,-11.1348021861485));
#77004=CARTESIAN_POINT('Ctrl Pts',(104.188611312035,36.5295219263909,-11.1339149346049));
#77005=CARTESIAN_POINT('Origin',(121.7,35.8608081321196,-8.01950930682725));
#77006=CARTESIAN_POINT('',(121.7,36.137971991873,-8.13431433653678));
#77007=CARTESIAN_POINT('Origin',(103.5,33.721602936662,-13.9679452813258));
#77008=CARTESIAN_POINT('',(104.3,36.5040885153898,-7.25043086005359));
#77009=CARTESIAN_POINT('Origin',(104.3,36.2269246556364,-7.13562583034406));
#77010=CARTESIAN_POINT('Origin',(104.3,0.,0.));
#77011=CARTESIAN_POINT('Origin',(104.087867965644,-2.22044604925031E-15,
-3.33066907387547E-15));
#77012=CARTESIAN_POINT('Origin',(104.3,36.2392735757121,-4.61924943271127));
#77013=CARTESIAN_POINT('Origin',(104.3,0.,0.));
#77014=CARTESIAN_POINT('Ctrl Pts',(104.,37.3598942576647,-6.22974103737681));
#77015=CARTESIAN_POINT('Ctrl Pts',(104.,37.3966300490656,-6.23457739606559));
#77016=CARTESIAN_POINT('Ctrl Pts',(104.008670719845,37.439866676382,-6.24026960603904));
#77017=CARTESIAN_POINT('Ctrl Pts',(104.037012788768,37.5077282445796,-6.24920375098245));
#77018=CARTESIAN_POINT('Ctrl Pts',(104.061688713442,37.5443644242305,-6.25402699553555));
#77019=CARTESIAN_POINT('Ctrl Pts',(104.087868240379,37.570335046313,-6.25744609279661));
#77020=CARTESIAN_POINT('Origin',(113.,37.2573594669753,-6.21624207609294));
#77021=CARTESIAN_POINT('',(121.811388243054,37.6702738824291,-6.27060329017727));
#77022=CARTESIAN_POINT('',(121.75,37.7311721243447,-6.27862069582415));
#77023=CARTESIAN_POINT('',(113.,37.6702738824291,-6.27060329017727));
#77024=CARTESIAN_POINT('',(104.3,36.018053390258,-6.05308433581787));
#77025=CARTESIAN_POINT('Origin',(104.3,35.7206199318459,-6.01392647815186));
#77026=CARTESIAN_POINT('',(121.7,36.018053390258,-6.05308433581787));
#77027=CARTESIAN_POINT('',(103.5,36.018053390258,-6.05308433581787));
#77028=CARTESIAN_POINT('Origin',(121.7,35.7206199318459,-6.01392647815186));
#77029=CARTESIAN_POINT('Origin',(121.7,36.1714159148471,-2.58979103627009));
#77030=CARTESIAN_POINT('',(121.7,36.4688493732593,-2.62894889393611));
#77031=CARTESIAN_POINT('Origin',(103.5,36.1877374401441,-4.76420601603192));
#77032=CARTESIAN_POINT('',(104.3,36.5114420903979,-2.30542508755795));
#77033=CARTESIAN_POINT('Origin',(104.3,36.2140086319858,-2.26626722989194));
#77034=CARTESIAN_POINT('Origin',(113.,37.6311160247631,-6.56803674858941));
#77035=CARTESIAN_POINT('',(121.5,37.9266483495649,-6.61961818902336));
#77036=CARTESIAN_POINT('Ctrl Pts',(121.811388687965,37.6702743232782,-6.27060334821649));
#77037=CARTESIAN_POINT('Ctrl Pts',(121.807962616873,37.6736730528646,-6.27105080458));
#77038=CARTESIAN_POINT('Ctrl Pts',(121.804557793905,37.6770410460387,-6.27155350246224));
#77039=CARTESIAN_POINT('Ctrl Pts',(121.765406035132,37.7156614242077,-6.27798207968718));
#77040=CARTESIAN_POINT('Ctrl Pts',(121.726559498935,37.7528860018039,-6.29095311068326));
#77041=CARTESIAN_POINT('Ctrl Pts',(121.652509215907,37.8210334610709,-6.33243037397719));
#77042=CARTESIAN_POINT('Ctrl Pts',(121.617288389766,37.8519870416124,-6.36085562876174));
#77043=CARTESIAN_POINT('Ctrl Pts',(121.56412779323,37.8955273033918,-6.42229411347671));
#77044=CARTESIAN_POINT('Ctrl Pts',(121.541159186122,37.9128668899463,-6.45742378699774));
#77045=CARTESIAN_POINT('Ctrl Pts',(121.517077828304,37.9272585576496,-6.51603387355182));
#77046=CARTESIAN_POINT('Ctrl Pts',(121.510716614322,37.930183837478,-6.53655145973756));
#77047=CARTESIAN_POINT('Ctrl Pts',(121.502178291748,37.9316657356348,-6.5781017989406));
#77048=CARTESIAN_POINT('Ctrl Pts',(121.5,37.9302235600485,-6.59913426579454));
#77049=CARTESIAN_POINT('Ctrl Pts',(121.5,37.9266483495649,-6.61961818902336));
#77050=CARTESIAN_POINT('',(113.,37.9266483495649,-6.61961818902336));
#77051=CARTESIAN_POINT('Origin',(121.75,0.,0.));
#77052=CARTESIAN_POINT('Origin',(121.5,0.,0.));
#77053=CARTESIAN_POINT('Origin',(113.,0.,0.));
#77054=CARTESIAN_POINT('Origin',(104.25,0.,0.));
#77055=CARTESIAN_POINT('Origin',(104.5,0.,0.));
#77056=CARTESIAN_POINT('Origin',(113.,0.,0.));
#77057=CARTESIAN_POINT('Origin',(121.75,0.,0.));
#77058=CARTESIAN_POINT('Origin',(121.75,0.,0.));
#77059=CARTESIAN_POINT('Origin',(104.25,0.,0.));
#77060=CARTESIAN_POINT('Origin',(104.5,0.,0.));
#77061=CARTESIAN_POINT('Origin',(113.,0.,0.));
#77062=CARTESIAN_POINT('Origin',(121.75,0.,0.));
#77063=CARTESIAN_POINT('Origin',(121.75,0.,0.));
#77064=CARTESIAN_POINT('Origin',(104.25,0.,0.));
#77065=CARTESIAN_POINT('Origin',(104.5,0.,0.));
#77066=CARTESIAN_POINT('Origin',(113.,0.,0.));
#77067=CARTESIAN_POINT('Origin',(121.75,0.,0.));
#77068=CARTESIAN_POINT('Origin',(121.75,0.,0.));
#77069=CARTESIAN_POINT('Origin',(104.25,0.,0.));
#77070=CARTESIAN_POINT('Origin',(121.75,0.,0.));
#77071=CARTESIAN_POINT('Origin',(121.75,0.,0.));
#77072=CARTESIAN_POINT('Origin',(104.25,0.,0.));
#77073=CARTESIAN_POINT('Origin',(104.5,0.,0.));
#77074=CARTESIAN_POINT('Origin',(113.,0.,0.));
#77075=CARTESIAN_POINT('Origin',(121.75,0.,0.));
#77076=CARTESIAN_POINT('Origin',(121.75,0.,0.));
#77077=CARTESIAN_POINT('Origin',(104.25,0.,0.));
#77078=CARTESIAN_POINT('Origin',(104.5,0.,0.));
#77079=CARTESIAN_POINT('Origin',(113.,0.,0.));
#77080=CARTESIAN_POINT('Origin',(121.75,0.,0.));
#77081=CARTESIAN_POINT('Origin',(121.75,0.,0.));
#77082=CARTESIAN_POINT('Origin',(104.25,0.,0.));
#77083=CARTESIAN_POINT('Origin',(104.5,0.,0.));
#77084=CARTESIAN_POINT('Origin',(113.,0.,0.));
#77085=CARTESIAN_POINT('Origin',(121.75,0.,0.));
#77086=CARTESIAN_POINT('Origin',(121.75,0.,0.));
#77087=CARTESIAN_POINT('Origin',(104.25,0.,0.));
#77088=CARTESIAN_POINT('Origin',(121.75,0.,0.));
#77089=CARTESIAN_POINT('Origin',(121.75,0.,0.));
#77090=CARTESIAN_POINT('Origin',(104.25,0.,0.));
#77091=CARTESIAN_POINT('Origin',(104.5,0.,0.));
#77092=CARTESIAN_POINT('Origin',(113.,0.,0.));
#77093=CARTESIAN_POINT('Origin',(121.75,0.,0.));
#77094=CARTESIAN_POINT('Origin',(121.75,0.,0.));
#77095=CARTESIAN_POINT('Origin',(104.25,0.,0.));
#77096=CARTESIAN_POINT('Origin',(104.5,0.,0.));
#77097=CARTESIAN_POINT('Origin',(113.,0.,0.));
#77098=CARTESIAN_POINT('Origin',(121.75,0.,0.));
#77099=CARTESIAN_POINT('Origin',(121.75,0.,0.));
#77100=CARTESIAN_POINT('Origin',(104.25,0.,0.));
#77101=CARTESIAN_POINT('Origin',(104.5,0.,0.));
#77102=CARTESIAN_POINT('Origin',(113.,0.,0.));
#77103=CARTESIAN_POINT('Origin',(121.75,0.,0.));
#77104=CARTESIAN_POINT('Origin',(121.75,0.,0.));
#77105=CARTESIAN_POINT('Origin',(104.25,0.,0.));
#77106=CARTESIAN_POINT('Origin',(121.75,0.,0.));
#77107=CARTESIAN_POINT('Origin',(121.75,0.,0.));
#77108=CARTESIAN_POINT('Origin',(104.25,0.,0.));
#77109=CARTESIAN_POINT('Origin',(104.5,0.,0.));
#77110=CARTESIAN_POINT('Origin',(113.,0.,0.));
#77111=CARTESIAN_POINT('Origin',(121.75,0.,0.));
#77112=CARTESIAN_POINT('Origin',(121.75,0.,0.));
#77113=CARTESIAN_POINT('Origin',(104.25,0.,0.));
#77114=CARTESIAN_POINT('Origin',(104.5,0.,0.));
#77115=CARTESIAN_POINT('Origin',(113.,0.,0.));
#77116=CARTESIAN_POINT('Origin',(121.75,0.,0.));
#77117=CARTESIAN_POINT('Origin',(121.75,0.,0.));
#77118=CARTESIAN_POINT('Origin',(104.25,0.,0.));
#77119=CARTESIAN_POINT('Origin',(104.5,0.,0.));
#77120=CARTESIAN_POINT('Origin',(113.,0.,0.));
#77121=CARTESIAN_POINT('Origin',(113.,36.127235183779,11.0261225267959));
#77122=CARTESIAN_POINT('Origin',(113.,37.2573594669753,6.2162420760929));
#77123=CARTESIAN_POINT('Origin',(121.75,0.,0.));
#77124=CARTESIAN_POINT('',(121.75,38.2279011681123,-1.3));
#77125=CARTESIAN_POINT('Origin',(113.,37.75,-1.3));
#90339=UNCERTAINTY_MEASURE_WITH_UNIT(LENGTH_MEASURE(0.01),#90375,
'DISTANCE_ACCURACY_VALUE',
'Maximum model space distance between geometric entities at asserted c
onnectivities');
#90355=UNCERTAINTY_MEASURE_WITH_UNIT(LENGTH_MEASURE(0.01),#90375,
'DISTANCE_ACCURACY_VALUE',
'Maximum model space distance between geometric entities at asserted c
onnectivities');
#90358=(
GEOMETRIC_REPRESENTATION_CONTEXT(3)
GLOBAL_UNCERTAINTY_ASSIGNED_CONTEXT((#90339))
GLOBAL_UNIT_ASSIGNED_CONTEXT((#90375,#90377,#90378))
REPRESENTATION_CONTEXT('','3D')
);
#90374=(
GEOMETRIC_REPRESENTATION_CONTEXT(3)
GLOBAL_UNCERTAINTY_ASSIGNED_CONTEXT((#90355))
GLOBAL_UNIT_ASSIGNED_CONTEXT((#90375,#90377,#90378))
REPRESENTATION_CONTEXT('','3D')
);
#90375=(
LENGTH_UNIT()
NAMED_UNIT(*)
SI_UNIT(.MILLI.,.METRE.)
);
#90377=(
NAMED_UNIT(*)
PLANE_ANGLE_UNIT()
SI_UNIT($,.RADIAN.)
);
#90378=(
NAMED_UNIT(*)
SI_UNIT($,.STERADIAN.)
SOLID_ANGLE_UNIT()
);
#90381=SHAPE_DEFINITION_REPRESENTATION(#90399,#90442);
#90399=PRODUCT_DEFINITION_SHAPE('',$,#90461);
#90442=SHAPE_REPRESENTATION('',(#40904),#90358);
#90458=PRODUCT_DEFINITION_CONTEXT('part definition',#90514,'design');
#90461=PRODUCT_DEFINITION('2026-10-11-12-53-08-361',
'02_ABS_Tone_Ring_48T',#90479,#90458);
#90479=PRODUCT_DEFINITION_FORMATION('',$,#90518);
#90514=APPLICATION_CONTEXT(
'Core Data for Automotive Mechanical Design Process');
#90515=PRODUCT_CONTEXT('part definition',#90514,'mechanical');
#90518=PRODUCT('2026-10-11-12-53-08-361','02_ABS_Tone_Ring_48T',$,(#90515));
#90667=COLOUR_RGB('Light Blue',0.38,0.62,0.78);
#90668=FILL_AREA_STYLE_COLOUR('',#90667);
#90669=FILL_AREA_STYLE('',(#90668));
#90670=SURFACE_STYLE_FILL_AREA(#90669);
#90671=SURFACE_SIDE_STYLE('',(#90670));
#90672=SURFACE_STYLE_USAGE(.BOTH.,#90671);
#90673=PRESENTATION_STYLE_ASSIGNMENT((#90672));
ENDSEC;
END-ISO-10303-21;
